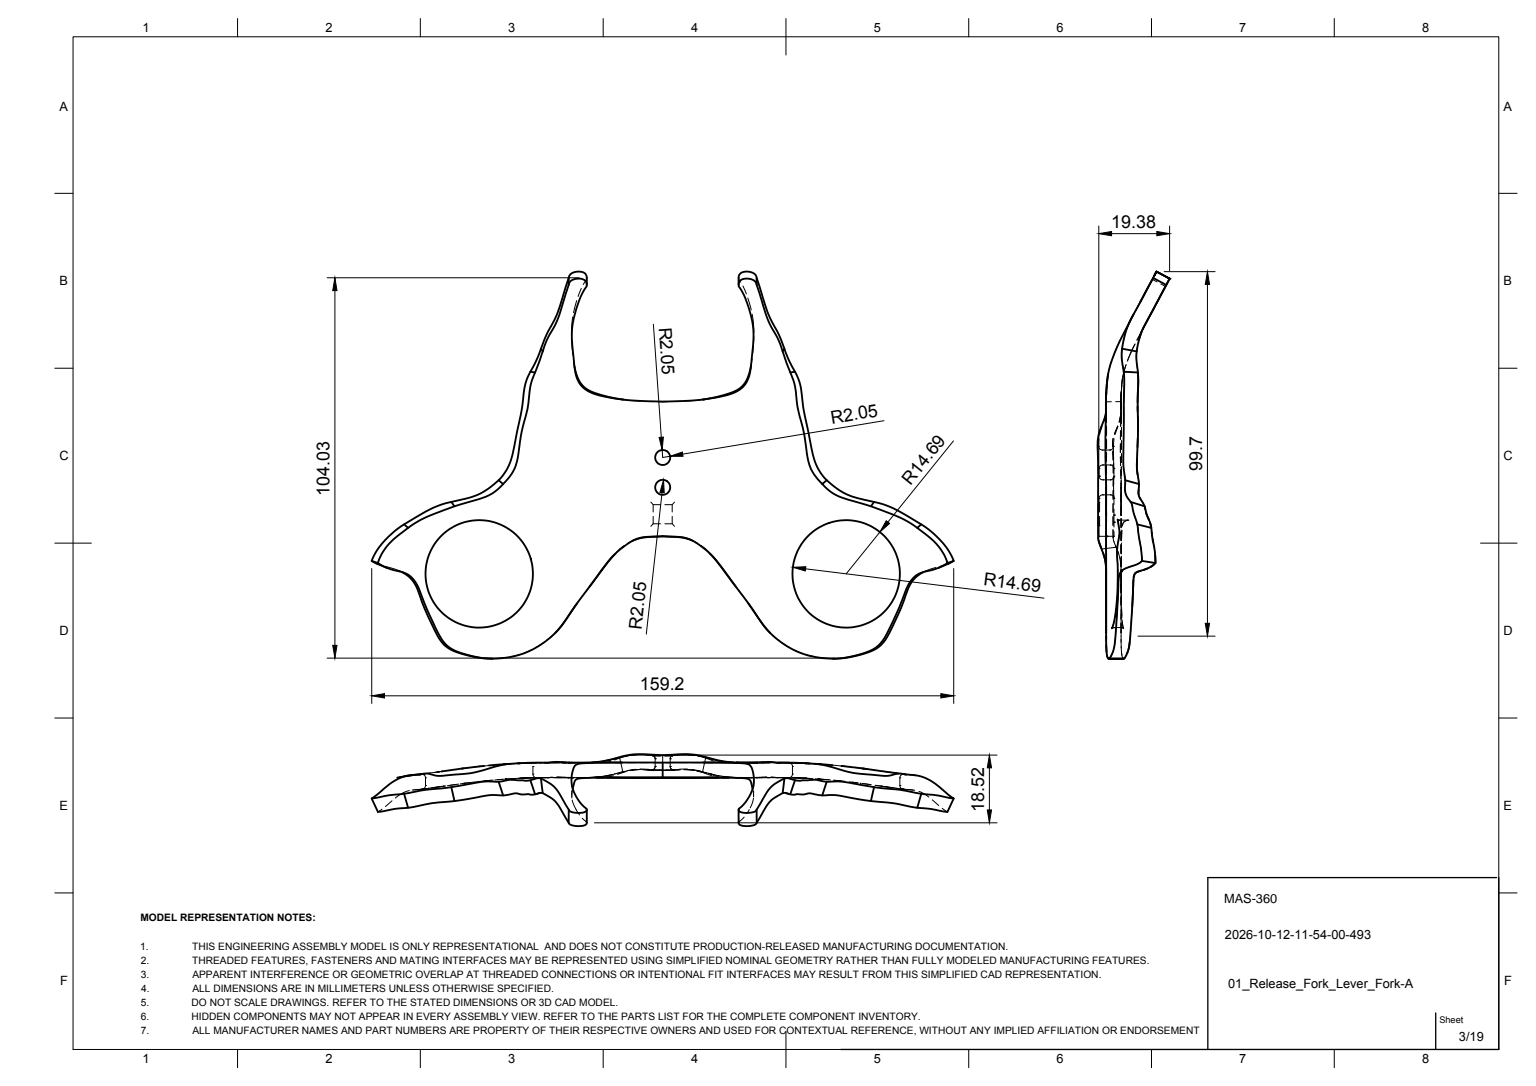
ISO-10303-21;
HEADER;
/* Generated by software containing ST-Developer
 * from STEP Tools, Inc. (www.steptools.com) 
 */

FILE_DESCRIPTION(
/* description */ (''),
/* implementation_level */ '2;1');

FILE_NAME(
/* name */ '01_Release_Fork_Lever_Fork-A.step',
/* time_stamp */ '2026-11-04T18:53:29-08:00',
/* author */ (''),
/* organization */ (''),
/* preprocessor_version */ 'ST-DEVELOPER v20.2',
/* originating_system */ 'Autodesk Translation Framework v15.17.0.0',
/* authorisation */ '');

FILE_SCHEMA (('AUTOMOTIVE_DESIGN { 1 0 10303 214 3 1 1 }'));
ENDSEC;

DATA;
#10=MECHANICAL_DESIGN_GEOMETRIC_PRESENTATION_REPRESENTATION('',(#1327),#100031);
#1291=SHAPE_REPRESENTATION_RELATIONSHIP('SRR','None',#100101,#1309);
#1309=ADVANCED_BREP_SHAPE_REPRESENTATION('',(#1345),#100013);
#1327=STYLED_ITEM('',(#100200),#1345);
#1345=MANIFOLD_SOLID_BREP('Body1',#20117);
#1363=PLANE('',#20342);
#1694=FACE_BOUND('',#6186,.T.);
#1695=FACE_BOUND('',#6187,.T.);
#1696=FACE_BOUND('',#6188,.T.);
#1697=FACE_BOUND('',#6189,.T.);
#1698=FACE_BOUND('',#6190,.T.);
#1699=FACE_BOUND('',#6193,.T.);
#1700=FACE_BOUND('',#6194,.T.);
#1701=FACE_BOUND('',#6195,.T.);
#1702=FACE_BOUND('',#6196,.T.);
#1811=ELLIPSE('',#20337,11.3271425811526,8.17324773003453);
#1812=ELLIPSE('',#20338,11.1453149409752,7.84400958474998);
#1980=LINE('',#28809,#3267);
#1981=LINE('',#55728,#3268);
#1982=LINE('',#56082,#3269);
#1983=LINE('',#56334,#3270);
#1984=LINE('',#56576,#3271);
#1985=LINE('',#56606,#3272);
#1986=LINE('',#56688,#3273);
#1987=LINE('',#56725,#3274);
#1988=LINE('',#56751,#3275);
#1989=LINE('',#56752,#3276);
#1990=LINE('',#56777,#3277);
#1991=LINE('',#56803,#3278);
#1992=LINE('',#56804,#3279);
#1993=LINE('',#56830,#3280);
#1994=LINE('',#56831,#3281);
#1995=LINE('',#56856,#3282);
#1996=LINE('',#56885,#3283);
#1997=LINE('',#56926,#3284);
#1998=LINE('',#56963,#3285);
#1999=LINE('',#56997,#3286);
#2000=LINE('',#56998,#3287);
#2001=LINE('',#57040,#3288);
#2002=LINE('',#57041,#3289);
#2003=LINE('',#57079,#3290);
#2004=LINE('',#57080,#3291);
#2005=LINE('',#57109,#3292);
#2006=LINE('',#57130,#3293);
#2007=LINE('',#57168,#3294);
#2008=LINE('',#57169,#3295);
#2009=LINE('',#57170,#3296);
#2010=LINE('',#57199,#3297);
#2011=LINE('',#57240,#3298);
#2012=LINE('',#57269,#3299);
#2013=LINE('',#57294,#3300);
#2014=LINE('',#57311,#3301);
#2015=LINE('',#57336,#3302);
#2016=LINE('',#57337,#3303);
#2017=LINE('',#57358,#3304);
#2018=LINE('',#57379,#3305);
#2019=LINE('',#57408,#3306);
#2020=LINE('',#57450,#3307);
#2021=LINE('',#57451,#3308);
#2022=LINE('',#57496,#3309);
#2023=LINE('',#57533,#3310);
#2024=LINE('',#57535,#3311);
#2025=LINE('',#57536,#3312);
#2026=LINE('',#57578,#3313);
#2027=LINE('',#57579,#3314);
#2028=LINE('',#57625,#3315);
#2029=LINE('',#57626,#3316);
#2030=LINE('',#57671,#3317);
#2031=LINE('',#57704,#3318);
#2032=LINE('',#57737,#3319);
#2033=LINE('',#57770,#3320);
#2034=LINE('',#57800,#3321);
#2035=LINE('',#57801,#3322);
#2036=LINE('',#57839,#3323);
#2037=LINE('',#57840,#3324);
#2038=LINE('',#57873,#3325);
#2039=LINE('',#57894,#3326);
#2040=LINE('',#57911,#3327);
#2041=LINE('',#57928,#3328);
#2042=LINE('',#57962,#3329);
#2043=LINE('',#57963,#3330);
#2044=LINE('',#57964,#3331);
#2045=LINE('',#58001,#3332);
#2046=LINE('',#58034,#3333);
#2047=LINE('',#58051,#3334);
#2048=LINE('',#58088,#3335);
#2049=LINE('',#58113,#3336);
#2050=LINE('',#58162,#3337);
#2051=LINE('',#58191,#3338);
#2052=LINE('',#58224,#3339);
#2053=LINE('',#58289,#3340);
#2054=LINE('',#58330,#3341);
#2055=LINE('',#58367,#3342);
#2056=LINE('',#58368,#3343);
#2057=LINE('',#58393,#3344);
#2058=LINE('',#58430,#3345);
#2059=LINE('',#58467,#3346);
#2060=LINE('',#58484,#3347);
#2061=LINE('',#58533,#3348);
#2062=LINE('',#58550,#3349);
#2063=LINE('',#58575,#3350);
#2064=LINE('',#58608,#3351);
#2065=LINE('',#58646,#3352);
#2066=LINE('',#58647,#3353);
#2067=LINE('',#58684,#3354);
#2068=LINE('',#58849,#3355);
#2069=LINE('',#59048,#3356);
#3267=VECTOR('',#22531,14.688);
#3268=VECTOR('',#22538,14.688);
#3269=VECTOR('',#22541,2.05);
#3270=VECTOR('',#22544,2.05);
#3271=VECTOR('',#22545,10.);
#3272=VECTOR('',#22546,10.);
#3273=VECTOR('',#22547,10.);
#3274=VECTOR('',#22548,10.);
#3275=VECTOR('',#22551,10.);
#3276=VECTOR('',#22552,10.);
#3277=VECTOR('',#22553,10.);
#3278=VECTOR('',#22554,10.);
#3279=VECTOR('',#22555,10.);
#3280=VECTOR('',#22556,10.);
#3281=VECTOR('',#22557,10.);
#3282=VECTOR('',#22558,10.);
#3283=VECTOR('',#22559,10.);
#3284=VECTOR('',#22560,10.);
#3285=VECTOR('',#22561,10.);
#3286=VECTOR('',#22562,10.);
#3287=VECTOR('',#22563,10.);
#3288=VECTOR('',#22564,10.);
#3289=VECTOR('',#22565,10.);
#3290=VECTOR('',#22566,10.);
#3291=VECTOR('',#22567,10.);
#3292=VECTOR('',#22568,10.);
#3293=VECTOR('',#22569,9.99999999999999);
#3294=VECTOR('',#22570,10.);
#3295=VECTOR('',#22571,10.);
#3296=VECTOR('',#22572,10.);
#3297=VECTOR('',#22573,10.);
#3298=VECTOR('',#22574,9.99999999999999);
#3299=VECTOR('',#22575,10.);
#3300=VECTOR('',#22576,10.);
#3301=VECTOR('',#22577,10.);
#3302=VECTOR('',#22578,9.99999999999999);
#3303=VECTOR('',#22579,10.);
#3304=VECTOR('',#22580,10.);
#3305=VECTOR('',#22581,10.);
#3306=VECTOR('',#22582,10.);
#3307=VECTOR('',#22583,10.);
#3308=VECTOR('',#22584,10.);
#3309=VECTOR('',#22585,10.);
#3310=VECTOR('',#22586,10.);
#3311=VECTOR('',#22587,10.);
#3312=VECTOR('',#22588,10.);
#3313=VECTOR('',#22589,10.);
#3314=VECTOR('',#22590,10.);
#3315=VECTOR('',#22591,10.);
#3316=VECTOR('',#22592,10.);
#3317=VECTOR('',#22593,10.);
#3318=VECTOR('',#22594,10.);
#3319=VECTOR('',#22595,10.);
#3320=VECTOR('',#22596,10.);
#3321=VECTOR('',#22597,10.);
#3322=VECTOR('',#22598,10.);
#3323=VECTOR('',#22599,10.);
#3324=VECTOR('',#22600,10.);
#3325=VECTOR('',#22601,10.);
#3326=VECTOR('',#22602,10.);
#3327=VECTOR('',#22603,10.);
#3328=VECTOR('',#22604,10.);
#3329=VECTOR('',#22605,10.);
#3330=VECTOR('',#22606,10.);
#3331=VECTOR('',#22607,10.);
#3332=VECTOR('',#22608,10.);
#3333=VECTOR('',#22609,10.);
#3334=VECTOR('',#22610,10.);
#3335=VECTOR('',#22611,10.);
#3336=VECTOR('',#22612,10.);
#3337=VECTOR('',#22613,10.);
#3338=VECTOR('',#22614,10.);
#3339=VECTOR('',#22615,10.);
#3340=VECTOR('',#22616,10.);
#3341=VECTOR('',#22617,10.);
#3342=VECTOR('',#22618,10.);
#3343=VECTOR('',#22619,10.);
#3344=VECTOR('',#22620,10.);
#3345=VECTOR('',#22621,10.);
#3346=VECTOR('',#22622,10.);
#3347=VECTOR('',#22623,10.);
#3348=VECTOR('',#22624,10.);
#3349=VECTOR('',#22625,10.);
#3350=VECTOR('',#22626,10.);
#3351=VECTOR('',#22627,10.);
#3352=VECTOR('',#22628,10.);
#3353=VECTOR('',#22629,10.);
#3354=VECTOR('',#22630,10.);
#3355=VECTOR('',#22631,10.);
#3356=VECTOR('',#22632,9.99999999999999);
#4554=CYLINDRICAL_SURFACE('',#20336,14.688);
#4555=CYLINDRICAL_SURFACE('',#20339,14.688);
#4556=CYLINDRICAL_SURFACE('',#20340,2.05);
#4557=CYLINDRICAL_SURFACE('',#20341,2.05);
#5026=FACE_OUTER_BOUND('',#6183,.T.);
#5027=FACE_OUTER_BOUND('',#6184,.T.);
#5028=FACE_OUTER_BOUND('',#6185,.T.);
#5029=FACE_OUTER_BOUND('',#6191,.T.);
#5030=FACE_OUTER_BOUND('',#6192,.T.);
#5031=FACE_OUTER_BOUND('',#6197,.T.);
#5032=FACE_OUTER_BOUND('',#6198,.T.);
#5033=FACE_OUTER_BOUND('',#6199,.T.);
#5034=FACE_OUTER_BOUND('',#6200,.T.);
#5035=FACE_OUTER_BOUND('',#6201,.T.);
#5036=FACE_OUTER_BOUND('',#6202,.T.);
#5037=FACE_OUTER_BOUND('',#6203,.T.);
#5038=FACE_OUTER_BOUND('',#6204,.T.);
#5039=FACE_OUTER_BOUND('',#6205,.T.);
#5040=FACE_OUTER_BOUND('',#6206,.T.);
#5041=FACE_OUTER_BOUND('',#6207,.T.);
#5042=FACE_OUTER_BOUND('',#6208,.T.);
#5043=FACE_OUTER_BOUND('',#6209,.T.);
#5044=FACE_OUTER_BOUND('',#6210,.T.);
#5045=FACE_OUTER_BOUND('',#6211,.T.);
#5046=FACE_OUTER_BOUND('',#6212,.T.);
#5047=FACE_OUTER_BOUND('',#6213,.T.);
#5048=FACE_OUTER_BOUND('',#6214,.T.);
#5049=FACE_OUTER_BOUND('',#6215,.T.);
#5050=FACE_OUTER_BOUND('',#6216,.T.);
#5051=FACE_OUTER_BOUND('',#6217,.T.);
#5052=FACE_OUTER_BOUND('',#6218,.T.);
#5053=FACE_OUTER_BOUND('',#6219,.T.);
#5054=FACE_OUTER_BOUND('',#6220,.T.);
#5055=FACE_OUTER_BOUND('',#6221,.T.);
#5056=FACE_OUTER_BOUND('',#6222,.T.);
#5057=FACE_OUTER_BOUND('',#6223,.T.);
#5058=FACE_OUTER_BOUND('',#6224,.T.);
#5059=FACE_OUTER_BOUND('',#6225,.T.);
#5060=FACE_OUTER_BOUND('',#6226,.T.);
#5061=FACE_OUTER_BOUND('',#6227,.T.);
#5062=FACE_OUTER_BOUND('',#6228,.T.);
#5063=FACE_OUTER_BOUND('',#6229,.T.);
#5064=FACE_OUTER_BOUND('',#6230,.T.);
#5065=FACE_OUTER_BOUND('',#6231,.T.);
#5066=FACE_OUTER_BOUND('',#6232,.T.);
#5067=FACE_OUTER_BOUND('',#6233,.T.);
#5068=FACE_OUTER_BOUND('',#6234,.T.);
#5069=FACE_OUTER_BOUND('',#6235,.T.);
#5070=FACE_OUTER_BOUND('',#6236,.T.);
#5071=FACE_OUTER_BOUND('',#6237,.T.);
#5072=FACE_OUTER_BOUND('',#6238,.T.);
#5073=FACE_OUTER_BOUND('',#6239,.T.);
#5074=FACE_OUTER_BOUND('',#6240,.T.);
#5075=FACE_OUTER_BOUND('',#6241,.T.);
#5076=FACE_OUTER_BOUND('',#6242,.T.);
#5077=FACE_OUTER_BOUND('',#6243,.T.);
#5078=FACE_OUTER_BOUND('',#6244,.T.);
#5079=FACE_OUTER_BOUND('',#6245,.T.);
#5080=FACE_OUTER_BOUND('',#6246,.T.);
#5081=FACE_OUTER_BOUND('',#6247,.T.);
#5082=FACE_OUTER_BOUND('',#6248,.T.);
#5083=FACE_OUTER_BOUND('',#6249,.T.);
#5084=FACE_OUTER_BOUND('',#6250,.T.);
#5085=FACE_OUTER_BOUND('',#6251,.T.);
#5086=FACE_OUTER_BOUND('',#6252,.T.);
#5087=FACE_OUTER_BOUND('',#6253,.T.);
#5088=FACE_OUTER_BOUND('',#6254,.T.);
#5089=FACE_OUTER_BOUND('',#6255,.T.);
#5090=FACE_OUTER_BOUND('',#6256,.T.);
#5091=FACE_OUTER_BOUND('',#6257,.T.);
#5092=FACE_OUTER_BOUND('',#6258,.T.);
#5093=FACE_OUTER_BOUND('',#6259,.T.);
#5094=FACE_OUTER_BOUND('',#6260,.T.);
#5095=FACE_OUTER_BOUND('',#6261,.T.);
#5096=FACE_OUTER_BOUND('',#6262,.T.);
#5097=FACE_OUTER_BOUND('',#6263,.T.);
#5098=FACE_OUTER_BOUND('',#6264,.T.);
#5099=FACE_OUTER_BOUND('',#6265,.T.);
#5100=FACE_OUTER_BOUND('',#6266,.T.);
#5101=FACE_OUTER_BOUND('',#6267,.T.);
#5102=FACE_OUTER_BOUND('',#6268,.T.);
#5103=FACE_OUTER_BOUND('',#6269,.T.);
#5104=FACE_OUTER_BOUND('',#6270,.T.);
#5105=FACE_OUTER_BOUND('',#6271,.T.);
#5106=FACE_OUTER_BOUND('',#6272,.T.);
#5107=FACE_OUTER_BOUND('',#6273,.T.);
#5108=FACE_OUTER_BOUND('',#6274,.T.);
#5109=FACE_OUTER_BOUND('',#6275,.T.);
#5110=FACE_OUTER_BOUND('',#6276,.T.);
#5111=FACE_OUTER_BOUND('',#6277,.T.);
#5112=FACE_OUTER_BOUND('',#6278,.T.);
#6183=EDGE_LOOP('',(#12899,#12900,#12901,#12902,#12903,#12904,#12905,#12906,
#12907,#12908,#12909,#12910,#12911,#12912,#12913));
#6184=EDGE_LOOP('',(#12914,#12915,#12916,#12917,#12918,#12919));
#6185=EDGE_LOOP('',(#12920,#12921,#12922,#12923,#12924,#12925,#12926,#12927,
#12928,#12929,#12930,#12931,#12932,#12933,#12934,#12935,#12936,#12937,#12938,
#12939,#12940,#12941,#12942,#12943,#12944,#12945,#12946,#12947,#12948,#12949,
#12950,#12951,#12952,#12953,#12954,#12955,#12956,#12957,#12958,#12959,#12960,
#12961,#12962,#12963,#12964,#12965,#12966,#12967,#12968,#12969,#12970,#12971,
#12972,#12973,#12974,#12975,#12976,#12977,#12978,#12979,#12980,#12981,#12982,
#12983,#12984,#12985,#12986,#12987));
#6186=EDGE_LOOP('',(#12988,#12989,#12990,#12991,#12992,#12993,#12994,#12995,
#12996,#12997,#12998));
#6187=EDGE_LOOP('',(#12999,#13000,#13001));
#6188=EDGE_LOOP('',(#13002,#13003,#13004,#13005,#13006,#13007,#13008,#13009,
#13010,#13011));
#6189=EDGE_LOOP('',(#13012,#13013,#13014));
#6190=EDGE_LOOP('',(#13015,#13016,#13017,#13018,#13019,#13020,#13021,#13022,
#13023,#13024,#13025));
#6191=EDGE_LOOP('',(#13026,#13027,#13028,#13029,#13030,#13031,#13032,#13033,
#13034,#13035,#13036,#13037,#13038,#13039,#13040));
#6192=EDGE_LOOP('',(#13041,#13042,#13043,#13044,#13045,#13046,#13047,#13048,
#13049,#13050,#13051,#13052,#13053,#13054,#13055,#13056,#13057,#13058,#13059,
#13060,#13061,#13062,#13063,#13064,#13065,#13066,#13067,#13068,#13069,#13070,
#13071,#13072,#13073,#13074,#13075,#13076,#13077,#13078,#13079,#13080,#13081,
#13082,#13083,#13084,#13085,#13086,#13087,#13088,#13089,#13090,#13091,#13092,
#13093,#13094,#13095,#13096,#13097,#13098,#13099,#13100,#13101,#13102,#13103,
#13104,#13105,#13106,#13107,#13108));
#6193=EDGE_LOOP('',(#13109,#13110,#13111,#13112,#13113,#13114,#13115,#13116,
#13117,#13118,#13119));
#6194=EDGE_LOOP('',(#13120,#13121,#13122));
#6195=EDGE_LOOP('',(#13123,#13124,#13125));
#6196=EDGE_LOOP('',(#13126,#13127,#13128,#13129,#13130,#13131,#13132,#13133,
#13134,#13135,#13136));
#6197=EDGE_LOOP('',(#13137,#13138,#13139,#13140,#13141,#13142,#13143,#13144,
#13145,#13146,#13147,#13148,#13149,#13150,#13151));
#6198=EDGE_LOOP('',(#13152,#13153,#13154,#13155,#13156,#13157));
#6199=EDGE_LOOP('',(#13158,#13159,#13160,#13161,#13162,#13163,#13164,#13165,
#13166,#13167,#13168,#13169,#13170,#13171,#13172));
#6200=EDGE_LOOP('',(#13173,#13174,#13175,#13176,#13177,#13178,#13179));
#6201=EDGE_LOOP('',(#13180,#13181,#13182,#13183,#13184,#13185));
#6202=EDGE_LOOP('',(#13186,#13187,#13188,#13189,#13190,#13191,#13192));
#6203=EDGE_LOOP('',(#13193,#13194,#13195,#13196,#13197,#13198,#13199));
#6204=EDGE_LOOP('',(#13200,#13201,#13202,#13203,#13204,#13205));
#6205=EDGE_LOOP('',(#13206,#13207,#13208,#13209,#13210,#13211,#13212));
#6206=EDGE_LOOP('',(#13213,#13214,#13215,#13216));
#6207=EDGE_LOOP('',(#13217,#13218,#13219,#13220,#13221));
#6208=EDGE_LOOP('',(#13222,#13223,#13224,#13225,#13226));
#6209=EDGE_LOOP('',(#13227,#13228,#13229,#13230,#13231,#13232,#13233,#13234));
#6210=EDGE_LOOP('',(#13235,#13236,#13237,#13238));
#6211=EDGE_LOOP('',(#13239,#13240,#13241,#13242));
#6212=EDGE_LOOP('',(#13243,#13244,#13245,#13246));
#6213=EDGE_LOOP('',(#13247,#13248,#13249,#13250,#13251));
#6214=EDGE_LOOP('',(#13252,#13253,#13254,#13255,#13256,#13257));
#6215=EDGE_LOOP('',(#13258,#13259,#13260,#13261,#13262));
#6216=EDGE_LOOP('',(#13263,#13264,#13265,#13266));
#6217=EDGE_LOOP('',(#13267,#13268,#13269,#13270));
#6218=EDGE_LOOP('',(#13271,#13272,#13273,#13274));
#6219=EDGE_LOOP('',(#13275,#13276,#13277,#13278,#13279));
#6220=EDGE_LOOP('',(#13280,#13281,#13282,#13283,#13284,#13285));
#6221=EDGE_LOOP('',(#13286,#13287,#13288,#13289,#13290,#13291));
#6222=EDGE_LOOP('',(#13292,#13293,#13294,#13295,#13296));
#6223=EDGE_LOOP('',(#13297,#13298,#13299,#13300));
#6224=EDGE_LOOP('',(#13301,#13302,#13303,#13304,#13305));
#6225=EDGE_LOOP('',(#13306,#13307,#13308,#13309));
#6226=EDGE_LOOP('',(#13310,#13311,#13312,#13313));
#6227=EDGE_LOOP('',(#13314,#13315,#13316,#13317));
#6228=EDGE_LOOP('',(#13318,#13319,#13320,#13321));
#6229=EDGE_LOOP('',(#13322,#13323,#13324,#13325));
#6230=EDGE_LOOP('',(#13326,#13327,#13328,#13329));
#6231=EDGE_LOOP('',(#13330,#13331,#13332,#13333));
#6232=EDGE_LOOP('',(#13334,#13335,#13336,#13337));
#6233=EDGE_LOOP('',(#13338,#13339,#13340,#13341));
#6234=EDGE_LOOP('',(#13342,#13343,#13344,#13345,#13346));
#6235=EDGE_LOOP('',(#13347,#13348,#13349,#13350,#13351));
#6236=EDGE_LOOP('',(#13352,#13353,#13354,#13355,#13356));
#6237=EDGE_LOOP('',(#13357,#13358,#13359,#13360,#13361,#13362));
#6238=EDGE_LOOP('',(#13363,#13364,#13365,#13366,#13367,#13368));
#6239=EDGE_LOOP('',(#13369,#13370,#13371,#13372,#13373));
#6240=EDGE_LOOP('',(#13374,#13375,#13376,#13377));
#6241=EDGE_LOOP('',(#13378,#13379,#13380,#13381));
#6242=EDGE_LOOP('',(#13382,#13383,#13384,#13385));
#6243=EDGE_LOOP('',(#13386,#13387,#13388,#13389,#13390));
#6244=EDGE_LOOP('',(#13391,#13392,#13393,#13394,#13395,#13396));
#6245=EDGE_LOOP('',(#13397,#13398,#13399,#13400,#13401));
#6246=EDGE_LOOP('',(#13402,#13403,#13404,#13405));
#6247=EDGE_LOOP('',(#13406,#13407,#13408,#13409));
#6248=EDGE_LOOP('',(#13410,#13411,#13412,#13413));
#6249=EDGE_LOOP('',(#13414,#13415,#13416,#13417,#13418));
#6250=EDGE_LOOP('',(#13419,#13420,#13421,#13422));
#6251=EDGE_LOOP('',(#13423,#13424,#13425,#13426));
#6252=EDGE_LOOP('',(#13427,#13428,#13429,#13430));
#6253=EDGE_LOOP('',(#13431,#13432,#13433,#13434));
#6254=EDGE_LOOP('',(#13435,#13436,#13437,#13438));
#6255=EDGE_LOOP('',(#13439,#13440,#13441,#13442));
#6256=EDGE_LOOP('',(#13443,#13444,#13445,#13446));
#6257=EDGE_LOOP('',(#13447,#13448,#13449,#13450));
#6258=EDGE_LOOP('',(#13451,#13452,#13453,#13454));
#6259=EDGE_LOOP('',(#13455,#13456,#13457,#13458));
#6260=EDGE_LOOP('',(#13459,#13460,#13461,#13462));
#6261=EDGE_LOOP('',(#13463,#13464,#13465,#13466));
#6262=EDGE_LOOP('',(#13467,#13468,#13469,#13470));
#6263=EDGE_LOOP('',(#13471,#13472,#13473,#13474));
#6264=EDGE_LOOP('',(#13475,#13476,#13477,#13478));
#6265=EDGE_LOOP('',(#13479,#13480,#13481,#13482));
#6266=EDGE_LOOP('',(#13483,#13484,#13485,#13486));
#6267=EDGE_LOOP('',(#13487,#13488,#13489,#13490));
#6268=EDGE_LOOP('',(#13491,#13492,#13493,#13494));
#6269=EDGE_LOOP('',(#13495,#13496,#13497,#13498,#13499));
#6270=EDGE_LOOP('',(#13500,#13501,#13502,#13503,#13504));
#6271=EDGE_LOOP('',(#13505,#13506,#13507,#13508));
#6272=EDGE_LOOP('',(#13509,#13510,#13511,#13512,#13513));
#6273=EDGE_LOOP('',(#13514,#13515,#13516,#13517));
#6274=EDGE_LOOP('',(#13518,#13519,#13520,#13521));
#6275=EDGE_LOOP('',(#13522,#13523,#13524,#13525));
#6276=EDGE_LOOP('',(#13526,#13527,#13528,#13529,#13530));
#6277=EDGE_LOOP('',(#13531,#13532,#13533,#13534));
#6278=EDGE_LOOP('',(#13535,#13536,#13537,#13538));
#7457=B_SPLINE_CURVE_WITH_KNOTS('',3,(#28468,#28469,#28470,#28471,#28472,
#28473),.UNSPECIFIED.,.F.,.F.,(4,1,1,4),(-0.999999999999995,-0.571428571428571,
-0.285714285714286,0.),.UNSPECIFIED.);
#7458=B_SPLINE_CURVE_WITH_KNOTS('',3,(#28475,#28476,#28477,#28478,#28479,
#28480,#28481,#28482),.UNSPECIFIED.,.F.,.F.,(4,2,2,4),(-13.0076216717983,
-12.6762562420903,-11.8531689108674,-11.7197155434785),.UNSPECIFIED.);
#7459=B_SPLINE_CURVE_WITH_KNOTS('',3,(#28483,#28484,#28485,#28486,#28487,
#28488,#28489,#28490,#28491,#28492,#28493,#28494,#28495,#28496,#28497,#28498,
#28499,#28500,#28501,#28502,#28503,#28504,#28505,#28506,#28507,#28508,#28509,
#28510,#28511,#28512,#28513,#28514,#28515,#28516,#28517,#28518,#28519,#28520,
#28521,#28522,#28523),.UNSPECIFIED.,.F.,.F.,(4,2,2,1,1,2,2,1,2,1,1,1,2,
1,1,1,2,1,1,1,1,1,1,1,1,1,1,2,1,1,4),(-11.7197155434785,-11.05258106389,
-10.1188927640438,-8.47830334468407,-7.04278760274435,-6.83771392532439,
-5.90055842268743,-5.54885349043522,-5.09666143468238,-4.98988621289018,
-4.88311099109797,-4.50939771482526,-4.24245966034475,-3.88978669781647,
-3.67818292029951,-3.43131184652972,-3.11390618025428,-3.0769781504351,
-2.96619406097756,-2.81848194170084,-2.7076978522433,-2.5230577031474,-1.93220922604053,
-1.78449710676381,-1.74756907694463,-1.34136074893366,-1.04593651038022,
-0.750512271826782,-0.60979122085926,-0.469070169891739,0.),
 .UNSPECIFIED.);
#7460=B_SPLINE_CURVE_WITH_KNOTS('',3,(#28525,#28526,#28527,#28528,#28529,
#28530),.UNSPECIFIED.,.F.,.F.,(4,1,1,4),(0.,0.469070169891739,0.60979122085926,
0.750512271826782),.UNSPECIFIED.);
#7461=B_SPLINE_CURVE_WITH_KNOTS('',3,(#28532,#28533,#28534,#28535,#28536,
#28537,#28538,#28539,#28540,#28541,#28542,#28543,#28544,#28545,#28546,#28547,
#28548,#28549,#28550,#28551,#28552,#28553,#28554,#28555,#28556,#28557,#28558,
#28559,#28560,#28561,#28562,#28563,#28564,#28565,#28566,#28567,#28568,#28569,
#28570,#28571,#28572,#28573,#28574,#28575,#28576,#28577,#28578,#28579,#28580,
#28581,#28582,#28583,#28584,#28585,#28586,#28587,#28588,#28589,#28590,#28591,
#28592,#28593,#28594,#28595,#28596,#28597,#28598,#28599,#28600,#28601,#28602,
#28603,#28604,#28605,#28606,#28607,#28608,#28609,#28610,#28611,#28612,#28613,
#28614,#28615,#28616,#28617,#28618,#28619,#28620,#28621,#28622,#28623,#28624,
#28625,#28626,#28627,#28628,#28629,#28630,#28631,#28632,#28633,#28634,#28635,
#28636,#28637,#28638,#28639,#28640,#28641,#28642,#28643,#28644,#28645,#28646,
#28647,#28648,#28649,#28650,#28651,#28652,#28653,#28654,#28655,#28656,#28657,
#28658,#28659,#28660,#28661,#28662,#28663,#28664,#28665,#28666,#28667,#28668,
#28669,#28670,#28671,#28672,#28673,#28674,#28675,#28676,#28677,#28678,#28679,
#28680,#28681,#28682,#28683,#28684,#28685,#28686,#28687,#28688,#28689,#28690,
#28691,#28692,#28693,#28694,#28695,#28696,#28697,#28698,#28699,#28700,#28701,
#28702,#28703,#28704,#28705,#28706),.UNSPECIFIED.,.F.,.F.,(4,3,3,3,3,3,
3,3,3,3,3,3,3,3,3,3,3,3,3,3,3,3,3,3,3,3,3,3,3,3,3,3,3,3,3,3,3,3,3,3,3,3,
3,3,3,3,3,3,3,3,3,3,3,3,3,3,3,3,4),(0.750707263401336,0.751073491522809,
0.770788600839354,0.797141727621928,0.801285493755856,0.847209334720936,
0.851576628686437,0.892702424300306,0.909155014790277,0.945842604423156,
0.959283328964777,0.973653029900114,1.02857295555953,1.04593651038022,1.10213659378528,
1.15946870078418,1.21910603297729,1.25714745759372,1.32249197142089,1.33169604227939,
1.34136074893366,1.40008364166717,1.46200856506941,1.53008670118818,1.60161378753395,
1.67565478609667,1.72643723062008,1.74756907694463,1.78449710676381,1.85969939535229,
1.93220922604053,2.0009848480779,2.06808195029472,2.1044635537539,2.17677612815408,
2.25426089464543,2.33537778995665,2.42383992559276,2.48665348358685,2.5230577031474,
2.55048767867042,2.63206152994388,2.7076978522433,2.81035120800203,2.81848194170084,
2.86928839618313,2.89438186295904,2.94470693815227,2.96619406097756,2.99737852476675,
3.02773642991363,3.05710875945002,3.07552489670663,3.0769781504351,3.08925644295071,
3.10116317170119,3.11177854192958,3.11306990045168,3.11390618025428),
 .UNSPECIFIED.);
#7462=B_SPLINE_CURVE_WITH_KNOTS('',3,(#28708,#28709,#28710,#28711,#28712,
#28713,#28714),.UNSPECIFIED.,.F.,.F.,(4,1,1,1,4),(3.1140516289664,3.43131184652972,
3.67818292029951,3.88978669781647,4.24245966034475),.UNSPECIFIED.);
#7463=B_SPLINE_CURVE_WITH_KNOTS('',3,(#28716,#28717,#28718,#28719,#28720,
#28721,#28722),.UNSPECIFIED.,.F.,.F.,(4,1,1,1,4),(4.24281193045545,4.50939771482526,
4.88311099109797,4.98988621289018,5.09562751764158),.UNSPECIFIED.);
#7464=B_SPLINE_CURVE_WITH_KNOTS('',3,(#28724,#28725,#28726,#28727,#28728,
#28729,#28730,#28731,#28732,#28733,#28734,#28735,#28736,#28737,#28738,#28739,
#28740,#28741,#28742,#28743,#28744,#28745,#28746,#28747,#28748,#28749,#28750,
#28751,#28752,#28753,#28754,#28755,#28756,#28757,#28758,#28759,#28760,#28761,
#28762,#28763,#28764,#28765,#28766,#28767,#28768,#28769,#28770,#28771,#28772,
#28773,#28774,#28775),.UNSPECIFIED.,.F.,.F.,(4,3,3,3,3,3,3,3,3,3,3,3,3,
3,3,3,3,4),(5.09666143468238,5.15433284711348,5.21357578985293,5.27511503720701,
5.34195092279717,5.41296344455248,5.48882370921057,5.4948675217662,5.54885349043522,
5.62257616633349,5.69588741785513,5.71679169498887,5.78286561201951,5.79781169784479,
5.83813276584378,5.84909385748713,5.87479360889014,5.90049336029315),
 .UNSPECIFIED.);
#7465=B_SPLINE_CURVE_WITH_KNOTS('',3,(#28777,#28778,#28779,#28780),
 .UNSPECIFIED.,.F.,.F.,(4,4),(5.90055842268743,6.83750114647945),
 .UNSPECIFIED.);
#7466=B_SPLINE_CURVE_WITH_KNOTS('',3,(#28782,#28783,#28784,#28785,#28786,
#28787),.UNSPECIFIED.,.F.,.F.,(4,1,1,4),(6.83771392532439,7.04278760274435,
8.47830334468407,10.1186669136909),.UNSPECIFIED.);
#7467=B_SPLINE_CURVE_WITH_KNOTS('',3,(#28789,#28790,#28791,#28792),
 .UNSPECIFIED.,.F.,.F.,(4,4),(10.1188927640438,11.05258106389),
 .UNSPECIFIED.);
#7468=B_SPLINE_CURVE_WITH_KNOTS('',3,(#28794,#28795,#28796,#28797),
 .UNSPECIFIED.,.F.,.F.,(4,4),(11.0525853415176,11.8531689108674),
 .UNSPECIFIED.);
#7469=B_SPLINE_CURVE_WITH_KNOTS('',3,(#28799,#28800,#28801,#28802),
 .UNSPECIFIED.,.F.,.F.,(4,4),(11.8532319611187,12.6762562420903),
 .UNSPECIFIED.);
#7470=B_SPLINE_CURVE_WITH_KNOTS('',3,(#28803,#28804,#28805,#28806),
 .UNSPECIFIED.,.F.,.F.,(4,4),(12.6763300349415,13.0076216717983),
 .UNSPECIFIED.);
#7471=B_SPLINE_CURVE_WITH_KNOTS('',3,(#28811,#28812,#28813,#28814,#28815,
#28816,#28817,#28818,#28819,#28820,#28821,#28822,#28823,#28824,#28825,#28826,
#28827,#28828,#28829,#28830,#28831,#28832,#28833,#28834,#28835,#28836,#28837,
#28838,#28839,#28840,#28841,#28842),.UNSPECIFIED.,.F.,.F.,(4,1,1,1,2,1,
1,1,1,2,1,1,1,2,1,1,1,2,2,1,2,2,4),(-9.55960092302324,-9.1896794456085,
-8.81975796819377,-8.44983649077903,-8.0799150133643,-8.03266253512535,
-7.98541005688641,-7.89090510040853,-7.70189518745276,-7.32387536154123,
-7.17881214312514,-7.03374892470906,-6.88868570629297,-6.74362248787689,
-6.67050437063,-6.59738625338311,-6.45115001888933,-6.15867754990177,-5.47160541199434,
-4.26766323501505,-3.06372105803577,-2.37819810334092,-1.88848372186453),
 .UNSPECIFIED.);
#7472=B_SPLINE_CURVE_WITH_KNOTS('',3,(#28843,#28844,#28845,#28846,#28847,
#28848,#28849,#28850,#28851,#28852,#28853,#28854,#28855),.UNSPECIFIED.,
 .F.,.F.,(4,2,2,1,2,1,1,4),(-1.88848372186453,-1.79056374069951,-1.18667868852568,
-0.800342864550781,-0.414007040575882,-0.310505280431912,-0.207003520287941,
0.),.UNSPECIFIED.);
#7473=B_SPLINE_CURVE_WITH_KNOTS('',3,(#38650,#38651,#38652,#38653,#38654,
#38655,#38656,#38657,#38658),.UNSPECIFIED.,.F.,.F.,(4,1,1,1,1,1,4),(0.,
0.208981284264062,0.626943852792187,0.835925137056249,1.04490642132031,
1.25388770558437,1.46286898984844),.UNSPECIFIED.);
#7474=B_SPLINE_CURVE_WITH_KNOTS('',3,(#38660,#38661,#38662,#38663,#38664,
#38665,#38666,#38667,#38668),.UNSPECIFIED.,.F.,.F.,(4,1,1,1,1,1,4),(1.46286898984844,
1.57811142102339,1.80859628337331,1.92383871454827,2.03908114572322,2.15432357689818,
2.26956600807314),.UNSPECIFIED.);
#7475=B_SPLINE_CURVE_WITH_KNOTS('',3,(#38670,#38671,#38672,#38673,#38674,
#38675,#38676,#38677,#38678,#38679,#38680,#38681,#38682,#38683,#38684,#38685,
#38686,#38687,#38688,#38689,#38690,#38691,#38692,#38693,#38694,#38695,#38696,
#38697,#38698,#38699,#38700,#38701,#38702,#38703,#38704,#38705,#38706,#38707,
#38708,#38709,#38710,#38711,#38712,#38713,#38714,#38715,#38716,#38717,#38718,
#38719,#38720,#38721,#38722,#38723,#38724,#38725,#38726,#38727,#38728,#38729,
#38730,#38731,#38732,#38733,#38734,#38735,#38736,#38737,#38738,#38739,#38740,
#38741,#38742,#38743,#38744,#38745,#38746,#38747,#38748,#38749,#38750,#38751,
#38752,#38753,#38754,#38755,#38756,#38757,#38758,#38759,#38760,#38761,#38762,
#38763),.UNSPECIFIED.,.F.,.F.,(4,3,3,3,3,3,3,3,3,3,3,3,3,3,3,3,3,3,3,3,
3,3,3,3,3,3,3,3,3,3,3,4),(2.26956600807314,2.31868576460897,2.36442460789209,
2.40351503906262,2.42718620051329,2.44122087175842,2.44260547023316,2.45341326627912,
2.46020489685124,2.46598765674336,2.4975277476721,2.51361070216978,2.52906783860085,
2.54765629078654,2.56502674195218,2.57656452038008,2.61240308621125,2.61582222590599,
2.62445098833827,2.62880283765034,2.63139315501457,2.63314063742138,2.65910316373393,
2.6848523253642,2.7024591242981,2.70904066964155,2.74512184182599,2.77027473318896,
2.78990851485099,2.83207741398362,2.86861528379491,2.87518401914012),
 .UNSPECIFIED.);
#7476=B_SPLINE_CURVE_WITH_KNOTS('',3,(#38765,#38766,#38767,#38768,#38769,
#38770,#38771,#38772,#38773,#38774),.UNSPECIFIED.,.F.,.F.,(4,2,2,2,4),(7.35574899264912E-13,
0.182950620511092,0.366672640482893,0.532787709398147,0.700945883028127),
 .UNSPECIFIED.);
#7477=B_SPLINE_CURVE_WITH_KNOTS('',3,(#38776,#38777,#38778,#38779,#38780,
#38781),.UNSPECIFIED.,.F.,.F.,(4,2,4),(0.,0.425557203103372,0.889753425869099),
 .UNSPECIFIED.);
#7478=B_SPLINE_CURVE_WITH_KNOTS('',3,(#38783,#38784,#38785,#38786,#38787,
#38788,#38789,#38790,#38791,#38792,#38793,#38794),.UNSPECIFIED.,.F.,.F.,
(4,1,1,1,1,1,1,1,1,4),(4.48918216137468,4.66429138725693,4.75184600019805,
4.83940061313917,5.53983751666817,5.89005596843266,6.06516519431491,6.24027442019716,
6.59049287196166,6.94071132372615),.UNSPECIFIED.);
#7479=B_SPLINE_CURVE_WITH_KNOTS('',3,(#38796,#38797,#38798,#38799),
 .UNSPECIFIED.,.F.,.F.,(4,4),(6.94071132372615,7.92790045161141),
 .UNSPECIFIED.);
#7480=B_SPLINE_CURVE_WITH_KNOTS('',3,(#38801,#38802,#38803,#38804,#38805,
#38806,#38807,#38808,#38809),.UNSPECIFIED.,.F.,.F.,(4,1,1,1,1,1,4),(7.92790045161141,
8.77117777664964,9.19281643916875,9.61445510168786,10.036093764207,10.4577324267261,
10.8793710892452),.UNSPECIFIED.);
#7481=B_SPLINE_CURVE_WITH_KNOTS('',3,(#38811,#38812,#38813,#38814,#38815,
#38816,#38817,#38818),.UNSPECIFIED.,.F.,.F.,(4,2,2,4),(3.5904242252203E-11,
0.260393756917535,0.343613662591379,0.431907573073398),.UNSPECIFIED.);
#7482=B_SPLINE_CURVE_WITH_KNOTS('',3,(#38820,#38821,#38822,#38823,#38824,
#38825),.UNSPECIFIED.,.F.,.F.,(4,1,1,4),(12.3501209228208,13.0134488895805,
13.455667534087,13.897886155505),.UNSPECIFIED.);
#7483=B_SPLINE_CURVE_WITH_KNOTS('',3,(#38827,#38828,#38829,#38830,#38831,
#38832,#38833,#38834,#38835,#38836,#38837,#38838,#38839,#38840,#38841,#38842,
#38843,#38844,#38845,#38846,#38847,#38848,#38849,#38850,#38851,#38852,#38853,
#38854,#38855,#38856,#38857,#38858,#38859,#38860,#38861,#38862,#38863,#38864,
#38865,#38866,#38867,#38868,#38869,#38870,#38871,#38872,#38873,#38874,#38875,
#38876,#38877,#38878,#38879,#38880,#38881,#38882,#38883,#38884,#38885,#38886,
#38887,#38888,#38889,#38890,#38891,#38892,#38893,#38894,#38895,#38896,#38897,
#38898,#38899,#38900,#38901,#38902,#38903,#38904,#38905,#38906,#38907,#38908,
#38909,#38910,#38911,#38912,#38913,#38914,#38915,#38916,#38917,#38918,#38919,
#38920,#38921,#38922,#38923,#38924,#38925,#38926,#38927,#38928,#38929,#38930,
#38931,#38932,#38933,#38934,#38935),.UNSPECIFIED.,.F.,.F.,(4,3,3,3,3,3,
3,3,3,3,3,3,3,3,3,3,3,3,3,3,3,3,3,3,3,3,3,3,3,3,3,3,3,3,3,3,4),(13.8978861785935,
13.9380361760921,13.9783662868224,14.0186963975526,14.0811238320635,14.1320902001938,
14.2193450517567,14.309644201861,14.3469219867698,14.4395096610908,14.5292417963811,
14.6174410389455,14.7034058274742,14.7629556872226,14.8165856516271,14.862262798083,
14.9374055100664,15.0109004941316,15.0838111850265,15.1563912070055,15.1837216712462,
15.255912890478,15.3277216735112,15.398965330592,15.4693404586375,15.5051805444094,
15.5645429684139,15.6227879721599,15.6376791692706,15.6977923210042,15.7622158692884,
15.8266394175726,15.8921244883675,15.960846906809,16.0317141617619,16.1063877532203,
16.1480982806684),.UNSPECIFIED.);
#7484=B_SPLINE_CURVE_WITH_KNOTS('',3,(#38937,#38938,#38939,#38940,#38941,
#38942,#38943,#38944),.UNSPECIFIED.,.F.,.F.,(4,1,1,1,1,4),(16.1480989104869,
17.1122318399124,17.4336096896379,17.7549875393634,17.9156764642262,18.3977432388145),
 .UNSPECIFIED.);
#7485=B_SPLINE_CURVE_WITH_KNOTS('',3,(#38946,#38947,#38948,#38949,#38950),
 .UNSPECIFIED.,.F.,.F.,(4,1,4),(-27.614177239717,-26.6900911654903,-25.4579763998548),
 .UNSPECIFIED.);
#7486=B_SPLINE_CURVE_WITH_KNOTS('',3,(#38952,#38953,#38954,#38955,#38956,
#38957,#38958,#38959,#38960,#38961,#38962,#38963,#38964,#38965,#38966,#38967,
#38968,#38969,#38970,#38971,#38972,#38973,#38974,#38975,#38976,#38977,#38978,
#38979,#38980,#38981,#38982,#38983,#38984,#38985,#38986,#38987,#38988,#38989,
#38990,#38991,#38992,#38993,#38994,#38995,#38996,#38997,#38998,#38999,#39000,
#39001,#39002,#39003,#39004,#39005,#39006,#39007,#39008,#39009,#39010,#39011,
#39012,#39013,#39014,#39015,#39016,#39017,#39018,#39019,#39020,#39021,#39022,
#39023,#39024,#39025,#39026,#39027,#39028,#39029,#39030,#39031,#39032,#39033,
#39034,#39035,#39036,#39037,#39038,#39039,#39040,#39041,#39042,#39043,#39044,
#39045,#39046,#39047,#39048,#39049,#39050,#39051),.UNSPECIFIED.,.F.,.F.,
(4,3,3,3,3,3,3,3,3,3,3,3,3,3,3,3,3,3,3,3,3,3,3,3,3,3,3,3,3,3,3,3,3,4),(-25.4579763998548,
-25.3889893896019,-25.3213768105525,-25.2555098807919,-25.2220083007855,
-25.1146742426374,-25.010880056723,-24.9872519938033,-24.8083237297656,
-24.6450684781262,-24.5215312467475,-24.3975168143727,-24.1846371236323,
-23.9923963326571,-23.8672870216316,-23.7144002286166,-23.6130418747886,
-23.4679899517189,-23.3238431903892,-23.1802452769976,-23.1590824865092,
-23.0157070639962,-22.8650467350538,-22.8068274361495,-22.7212423399242,
-22.5325850737667,-22.3597054148946,-22.2394602855688,-22.0850152108554,
-21.9930212690266,-21.8160728505053,-21.7959801689209,-21.7477190509971,
-21.7463678515301),.UNSPECIFIED.);
#7487=B_SPLINE_CURVE_WITH_KNOTS('',3,(#39053,#39054,#39055,#39056,#39057,
#39058,#39059,#39060,#39061),.UNSPECIFIED.,.F.,.F.,(4,1,1,1,1,1,4),(-21.7463678506673,
-21.0251854504292,-19.5828206499531,-18.861638249715,-18.140455849477,-17.4192734492389,
-16.6980910490008),.UNSPECIFIED.);
#7488=B_SPLINE_CURVE_WITH_KNOTS('',3,(#39063,#39064,#39065,#39066,#39067,
#39068,#39069,#39070,#39071,#39072),.UNSPECIFIED.,.F.,.F.,(4,1,1,1,1,1,
1,4),(-16.6980910490008,-16.0242682824596,-14.6766227493771,-14.0027999828359,
-13.3289772162947,-12.6551544497534,-12.3182430664828,-11.9813316832122),
 .UNSPECIFIED.);
#7489=B_SPLINE_CURVE_WITH_KNOTS('',3,(#39074,#39075,#39076,#39077,#39078,
#39079,#39080,#39081),.UNSPECIFIED.,.F.,.F.,(4,1,1,1,1,4),(-11.9813316832122,
-11.8608434310554,-11.7403551788986,-11.2584021702716,-10.7764491616445,
-10.2944961530174),.UNSPECIFIED.);
#7490=B_SPLINE_CURVE_WITH_KNOTS('',3,(#39083,#39084,#39085,#39086,#39087,
#39088,#39089,#39090,#39091),.UNSPECIFIED.,.F.,.F.,(4,1,1,1,1,1,4),(-10.2944961530174,
-9.9233650238383,-9.5522338946592,-9.18110276548009,-8.43884050712189,-8.06770937794279,
-7.69657824876369),.UNSPECIFIED.);
#7491=B_SPLINE_CURVE_WITH_KNOTS('',3,(#39093,#39094,#39095,#39096,#39097,
#39098,#39099,#39100,#39101,#39102),.UNSPECIFIED.,.F.,.F.,(4,1,1,1,1,1,
1,4),(-7.69657824876369,-7.30181972429585,-7.10444046206193,-6.90706119982801,
-6.80837156871105,-6.70968193759409,-6.51230267536017,-6.31492341312625),
 .UNSPECIFIED.);
#7492=B_SPLINE_CURVE_WITH_KNOTS('',3,(#39104,#39105,#39106,#39107,#39108,
#39109,#39110,#39111,#39112,#39113),.UNSPECIFIED.,.F.,.F.,(4,2,2,2,4),(6.84506442931943E-11,
0.102096969345333,0.201193147379825,0.268916988037693,0.641886390881406),
 .UNSPECIFIED.);
#7493=B_SPLINE_CURVE_WITH_KNOTS('',3,(#39115,#39116,#39117,#39118,#39119,
#39120),.UNSPECIFIED.,.F.,.F.,(4,1,1,4),(-5.24963521037055,-5.08288401419063,
-4.74938156648641,-4.08237667107798),.UNSPECIFIED.);
#7494=B_SPLINE_CURVE_WITH_KNOTS('',3,(#39122,#39123,#39124,#39125,#39126,
#39127),.UNSPECIFIED.,.F.,.F.,(4,1,1,4),(-4.08237667107798,-3.69276867472374,
-3.43303001048758,-3.17329134625142),.UNSPECIFIED.);
#7495=B_SPLINE_CURVE_WITH_KNOTS('',3,(#39129,#39130,#39131,#39132,#39133,
#39134),.UNSPECIFIED.,.F.,.F.,(4,1,1,4),(-3.17329134625142,-3.0004111005852,
-2.65465060925274,-1.96312962658784),.UNSPECIFIED.);
#7496=B_SPLINE_CURVE_WITH_KNOTS('',3,(#39136,#39137,#39138,#39139,#39140,
#39141),.UNSPECIFIED.,.F.,.F.,(4,1,1,4),(-1.96312962658784,-1.63061718285122,
-1.46436096098291,-0.799336073509661),.UNSPECIFIED.);
#7497=B_SPLINE_CURVE_WITH_KNOTS('',3,(#39143,#39144,#39145,#39146,#39147,
#39148,#39149,#39150,#39151,#39152,#39153,#39154,#39155,#39156,#39157,#39158),
 .UNSPECIFIED.,.F.,.F.,(4,2,2,2,2,2,2,4),(0.,0.0152664079390442,0.027653014192354,
0.0523618805947198,0.101540119432788,0.198808909364561,0.307282372348676,
0.415444261708341),.UNSPECIFIED.);
#7498=B_SPLINE_CURVE_WITH_KNOTS('',3,(#39160,#39161,#39162,#39163),
 .UNSPECIFIED.,.F.,.F.,(4,4),(-0.083360384276397,0.),.UNSPECIFIED.);
#7499=B_SPLINE_CURVE_WITH_KNOTS('',3,(#39165,#39166,#39167,#39168,#39169,
#39170,#39171,#39172,#39173,#39174,#39175,#39176,#39177,#39178,#39179,#39180,
#39181,#39182,#39183,#39184),.UNSPECIFIED.,.F.,.F.,(4,2,2,2,2,2,2,2,2,4),
(-0.858618632215441,-0.796721982029608,-0.711742820019591,-0.588477642133705,
-0.447897244908574,-0.350522204727673,-0.263299666311678,-0.166095103471627,
-0.0806423683440006,0.),.UNSPECIFIED.);
#7500=B_SPLINE_CURVE_WITH_KNOTS('',3,(#39186,#39187,#39188,#39189),
 .UNSPECIFIED.,.F.,.F.,(4,4),(0.,0.0412699530886637),.UNSPECIFIED.);
#7501=B_SPLINE_CURVE_WITH_KNOTS('',3,(#39191,#39192,#39193,#39194,#39195,
#39196,#39197,#39198,#39199,#39200,#39201,#39202,#39203,#39204,#39205,#39206,
#39207,#39208,#39209,#39210,#39211,#39212,#39213,#39214,#39215,#39216,#39217,
#39218,#39219,#39220,#39221,#39222,#39223,#39224,#39225,#39226,#39227,#39228,
#39229,#39230,#39231,#39232,#39233,#39234,#39235,#39236,#39237,#39238,#39239,
#39240,#39241,#39242,#39243,#39244,#39245,#39246,#39247,#39248,#39249,#39250,
#39251,#39252,#39253,#39254,#39255,#39256,#39257,#39258,#39259,#39260,#39261,
#39262,#39263),.UNSPECIFIED.,.F.,.F.,(4,3,3,3,3,3,3,3,3,3,3,3,3,3,3,3,3,
3,3,3,3,3,3,3,4),(0.0412699530886637,0.0818316212945925,0.127280583877176,
0.167222965675975,0.208677982151513,0.222888544302312,0.27017141431169,
0.306401513271525,0.345336818831997,0.360014116656582,0.363335263361059,
0.366168598848722,0.380743899105821,0.389827752889108,0.404046010130338,
0.437987441830756,0.459544829305343,0.475688276182035,0.525660573069947,
0.570392796077007,0.596688962991176,0.616464757561649,0.631242934104657,
0.642319205961073,0.675577463733683),.UNSPECIFIED.);
#7502=B_SPLINE_CURVE_WITH_KNOTS('',3,(#39265,#39266,#39267,#39268,#39269,
#39270,#39271),.UNSPECIFIED.,.F.,.F.,(4,1,1,1,4),(0.675577463735769,0.762573445120124,
0.936565407888833,1.11055737065754,1.28454933342625),.UNSPECIFIED.);
#7503=B_SPLINE_CURVE_WITH_KNOTS('',3,(#39273,#39274,#39275,#39276,#39277,
#39278,#39279,#39280,#39281,#39282),.UNSPECIFIED.,.F.,.F.,(4,1,1,1,1,1,
1,4),(1.28454933342625,1.68637707337851,1.88729094335464,1.93751941084867,
1.9877478783427,2.08820481333076,2.28911868330689,2.69094642325915),
 .UNSPECIFIED.);
#7504=B_SPLINE_CURVE_WITH_KNOTS('',3,(#39284,#39285,#39286,#39287,#39288,
#39289,#39290),.UNSPECIFIED.,.F.,.F.,(4,1,1,1,4),(2.69094642325915,3.62889794602885,
4.25419896120866,4.56684946879856,4.87949997638846),.UNSPECIFIED.);
#7505=B_SPLINE_CURVE_WITH_KNOTS('',3,(#39292,#39293,#39294,#39295,#39296,
#39297,#39298,#39299,#39300,#39301,#39302,#39303,#39304,#39305,#39306,#39307,
#39308,#39309,#39310,#39311,#39312,#39313,#39314,#39315,#39316,#39317,#39318,
#39319,#39320,#39321,#39322,#39323,#39324,#39325,#39326,#39327,#39328,#39329,
#39330,#39331,#39332,#39333,#39334,#39335,#39336,#39337,#39338,#39339,#39340,
#39341,#39342,#39343,#39344,#39345,#39346,#39347,#39348,#39349,#39350,#39351,
#39352,#39353,#39354,#39355,#39356,#39357,#39358,#39359,#39360,#39361,#39362,
#39363,#39364,#39365,#39366,#39367,#39368,#39369,#39370),.UNSPECIFIED.,
 .F.,.F.,(4,3,3,3,3,3,3,3,3,3,3,3,3,3,3,3,3,3,3,3,3,3,3,3,3,3,4),(4.87949998907266,
4.95846601833617,5.03754218990488,5.11201692992118,5.20633440915355,5.23893182822998,
5.33304562294149,5.42574668845617,5.51308570121414,5.56887242574961,5.57705083698662,
5.58713238475521,5.66474271049979,5.74432138797377,5.80956779051934,5.8835277857574,
5.96178045115228,5.96678376268769,6.04208474405206,6.13407813110945,6.21754073459664,
6.27460169758478,6.34310415203667,6.36106023233793,6.39702927495987,6.45672816597949,
6.5071186511175),.UNSPECIFIED.);
#7506=B_SPLINE_CURVE_WITH_KNOTS('',3,(#39372,#39373,#39374,#39375,#39376,
#39377,#39378,#39379,#39380,#39381,#39382,#39383,#39384,#39385,#39386,#39387,
#39388,#39389,#39390,#39391,#39392,#39393,#39394,#39395,#39396,#39397,#39398,
#39399,#39400,#39401,#39402,#39403,#39404,#39405,#39406,#39407,#39408,#39409,
#39410,#39411,#39412,#39413,#39414,#39415,#39416,#39417,#39418,#39419,#39420,
#39421,#39422,#39423,#39424,#39425,#39426,#39427,#39428,#39429,#39430,#39431,
#39432,#39433,#39434,#39435,#39436,#39437,#39438,#39439,#39440,#39441,#39442,
#39443,#39444,#39445,#39446,#39447,#39448,#39449,#39450,#39451,#39452,#39453,
#39454,#39455,#39456,#39457,#39458,#39459,#39460,#39461,#39462,#39463,#39464,
#39465,#39466,#39467,#39468,#39469,#39470,#39471,#39472,#39473,#39474),
 .UNSPECIFIED.,.F.,.F.,(4,3,3,3,3,3,3,3,3,3,3,3,3,3,3,3,3,3,3,3,3,3,3,3,
3,3,3,3,3,3,3,3,3,3,4),(6.50711865139611,6.50759747783067,6.55849518506602,
6.6055514827624,6.62030760880029,6.68061776690407,6.712779658626,6.76357285335593,
6.7827251429892,6.78667493342774,6.84072368001367,6.89838802619721,6.91844066613449,
6.9313826792552,6.93513738770287,6.96985591801162,7.02127116988874,7.08319431987471,
7.12333562472304,7.21448912595546,7.22693217739724,7.31027538715254,7.32976268115149,
7.39278093652575,7.48282966703091,7.48400843678286,7.53542368865998,7.54291222503036,
7.6182601558594,7.67703169440616,7.74108469616848,7.80585932729412,7.89114585771929,
7.94672668976107,7.94674570367697),.UNSPECIFIED.);
#7507=B_SPLINE_CURVE_WITH_KNOTS('',3,(#39476,#39477,#39478,#39479,#39480,
#39481,#39482,#39483,#39484,#39485,#39486),.UNSPECIFIED.,.F.,.F.,(4,1,1,
1,1,1,1,1,4),(0.,0.561198674779733,0.701498343474666,0.841798012169599,
0.982097680864532,1.12239734955947,1.40299668694933,1.6835960243392,1.96419536172906),
 .UNSPECIFIED.);
#7508=B_SPLINE_CURVE_WITH_KNOTS('',3,(#39488,#39489,#39490,#39491,#39492,
#39493,#39494,#39495,#39496,#39497,#39498,#39499,#39500,#39501,#39502,#39503,
#39504,#39505,#39506,#39507,#39508,#39509,#39510,#39511,#39512,#39513,#39514,
#39515,#39516,#39517,#39518,#39519,#39520,#39521,#39522,#39523,#39524,#39525,
#39526,#39527,#39528,#39529,#39530,#39531,#39532,#39533,#39534,#39535,#39536,
#39537,#39538,#39539,#39540,#39541,#39542,#39543,#39544,#39545,#39546,#39547,
#39548,#39549,#39550,#39551,#39552,#39553,#39554,#39555,#39556,#39557,#39558,
#39559,#39560,#39561,#39562,#39563,#39564,#39565,#39566,#39567,#39568,#39569,
#39570,#39571,#39572,#39573,#39574,#39575,#39576,#39577,#39578,#39579,#39580,
#39581),.UNSPECIFIED.,.F.,.F.,(4,3,3,3,3,3,3,3,3,3,3,3,3,3,3,3,3,3,3,3,
3,3,3,3,3,3,3,3,3,3,3,4),(1.96419536172906,2.02278079718735,2.08132684226757,
2.14059323164455,2.1643872272574,2.1995405412518,2.29893902795959,2.31381748093507,
2.34843033506652,2.43488572077454,2.55267608477937,2.66314540186569,2.67023090029728,
2.67711184811797,2.7608378847451,2.83320698228256,2.89993723462245,2.90557607982002,
2.97452259973018,3.04107121308078,3.10415755340534,3.12000863076421,3.14092125934276,
3.20590661407528,3.26963227096302,3.33186628772024,3.3762664388655,3.37817772008658,
3.45298028284022,3.52444999935711,3.59189483482569,3.61161161838824),
 .UNSPECIFIED.);
#7509=B_SPLINE_CURVE_WITH_KNOTS('',3,(#39583,#39584,#39585,#39586,#39587,
#39588,#39589),.UNSPECIFIED.,.F.,.F.,(4,1,1,1,4),(3.61161161838824,4.07783568596737,
4.23324370849375,4.54405975354651,4.69946777607289),.UNSPECIFIED.);
#7510=B_SPLINE_CURVE_WITH_KNOTS('',3,(#39591,#39592,#39593,#39594,#39595,
#39596,#39597,#39598,#39599,#39600,#39601,#39602,#39603,#39604,#39605,#39606,
#39607,#39608,#39609,#39610,#39611,#39612,#39613,#39614,#39615,#39616,#39617,
#39618,#39619,#39620,#39621,#39622,#39623,#39624,#39625,#39626,#39627,#39628,
#39629,#39630,#39631,#39632,#39633,#39634,#39635,#39636,#39637,#39638,#39639,
#39640,#39641,#39642,#39643,#39644,#39645,#39646,#39647,#39648,#39649,#39650,
#39651,#39652,#39653,#39654,#39655,#39656,#39657,#39658,#39659,#39660,#39661,
#39662,#39663,#39664,#39665,#39666,#39667,#39668,#39669),.UNSPECIFIED.,
 .F.,.F.,(4,3,3,3,3,3,3,3,3,3,3,3,3,3,3,3,3,3,3,3,3,3,3,3,3,3,4),(4.69946777607289,
4.70008212677047,4.72337034362506,4.74665856047964,4.78464222436074,4.79437105296614,
4.86335173767338,4.89331619143087,4.99100694367976,5.09449896259877,5.10579756798661,
5.21863815454279,5.34210882161955,5.47819569571612,5.58490842306537,5.73454801258545,
5.80455488046634,5.84054271537192,6.04704511696064,6.10124092996291,6.16726926099793,
6.23355124993576,6.36668501266555,6.43343772256572,6.46683837248413,6.50024667222643,
6.63337020876143),.UNSPECIFIED.);
#7511=B_SPLINE_CURVE_WITH_KNOTS('',3,(#39671,#39672,#39673,#39674,#39675,
#39676,#39677,#39678,#39679,#39680,#39681,#39682,#39683,#39684,#39685,#39686,
#39687,#39688,#39689,#39690,#39691,#39692,#39693,#39694,#39695,#39696,#39697,
#39698,#39699,#39700,#39701,#39702,#39703,#39704,#39705,#39706,#39707,#39708,
#39709,#39710,#39711,#39712,#39713,#39714,#39715,#39716,#39717,#39718,#39719,
#39720,#39721,#39722),.UNSPECIFIED.,.F.,.F.,(4,3,3,3,3,3,3,3,3,3,3,3,3,
3,3,3,3,4),(6.63337020876143,6.71835164595222,6.76468949711311,6.7848176488122,
6.86918510077649,6.91824398486027,7.12465942928312,7.21977330459364,7.45975726452654,
7.55231050612421,7.69215232698206,7.72134807390837,7.73908189390303,7.95493068281924,
8.18846010117661,8.41215537152321,8.61841637768341,8.77692550510397),
 .UNSPECIFIED.);
#7512=B_SPLINE_CURVE_WITH_KNOTS('',3,(#39724,#39725,#39726,#39727,#39728,
#39729),.UNSPECIFIED.,.F.,.F.,(4,1,1,4),(8.77692550510397,9.17723620667681,
9.97785760982251,11.5791004161139),.UNSPECIFIED.);
#7513=B_SPLINE_CURVE_WITH_KNOTS('',3,(#39731,#39732,#39733,#39734),
 .UNSPECIFIED.,.F.,.F.,(4,4),(11.5791004161139,11.7855397152994),
 .UNSPECIFIED.);
#7514=B_SPLINE_CURVE_WITH_KNOTS('',3,(#39736,#39737,#39738,#39739,#39740,
#39741,#39742,#39743,#39744,#39745,#39746,#39747,#39748,#39749,#39750,#39751,
#39752,#39753,#39754,#39755,#39756,#39757,#39758,#39759,#39760,#39761,#39762,
#39763,#39764,#39765,#39766,#39767,#39768,#39769,#39770,#39771,#39772,#39773,
#39774,#39775,#39776,#39777,#39778,#39779,#39780,#39781,#39782,#39783,#39784,
#39785,#39786,#39787),.UNSPECIFIED.,.F.,.F.,(4,3,3,3,3,3,3,3,3,3,3,3,3,
3,3,3,3,4),(0.,0.0536833715747986,0.107366743149597,0.161050114724396,0.214733486299194,
0.228154329192894,0.241575172086594,0.268416857873993,0.322100229448792,
0.34058124806175,0.37578360102359,0.429466972598389,0.509992029960587,0.590517087322785,
0.644200458897583,0.648567865518541,0.697883830472382,0.75156720204718),
 .UNSPECIFIED.);
#7515=B_SPLINE_CURVE_WITH_KNOTS('',3,(#39789,#39790,#39791,#39792),
 .UNSPECIFIED.,.F.,.F.,(4,4),(-76.3862538744791,-75.2949305236969),
 .UNSPECIFIED.);
#7516=B_SPLINE_CURVE_WITH_KNOTS('',3,(#39794,#39795,#39796,#39797,#39798,
#39799,#39800,#39801,#39802,#39803,#39804,#39805,#39806,#39807,#39808,#39809),
 .UNSPECIFIED.,.F.,.F.,(4,2,2,2,2,2,2,4),(0.,0.183117048783268,0.366537301552345,
0.538130301316899,0.626221380614023,0.670497094381026,0.692705457368327,
0.719797781043186),.UNSPECIFIED.);
#7517=B_SPLINE_CURVE_WITH_KNOTS('',3,(#39811,#39812,#39813,#39814,#39815),
 .UNSPECIFIED.,.F.,.F.,(4,1,4),(-66.1031756239825,-60.0916422517874,-52.076264422194),
 .UNSPECIFIED.);
#7518=B_SPLINE_CURVE_WITH_KNOTS('',3,(#39817,#39818,#39819,#39820,#39821,
#39822,#39823,#39824),.UNSPECIFIED.,.F.,.F.,(4,1,1,1,1,4),(-52.076264422194,
-47.0953817384218,-43.7747932825737,-42.1144990546496,-41.2843519406876,
-40.4542048267256),.UNSPECIFIED.);
#7519=B_SPLINE_CURVE_WITH_KNOTS('',3,(#39826,#39827,#39828,#39829,#39830,
#39831,#39832,#39833,#39834,#39835,#39836,#39837,#39838,#39839,#39840,#39841,
#39842,#39843,#39844,#39845,#39846,#39847,#39848,#39849,#39850,#39851,#39852,
#39853,#39854,#39855,#39856,#39857,#39858,#39859,#39860,#39861,#39862,#39863,
#39864,#39865,#39866,#39867,#39868,#39869,#39870,#39871,#39872,#39873,#39874,
#39875,#39876,#39877,#39878,#39879,#39880,#39881,#39882,#39883,#39884,#39885,
#39886,#39887,#39888,#39889,#39890,#39891,#39892,#39893,#39894,#39895,#39896,
#39897,#39898,#39899,#39900,#39901,#39902,#39903,#39904,#39905,#39906,#39907,
#39908,#39909,#39910,#39911,#39912,#39913,#39914,#39915,#39916,#39917,#39918,
#39919,#39920,#39921,#39922,#39923,#39924,#39925,#39926,#39927,#39928,#39929,
#39930,#39931,#39932,#39933,#39934,#39935,#39936,#39937,#39938,#39939,#39940,
#39941,#39942,#39943,#39944,#39945,#39946,#39947,#39948,#39949,#39950,#39951,
#39952,#39953,#39954,#39955,#39956,#39957,#39958,#39959,#39960,#39961),
 .UNSPECIFIED.,.F.,.F.,(4,3,3,3,3,3,3,3,3,3,3,3,3,3,3,3,3,3,3,3,3,3,3,3,
3,3,3,3,3,3,3,3,3,3,3,3,3,3,3,3,3,3,3,3,3,4),(-40.4542048267256,-40.1022888941731,
-39.7562065398827,-39.4194632193958,-39.1058191008429,-38.933143939164,
-38.6244983462993,-38.3981006364017,-38.3280947633795,-38.2582169507945,
-38.1717029265041,-38.1044071679005,-38.0424313761866,-37.8847341943161,
-37.8522360082441,-37.8370823843021,-37.6848449686041,-37.5482438086545,
-37.5103390037277,-37.4116426487049,-37.3168209132788,-37.26909277659,-37.2226826845227,
-37.0094865067236,-36.83127763601,-36.7421017606314,-36.702172602122,-36.6530687652964,
-36.5482684339635,-36.4793361229095,-36.3083732393702,-36.2040398925353,
-36.1567733945135,-36.1373900755466,-36.119432910608,-35.9439828384436,
-35.8910398520304,-35.7861271288821,-35.6763044151121,-35.5398153198633,
-35.475355900409,-35.431857525938,-35.3193842642253,-35.2761527725057,-35.1765274058965,
-35.1303480341168),.UNSPECIFIED.);
#7520=B_SPLINE_CURVE_WITH_KNOTS('',3,(#39963,#39964,#39965,#39966,#39967,
#39968,#39969,#39970,#39971,#39972,#39973,#39974,#39975,#39976,#39977,#39978,
#39979,#39980,#39981,#39982,#39983,#39984,#39985,#39986,#39987,#39988,#39989,
#39990,#39991,#39992,#39993,#39994,#39995,#39996,#39997,#39998,#39999,#40000,
#40001,#40002,#40003,#40004,#40005,#40006,#40007,#40008,#40009,#40010,#40011,
#40012,#40013,#40014,#40015,#40016,#40017,#40018,#40019,#40020,#40021,#40022,
#40023,#40024,#40025,#40026,#40027,#40028,#40029,#40030,#40031,#40032,#40033,
#40034,#40035),.UNSPECIFIED.,.F.,.F.,(4,3,3,3,3,3,3,3,3,3,3,3,3,3,3,3,3,
3,3,3,3,3,3,3,4),(-35.1303480022468,-35.1258447959463,-34.8587472887927,
-34.5695675087557,-34.2705671521664,-33.9510365315198,-33.7020281686448,
-33.4584584867811,-33.1570167675092,-32.7424918126182,-32.3093224434396,
-32.2207562081337,-31.7865689394453,-31.4628125680942,-31.1408963345733,
-30.9506241657775,-30.8303818716246,-30.4481649386763,-30.0912580436924,
-29.8395659206186,-29.6953645849095,-29.5361530629831,-29.3729500851293,
-29.2794465468541,-29.2787346184417),.UNSPECIFIED.);
#7521=B_SPLINE_CURVE_WITH_KNOTS('',3,(#40037,#40038,#40039,#40040,#40041,
#40042,#40043,#40044,#40045,#40046),.UNSPECIFIED.,.F.,.F.,(4,2,2,2,4),(0.,
0.081213735526853,0.152682973202012,0.298883812384628,0.584812965668925),
 .UNSPECIFIED.);
#7522=B_SPLINE_CURVE_WITH_KNOTS('',3,(#40048,#40049,#40050,#40051,#40052,
#40053,#40054,#40055),.UNSPECIFIED.,.F.,.F.,(4,1,1,1,1,4),(-20.9230961620266,
-17.7936201740765,-15.7073028487765,-14.6641441861265,-14.1425648548015,
-13.6209855234765),.UNSPECIFIED.);
#7523=B_SPLINE_CURVE_WITH_KNOTS('',3,(#40057,#40058,#40059,#40060,#40061,
#40062,#40063,#40064),.UNSPECIFIED.,.F.,.F.,(4,1,1,1,1,4),(-13.6209855234765,
-10.9458199140635,-10.0540980442592,-9.16237617445491,-8.2706543046506,
-7.37893243484629),.UNSPECIFIED.);
#7524=B_SPLINE_CURVE_WITH_KNOTS('',3,(#40066,#40067,#40068,#40069,#40070,
#40071,#40072,#40073,#40074,#40075,#40076),.UNSPECIFIED.,.F.,.F.,(4,1,1,
1,1,1,1,1,4),(-7.37893243484629,-6.86694230253758,-5.84296203792017,-4.81898177330275,
-4.56298670714839,-4.46698855734051,-4.30699164099404,-4.05099657483969,
-3.79500150868533),.UNSPECIFIED.);
#7525=B_SPLINE_CURVE_WITH_KNOTS('',3,(#40078,#40079,#40080,#40081,#40082,
#40083,#40084,#40085,#40086,#40087,#40088),.UNSPECIFIED.,.F.,.F.,(4,1,1,
1,1,1,1,1,4),(-3.79500150868533,-3.54558322444133,-3.04674665595333,-2.92203751383133,
-2.79732837170933,-2.67261922958733,-2.54791008746534,-2.29849180322134,
-2.04907351897734),.UNSPECIFIED.);
#7526=B_SPLINE_CURVE_WITH_KNOTS('',3,(#40090,#40091,#40092,#40093,#40094,
#40095,#40096,#40097,#40098,#40099),.UNSPECIFIED.,.F.,.F.,(4,1,1,1,1,1,
1,4),(-2.04907351897734,-1.91473526774895,-1.64605876529219,-1.5117205140638,
-1.37738226283542,-1.24304401160704,-1.17587488599285,-1.10870576037865),
 .UNSPECIFIED.);
#7527=B_SPLINE_CURVE_WITH_KNOTS('',3,(#40101,#40102,#40103,#40104,#40105,
#40106,#40107,#40108,#40109),.UNSPECIFIED.,.F.,.F.,(4,1,1,1,1,1,4),(-1.10870576037865,
-1.01091721837057,-0.913128676362484,-0.815340134354398,-0.766445863350356,
-0.619763050338228,-0.424185966322057),.UNSPECIFIED.);
#7528=B_SPLINE_CURVE_WITH_KNOTS('',3,(#40111,#40112,#40113,#40114),
 .UNSPECIFIED.,.F.,.F.,(4,4),(-0.424185966322057,0.),.UNSPECIFIED.);
#7529=B_SPLINE_CURVE_WITH_KNOTS('',3,(#40116,#40117,#40118,#40119,#40120,
#40121,#40122,#40123,#40124,#40125),.UNSPECIFIED.,.F.,.F.,(4,1,1,1,1,1,
1,4),(0.,0.21623669638068,0.324355044571019,0.432473392761359,0.540591740951699,
0.648710089142039,0.702769263237209,0.756828282974645),.UNSPECIFIED.);
#7530=B_SPLINE_CURVE_WITH_KNOTS('',3,(#40127,#40128,#40129,#40130,#40131,
#40132,#40133,#40134,#40135,#40136,#40137,#40138,#40139,#40140,#40141,#40142,
#40143,#40144,#40145,#40146,#40147,#40148,#40149,#40150,#40151,#40152,#40153,
#40154,#40155,#40156,#40157,#40158,#40159,#40160,#40161,#40162,#40163,#40164,
#40165,#40166,#40167,#40168,#40169,#40170,#40171,#40172,#40173,#40174,#40175,
#40176,#40177,#40178,#40179,#40180,#40181,#40182,#40183,#40184,#40185,#40186,
#40187,#40188,#40189,#40190,#40191,#40192,#40193,#40194,#40195,#40196,#40197,
#40198,#40199,#40200,#40201,#40202,#40203,#40204,#40205,#40206,#40207,#40208,
#40209,#40210,#40211,#40212,#40213,#40214,#40215,#40216,#40217,#40218,#40219,
#40220,#40221,#40222,#40223,#40224,#40225,#40226,#40227,#40228,#40229,#40230,
#40231,#40232,#40233,#40234,#40235,#40236,#40237,#40238,#40239,#40240,#40241,
#40242,#40243,#40244,#40245,#40246,#40247,#40248,#40249,#40250),
 .UNSPECIFIED.,.F.,.F.,(4,3,3,3,3,3,3,3,3,3,3,3,3,3,3,3,3,3,3,3,3,3,3,3,
3,3,3,3,3,3,3,3,3,3,3,3,3,3,3,3,3,4),(0.75682843983895,0.777855768006281,
0.798415570084359,0.818399869123068,0.828970599685942,0.84657569246793,
0.863552669234487,0.879734247088197,0.887389032088879,0.901112762039505,
0.912418616344217,0.919148302627896,0.933698235587157,0.937183843216286,
0.958433684197906,0.973254924393068,0.994408075484192,1.00932600556985,
1.02736154615824,1.03637931645244,1.04539708674663,1.06102318516838,1.07723388409314,
1.09375127908744,1.11068703369019,1.11753924910019,1.12521404406605,1.13678529162007,
1.15070887827124,1.16479420266661,1.17931025663697,1.18968141145376,1.20343576632493,
1.20608689093743,1.22052173269292,1.22575249263054,1.23445659171005,1.24399746592949,
1.2482472022461,1.254096563094,1.25979095927171,1.26182357380732),
 .UNSPECIFIED.);
#7531=B_SPLINE_CURVE_WITH_KNOTS('',3,(#40252,#40253,#40254,#40255,#40256,
#40257,#40258,#40259,#40260,#40261,#40262,#40263,#40264,#40265,#40266,#40267,
#40268,#40269,#40270,#40271,#40272,#40273,#40274,#40275,#40276,#40277,#40278,
#40279,#40280,#40281,#40282,#40283,#40284,#40285,#40286,#40287,#40288,#40289,
#40290,#40291,#40292,#40293,#40294,#40295,#40296,#40297,#40298,#40299,#40300,
#40301,#40302,#40303,#40304,#40305,#40306,#40307,#40308,#40309,#40310,#40311,
#40312,#40313,#40314,#40315,#40316,#40317,#40318),.UNSPECIFIED.,.F.,.F.,
(4,3,3,3,3,3,3,3,3,3,3,3,3,3,3,3,3,3,3,3,3,3,4),(1.26182357380732,1.26310836126709,
1.26448943174598,1.28057362669222,1.28823756969933,1.30269384661357,1.30996639391098,
1.32430281701794,1.32960413527727,1.33493261849779,1.34310096601661,1.3469432325596,
1.34924187664357,1.35187874054377,1.3592939367365,1.36865825613663,1.38371245588514,
1.38814353058811,1.39144562654905,1.39590278038911,1.4118599289142,1.42978166972109,
1.43249195629979),.UNSPECIFIED.);
#7532=B_SPLINE_CURVE_WITH_KNOTS('',3,(#40320,#40321,#40322,#40323,#40324,
#40325,#40326,#40327,#40328,#40329,#40330,#40331,#40332,#40333),
 .UNSPECIFIED.,.F.,.F.,(4,2,2,2,2,2,4),(0.,0.0578367417336795,0.106933208379369,
0.202213644056447,0.263225317305196,0.417445308347203,0.566894598811129),
 .UNSPECIFIED.);
#7533=B_SPLINE_CURVE_WITH_KNOTS('',3,(#40335,#40336,#40337,#40338,#40339,
#40340,#40341,#40342,#40343,#40344,#40345,#40346,#40347,#40348,#40349,#40350,
#40351,#40352,#40353,#40354,#40355,#40356,#40357,#40358,#40359,#40360,#40361,
#40362,#40363,#40364,#40365,#40366,#40367,#40368,#40369,#40370,#40371,#40372,
#40373,#40374,#40375,#40376,#40377,#40378,#40379,#40380,#40381,#40382,#40383,
#40384,#40385,#40386,#40387,#40388,#40389,#40390,#40391,#40392,#40393,#40394,
#40395,#40396,#40397,#40398,#40399,#40400,#40401,#40402,#40403,#40404,#40405,
#40406,#40407,#40408,#40409,#40410,#40411,#40412,#40413,#40414,#40415,#40416,
#40417,#40418,#40419,#40420,#40421,#40422,#40423,#40424,#40425),
 .UNSPECIFIED.,.F.,.F.,(4,3,3,3,3,3,3,3,3,3,3,3,3,3,3,3,3,3,3,3,3,3,3,3,
3,3,3,3,3,3,4),(1.56845677767309,1.56846172637483,1.57845303864828,1.58918112661639,
1.60105011224252,1.60181606521468,1.62530741495631,1.65075769300814,1.65649085724454,
1.66853464029784,1.67051106563605,1.69204727198684,1.70189392783942,1.71900500530774,
1.735253215381,1.73723529695383,1.7435930372664,1.74892582684199,1.75193285915179,
1.75254514822567,1.75874043000982,1.76460430548112,1.76861250292259,1.77474630213318,
1.78135331945415,1.78529214669338,1.79226862981698,1.79301029063736,1.79918428811343,
1.80197176948314,1.80197179046417),.UNSPECIFIED.);
#7534=B_SPLINE_CURVE_WITH_KNOTS('',3,(#40427,#40428,#40429,#40430,#40431,
#40432),.UNSPECIFIED.,.F.,.F.,(4,1,1,4),(1.80197179046417,1.80928949299685,
1.8129483442632,1.82758374932857),.UNSPECIFIED.);
#7535=B_SPLINE_CURVE_WITH_KNOTS('',3,(#40434,#40435,#40436,#40437,#40438,
#40439,#40440,#40441,#40442),.UNSPECIFIED.,.F.,.F.,(4,1,1,1,1,1,4),(1.82758374932857,
1.83805116497033,1.84328487279121,1.85898599625385,1.87992082753738,1.89038824317914,
1.9008556588209),.UNSPECIFIED.);
#7536=B_SPLINE_CURVE_WITH_KNOTS('',3,(#40444,#40445,#40446,#40447,#40448,
#40449,#40450,#40451,#40452,#40453,#40454,#40455),.UNSPECIFIED.,.F.,.F.,
(4,2,2,2,2,4),(0.,0.399925490199206,0.590873146475409,0.6853407600757,0.732736191576422,
0.780059088229237),.UNSPECIFIED.);
#7537=B_SPLINE_CURVE_WITH_KNOTS('',3,(#40457,#40458,#40459,#40460,#40461,
#40462,#40463,#40464),.UNSPECIFIED.,.F.,.F.,(4,1,1,1,1,4),(1.96650114296421,
1.97401285460172,1.97651675848088,1.98653237399755,2.00656360503089,2.03661045158091),
 .UNSPECIFIED.);
#7538=B_SPLINE_CURVE_WITH_KNOTS('',3,(#40466,#40467,#40468,#40469,#40470,
#40471,#40472,#40473,#40474,#40475,#40476,#40477,#40478,#40479,#40480,#40481,
#40482,#40483,#40484,#40485,#40486,#40487,#40488,#40489,#40490,#40491,#40492,
#40493,#40494,#40495,#40496,#40497,#40498,#40499,#40500,#40501,#40502,#40503,
#40504,#40505,#40506,#40507,#40508,#40509,#40510,#40511,#40512,#40513,#40514,
#40515,#40516,#40517,#40518,#40519,#40520,#40521,#40522,#40523,#40524,#40525,
#40526,#40527,#40528,#40529,#40530,#40531,#40532,#40533,#40534,#40535,#40536,
#40537,#40538,#40539,#40540,#40541),.UNSPECIFIED.,.F.,.F.,(4,3,3,3,3,3,
3,3,3,3,3,3,3,3,3,3,3,3,3,3,3,3,3,3,3,4),(2.03661045158091,2.04094396755524,
2.04146916453237,2.04613737339918,2.05247626445997,2.05498033734634,2.05614902505797,
2.05989481366869,2.06138177904424,2.06402869927639,2.06416861681123,2.06575962872735,
2.06835564146826,2.06972997740258,2.07334626528165,2.07526740689269,2.07848486059925,
2.08105152526794,2.08251647649159,2.0869107221265,2.09126152036397,2.09170330290054,
2.09261961436811,2.09495872614039,2.09994461036642,2.10087562037983),
 .UNSPECIFIED.);
#7539=B_SPLINE_CURVE_WITH_KNOTS('',3,(#40543,#40544,#40545,#40546,#40547,
#40548,#40549,#40550),.UNSPECIFIED.,.F.,.F.,(4,1,1,1,1,4),(2.10087562037983,
2.11383027239681,2.12678492441379,2.13973957643076,2.15269422844774,2.19155818449868),
 .UNSPECIFIED.);
#7540=B_SPLINE_CURVE_WITH_KNOTS('',3,(#40551,#40552,#40553,#40554,#40555,
#40556,#40557,#40558,#40559,#40560,#40561),.UNSPECIFIED.,.F.,.F.,(4,1,1,
1,1,1,1,1,4),(2.19155818449868,2.25090656855756,2.280580760587,2.31025495261644,
2.32509204863116,2.33992914464588,2.36960333667532,2.48830010479308,2.60699687291084),
 .UNSPECIFIED.);
#7541=B_SPLINE_CURVE_WITH_KNOTS('',3,(#40564,#40565,#40566,#40567),
 .UNSPECIFIED.,.F.,.F.,(4,4),(8.92039936009897,9.19419977830157),
 .UNSPECIFIED.);
#7542=B_SPLINE_CURVE_WITH_KNOTS('',3,(#40569,#40570,#40571,#40572,#40573),
 .UNSPECIFIED.,.F.,.F.,(4,1,4),(8.15775006426363,8.53897544224619,8.92020082022876),
 .UNSPECIFIED.);
#7543=B_SPLINE_CURVE_WITH_KNOTS('',3,(#40575,#40576,#40577,#40578,#40579,
#40580,#40581,#40582,#40583,#40584),.UNSPECIFIED.,.F.,.F.,(4,1,1,1,1,1,
1,4),(6.48647098475663,6.695380869695,6.79983581216419,7.11320063957175,
7.32211052451013,7.73993029438688,7.94884017932526,8.15741223597716),
 .UNSPECIFIED.);
#7544=B_SPLINE_CURVE_WITH_KNOTS('',3,(#40586,#40587,#40588,#40589,#40590,
#40591,#40592,#40593),.UNSPECIFIED.,.F.,.F.,(4,1,1,1,1,4),(5.69008244730366,
5.73985673089448,6.08827671603015,6.28737385039339,6.38692241757501,6.48619760405534),
 .UNSPECIFIED.);
#7545=B_SPLINE_CURVE_WITH_KNOTS('',3,(#40595,#40596,#40597,#40598,#40599,
#40600),.UNSPECIFIED.,.F.,.F.,(4,1,1,4),(5.0872072523488,5.23775148821748,
5.46391696776057,5.68999089118309),.UNSPECIFIED.);
#7546=B_SPLINE_CURVE_WITH_KNOTS('',3,(#40602,#40603,#40604,#40605,#40606,
#40607,#40608,#40609,#40610,#40611,#40612,#40613,#40614,#40615,#40616,#40617,
#40618,#40619,#40620,#40621,#40622,#40623,#40624,#40625,#40626,#40627,#40628,
#40629,#40630,#40631,#40632,#40633,#40634,#40635,#40636,#40637,#40638,#40639,
#40640,#40641,#40642,#40643,#40644,#40645,#40646,#40647,#40648,#40649,#40650,
#40651,#40652,#40653,#40654,#40655,#40656,#40657,#40658,#40659,#40660,#40661,
#40662,#40663,#40664,#40665,#40666,#40667,#40668,#40669,#40670,#40671,#40672,
#40673,#40674,#40675,#40676,#40677,#40678,#40679,#40680,#40681,#40682,#40683,
#40684,#40685,#40686,#40687,#40688,#40689),.UNSPECIFIED.,.F.,.F.,(4,3,3,
3,3,3,3,3,3,3,3,3,3,3,3,3,3,3,3,3,3,3,3,3,3,3,3,3,3,4),(4.51907254078117,
4.53712760209195,4.55524502799627,4.58345241158194,4.59126693036747,4.63722241805352,
4.67952721516863,4.7331373450095,4.76807910083128,4.77947322679447,4.78810538931333,
4.79482326640033,4.80302085665306,4.85270069873456,4.89887935926951,4.92360162081649,
4.94505801980446,4.95913352209898,4.9876580014522,4.99800173990669,5.00635849847016,
5.01618248080543,5.0429821330202,5.04445279252107,5.04585552133343,5.06059676426369,
5.06978178523498,5.07641636177966,5.08212660863856,5.08697450185542),
 .UNSPECIFIED.);
#7547=B_SPLINE_CURVE_WITH_KNOTS('',3,(#40691,#40692,#40693,#40694,#40695,
#40696,#40697,#40698,#40699,#40700,#40701,#40702,#40703,#40704,#40705,#40706,
#40707,#40708,#40709,#40710,#40711,#40712,#40713,#40714,#40715,#40716,#40717,
#40718,#40719,#40720,#40721,#40722,#40723,#40724,#40725,#40726,#40727),
 .UNSPECIFIED.,.F.,.F.,(4,3,3,3,3,3,3,3,3,3,3,3,4),(3.85684119100481,3.91047824257307,
3.95181977233274,4.01079062239622,4.04211759527654,4.1085062410119,4.17423090387904,
4.21136616955803,4.27069680674408,4.33497634591462,4.3997079256963,4.46637693241926,
4.51901017618764),.UNSPECIFIED.);
#7548=B_SPLINE_CURVE_WITH_KNOTS('',3,(#40729,#40730,#40731,#40732,#40733,
#40734,#40735,#40736,#40737,#40738,#40739,#40740,#40741,#40742,#40743,#40744,
#40745,#40746,#40747,#40748,#40749,#40750,#40751,#40752,#40753,#40754,#40755,
#40756,#40757,#40758,#40759,#40760,#40761,#40762,#40763,#40764,#40765,#40766,
#40767,#40768,#40769,#40770,#40771,#40772,#40773,#40774,#40775,#40776,#40777,
#40778,#40779,#40780,#40781,#40782,#40783,#40784,#40785,#40786,#40787,#40788,
#40789,#40790,#40791,#40792,#40793,#40794,#40795,#40796,#40797,#40798,#40799,
#40800,#40801,#40802,#40803,#40804,#40805,#40806,#40807,#40808,#40809,#40810,
#40811,#40812,#40813,#40814,#40815,#40816,#40817,#40818,#40819,#40820,#40821,
#40822,#40823,#40824,#40825,#40826,#40827,#40828),.UNSPECIFIED.,.F.,.F.,
(4,3,3,3,3,3,3,3,3,3,3,3,3,3,3,3,3,3,3,3,3,3,3,3,3,3,3,3,3,3,3,3,3,4),(1.53737298748225,
1.537475501564,1.62471277683277,1.68224296751281,1.77970297709453,1.78982695102308,
1.89509654051106,1.94309417534619,2.01390543033174,2.13717094946317,2.22810612528141,
2.34701828393927,2.47132786358456,2.4844090542388,2.49779593851528,2.611265334802,
2.69705547180907,2.7627193750795,2.88707829944944,2.90505995762026,3.03180902855002,
3.05948850905774,3.17551646821549,3.28049105931471,3.31567602520587,3.3763625860723,
3.46415464024906,3.54686387816802,3.61857318381905,3.62957311608698,3.69899296203923,
3.76450131194205,3.82520333218962,3.8565699837029),.UNSPECIFIED.);
#7549=B_SPLINE_CURVE_WITH_KNOTS('',3,(#40830,#40831,#40832,#40833,#40834),
 .UNSPECIFIED.,.F.,.F.,(4,1,4),(0.876829184656479,1.28960453962952,1.53726975261334),
 .UNSPECIFIED.);
#7550=B_SPLINE_CURVE_WITH_KNOTS('',3,(#40836,#40837,#40838,#40839),
 .UNSPECIFIED.,.F.,.F.,(4,4),(0.308773622131097,0.87661110736348),
 .UNSPECIFIED.);
#7551=B_SPLINE_CURVE_WITH_KNOTS('',3,(#40843,#40844,#40845,#40846,#40847,
#40848,#40849,#40850),.UNSPECIFIED.,.F.,.F.,(4,1,1,1,1,4),(0.775828301632668,
0.878761919402114,0.982054302260506,1.0853466851189,1.18863906797729,1.29193144447076),
 .UNSPECIFIED.);
#7552=B_SPLINE_CURVE_WITH_KNOTS('',3,(#40852,#40853,#40854,#40855,#40856,
#40857,#40858,#40859,#40860,#40861,#40862,#40863,#40864,#40865,#40866,#40867,
#40868,#40869,#40870,#40871,#40872,#40873,#40874,#40875,#40876,#40877,#40878,
#40879,#40880,#40881,#40882,#40883,#40884,#40885,#40886,#40887,#40888,#40889,
#40890,#40891,#40892,#40893,#40894,#40895,#40896,#40897,#40898,#40899,#40900,
#40901,#40902,#40903,#40904,#40905,#40906,#40907,#40908,#40909,#40910,#40911,
#40912,#40913,#40914,#40915,#40916,#40917,#40918,#40919,#40920,#40921),
 .UNSPECIFIED.,.F.,.F.,(4,3,3,3,3,3,3,3,3,3,3,3,3,3,3,3,3,3,3,3,3,3,3,4),
(0.226711159264386,0.240430118696369,0.254149078128352,0.281586996992319,
0.309024915856286,0.336462834720253,0.345475183164287,0.367386959070664,
0.395956346646867,0.424538765869713,0.44621451017612,0.473767544818013,
0.501191131249028,0.528641986740118,0.555966185631988,0.582919689839201,
0.609300375584998,0.634902866651908,0.6564639477599,0.665717861087855,0.694693069811103,
0.720593698815789,0.751264274684911,0.775469536543723),.UNSPECIFIED.);
#7553=B_SPLINE_CURVE_WITH_KNOTS('',3,(#40922,#40923,#40924,#40925,#40926,
#40927,#40928,#40929,#40930,#40931,#40932,#40933,#40934,#40935,#40936,#40937,
#40938,#40939,#40940,#40941,#40942,#40943,#40944,#40945,#40946,#40947,#40948,
#40949,#40950,#40951,#40952,#40953,#40954,#40955,#40956,#40957,#40958,#40959,
#40960,#40961,#40962,#40963,#40964,#40965,#40966,#40967,#40968,#40969,#40970,
#40971,#40972,#40973,#40974,#40975,#40976),.UNSPECIFIED.,.F.,.F.,(4,3,3,
3,3,3,3,3,3,3,3,3,3,3,3,3,3,3,4),(0.,0.00642281904770877,0.0274552042125774,
0.0483280032850625,0.0693493298709818,0.0906129623706381,0.112532404043595,
0.127771446025698,0.136026695558631,0.157567456770955,0.177849900137661,
0.181368927411508,0.193072040312714,0.201907114453229,0.209483636975919,
0.213952085004803,0.218360348732736,0.222453779943677,0.226477259692083),
 .UNSPECIFIED.);
#7554=B_SPLINE_CURVE_WITH_KNOTS('',3,(#40979,#40980,#40981,#40982),
 .UNSPECIFIED.,.F.,.F.,(4,4),(-0.314285883924713,-0.267175740076542),
 .UNSPECIFIED.);
#7555=B_SPLINE_CURVE_WITH_KNOTS('',3,(#40984,#40985,#40986,#40987,#40988,
#40989,#40990,#40991,#40992,#40993,#40994,#40995,#40996,#40997,#40998,#40999,
#41000,#41001,#41002,#41003,#41004,#41005,#41006,#41007,#41008,#41009,#41010,
#41011,#41012,#41013,#41014),.UNSPECIFIED.,.F.,.F.,(4,3,3,3,3,3,3,3,3,3,
4),(-0.267175770913084,-0.202641536318522,-0.184830688168289,-0.122723770586227,
-0.0570251245949306,7.73147172802893E-5,0.0628601143819659,0.123897646499237,
0.184935178616508,0.242766080933253,0.26717572254583),.UNSPECIFIED.);
#7556=B_SPLINE_CURVE_WITH_KNOTS('',3,(#41016,#41017,#41018,#41019),
 .UNSPECIFIED.,.F.,.F.,(4,4),(0.267175770913084,0.314279348079497),
 .UNSPECIFIED.);
#7557=B_SPLINE_CURVE_WITH_KNOTS('',3,(#41021,#41022,#41023,#41024),
 .UNSPECIFIED.,.F.,.F.,(4,4),(0.314279364233837,0.330164730316111),
 .UNSPECIFIED.);
#7558=B_SPLINE_CURVE_WITH_KNOTS('',3,(#41026,#41027,#41028,#41029,#41030,
#41031,#41032,#41033,#41034,#41035,#41036,#41037,#41038,#41039,#41040),
 .UNSPECIFIED.,.F.,.F.,(4,1,1,1,1,1,1,1,1,1,2,4),(-0.292787369885449,-0.24676514268468,
-0.186369611422536,-0.125974080160392,-0.0655785488982472,-0.00518301763610282,
0.0552125136260416,0.115608044888186,0.17600357615033,0.236399107412475,
0.296794638674619,0.297794018458462),.UNSPECIFIED.);
#7559=B_SPLINE_CURVE_WITH_KNOTS('',3,(#41042,#41043,#41044,#41045,#41046,
#41047),.UNSPECIFIED.,.F.,.F.,(4,2,4),(0.292787369885449,0.307160673946825,
0.361386326815235),.UNSPECIFIED.);
#7560=B_SPLINE_CURVE_WITH_KNOTS('',3,(#41049,#41050,#41051,#41052,#41053),
 .UNSPECIFIED.,.F.,.F.,(4,1,4),(-0.297985235446007,0.0164065923085981,0.299498223131783),
 .UNSPECIFIED.);
#7561=B_SPLINE_CURVE_WITH_KNOTS('',3,(#41055,#41056,#41057,#41058),
 .UNSPECIFIED.,.F.,.F.,(4,4),(0.297985235446007,0.361048915455649),
 .UNSPECIFIED.);
#7562=B_SPLINE_CURVE_WITH_KNOTS('',3,(#41060,#41061,#41062,#41063,#41064,
#41065,#41066,#41067),.UNSPECIFIED.,.F.,.F.,(4,2,2,4),(-0.329193263838381,
-0.328202711224253,0.275040863381023,0.32931292451793),.UNSPECIFIED.);
#7563=B_SPLINE_CURVE_WITH_KNOTS('',3,(#41068,#41069,#41070,#41071),
 .UNSPECIFIED.,.F.,.F.,(4,4),(-0.330172300337303,-0.314285888542252),
 .UNSPECIFIED.);
#7564=B_SPLINE_CURVE_WITH_KNOTS('',3,(#41074,#41075,#41076,#41077,#41078,
#41079,#41080,#41081,#41082,#41083,#41084,#41085,#41086,#41087,#41088,#41089,
#41090,#41091,#41092,#41093,#41094,#41095,#41096,#41097,#41098,#41099,#41100,
#41101,#41102,#41103,#41104,#41105,#41106,#41107,#41108,#41109,#41110,#41111,
#41112,#41113,#41114,#41115,#41116,#41117,#41118,#41119,#41120,#41121,#41122,
#41123,#41124,#41125,#41126,#41127,#41128,#41129,#41130,#41131),
 .UNSPECIFIED.,.F.,.F.,(4,3,3,3,3,3,3,3,3,3,3,3,3,3,3,3,3,3,3,4),(0.922264651271228,
0.95196229570932,0.980227193678782,0.985427844641358,1.01109405489662,1.03772298675017,
1.06426603988274,1.07002883462318,1.08636335889452,1.11299901067983,1.14013007212248,
1.14501308601341,1.17206434693218,1.19916477205921,1.2038740932211,1.21783674573549,
1.2452436598711,1.27296352011674,1.27880009503193,1.29174070129165),
 .UNSPECIFIED.);
#7565=B_SPLINE_CURVE_WITH_KNOTS('',3,(#41133,#41134,#41135,#41136,#41137,
#41138,#41139,#41140,#41141,#41142,#41143),.UNSPECIFIED.,.F.,.F.,(4,1,1,
1,1,1,1,1,4),(0.076362086282034,0.245533853727799,0.330119737450682,0.414705621173564,
0.583877388619329,0.668463272342212,0.753049156065094,0.795342097926536,
0.922220923510859),.UNSPECIFIED.);
#7566=B_SPLINE_CURVE_WITH_KNOTS('',3,(#41144,#41145,#41146,#41147,#41148,
#41149,#41150,#41151,#41152,#41153,#41154,#41155,#41156),.UNSPECIFIED.,
 .F.,.F.,(4,3,3,3,4),(0.,0.0131413461079839,0.0403155240278326,0.046632901256244,
0.076362086282034),.UNSPECIFIED.);
#7567=B_SPLINE_CURVE_WITH_KNOTS('',3,(#41363,#41364,#41365,#41366,#41367),
 .UNSPECIFIED.,.F.,.F.,(4,1,4),(-1.,-0.571428571428571,0.),
 .UNSPECIFIED.);
#7568=B_SPLINE_CURVE_WITH_KNOTS('',3,(#41369,#41370,#41371,#41372,#41373,
#41374),.UNSPECIFIED.,.F.,.F.,(4,1,1,4),(0.,0.207003520287941,0.310505280431912,
0.414007040575882),.UNSPECIFIED.);
#7569=B_SPLINE_CURVE_WITH_KNOTS('',3,(#41376,#41377,#41378,#41379,#41380),
 .UNSPECIFIED.,.F.,.F.,(4,1,4),(0.41430190159583,0.800342864550781,1.18640341854514),
 .UNSPECIFIED.);
#7570=B_SPLINE_CURVE_WITH_KNOTS('',3,(#41382,#41383,#41384,#41385),
 .UNSPECIFIED.,.F.,.F.,(4,4),(1.18667868852568,1.79026296795331),
 .UNSPECIFIED.);
#7571=B_SPLINE_CURVE_WITH_KNOTS('',3,(#41387,#41388,#41389,#41390),
 .UNSPECIFIED.,.F.,.F.,(4,4),(1.79056374069951,2.37790470859936),
 .UNSPECIFIED.);
#7572=B_SPLINE_CURVE_WITH_KNOTS('',3,(#41392,#41393,#41394,#41395),
 .UNSPECIFIED.,.F.,.F.,(4,4),(2.37819810334092,3.06372105803577),
 .UNSPECIFIED.);
#7573=B_SPLINE_CURVE_WITH_KNOTS('',3,(#41397,#41398,#41399,#41400,#41401),
 .UNSPECIFIED.,.F.,.F.,(4,1,4),(3.06374723112025,4.26766323501505,5.47160541199434),
 .UNSPECIFIED.);
#7574=B_SPLINE_CURVE_WITH_KNOTS('',3,(#41403,#41404,#41405,#41406,#41407,
#41408,#41409,#41410,#41411,#41412,#41413,#41414,#41415,#41416,#41417,#41418,
#41419,#41420,#41421,#41422,#41423,#41424,#41425,#41426,#41427,#41428,#41429,
#41430,#41431,#41432,#41433,#41434,#41435,#41436,#41437,#41438,#41439,#41440,
#41441,#41442,#41443,#41444,#41445,#41446,#41447,#41448,#41449,#41450,#41451,
#41452,#41453,#41454),.UNSPECIFIED.,.F.,.F.,(4,3,3,3,3,3,3,3,3,3,3,3,3,
3,3,3,3,4),(5.47162410746305,5.47176153560927,5.52922135523733,5.57009016359045,
5.58683833384667,5.64822065753784,5.66347324806546,5.72523068157049,5.78644857689101,
5.83662615005217,5.83886338715682,5.90578533070501,5.97118984657676,5.99390868625701,
6.00292892981675,6.0644494923277,6.1289173026227,6.15867754990177),
 .UNSPECIFIED.);
#7575=B_SPLINE_CURVE_WITH_KNOTS('',3,(#41456,#41457,#41458,#41459,#41460,
#41461,#41462,#41463,#41464,#41465,#41466,#41467,#41468,#41469,#41470,#41471,
#41472,#41473,#41474,#41475,#41476,#41477,#41478,#41479,#41480,#41481,#41482,
#41483,#41484,#41485,#41486,#41487,#41488,#41489,#41490,#41491,#41492,#41493,
#41494,#41495,#41496,#41497,#41498,#41499,#41500,#41501,#41502,#41503,#41504,
#41505,#41506,#41507,#41508,#41509,#41510,#41511,#41512,#41513,#41514,#41515,
#41516),.UNSPECIFIED.,.F.,.F.,(4,3,3,3,3,3,3,3,3,3,3,3,3,3,3,3,3,3,3,3,
4),(6.15871642666174,6.15875530745073,6.17769523512538,6.19663516280003,
6.19981654499319,6.22890881990579,6.23445739445574,6.28406964878603,6.30977254860284,
6.36393898412319,6.4210906697559,6.45115001888933,6.4580679089126,6.52098880059716,
6.5825270089927,6.59738625338311,6.63690964823477,6.67050437063,6.70043365602453,
6.7287738754379,6.74301820316605),.UNSPECIFIED.);
#7576=B_SPLINE_CURVE_WITH_KNOTS('',3,(#41518,#41519,#41520,#41521,#41522,
#41523,#41524),.UNSPECIFIED.,.F.,.F.,(4,1,1,1,4),(6.74362248787689,6.88868570629297,
7.03374892470906,7.17881214312514,7.32387536154123),.UNSPECIFIED.);
#7577=B_SPLINE_CURVE_WITH_KNOTS('',3,(#41526,#41527,#41528,#41529,#41530,
#41531,#41532,#41533),.UNSPECIFIED.,.F.,.F.,(4,1,1,1,1,4),(7.32434227776303,
7.70189518745276,7.89090510040853,7.98541005688641,8.03266253512535,8.0799150133643),
 .UNSPECIFIED.);
#7578=B_SPLINE_CURVE_WITH_KNOTS('',3,(#41534,#41535,#41536,#41537,#41538,
#41539,#41540),.UNSPECIFIED.,.F.,.F.,(4,1,1,1,4),(8.08029222326494,8.44983649077903,
8.81975796819377,9.1896794456085,9.55960092302324),.UNSPECIFIED.);
#7579=B_SPLINE_CURVE_WITH_KNOTS('',3,(#52343,#52344,#52345,#52346,#52347,
#52348,#52349,#52350,#52351),.UNSPECIFIED.,.F.,.F.,(4,1,1,1,1,1,4),(0.,
0.208981284264062,0.626943852792187,0.835925137056249,1.04490642132031,
1.25388770558437,1.46286897295086),.UNSPECIFIED.);
#7580=B_SPLINE_CURVE_WITH_KNOTS('',3,(#52353,#52354,#52355,#52356,#52357,
#52358,#52359,#52360,#52361,#52362,#52363),.UNSPECIFIED.,.F.,.F.,(4,1,1,
1,1,1,1,1,4),(2.19155818661609,2.25090656855756,2.280580760587,2.31025495261644,
2.32509204863116,2.33992914464588,2.36960333667532,2.48830010479308,2.60699687291084),
 .UNSPECIFIED.);
#7581=B_SPLINE_CURVE_WITH_KNOTS('',3,(#52365,#52366,#52367,#52368,#52369,
#52370,#52371,#52372,#52373,#52374,#52375,#52376,#52377,#52378,#52379,#52380,
#52381,#52382,#52383,#52384,#52385,#52386,#52387,#52388,#52389,#52390,#52391,
#52392,#52393,#52394,#52395,#52396,#52397,#52398,#52399,#52400,#52401,#52402,
#52403,#52404,#52405,#52406,#52407,#52408,#52409,#52410,#52411,#52412,#52413,
#52414,#52415,#52416,#52417,#52418,#52419,#52420,#52421,#52422,#52423,#52424,
#52425,#52426,#52427,#52428,#52429,#52430,#52431,#52432,#52433,#52434,#52435,
#52436,#52437,#52438,#52439,#52440,#52441,#52442,#52443,#52444,#52445,#52446,
#52447,#52448,#52449),.UNSPECIFIED.,.F.,.F.,(4,3,3,3,3,3,3,3,3,3,3,3,3,
3,3,3,3,3,3,3,3,3,3,3,3,3,3,3,4),(2.10087562040851,2.10088372270372,2.10247346027013,
2.10307601393069,2.10530413110765,2.10956542752656,2.1098519820788,2.11383027239681,
2.1191966968775,2.12453719979532,2.12678492441379,2.12874159509156,2.13208059695754,
2.13544318756292,2.13854861386098,2.13973957643076,2.14058122681814,2.14566146932938,
2.1509697282011,2.15269422844774,2.15809938906919,2.16160847183393,2.16688124293776,
2.17213694886275,2.17745117941117,2.18283434334936,2.18837389162331,2.19070800154593,
2.1915581843749),.UNSPECIFIED.);
#7582=B_SPLINE_CURVE_WITH_KNOTS('',3,(#52451,#52452,#52453,#52454,#52455,
#52456,#52457,#52458,#52459,#52460,#52461,#52462,#52463,#52464,#52465,#52466,
#52467,#52468,#52469,#52470,#52471,#52472,#52473,#52474,#52475,#52476,#52477,
#52478,#52479,#52480,#52481,#52482,#52483,#52484,#52485,#52486,#52487,#52488,
#52489,#52490,#52491,#52492,#52493,#52494,#52495,#52496,#52497,#52498,#52499,
#52500,#52501,#52502,#52503,#52504,#52505,#52506,#52507,#52508,#52509,#52510,
#52511,#52512,#52513,#52514,#52515,#52516,#52517,#52518,#52519,#52520,#52521,
#52522,#52523,#52524,#52525,#52526,#52527,#52528,#52529),.UNSPECIFIED.,
 .F.,.F.,(4,3,3,3,3,3,3,3,3,3,3,3,3,3,3,3,3,3,3,3,3,3,3,3,3,3,4),(2.03661045158091,
2.04096442896004,2.04146916453237,2.04613737339918,2.05268993684172,2.05312613965519,
2.05483225415638,2.05497936272896,2.05614902505797,2.05989669434489,2.06181300865997,
2.06416787026005,2.06638674823242,2.06835564146826,2.06972997740258,2.07334448964751,
2.07503624001787,2.07828886994786,2.08055225390468,2.08251295441833,2.08611159999046,
2.09083174338144,2.09155081643771,2.09169749444627,2.09495872614039,2.10019830691549,
2.10087562037779),.UNSPECIFIED.);
#7583=B_SPLINE_CURVE_WITH_KNOTS('',3,(#52531,#52532,#52533,#52534,#52535,
#52536,#52537,#52538),.UNSPECIFIED.,.F.,.F.,(4,1,1,1,1,4),(1.96650114296421,
1.97401285460172,1.97651675848088,1.98653237399755,2.00656360503089,2.03661045158091),
 .UNSPECIFIED.);
#7584=B_SPLINE_CURVE_WITH_KNOTS('',3,(#52540,#52541,#52542,#52543),
 .UNSPECIFIED.,.F.,.F.,(4,4),(1.9008556588209,1.96650114296421),
 .UNSPECIFIED.);
#7585=B_SPLINE_CURVE_WITH_KNOTS('',3,(#52545,#52546,#52547,#52548,#52549,
#52550,#52551,#52552,#52553,#52554,#52555,#52556,#52557,#52558,#52559,#52560,
#52561,#52562,#52563,#52564,#52565,#52566,#52567,#52568,#52569,#52570,#52571,
#52572,#52573,#52574,#52575,#52576,#52577,#52578,#52579,#52580,#52581,#52582,
#52583,#52584,#52585,#52586,#52587,#52588,#52589,#52590,#52591,#52592,#52593,
#52594,#52595,#52596,#52597,#52598,#52599,#52600,#52601,#52602,#52603,#52604,
#52605,#52606,#52607,#52608),.UNSPECIFIED.,.F.,.F.,(4,3,3,3,3,3,3,3,3,3,
3,3,3,3,3,3,3,3,3,3,3,4),(1.82758374932864,1.83223656565234,1.83571939203226,
1.83805116497033,1.84328487279121,1.84723441497955,1.84752017146434,1.85145117989987,
1.85343502410761,1.85550702434553,1.85898599625385,1.85962279895688,1.86512727908069,
1.8703298765575,1.87389394219687,1.878955199903,1.87992082753738,1.8853048835742,
1.89038824317914,1.89383938180255,1.89888316294158,1.90085565882082),
 .UNSPECIFIED.);
#7586=B_SPLINE_CURVE_WITH_KNOTS('',3,(#52610,#52611,#52612,#52613,#52614,
#52615,#52616,#52617),.UNSPECIFIED.,.F.,.F.,(4,2,2,4),(0.,0.115811547018689,
0.233145512161403,0.495737219621106),.UNSPECIFIED.);
#7587=B_SPLINE_CURVE_WITH_KNOTS('',3,(#52619,#52620,#52621,#52622,#52623,
#52624,#52625,#52626,#52627,#52628,#52629,#52630,#52631,#52632,#52633,#52634,
#52635,#52636,#52637,#52638,#52639,#52640,#52641,#52642,#52643,#52644,#52645,
#52646,#52647,#52648,#52649,#52650,#52651,#52652,#52653,#52654,#52655,#52656,
#52657,#52658,#52659,#52660,#52661,#52662,#52663,#52664,#52665,#52666,#52667,
#52668,#52669,#52670,#52671,#52672,#52673,#52674,#52675,#52676,#52677,#52678,
#52679,#52680,#52681,#52682,#52683,#52684,#52685,#52686,#52687,#52688,#52689,
#52690,#52691,#52692,#52693,#52694,#52695,#52696,#52697,#52698,#52699,#52700,
#52701,#52702,#52703),.UNSPECIFIED.,.F.,.F.,(4,3,3,3,3,3,3,3,3,3,3,3,3,
3,3,3,3,3,3,3,3,3,3,3,3,3,3,3,4),(1.56845677768168,1.57875898200853,1.5902875236116,
1.60181606521468,1.6232153440662,1.64400711162625,1.65649115942018,1.66853464029784,
1.67051171542687,1.69446829604668,1.70189392783942,1.71857357161021,1.73390383611253,
1.735253215381,1.7372376198041,1.7435930372664,1.74883573095845,1.75193285915179,
1.7525462632204,1.75878493231427,1.76473025775148,1.76861250292259,1.774746297528,
1.78151033410548,1.78529214669338,1.79301009099815,1.79922230536369,1.8019717371715,
1.80197179046417),.UNSPECIFIED.);
#7588=B_SPLINE_CURVE_WITH_KNOTS('',3,(#52705,#52706,#52707,#52708,#52709,
#52710,#52711),.UNSPECIFIED.,.F.,.F.,(4,1,1,1,4),(1.43249195629979,1.45191550221026,
1.4616272751655,1.4907625940312,1.56845677767309),.UNSPECIFIED.);
#7589=B_SPLINE_CURVE_WITH_KNOTS('',3,(#52713,#52714,#52715,#52716,#52717,
#52718,#52719,#52720,#52721,#52722,#52723,#52724,#52725,#52726,#52727,#52728,
#52729,#52730,#52731,#52732,#52733,#52734,#52735,#52736,#52737,#52738,#52739,
#52740,#52741,#52742,#52743,#52744,#52745,#52746,#52747,#52748,#52749,#52750,
#52751,#52752,#52753,#52754,#52755,#52756,#52757,#52758,#52759,#52760,#52761,
#52762,#52763,#52764,#52765,#52766,#52767,#52768,#52769,#52770,#52771,#52772,
#52773,#52774,#52775,#52776,#52777,#52778,#52779,#52780,#52781,#52782),
 .UNSPECIFIED.,.F.,.F.,(4,3,3,3,3,3,3,3,3,3,3,3,3,3,3,3,3,3,3,3,3,3,3,4),
(1.26182357380732,1.26321146371325,1.27965145505579,1.28695964770261,1.30171395524456,
1.30640755132645,1.31070783169197,1.32482659735197,1.32772758608418,1.33496166264828,
1.34362369478369,1.34924187664357,1.35187874054377,1.35931072547827,1.36767009102177,
1.36865825613663,1.38372247757944,1.38551167246194,1.39144562654905,1.39591154434102,
1.40850579340837,1.41185992891419,1.41833945977598,1.43249195629979),
 .UNSPECIFIED.);
#7590=B_SPLINE_CURVE_WITH_KNOTS('',3,(#52784,#52785,#52786,#52787,#52788,
#52789,#52790,#52791,#52792,#52793,#52794,#52795,#52796,#52797,#52798,#52799,
#52800,#52801,#52802,#52803,#52804,#52805,#52806,#52807,#52808,#52809,#52810,
#52811,#52812,#52813,#52814,#52815,#52816,#52817,#52818,#52819,#52820,#52821,
#52822,#52823,#52824,#52825,#52826,#52827,#52828,#52829,#52830,#52831,#52832,
#52833,#52834,#52835,#52836,#52837,#52838,#52839,#52840,#52841,#52842,#52843,
#52844,#52845,#52846,#52847,#52848,#52849,#52850,#52851,#52852,#52853,#52854,
#52855,#52856,#52857,#52858,#52859,#52860,#52861,#52862,#52863,#52864,#52865,
#52866,#52867,#52868,#52869,#52870,#52871,#52872,#52873,#52874,#52875,#52876,
#52877,#52878,#52879,#52880,#52881,#52882,#52883,#52884,#52885,#52886,#52887,
#52888,#52889,#52890,#52891,#52892,#52893,#52894,#52895,#52896,#52897,#52898,
#52899,#52900,#52901,#52902,#52903,#52904,#52905,#52906,#52907),
 .UNSPECIFIED.,.F.,.F.,(4,3,3,3,3,3,3,3,3,3,3,3,3,3,3,3,3,3,3,3,3,3,3,3,
3,3,3,3,3,3,3,3,3,3,3,3,3,3,3,3,3,4),(0.756828437332379,0.758034303676285,
0.783022641448518,0.80599662056723,0.828970599685942,0.847245434940196,
0.865650791288596,0.884491811769908,0.887471652364765,0.901112762039505,
0.914245954975312,0.919148302627896,0.935599586414352,0.937183843216286,
0.958717360320901,0.973254924393068,0.995700399707761,1.00932600556985,
1.02736154615824,1.03637931645244,1.04539708674663,1.06072425960333,1.07628417862955,
1.09205523917646,1.10854629296799,1.11753924910019,1.12498697740592,1.13697906116791,
1.15138005679454,1.16628135084883,1.18230149406609,1.18968141145376,1.20308754755323,
1.20616298993056,1.2203814875239,1.22575249263054,1.23458163997862,1.24312622221273,
1.24848732199679,1.25626046603962,1.26177001350472,1.26182357380732),
 .UNSPECIFIED.);
#7591=B_SPLINE_CURVE_WITH_KNOTS('',3,(#52909,#52910,#52911,#52912,#52913,
#52914,#52915,#52916,#52917,#52918,#52919,#52920,#52921,#52922,#52923,#52924,
#52925,#52926,#52927,#52928,#52929,#52930,#52931,#52932,#52933,#52934,#52935,
#52936,#52937,#52938,#52939,#52940,#52941,#52942,#52943,#52944,#52945,#52946,
#52947,#52948,#52949,#52950,#52951,#52952,#52953,#52954,#52955,#52956,#52957,
#52958,#52959,#52960,#52961,#52962,#52963,#52964,#52965,#52966,#52967,#52968,
#52969,#52970,#52971,#52972,#52973,#52974,#52975,#52976,#52977,#52978,#52979,
#52980,#52981,#52982,#52983,#52984,#52985,#52986,#52987,#52988,#52989,#52990),
 .UNSPECIFIED.,.F.,.F.,(4,3,3,3,3,3,3,3,3,3,3,3,3,3,3,3,3,3,3,3,3,3,3,3,
3,3,3,4),(0.,0.039559842189632,0.0812965112238326,0.126691965812033,0.168113098584215,
0.21623669638068,0.255008832123529,0.297122618085817,0.324355044571019,
0.340152984197433,0.385149402756223,0.417620481855091,0.432473392761359,
0.483357467834262,0.537497172053552,0.540591740951699,0.571362633267615,
0.597869133211754,0.626131984061165,0.648710089142039,0.661547104722673,
0.678554902855057,0.689471163857318,0.702769263237209,0.720830101771721,
0.738829266170943,0.75573965977665,0.756828430570164),.UNSPECIFIED.);
#7592=B_SPLINE_CURVE_WITH_KNOTS('',3,(#52992,#52993,#52994,#52995,#52996,
#52997),.UNSPECIFIED.,.F.,.F.,(4,2,4),(1.03501879872334E-10,0.211555879027688,
0.425996794857508),.UNSPECIFIED.);
#7593=B_SPLINE_CURVE_WITH_KNOTS('',3,(#52999,#53000,#53001,#53002,#53003,
#53004,#53005,#53006,#53007),.UNSPECIFIED.,.F.,.F.,(4,1,1,1,1,1,4),(-1.10870576037865,
-1.01091721837057,-0.913128676362484,-0.815340134354398,-0.766445863350356,
-0.619763050338228,-0.424185972875504),.UNSPECIFIED.);
#7594=B_SPLINE_CURVE_WITH_KNOTS('',3,(#53009,#53010,#53011,#53012,#53013,
#53014,#53015,#53016,#53017,#53018),.UNSPECIFIED.,.F.,.F.,(4,1,1,1,1,1,
1,4),(-2.04907351897734,-1.91473526774895,-1.64605876529219,-1.5117205140638,
-1.37738226283542,-1.24304401160704,-1.17587488599285,-1.10870576037865),
 .UNSPECIFIED.);
#7595=B_SPLINE_CURVE_WITH_KNOTS('',3,(#53020,#53021,#53022,#53023,#53024,
#53025,#53026,#53027,#53028,#53029,#53030),.UNSPECIFIED.,.F.,.F.,(4,1,1,
1,1,1,1,1,4),(-3.79500099688023,-3.54558322444133,-3.04674665595333,-2.92203751383133,
-2.79732837170933,-2.67261922958733,-2.54791008746534,-2.29849180322134,
-2.04907351897734),.UNSPECIFIED.);
#7596=B_SPLINE_CURVE_WITH_KNOTS('',3,(#53032,#53033,#53034,#53035,#53036,
#53037,#53038,#53039,#53040,#53041,#53042,#53043,#53044,#53045,#53046,#53047,
#53048,#53049,#53050,#53051,#53052,#53053,#53054,#53055,#53056,#53057,#53058,
#53059,#53060,#53061,#53062,#53063,#53064,#53065,#53066,#53067,#53068,#53069,
#53070,#53071,#53072,#53073,#53074,#53075,#53076,#53077,#53078,#53079,#53080,
#53081,#53082,#53083,#53084,#53085,#53086,#53087,#53088,#53089,#53090,#53091,
#53092,#53093,#53094,#53095,#53096,#53097,#53098,#53099,#53100,#53101,#53102,
#53103,#53104,#53105,#53106,#53107,#53108,#53109,#53110,#53111,#53112,#53113,
#53114,#53115,#53116,#53117,#53118,#53119,#53120,#53121,#53122,#53123,#53124,
#53125),.UNSPECIFIED.,.F.,.F.,(4,3,3,3,3,3,3,3,3,3,3,3,3,3,3,3,3,3,3,3,
3,3,3,3,3,3,3,3,3,3,3,4),(-7.37893243484629,-7.09721253804601,-6.86694230253758,
-6.54165526017816,-6.25323500527255,-6.10927151562258,-5.88100661174727,
-5.84296203792017,-5.64313657722973,-5.45391307940915,-5.27371499028469,
-5.10400017747741,-5.04555890996164,-4.89298656830114,-4.81898177330275,
-4.64872543377383,-4.56298670714839,-4.50669086603314,-4.46698855734051,
-4.38699009916728,-4.30699164099404,-4.2439746894317,-4.17377747724209,
-4.1052835011459,-4.05099657483969,-4.00647424691738,-3.94815423137164,
-3.9004735048502,-3.87188483858507,-3.84491918341313,-3.81938938067703,
-3.79500153778596),.UNSPECIFIED.);
#7597=B_SPLINE_CURVE_WITH_KNOTS('',3,(#53127,#53128,#53129,#53130,#53131,
#53132,#53133,#53134,#53135,#53136,#53137,#53138,#53139,#53140,#53141,#53142,
#53143,#53144,#53145,#53146,#53147,#53148,#53149,#53150,#53151,#53152,#53153,
#53154,#53155,#53156,#53157,#53158,#53159,#53160,#53161,#53162,#53163,#53164,
#53165,#53166,#53167,#53168,#53169,#53170,#53171,#53172,#53173,#53174,#53175,
#53176,#53177,#53178,#53179,#53180,#53181,#53182,#53183,#53184,#53185,#53186,
#53187,#53188,#53189,#53190),.UNSPECIFIED.,.F.,.F.,(4,3,3,3,3,3,3,3,3,3,
3,3,3,3,3,3,3,3,3,3,3,4),(-13.6209854494249,-12.8511378970195,-12.0643898935444,
-11.3085768590722,-10.9458199140635,-10.4479935674583,-10.0540980442592,
-9.67335324653639,-9.31475312865825,-9.16237617445491,-8.77668431314733,
-8.42708589080824,-8.2706543046506,-8.04416328397843,-7.81656010161982,
-7.70334373657069,-7.58867356571361,-7.5400351581434,-7.47104988566852,
-7.40480342889605,-7.38202025346192,-7.37893251061186),.UNSPECIFIED.);
#7598=B_SPLINE_CURVE_WITH_KNOTS('',3,(#53192,#53193,#53194,#53195,#53196,
#53197,#53198,#53199),.UNSPECIFIED.,.F.,.F.,(4,1,1,1,1,4),(-20.9230961620266,
-17.7936201740765,-15.7073028487765,-14.6641441861265,-14.1425648548015,
-13.6209855234765),.UNSPECIFIED.);
#7599=B_SPLINE_CURVE_WITH_KNOTS('',3,(#53201,#53202,#53203,#53204,#53205,
#53206,#53207,#53208,#53209,#53210,#53211,#53212,#53213,#53214,#53215,#53216,
#53217,#53218,#53219,#53220,#53221,#53222,#53223,#53224,#53225,#53226,#53227,
#53228,#53229,#53230,#53231,#53232,#53233,#53234,#53235,#53236,#53237,#53238,
#53239,#53240,#53241,#53242,#53243,#53244,#53245,#53246,#53247,#53248,#53249,
#53250,#53251,#53252,#53253,#53254,#53255,#53256,#53257,#53258,#53259,#53260,
#53261,#53262,#53263,#53264,#53265,#53266,#53267,#53268,#53269,#53270,#53271,
#53272,#53273,#53274,#53275,#53276,#53277,#53278,#53279,#53280,#53281,#53282,
#53283,#53284,#53285,#53286,#53287,#53288,#53289,#53290,#53291,#53292,#53293,
#53294,#53295,#53296,#53297),.UNSPECIFIED.,.F.,.F.,(4,3,3,3,3,3,3,3,3,3,
3,3,3,3,3,3,3,3,3,3,3,3,3,3,3,3,3,3,3,3,3,3,4),(-29.2787346184417,-29.1096960603127,
-28.9240346326721,-28.7261490220601,-28.6427305271377,-28.6263089729943,
-28.4309678069006,-28.3150441010112,-28.2510346319925,-28.0852673066811,
-27.7865835801735,-27.7048845006206,-27.1030463193419,-26.3994219069812,
-26.2152821750297,-26.0888102114573,-25.6957974946206,-25.5456719507069,
-25.467698483279,-25.227004099114,-25.196215795191,-25.1722521850178,-24.8236888062035,
-24.5049209466192,-23.9082511095742,-23.4566708142076,-23.3115812725292,
-22.884956861632,-22.600429531231,-22.1810961889299,-22.0014436072201,-21.4779708271961,
-20.9230961620266),.UNSPECIFIED.);
#7600=B_SPLINE_CURVE_WITH_KNOTS('',3,(#53299,#53300,#53301,#53302,#53303,
#53304,#53305),.UNSPECIFIED.,.F.,.F.,(4,1,1,1,4),(-35.1303480341168,-33.4584584867811,
-31.7865689394453,-30.9506241657775,-29.2787346184417),.UNSPECIFIED.);
#7601=B_SPLINE_CURVE_WITH_KNOTS('',3,(#53307,#53308,#53309,#53310,#53311,
#53312,#53313,#53314,#53315,#53316,#53317,#53318,#53319,#53320,#53321,#53322,
#53323,#53324,#53325,#53326,#53327,#53328,#53329,#53330,#53331,#53332,#53333,
#53334,#53335,#53336,#53337,#53338,#53339,#53340,#53341,#53342,#53343,#53344,
#53345,#53346,#53347,#53348,#53349,#53350,#53351,#53352,#53353,#53354,#53355,
#53356,#53357,#53358,#53359,#53360,#53361,#53362,#53363,#53364,#53365,#53366,
#53367,#53368,#53369,#53370,#53371,#53372,#53373,#53374,#53375,#53376,#53377,
#53378,#53379,#53380,#53381,#53382,#53383,#53384,#53385,#53386,#53387,#53388,
#53389,#53390,#53391,#53392,#53393,#53394,#53395,#53396,#53397,#53398,#53399,
#53400,#53401,#53402,#53403,#53404,#53405,#53406,#53407,#53408,#53409,#53410,
#53411,#53412,#53413,#53414,#53415,#53416,#53417,#53418,#53419,#53420,#53421,
#53422,#53423,#53424,#53425,#53426,#53427,#53428,#53429,#53430,#53431,#53432,
#53433,#53434,#53435,#53436,#53437,#53438,#53439),.UNSPECIFIED.,.F.,.F.,
(4,3,3,3,3,3,3,3,3,3,3,3,3,3,3,3,3,3,3,3,3,3,3,3,3,3,3,3,3,3,3,3,3,3,3,
3,3,3,3,3,3,3,3,3,4),(-40.4542025593683,-40.2883379357545,-40.1291560510175,
-40.0863253858464,-39.7317546341407,-39.3799231675408,-39.1055719541562,
-38.9809430220555,-38.932487814856,-38.7733967870736,-38.6017505770459,
-38.38709626168,-38.3278541581916,-38.2684208184249,-38.172441946314,-38.0773070542021,
-38.015978412303,-37.8649593582531,-37.8489781650965,-37.8363222855412,
-37.6893279450614,-37.5506150705823,-37.5098081397409,-37.4119021961033,
-37.308503196221,-37.2599229565623,-37.0129942138183,-36.9983061965739,
-36.8094454257336,-36.7412333947959,-36.6544112504103,-36.5012970422284,
-36.3546539033726,-36.1589984452356,-36.1281858125416,-35.929935933668,
-35.8935455269148,-35.8445105517863,-35.7695403285612,-35.5371810458801,
-35.4574426980158,-35.314925666407,-35.27725046187,-35.1434968058668,-35.1303480341168),
 .UNSPECIFIED.);
#7602=B_SPLINE_CURVE_WITH_KNOTS('',3,(#53441,#53442,#53443,#53444,#53445,
#53446,#53447,#53448,#53449,#53450,#53451,#53452,#53453,#53454,#53455,#53456,
#53457,#53458,#53459,#53460,#53461,#53462,#53463,#53464,#53465,#53466,#53467,
#53468,#53469,#53470,#53471,#53472,#53473,#53474,#53475,#53476,#53477,#53478,
#53479,#53480,#53481,#53482,#53483,#53484,#53485,#53486,#53487,#53488,#53489,
#53490,#53491,#53492,#53493,#53494,#53495,#53496,#53497,#53498,#53499,#53500,
#53501,#53502,#53503,#53504,#53505,#53506,#53507,#53508,#53509,#53510,#53511,
#53512,#53513,#53514,#53515,#53516,#53517,#53518,#53519,#53520,#53521,#53522,
#53523,#53524,#53525,#53526,#53527,#53528,#53529,#53530,#53531,#53532,#53533,
#53534,#53535,#53536,#53537),.UNSPECIFIED.,.F.,.F.,(4,3,3,3,3,3,3,3,3,3,
3,3,3,3,3,3,3,3,3,3,3,3,3,3,3,3,3,3,3,3,3,3,4),(-52.076264422194,-52.0737402609872,
-51.1412180731238,-50.9105567633614,-50.6813407101697,-50.2280521562142,
-49.3467857029178,-49.298229902108,-48.9208946312172,-48.5057751083927,
-47.6156904523358,-47.0953817384218,-46.9581990673406,-46.257134327466,
-45.5668109774429,-44.8893364381591,-44.1815864308004,-43.7747932825737,
-42.9979057491396,-42.1621977116501,-42.1144990546496,-41.7255776485795,
-41.2843519406876,-41.0649893227899,-40.9009393220907,-40.7763014969501,
-40.7368893213915,-40.6649750650259,-40.5977989171732,-40.5344428881694,
-40.4755069476578,-40.4591070372058,-40.4542057498323),.UNSPECIFIED.);
#7603=B_SPLINE_CURVE_WITH_KNOTS('',3,(#53539,#53540,#53541,#53542,#53543),
 .UNSPECIFIED.,.F.,.F.,(4,1,4),(-66.1031756239825,-60.0916422517874,-52.076264422194),
 .UNSPECIFIED.);
#7604=B_SPLINE_CURVE_WITH_KNOTS('',3,(#53545,#53546,#53547,#53548),
 .UNSPECIFIED.,.F.,.F.,(4,4),(-75.2949305236969,-66.1031756239825),
 .UNSPECIFIED.);
#7605=B_SPLINE_CURVE_WITH_KNOTS('',3,(#53550,#53551,#53552,#53553,#53554,
#53555),.UNSPECIFIED.,.F.,.F.,(4,2,4),(0.,0.0420132838931537,0.0846653479954924),
 .UNSPECIFIED.);
#7606=B_SPLINE_CURVE_WITH_KNOTS('',3,(#53557,#53558,#53559,#53560,#53561,
#53562,#53563,#53564,#53565,#53566,#53567,#53568,#53569,#53570,#53571,#53572,
#53573,#53574),.UNSPECIFIED.,.F.,.F.,(4,1,1,1,1,1,1,1,1,1,1,1,1,1,1,4),
(0.,0.0536833715747986,0.107366743149597,0.161050114724396,0.214733486299194,
0.228154329192894,0.241575172086594,0.268416857873993,0.322100229448792,
0.37578360102359,0.429466972598389,0.509992029960587,0.590517087322785,
0.644200458897583,0.697883830472382,0.75156720204718),.UNSPECIFIED.);
#7607=B_SPLINE_CURVE_WITH_KNOTS('',3,(#53576,#53577,#53578,#53579,#53580,
#53581),.UNSPECIFIED.,.F.,.F.,(4,2,4),(0.,0.021085550105349,0.0417920803786918),
 .UNSPECIFIED.);
#7608=B_SPLINE_CURVE_WITH_KNOTS('',3,(#53583,#53584,#53585,#53586,#53587,
#53588,#53589,#53590,#53591,#53592,#53593,#53594),.UNSPECIFIED.,.F.,.F.,
(4,2,2,2,2,4),(0.,0.050505315546523,0.100790126577494,0.199632092084437,
0.400786097856356,0.745503643800359),.UNSPECIFIED.);
#7609=B_SPLINE_CURVE_WITH_KNOTS('',3,(#53596,#53597,#53598,#53599,#53600,
#53601,#53602,#53603,#53604,#53605,#53606,#53607,#53608,#53609,#53610,#53611,
#53612,#53613,#53614,#53615,#53616,#53617,#53618,#53619,#53620,#53621,#53622,
#53623,#53624,#53625,#53626,#53627,#53628,#53629,#53630,#53631,#53632,#53633,
#53634,#53635,#53636,#53637,#53638,#53639,#53640,#53641,#53642,#53643,#53644),
 .UNSPECIFIED.,.F.,.F.,(4,3,3,3,3,3,3,3,3,3,3,3,3,3,3,3,4),(6.63337020876143,
6.7190850448111,6.73676856887547,6.77580516745678,6.89645053985051,6.91763430915923,
7.16564608140866,7.19816645514471,7.4501548123097,7.55120883330657,7.59415354968106,
7.72134807390837,7.95982866477617,8.31850358376712,8.58822017944783,8.63541402258988,
8.77692550510397),.UNSPECIFIED.);
#7610=B_SPLINE_CURVE_WITH_KNOTS('',3,(#53646,#53647,#53648,#53649,#53650),
 .UNSPECIFIED.,.F.,.F.,(4,1,4),(4.69946777607289,5.80455488046634,6.63337020876143),
 .UNSPECIFIED.);
#7611=B_SPLINE_CURVE_WITH_KNOTS('',3,(#53652,#53653,#53654,#53655,#53656,
#53657,#53658,#53659,#53660,#53661,#53662,#53663,#53664,#53665,#53666,#53667,
#53668,#53669),.UNSPECIFIED.,.F.,.F.,(4,2,2,2,2,2,2,2,4),(5.5366310029957E-11,
0.170051968698641,0.346390851185846,0.408566423903585,0.45559735651897,
0.526633190057164,0.562379031383655,0.580309052858196,0.602548551079055),
 .UNSPECIFIED.);
#7612=B_SPLINE_CURVE_WITH_KNOTS('',3,(#53671,#53672,#53673,#53674,#53675,
#53676,#53677,#53678,#53679,#53680,#53681,#53682,#53683,#53684,#53685,#53686,
#53687,#53688,#53689,#53690,#53691,#53692,#53693,#53694,#53695,#53696,#53697,
#53698,#53699,#53700,#53701,#53702,#53703,#53704,#53705,#53706,#53707,#53708,
#53709,#53710,#53711,#53712,#53713,#53714,#53715,#53716,#53717,#53718,#53719,
#53720,#53721,#53722,#53723,#53724,#53725,#53726,#53727,#53728,#53729,#53730,
#53731,#53732,#53733,#53734,#53735,#53736,#53737,#53738,#53739,#53740,#53741,
#53742,#53743,#53744,#53745,#53746,#53747,#53748,#53749,#53750,#53751,#53752,
#53753,#53754,#53755,#53756,#53757,#53758,#53759,#53760,#53761,#53762,#53763,
#53764,#53765,#53766,#53767),.UNSPECIFIED.,.F.,.F.,(4,3,3,3,3,3,3,3,3,3,
3,3,3,3,3,3,3,3,3,3,3,3,3,3,3,3,3,3,3,3,3,3,4),(1.96419536172906,1.96505190012007,
2.00759893446084,2.05907348647213,2.14856512578498,2.16116833461418,2.1995405412518,
2.29009841588943,2.31368035746746,2.34538948007777,2.43488572077454,2.56742771999767,
2.67023090029728,2.67502081956359,2.75992963007049,2.83275285494525,2.90048454253916,
2.90557607982002,2.9770366712957,3.04749917809138,3.10307095323777,3.12007497461443,
3.14092125934276,3.20896093626124,3.27403989704861,3.33678902877863,3.3762664388655,
3.37737317695638,3.45628612936796,3.53381374195537,3.60353111799624,3.61134135454277,
3.61161161790059),.UNSPECIFIED.);
#7613=B_SPLINE_CURVE_WITH_KNOTS('',3,(#53769,#53770,#53771,#53772,#53773,
#53774,#53775,#53776,#53777,#53778,#53779,#53780,#53781,#53782,#53783,#53784,
#53785,#53786,#53787,#53788,#53789,#53790,#53791,#53792,#53793,#53794,#53795,
#53796,#53797,#53798,#53799,#53800,#53801,#53802,#53803,#53804,#53805,#53806,
#53807,#53808,#53809,#53810,#53811,#53812,#53813,#53814,#53815,#53816,#53817,
#53818,#53819,#53820,#53821,#53822,#53823,#53824,#53825,#53826,#53827,#53828,
#53829,#53830,#53831,#53832,#53833,#53834,#53835,#53836,#53837,#53838,#53839,
#53840,#53841,#53842,#53843,#53844,#53845,#53846,#53847,#53848,#53849,#53850,
#53851,#53852,#53853,#53854,#53855,#53856,#53857,#53858,#53859,#53860,#53861,
#53862,#53863,#53864,#53865),.UNSPECIFIED.,.F.,.F.,(4,3,3,3,3,3,3,3,3,3,
3,3,3,3,3,3,3,3,3,3,3,3,3,3,3,3,3,3,3,3,3,3,4),(0.,1.8138297394372E-5,0.121063268185862,
0.17473067075732,0.307769204317186,0.337354379440942,0.449276527110338,
0.552000632372627,0.561198674779733,0.602830722877044,0.699305190558911,
0.701498343474666,0.823662523240613,0.841798012169599,0.955815263928068,
0.982097680864532,1.06417937027259,1.11100143720994,1.12239734955947,1.22569592643638,
1.32149205669811,1.32899450331328,1.40299668694933,1.42878061011154,1.50546259251116,
1.55154822774982,1.62807430325076,1.6835960243392,1.77144305862835,1.79740964584924,
1.87394598522444,1.9554396253416,1.96419535735387),.UNSPECIFIED.);
#7614=B_SPLINE_CURVE_WITH_KNOTS('',3,(#53867,#53868,#53869,#53870,#53871,
#53872,#53873,#53874,#53875,#53876,#53877,#53878,#53879),.UNSPECIFIED.,
 .F.,.F.,(4,1,1,1,1,1,1,1,1,1,4),(6.5071186511175,6.712779658626,6.91844066613449,
6.96985591801162,7.02127116988874,7.22693217739724,7.32976268115149,7.48400843678286,
7.53542368865998,7.74108469616848,7.94674570367697),.UNSPECIFIED.);
#7615=B_SPLINE_CURVE_WITH_KNOTS('',3,(#53881,#53882,#53883,#53884,#53885,
#53886,#53887,#53888,#53889),.UNSPECIFIED.,.F.,.F.,(4,1,1,1,1,1,4),(4.87949997638846,
5.11201692992118,5.57705083698662,5.80956779051934,6.04208474405206,6.27460169758478,
6.5071186511175),.UNSPECIFIED.);
#7616=B_SPLINE_CURVE_WITH_KNOTS('',3,(#53891,#53892,#53893,#53894,#53895,
#53896,#53897),.UNSPECIFIED.,.F.,.F.,(4,1,1,1,4),(2.69094642325915,3.62889794602885,
4.25419896120866,4.56684946879856,4.87949997638846),.UNSPECIFIED.);
#7617=B_SPLINE_CURVE_WITH_KNOTS('',3,(#53899,#53900,#53901,#53902,#53903,
#53904,#53905,#53906,#53907,#53908,#53909,#53910,#53911,#53912,#53913,#53914,
#53915,#53916,#53917,#53918,#53919,#53920,#53921,#53922,#53923,#53924,#53925,
#53926,#53927,#53928,#53929,#53930,#53931,#53932,#53933,#53934,#53935,#53936,
#53937,#53938,#53939,#53940,#53941,#53942,#53943,#53944,#53945,#53946,#53947,
#53948,#53949,#53950,#53951,#53952,#53953,#53954,#53955,#53956,#53957,#53958,
#53959,#53960,#53961,#53962,#53963,#53964,#53965,#53966,#53967,#53968,#53969,
#53970,#53971,#53972,#53973,#53974,#53975,#53976,#53977,#53978,#53979,#53980,
#53981,#53982,#53983,#53984,#53985,#53986,#53987,#53988,#53989,#53990,#53991,
#53992,#53993,#53994,#53995,#53996,#53997,#53998),.UNSPECIFIED.,.F.,.F.,
(4,3,3,3,3,3,3,3,3,3,3,3,3,3,3,3,3,3,3,3,3,3,3,3,3,3,3,3,3,3,3,3,3,4),(1.28454933342625,
1.284663099846,1.32335780443299,1.33323468515429,1.34320009665895,1.36341289207583,
1.40509748435979,1.42665711008932,1.44876554198746,1.4998586819635,1.54419214844141,
1.59590059132183,1.64959023195339,1.65716554088604,1.68637707337851,1.75981977009417,
1.84800901712936,1.88729094335464,1.92692609574672,1.93751941084867,1.9877478783427,
2.07341022478126,2.08212877066919,2.08820481333076,2.24310543462275,2.28911868330689,
2.38245055444688,2.50274947638037,2.53443926298747,2.59672405888692,2.61222200346954,
2.65158421336434,2.68765429596537,2.69094642325915),.UNSPECIFIED.);
#7618=B_SPLINE_CURVE_WITH_KNOTS('',3,(#54000,#54001,#54002,#54003,#54004,
#54005,#54006),.UNSPECIFIED.,.F.,.F.,(4,1,1,1,4),(0.675577463735769,0.762573445120124,
0.936565407888833,1.11055737065754,1.28454933342625),.UNSPECIFIED.);
#7619=B_SPLINE_CURVE_WITH_KNOTS('',3,(#54008,#54009,#54010,#54011,#54012,
#54013,#54014,#54015,#54016,#54017,#54018,#54019,#54020,#54021,#54022,#54023,
#54024,#54025,#54026,#54027,#54028,#54029,#54030,#54031,#54032,#54033,#54034,
#54035,#54036,#54037,#54038,#54039,#54040,#54041,#54042,#54043,#54044,#54045,
#54046,#54047,#54048,#54049,#54050,#54051,#54052,#54053,#54054,#54055,#54056,
#54057,#54058,#54059,#54060,#54061,#54062),.UNSPECIFIED.,.F.,.F.,(4,3,3,
3,3,3,3,3,3,3,3,3,3,3,3,3,3,3,4),(0.0412699530928034,0.0821005929720136,
0.127945523936301,0.168857136488049,0.20941548589726,0.22294409466857,0.269878070913077,
0.316812047157585,0.355434901557536,0.364399147418465,0.383769517079644,
0.404141522876379,0.451848303292714,0.459901618097689,0.522642871293701,
0.532913366941116,0.604380509650793,0.639978986693281,0.675577463735768),
 .UNSPECIFIED.);
#7620=B_SPLINE_CURVE_WITH_KNOTS('',3,(#54064,#54065,#54066,#54067),
 .UNSPECIFIED.,.F.,.F.,(4,4),(0.,0.0412699530886637),.UNSPECIFIED.);
#7621=B_SPLINE_CURVE_WITH_KNOTS('',3,(#54069,#54070,#54071,#54072,#54073,
#54074,#54075,#54076,#54077,#54078,#54079,#54080,#54081,#54082,#54083,#54084,
#54085,#54086,#54087,#54088,#54089,#54090,#54091,#54092,#54093,#54094),
 .UNSPECIFIED.,.F.,.F.,(4,1,1,1,1,1,1,1,1,1,1,1,1,1,1,1,1,1,1,1,1,1,1,4),
(0.,0.0539979975781232,0.107995995156246,0.215991990312493,0.269989987890616,
0.323987985468739,0.377985983046862,0.431983980624985,0.458982979414047,
0.472482478808578,0.485981978203109,0.49948147759764,0.51298097699217,0.519730726689436,
0.521418164113752,0.526480476386701,0.529855351235334,0.533230226083967,
0.536605100932599,0.538292538356915,0.539979975781232,0.593977973359355,
0.647975970937478,0.755971966093725),.UNSPECIFIED.);
#7622=B_SPLINE_CURVE_WITH_KNOTS('',3,(#54096,#54097,#54098,#54099),
 .UNSPECIFIED.,.F.,.F.,(4,4),(-0.0833603842763953,0.),.UNSPECIFIED.);
#7623=B_SPLINE_CURVE_WITH_KNOTS('',3,(#54101,#54102,#54103,#54104,#54105,
#54106),.UNSPECIFIED.,.F.,.F.,(4,1,1,4),(-0.799336073509661,-0.594771590871585,
-0.39020710823351,-0.0833603842763964),.UNSPECIFIED.);
#7624=B_SPLINE_CURVE_WITH_KNOTS('',3,(#54108,#54109,#54110,#54111,#54112,
#54113,#54114,#54115,#54116,#54117,#54118,#54119,#54120,#54121,#54122,#54123),
 .UNSPECIFIED.,.F.,.F.,(4,2,2,2,2,2,2,4),(0.0118379321062938,0.107024163210369,
0.335817375141192,0.559775143232002,0.672782851896336,0.729545183131027,
0.757993915544536,0.787301420911162),.UNSPECIFIED.);
#7625=B_SPLINE_CURVE_WITH_KNOTS('',3,(#54125,#54126,#54127,#54128,#54129,
#54130),.UNSPECIFIED.,.F.,.F.,(4,1,1,4),(-3.17329134625142,-3.0004111005852,
-2.65465060925274,-1.96312962658784),.UNSPECIFIED.);
#7626=B_SPLINE_CURVE_WITH_KNOTS('',3,(#54132,#54133,#54134,#54135,#54136,
#54137),.UNSPECIFIED.,.F.,.F.,(4,1,1,4),(-4.08237667107798,-3.69276867472374,
-3.43303001048758,-3.17329134625142),.UNSPECIFIED.);
#7627=B_SPLINE_CURVE_WITH_KNOTS('',3,(#54139,#54140,#54141,#54142,#54143,
#54144,#54145,#54146,#54147,#54148,#54149,#54150,#54151,#54152,#54153,#54154,
#54155,#54156,#54157,#54158,#54159,#54160,#54161,#54162,#54163,#54164,#54165,
#54166,#54167,#54168,#54169,#54170,#54171,#54172,#54173,#54174,#54175,#54176,
#54177,#54178,#54179,#54180,#54181,#54182,#54183,#54184,#54185,#54186,#54187,
#54188,#54189,#54190,#54191,#54192,#54193,#54194,#54195,#54196,#54197,#54198,
#54199,#54200,#54201,#54202,#54203,#54204,#54205,#54206,#54207,#54208,#54209,
#54210,#54211),.UNSPECIFIED.,.F.,.F.,(4,3,3,3,3,3,3,3,3,3,3,3,3,3,3,3,3,
3,3,3,3,3,3,3,4),(-5.24963523804274,-5.22555794291826,-5.19586107911791,
-5.18687812799744,-5.14098553954611,-5.12430645426268,-5.08288401419063,
-5.01504766740605,-4.99102394383036,-4.91855573999006,-4.84257002484868,
-4.76122999602307,-4.74938156648641,-4.68977118521554,-4.60201605684906,
-4.51864743190061,-4.48764588312174,-4.41261409008418,-4.37103514543172,
-4.30477017347109,-4.24196226368263,-4.18335539931493,-4.16463763971098,
-4.11019379776344,-4.08237667199167),.UNSPECIFIED.);
#7628=B_SPLINE_CURVE_WITH_KNOTS('',3,(#54213,#54214,#54215,#54216,#54217,
#54218,#54219),.UNSPECIFIED.,.F.,.F.,(4,1,1,1,4),(-6.31492339087005,-6.01055536310239,
-5.85837133809046,-5.5540032880666,-5.24963523804274),.UNSPECIFIED.);
#7629=B_SPLINE_CURVE_WITH_KNOTS('',3,(#54221,#54222,#54223,#54224,#54225,
#54226,#54227,#54228,#54229,#54230,#54231,#54232,#54233,#54234,#54235,#54236,
#54237,#54238,#54239,#54240,#54241,#54242,#54243,#54244,#54245,#54246,#54247,
#54248,#54249,#54250,#54251,#54252,#54253,#54254,#54255,#54256,#54257,#54258,
#54259,#54260,#54261,#54262,#54263,#54264,#54265,#54266,#54267,#54268,#54269,
#54270,#54271,#54272,#54273,#54274,#54275,#54276,#54277,#54278,#54279,#54280,
#54281,#54282,#54283,#54284),.UNSPECIFIED.,.F.,.F.,(4,3,3,3,3,3,3,3,3,3,
3,3,3,3,3,3,3,3,3,3,3,4),(-7.69657824876369,-7.69585220010023,-7.63949305537026,
-7.5897176515031,-7.56210720609799,-7.48884902843925,-7.43938651036202,
-7.32366994771237,-7.30181972429585,-7.22643881215268,-7.10444046206193,
-7.091900638509,-6.97438837483062,-6.90706119982801,-6.89058485139341,-6.80837156871105,
-6.74329402873901,-6.70968193759409,-6.54917179381872,-6.51230267536017,
-6.37970879985935,-6.31492341362349),.UNSPECIFIED.);
#7630=B_SPLINE_CURVE_WITH_KNOTS('',3,(#54286,#54287,#54288,#54289,#54290,
#54291,#54292,#54293,#54294),.UNSPECIFIED.,.F.,.F.,(4,1,1,1,1,1,4),(-10.2944961530174,
-9.9233650238383,-9.5522338946592,-9.18110276548009,-8.43884050712189,-8.06770937794279,
-7.69657825451453),.UNSPECIFIED.);
#7631=B_SPLINE_CURVE_WITH_KNOTS('',3,(#54296,#54297,#54298,#54299,#54300,
#54301,#54302,#54303),.UNSPECIFIED.,.F.,.F.,(4,1,1,1,1,4),(-11.9813316832122,
-11.8608434310554,-11.7403551788986,-11.2584021702716,-10.7764491616445,
-10.2944961530174),.UNSPECIFIED.);
#7632=B_SPLINE_CURVE_WITH_KNOTS('',3,(#54305,#54306,#54307,#54308,#54309,
#54310,#54311,#54312,#54313,#54314),.UNSPECIFIED.,.F.,.F.,(4,1,1,1,1,1,
1,4),(-16.6980910490008,-16.0242682824596,-14.6766227493771,-14.0027999828359,
-13.3289772162947,-12.6551544497534,-12.3182430664828,-11.9813316832122),
 .UNSPECIFIED.);
#7633=B_SPLINE_CURVE_WITH_KNOTS('',3,(#54316,#54317,#54318,#54319,#54320,
#54321,#54322,#54323,#54324),.UNSPECIFIED.,.F.,.F.,(4,1,1,1,1,1,4),(-21.7463678506673,
-21.0251854504292,-19.5828206499531,-18.861638249715,-18.140455849477,-17.4192734492389,
-16.6980910490008),.UNSPECIFIED.);
#7634=B_SPLINE_CURVE_WITH_KNOTS('',3,(#54326,#54327,#54328,#54329,#54330,
#54331,#54332),.UNSPECIFIED.,.F.,.F.,(4,1,1,1,4),(-25.457976371469,-24.3975168143727,
-23.8672870216316,-22.8068274361495,-21.7463678506673),.UNSPECIFIED.);
#7635=B_SPLINE_CURVE_WITH_KNOTS('',3,(#54334,#54335,#54336,#54337,#54338,
#54339,#54340,#54341),.UNSPECIFIED.,.F.,.F.,(4,2,2,4),(0.,0.213844974168118,
0.318336498142317,0.426627456126852),.UNSPECIFIED.);
#7636=B_SPLINE_CURVE_WITH_KNOTS('',3,(#54343,#54344,#54345,#54346,#54347,
#54348,#54349,#54350,#54351,#54352,#54353,#54354,#54355,#54356,#54357,#54358,
#54359,#54360,#54361,#54362,#54363,#54364,#54365,#54366,#54367,#54368,#54369,
#54370,#54371,#54372,#54373,#54374,#54375,#54376,#54377,#54378,#54379,#54380,
#54381,#54382,#54383,#54384,#54385,#54386,#54387,#54388,#54389,#54390,#54391,
#54392,#54393,#54394,#54395,#54396,#54397,#54398,#54399,#54400,#54401,#54402,
#54403,#54404,#54405,#54406,#54407,#54408,#54409,#54410,#54411,#54412,#54413,
#54414,#54415,#54416,#54417,#54418,#54419,#54420,#54421,#54422,#54423,#54424,
#54425,#54426,#54427),.UNSPECIFIED.,.F.,.F.,(4,3,3,3,3,3,3,3,3,3,3,3,3,
3,3,3,3,3,3,3,3,3,3,3,3,3,3,3,4),(16.1480982907358,16.2248435932826,16.3131664751049,
16.4010510064408,16.4871457020177,16.6179036047363,16.6781446318289,16.8189376696365,
16.955144254623,17.0336892409042,17.0716499935151,17.0956876497882,17.1122342271853,
17.1875859385791,17.2753698848045,17.3642719148437,17.402362983002,17.4328164230854,
17.5413519673841,17.6932989709641,17.7543954310227,17.8465699788546,17.9023081464328,
17.9153013030841,18.0357572506602,18.1619936402749,18.2808910196376,18.3561955540817,
18.3977432388145),.UNSPECIFIED.);
#7637=B_SPLINE_CURVE_WITH_KNOTS('',3,(#54429,#54430,#54431,#54432,#54433,
#54434,#54435,#54436,#54437,#54438,#54439,#54440,#54441,#54442,#54443,#54444,
#54445,#54446,#54447,#54448,#54449,#54450,#54451,#54452,#54453,#54454,#54455,
#54456,#54457,#54458,#54459,#54460,#54461,#54462,#54463,#54464,#54465,#54466,
#54467,#54468,#54469,#54470,#54471,#54472,#54473,#54474,#54475,#54476,#54477,
#54478,#54479,#54480,#54481,#54482,#54483,#54484,#54485,#54486,#54487,#54488,
#54489,#54490,#54491,#54492,#54493,#54494,#54495,#54496,#54497,#54498,#54499,
#54500,#54501,#54502,#54503,#54504,#54505,#54506,#54507,#54508,#54509,#54510,
#54511,#54512,#54513,#54514,#54515,#54516,#54517,#54518,#54519,#54520,#54521,
#54522,#54523,#54524,#54525,#54526,#54527,#54528,#54529,#54530,#54531,#54532,
#54533,#54534),.UNSPECIFIED.,.F.,.F.,(4,3,3,3,3,3,3,3,3,3,3,3,3,3,3,3,3,
3,3,3,3,3,3,3,3,3,3,3,3,3,3,3,3,3,3,4),(13.8978862047801,13.8984130587941,
13.9451297113282,13.9886893494331,14.0168480477334,14.0848270634095,14.131175493238,
14.2193450517567,14.3102533857122,14.3465462347775,14.4385871510249,14.5269329935135,
14.6138701631047,14.6996609714898,14.7622448570774,14.8183725724115,14.862262798083,
14.9426275163738,15.0148788949253,15.0849903110361,15.1538012013756,15.1837216712462,
15.2582774812726,15.3362859342931,15.420896880999,15.5051805444094,15.5789709859087,
15.6375672112739,15.7048255919162,15.7713399419104,15.8266394175726,15.9080154600573,
15.9937473972911,16.0847574555634,16.1427982324843,16.1480982907358),
 .UNSPECIFIED.);
#7638=B_SPLINE_CURVE_WITH_KNOTS('',3,(#54536,#54537,#54538,#54539,#54540,
#54541,#54542,#54543,#54544,#54545,#54546,#54547,#54548,#54549,#54550,#54551,
#54552,#54553,#54554,#54555,#54556,#54557,#54558,#54559,#54560,#54561,#54562,
#54563,#54564,#54565,#54566,#54567,#54568,#54569,#54570,#54571,#54572,#54573,
#54574,#54575,#54576,#54577,#54578,#54579,#54580,#54581,#54582,#54583,#54584),
 .UNSPECIFIED.,.F.,.F.,(4,3,3,3,3,3,3,3,3,3,3,3,3,3,3,3,4),(12.3501209228208,
12.3501377830757,12.4774048190594,12.5359956487871,12.6983861874045,12.7208084228289,
12.8726544490315,12.9290663407961,13.0134488895805,13.0860855995525,13.231115647179,
13.3679133715857,13.455667534087,13.4592103546039,13.6071368603549,13.7603835918095,
13.8978861785935),.UNSPECIFIED.);
#7639=B_SPLINE_CURVE_WITH_KNOTS('',3,(#54586,#54587,#54588,#54589,#54590,
#54591,#54592,#54593,#54594),.UNSPECIFIED.,.F.,.F.,(4,1,1,1,1,1,4),(10.8793710892452,
11.0894782083274,11.2995853274097,11.5096924464919,11.7197995655741,11.9299066846563,
12.3501209228208),.UNSPECIFIED.);
#7640=B_SPLINE_CURVE_WITH_KNOTS('',3,(#54596,#54597,#54598,#54599,#54600,
#54601,#54602,#54603,#54604,#54605,#54606,#54607,#54608,#54609,#54610,#54611,
#54612,#54613,#54614,#54615,#54616,#54617,#54618,#54619,#54620,#54621,#54622,
#54623,#54624,#54625,#54626,#54627,#54628,#54629,#54630,#54631,#54632,#54633,
#54634,#54635,#54636,#54637,#54638,#54639,#54640,#54641,#54642,#54643,#54644,
#54645,#54646,#54647,#54648,#54649,#54650,#54651,#54652,#54653,#54654,#54655,
#54656,#54657,#54658,#54659,#54660,#54661,#54662,#54663,#54664,#54665,#54666,
#54667,#54668),.UNSPECIFIED.,.F.,.F.,(4,3,3,3,3,3,3,3,3,3,3,3,3,3,3,3,3,
3,3,3,3,3,3,3,4),(7.92790045161141,7.92790443383917,8.08238192001809,8.21014604617211,
8.3584935347356,8.50965281881294,8.66649295639789,8.68369720698906,8.77117777664964,
8.93535063493343,9.07053253199945,9.19281643916875,9.2095400889765,9.34694768700197,
9.5026441951939,9.61445510168786,9.81054146163073,9.89179677630612,10.0351653028737,
10.036093764207,10.2469130954665,10.4577324267261,10.6253794515734,10.7842352433031,
10.8793710891041),.UNSPECIFIED.);
#7641=B_SPLINE_CURVE_WITH_KNOTS('',3,(#54670,#54671,#54672,#54673,#54674,
#54675),.UNSPECIFIED.,.F.,.F.,(4,2,4),(0.,0.241870352729709,0.496358334674456),
 .UNSPECIFIED.);
#7642=B_SPLINE_CURVE_WITH_KNOTS('',3,(#54677,#54678,#54679,#54680,#54681,
#54682,#54683,#54684,#54685,#54686,#54687,#54688,#54689,#54690,#54691,#54692,
#54693,#54694,#54695,#54696,#54697,#54698,#54699,#54700,#54701,#54702,#54703,
#54704,#54705,#54706,#54707,#54708,#54709,#54710,#54711,#54712,#54713,#54714,
#54715,#54716,#54717,#54718,#54719,#54720,#54721,#54722,#54723,#54724,#54725,
#54726,#54727,#54728,#54729,#54730,#54731,#54732,#54733,#54734,#54735,#54736,
#54737,#54738,#54739,#54740,#54741,#54742,#54743,#54744,#54745,#54746,#54747,
#54748,#54749,#54750,#54751,#54752,#54753,#54754,#54755),.UNSPECIFIED.,
 .F.,.F.,(4,3,3,3,3,3,3,3,3,3,3,3,3,3,3,3,3,3,3,3,3,3,3,3,3,3,4),(4.48918216137468,
4.57836268956684,4.66429138725693,4.70204447593824,4.75184600019805,4.83940061313917,
4.92497557084337,5.00655520602809,5.10614528180705,5.20279005119437,5.30456419127571,
5.44718714106359,5.5287983194506,5.53983751666817,5.74220502779296,5.79984794218939,
5.89005596843266,5.98727783913441,6.06516519431491,6.21635416528659,6.24027442019716,
6.44087192221132,6.52618822266893,6.59049287196166,6.84221467108407,6.94070913857473,
6.94071132372615),.UNSPECIFIED.);
#7643=B_SPLINE_CURVE_WITH_KNOTS('',3,(#54757,#54758,#54759,#54760),
 .UNSPECIFIED.,.F.,.F.,(4,4),(3.57654770812807,4.48918216137468),
 .UNSPECIFIED.);
#7644=B_SPLINE_CURVE_WITH_KNOTS('',3,(#54762,#54763,#54764,#54765,#54766,
#54767,#54768,#54769,#54770,#54771,#54772,#54773,#54774,#54775,#54776,#54777,
#54778,#54779,#54780,#54781,#54782,#54783,#54784,#54785,#54786,#54787,#54788,
#54789,#54790,#54791,#54792,#54793,#54794,#54795,#54796,#54797,#54798,#54799,
#54800,#54801),.UNSPECIFIED.,.F.,.F.,(4,3,3,3,3,3,3,3,3,3,3,3,3,4),(2.87518401914012,
3.02563515937007,3.11017562117646,3.17608629960003,3.18735576179043,3.2379900880792,
3.30733349478453,3.35480663273688,3.37667690148986,3.39282841371691,3.43385902271625,
3.47939932986374,3.53071044652234,3.57654770812807),.UNSPECIFIED.);
#7645=B_SPLINE_CURVE_WITH_KNOTS('',3,(#54803,#54804,#54805,#54806,#54807,
#54808,#54809,#54810,#54811,#54812,#54813,#54814,#54815,#54816,#54817,#54818,
#54819,#54820,#54821,#54822,#54823,#54824,#54825,#54826,#54827,#54828,#54829,
#54830,#54831,#54832,#54833,#54834,#54835,#54836,#54837,#54838,#54839,#54840,
#54841,#54842,#54843,#54844,#54845,#54846,#54847,#54848,#54849,#54850,#54851,
#54852,#54853,#54854,#54855,#54856,#54857,#54858,#54859,#54860,#54861,#54862,
#54863,#54864,#54865,#54866,#54867,#54868,#54869,#54870,#54871,#54872,#54873,
#54874,#54875,#54876,#54877,#54878,#54879,#54880,#54881),.UNSPECIFIED.,
 .F.,.F.,(4,3,3,3,3,3,3,3,3,3,3,3,3,3,3,3,3,3,3,3,3,3,3,3,3,3,4),(2.26956600808026,
2.30568082207415,2.31814480426122,2.35518314641223,2.39329029907104,2.43342479089149,
2.44265392439187,2.46304008322477,2.5008316930767,2.50395325324957,2.52910268948728,
2.55062012891362,2.55910730470815,2.57081062046563,2.60742859742941,2.61583165898047,
2.62631661195726,2.63142841550033,2.65685256816584,2.68832611522751,2.70246454006634,
2.70904066964155,2.74494826348243,2.77791213560758,2.82654807737385,2.85614989666385,
2.87518401914012),.UNSPECIFIED.);
#7646=B_SPLINE_CURVE_WITH_KNOTS('',3,(#54882,#54883,#54884,#54885,#54886,
#54887,#54888,#54889,#54890,#54891,#54892,#54893,#54894,#54895,#54896,#54897,
#54898,#54899,#54900,#54901,#54902,#54903,#54904,#54905,#54906,#54907,#54908,
#54909,#54910,#54911,#54912,#54913,#54914,#54915,#54916,#54917,#54918,#54919,
#54920,#54921,#54922,#54923,#54924,#54925,#54926,#54927,#54928,#54929,#54930,
#54931,#54932,#54933,#54934,#54935,#54936,#54937,#54938,#54939,#54940,#54941,
#54942,#54943,#54944,#54945,#54946,#54947,#54948,#54949,#54950,#54951,#54952,
#54953,#54954,#54955,#54956,#54957,#54958,#54959,#54960,#54961,#54962,#54963,
#54964,#54965,#54966,#54967,#54968,#54969,#54970,#54971,#54972,#54973,#54974,
#54975,#54976,#54977,#54978),.UNSPECIFIED.,.F.,.F.,(4,3,3,3,3,3,3,3,3,3,
3,3,3,3,3,3,3,3,3,3,3,3,3,3,3,3,3,3,3,3,3,3,4),(1.46286899092626,1.46985285769437,
1.5137075307432,1.55730858759994,1.57811142102339,1.61237368561188,1.64995874630276,
1.68914538920166,1.72860789735176,1.74425867666418,1.78111773623103,1.79707974781328,
1.80859628337331,1.84907728093944,1.889870666217,1.92383871454827,1.96141591955071,
1.96555135546924,2.00234636696739,2.03908114572322,2.05196363571095,2.07839684177744,
2.10581001941975,2.12770951388927,2.15432357689818,2.18891560494525,2.1991989789344,
2.22850627287637,2.23444430767235,2.25199383424393,2.26342001656095,2.26950924404891,
2.26956600807314),.UNSPECIFIED.);
#7647=B_SPLINE_CURVE_WITH_KNOTS('',3,(#54983,#54984,#54985,#54986),
 .UNSPECIFIED.,.F.,.F.,(4,4),(8.29205753853133,8.85500373849296),
 .UNSPECIFIED.);
#7648=B_SPLINE_CURVE_WITH_KNOTS('',3,(#54988,#54989,#54990,#54991),
 .UNSPECIFIED.,.F.,.F.,(4,4),(7.63533633256183,8.29189845043642),
 .UNSPECIFIED.);
#7649=B_SPLINE_CURVE_WITH_KNOTS('',3,(#54993,#54994,#54995,#54996,#54997),
 .UNSPECIFIED.,.F.,.F.,(4,1,4),(5.32811515172559,6.48172574214371,7.63514290575142),
 .UNSPECIFIED.);
#7650=B_SPLINE_CURVE_WITH_KNOTS('',3,(#54999,#55000,#55001,#55002,#55003,
#55004,#55005,#55006,#55007,#55008,#55009,#55010,#55011,#55012,#55013,#55014,
#55015,#55016,#55017,#55018,#55019,#55020,#55021,#55022,#55023,#55024,#55025,
#55026,#55027,#55028,#55029,#55030,#55031,#55032,#55033,#55034,#55035,#55036,
#55037,#55038,#55039,#55040,#55041,#55042,#55043,#55044,#55045,#55046,#55047,
#55048,#55049,#55050),.UNSPECIFIED.,.F.,.F.,(4,3,3,3,3,3,3,3,3,3,3,3,3,
3,3,3,3,4),(4.66932841177279,4.73492083097529,4.79747132048363,4.8190732798771,
4.8275011041002,4.8860357191341,4.94431270889177,4.97628795542774,4.97834918285331,
5.03679836578301,5.09530709015466,5.14398063744379,5.2028087815468,5.21750136742543,
5.23326287582971,5.28067425968518,5.32743480017277,5.32765283089508),
 .UNSPECIFIED.);
#7651=B_SPLINE_CURVE_WITH_KNOTS('',3,(#55052,#55053,#55054,#55055),
 .UNSPECIFIED.,.F.,.F.,(4,4),(4.10897615004708,4.66916207727921),
 .UNSPECIFIED.);
#7652=B_SPLINE_CURVE_WITH_KNOTS('',3,(#55057,#55058,#55059,#55060,#55061,
#55062,#55063,#55064,#55065,#55066,#55067,#55068,#55069,#55070,#55071,#55072,
#55073,#55074,#55075,#55076,#55077,#55078,#55079,#55080,#55081,#55082,#55083,
#55084,#55085,#55086,#55087,#55088,#55089,#55090,#55091,#55092,#55093,#55094,
#55095,#55096,#55097,#55098,#55099,#55100,#55101,#55102,#55103,#55104,#55105,
#55106,#55107,#55108,#55109,#55110,#55111,#55112,#55113,#55114,#55115,#55116,
#55117,#55118,#55119,#55120,#55121,#55122,#55123,#55124,#55125,#55126,#55127,
#55128,#55129,#55130,#55131,#55132,#55133,#55134,#55135,#55136,#55137,#55138),
 .UNSPECIFIED.,.F.,.F.,(4,3,3,3,3,3,3,3,3,3,3,3,3,3,3,3,3,3,3,3,3,3,3,3,
3,3,3,4),(3.55050287755944,3.58233413005538,3.61346023613394,3.64477916715078,
3.67699342493071,3.685706834098,3.71988312339799,3.7380145269766,3.77519268224312,
3.81488249921756,3.82215303959738,3.8294256312647,3.86853740020997,3.89174467951658,
3.93186243524685,3.96260357314154,3.96888700811733,4.00385538849654,4.03492331319416,
4.03861769654365,4.05423052961338,4.07222654910159,4.08279331553507,4.09092247278122,
4.09689520868099,4.10262179682547,4.10783906800098,4.10834838496996),
 .UNSPECIFIED.);
#7653=B_SPLINE_CURVE_WITH_KNOTS('',3,(#55140,#55141,#55142,#55143,#55144),
 .UNSPECIFIED.,.F.,.F.,(4,1,4),(2.82488904953941,3.18769596354942,3.5497180136926),
 .UNSPECIFIED.);
#7654=B_SPLINE_CURVE_WITH_KNOTS('',3,(#55146,#55147,#55148,#55149,#55150,
#55151,#55152,#55153,#55154,#55155,#55156),.UNSPECIFIED.,.F.,.F.,(4,1,1,
1,1,1,1,1,4),(1.00983872354131,1.23672001429108,1.46360130504084,1.91736388654036,
2.37112646803988,2.59800775878964,2.71144840416452,2.76816872685197,2.82467737519672),
 .UNSPECIFIED.);
#7655=B_SPLINE_CURVE_WITH_KNOTS('',3,(#55158,#55159,#55160,#55161,#55162,
#55163),.UNSPECIFIED.,.F.,.F.,(4,1,1,4),(0.268956516008204,0.639397619774759,
0.824618171658037,1.00958216337679),.UNSPECIFIED.);
#7656=B_SPLINE_CURVE_WITH_KNOTS('',3,(#55164,#55165,#55166,#55167),
 .UNSPECIFIED.,.F.,.F.,(4,4),(0.,0.268918781548623),.UNSPECIFIED.);
#7657=B_SPLINE_CURVE_WITH_KNOTS('',3,(#55170,#55171,#55172,#55173,#55174),
 .UNSPECIFIED.,.F.,.F.,(4,1,4),(1.03844659662145,1.19032888736264,1.29158374785677),
 .UNSPECIFIED.);
#7658=B_SPLINE_CURVE_WITH_KNOTS('',3,(#55176,#55177,#55178,#55179,#55180,
#55181,#55182,#55183,#55184),.UNSPECIFIED.,.F.,.F.,(4,1,1,1,1,1,4),(0.489962919054084,
0.599485472462595,0.709225753502309,0.818966034542023,0.928706315581737,
0.983576456101594,1.03817397537901),.UNSPECIFIED.);
#7659=B_SPLINE_CURVE_WITH_KNOTS('',3,(#55185,#55186,#55187,#55188,#55189,
#55190,#55191,#55192,#55193),.UNSPECIFIED.,.F.,.F.,(4,1,1,1,1,1,4),(0.,
0.0979490382845762,0.195898076569152,0.293847114853729,0.391796153138305,
0.440770672280593,0.489745191422881),.UNSPECIFIED.);
#7660=B_SPLINE_CURVE_WITH_KNOTS('',3,(#55196,#55197,#55198,#55199),
 .UNSPECIFIED.,.F.,.F.,(4,4),(1.18065640410841,1.2915881661436),
 .UNSPECIFIED.);
#7661=B_SPLINE_CURVE_WITH_KNOTS('',3,(#55201,#55202,#55203,#55204,#55205,
#55206,#55207,#55208,#55209),.UNSPECIFIED.,.F.,.F.,(4,1,1,1,1,1,4),(0.334860544053774,
0.50397957342097,0.673148781092829,0.757733384928759,0.842317988764689,
1.01148719643655,1.18065599249865),.UNSPECIFIED.);
#7662=B_SPLINE_CURVE_WITH_KNOTS('',3,(#55210,#55211,#55212,#55213,#55214,
#55215),.UNSPECIFIED.,.F.,.F.,(4,1,1,4),(0.,0.133924146299644,0.234367256024377,
0.334810365749111),.UNSPECIFIED.);
#7663=B_SPLINE_CURVE_WITH_KNOTS('',3,(#55493,#55494,#55495,#55496,#55497,
#55498),.UNSPECIFIED.,.F.,.F.,(4,1,1,4),(-1.,-0.571428571428571,-0.285714285714286,
0.),.UNSPECIFIED.);
#7664=B_SPLINE_CURVE_WITH_KNOTS('',3,(#55500,#55501,#55502,#55503,#55504,
#55505,#55506,#55507,#55508,#55509,#55510,#55511,#55512,#55513,#55514,#55515,
#55516,#55517,#55518,#55519,#55520,#55521,#55522,#55523,#55524,#55525,#55526,
#55527,#55528,#55529,#55530,#55531,#55532,#55533,#55534,#55535,#55536,#55537,
#55538,#55539,#55540,#55541,#55542,#55543,#55544,#55545,#55546,#55547,#55548,
#55549,#55550,#55551,#55552,#55553,#55554,#55555,#55556,#55557,#55558,#55559,
#55560,#55561,#55562,#55563,#55564,#55565,#55566,#55567,#55568,#55569,#55570,
#55571,#55572,#55573,#55574,#55575,#55576,#55577,#55578,#55579,#55580,#55581,
#55582,#55583,#55584,#55585,#55586,#55587,#55588,#55589,#55590,#55591,#55592,
#55593,#55594,#55595,#55596,#55597,#55598,#55599,#55600,#55601,#55602,#55603,
#55604,#55605,#55606,#55607,#55608,#55609,#55610,#55611,#55612,#55613,#55614,
#55615,#55616,#55617,#55618,#55619,#55620,#55621,#55622,#55623,#55624,#55625,
#55626,#55627,#55628,#55629,#55630,#55631,#55632,#55633,#55634,#55635,#55636,
#55637,#55638,#55639,#55640,#55641,#55642,#55643,#55644,#55645,#55646,#55647,
#55648,#55649,#55650,#55651,#55652,#55653,#55654,#55655,#55656,#55657,#55658,
#55659,#55660,#55661,#55662,#55663,#55664,#55665,#55666,#55667,#55668,#55669,
#55670,#55671,#55672,#55673,#55674,#55675,#55676,#55677,#55678,#55679,#55680,
#55681,#55682,#55683,#55684,#55685,#55686,#55687,#55688,#55689,#55690,#55691,
#55692,#55693,#55694,#55695,#55696,#55697,#55698,#55699,#55700,#55701,#55702,
#55703,#55704),.UNSPECIFIED.,.F.,.F.,(4,3,3,3,3,3,3,3,3,3,3,3,3,3,3,3,3,
3,3,3,3,3,3,3,3,3,3,3,3,3,3,3,3,3,3,3,3,3,3,3,3,3,3,3,3,3,3,3,3,3,3,3,3,
3,3,3,3,3,3,3,3,3,3,3,3,3,3,3,4),(-9.19419977830157,-9.10967608036533,-9.02523282363516,
-8.94087429868734,-8.92020082022876,-8.83188380164302,-8.74236525285732,
-8.65258172389636,-8.56298604858251,-8.53897544224619,-8.46560848396481,
-8.38864387903952,-8.31528837316212,-8.2419149911821,-8.16847927352024,
-8.15775006426363,-8.07380735585024,-7.98974952828677,-7.94884017932526,
-7.87139630781852,-7.79379299394296,-7.73993029438688,-7.66519283888366,
-7.59001323218429,-7.5145357766191,-7.43911146275571,-7.36405403236351,
-7.32211052451013,-7.21765558204094,-7.12139380485458,-7.11320063957175,
-7.04908916983143,-6.9851270843274,-6.92121820544923,-6.85730830828777,
-6.79983581216419,-6.73688596392217,-6.695380869695,-6.62424896314964,-6.55311746674484,
-6.48647098475663,-6.43485622044857,-6.38692241757501,-6.33535788303195,
-6.28737385039339,-6.22503102968951,-6.16273885291714,-6.1004508403693,
-6.08827671603015,-5.99093468403265,-5.89334485331293,-5.79536092392622,
-5.73985673089448,-5.70857737642468,-5.69008244730366,-5.63354107741789,
-5.5779611592562,-5.52093906350838,-5.46391696776057,-5.39948019473393,
-5.33491566029492,-5.27038189381646,-5.23775148821748,-5.16837194734185,
-5.09905627112296,-5.08697450185542,-5.0692256166783,-5.01597896114694,
-4.99026184062722),.UNSPECIFIED.);
#7665=B_SPLINE_CURVE_WITH_KNOTS('',3,(#55705,#55706,#55707,#55708,#55709,
#55710,#55711,#55712,#55713,#55714,#55715,#55716,#55717,#55718,#55719,#55720,
#55721,#55722,#55723,#55724,#55725),.UNSPECIFIED.,.F.,.F.,(4,1,1,2,1,2,
1,1,1,2,1,2,2,4),(-4.99026184062445,-4.94498342043847,-4.80299233902153,
-4.51901017618764,-4.27069680674408,-3.85684119100481,-3.05948850905774,
-2.69705547180907,-1.68224296751281,-1.53726975261334,-1.28960453962952,
-0.876829184656479,-0.308773384377632,0.),.UNSPECIFIED.);
#7666=B_SPLINE_CURVE_WITH_KNOTS('',3,(#55730,#55731,#55732,#55733,#55734,
#55735,#55736,#55737,#55738,#55739,#55740,#55741,#55742,#55743,#55744),
 .UNSPECIFIED.,.F.,.F.,(4,2,2,2,1,2,2,4),(-9.1649736818217,-8.85500373849296,
-8.29205753853133,-7.63533633256183,-6.48172574214371,-5.32811515172559,
-4.66932841177279,-4.19968198790815),.UNSPECIFIED.);
#7667=B_SPLINE_CURVE_WITH_KNOTS('',3,(#55745,#55746,#55747,#55748,#55749,
#55750,#55751,#55752,#55753,#55754,#55755,#55756,#55757,#55758,#55759,#55760,
#55761,#55762,#55763,#55764,#55765,#55766,#55767,#55768,#55769,#55770,#55771),
 .UNSPECIFIED.,.F.,.F.,(4,2,1,1,1,2,1,2,1,1,1,1,1,1,1,2,1,1,2,4),(-4.19968198790815,
-4.10834838496996,-4.03861769654365,-3.96888700811733,-3.8294256312647,
-3.55050287755944,-3.18769596354942,-2.82488904953941,-2.76816872685197,
-2.71144840416452,-2.59800775878964,-2.37112646803988,-1.91736388654036,
-1.46360130504084,-1.23672001429108,-1.00983872354131,-0.824618171658037,
-0.639397619774759,-0.268956516008204,0.),.UNSPECIFIED.);
#7668=B_SPLINE_CURVE_WITH_KNOTS('',3,(#55962,#55963,#55964,#55965,#55966),
 .UNSPECIFIED.,.F.,.F.,(4,1,4),(-1.,-0.571428571428571,0.),
 .UNSPECIFIED.);
#7669=B_SPLINE_CURVE_WITH_KNOTS('',3,(#56053,#56054,#56055,#56056,#56057),
 .UNSPECIFIED.,.F.,.F.,(4,1,4),(-0.999999907726918,-0.571428571428571,0.),
 .UNSPECIFIED.);
#7670=B_SPLINE_CURVE_WITH_KNOTS('',3,(#56059,#56060,#56061,#56062,#56063,
#56064,#56065,#56066),.UNSPECIFIED.,.F.,.F.,(4,1,1,2,4),(-1.29174070129165,
-1.21783674573549,-1.07002883462318,-0.922220923510859,-0.822192426456486),
 .UNSPECIFIED.);
#7671=B_SPLINE_CURVE_WITH_KNOTS('',3,(#56067,#56068,#56069,#56070,#56071,
#56072,#56073,#56074,#56075,#56076,#56077,#56078,#56079),.UNSPECIFIED.,
 .F.,.F.,(4,1,1,1,1,1,1,1,2,4),(-0.822192426456486,-0.795342097926536,-0.753049156065094,
-0.668463272342212,-0.583877388619329,-0.414705621173564,-0.330119737450682,
-0.245533853727799,-0.076362086282034,0.),.UNSPECIFIED.);
#7672=B_SPLINE_CURVE_WITH_KNOTS('',3,(#56084,#56085,#56086,#56087,#56088,
#56089,#56090,#56091,#56092,#56093,#56094),.UNSPECIFIED.,.F.,.F.,(4,2,1,
1,1,1,1,4),(-1.2915881661436,-1.18065640410841,-1.01148719643655,-0.842317988764689,
-0.757733384928759,-0.673148781092829,-0.50397957342097,-0.434852353670097),
 .UNSPECIFIED.);
#7673=B_SPLINE_CURVE_WITH_KNOTS('',3,(#56095,#56096,#56097,#56098,#56099,
#56100,#56101,#56102),.UNSPECIFIED.,.F.,.F.,(4,2,1,1,4),(-0.434852353670097,
-0.334810365749111,-0.234367256024377,-0.133924146299644,0.),
 .UNSPECIFIED.);
#7674=B_SPLINE_CURVE_WITH_KNOTS('',3,(#56178,#56179,#56180,#56181,#56182),
 .UNSPECIFIED.,.F.,.F.,(4,1,4),(-1.,-0.571428571428571,0.),
 .UNSPECIFIED.);
#7675=B_SPLINE_CURVE_WITH_KNOTS('',3,(#56299,#56300,#56301,#56302,#56303),
 .UNSPECIFIED.,.F.,.F.,(4,1,4),(-0.999999920592112,-0.571428571428571,0.),
 .UNSPECIFIED.);
#7676=B_SPLINE_CURVE_WITH_KNOTS('',3,(#56305,#56306,#56307,#56308,#56309,
#56310,#56311,#56312),.UNSPECIFIED.,.F.,.F.,(4,1,1,1,1,4),(-1.29193145083568,
-1.18863906797729,-1.0853466851189,-0.982054302260506,-0.878761919402114,
-0.824095347984701),.UNSPECIFIED.);
#7677=B_SPLINE_CURVE_WITH_KNOTS('',3,(#56313,#56314,#56315,#56316,#56317,
#56318,#56319,#56320,#56321,#56322,#56323,#56324,#56325,#56326,#56327,#56328,
#56329,#56330,#56331),.UNSPECIFIED.,.F.,.F.,(4,2,1,1,1,1,1,1,1,1,1,2,1,
1,4),(-0.824095347984701,-0.775469536543723,-0.720593698815789,-0.665717861087855,
-0.555966185631988,-0.44621451017612,-0.336462834720253,-0.309024915856286,
-0.281586996992319,-0.254149078128352,-0.240430118696369,-0.226711159264386,
-0.181368927411508,-0.136026695558631,0.),.UNSPECIFIED.);
#7678=B_SPLINE_CURVE_WITH_KNOTS('',3,(#56336,#56337,#56338,#56339,#56340,
#56341,#56342,#56343,#56344,#56345,#56346,#56347,#56348,#56349),
 .UNSPECIFIED.,.F.,.F.,(4,1,2,1,1,1,1,1,2,4),(-1.29158374785677,-1.19032888736264,
-1.03844659662145,-0.983576456101594,-0.928706315581737,-0.818966034542023,
-0.709225753502309,-0.599485472462595,-0.489745191422881,-0.441202445761129),
 .UNSPECIFIED.);
#7679=B_SPLINE_CURVE_WITH_KNOTS('',3,(#56350,#56351,#56352,#56353,#56354,
#56355,#56356,#56357,#56358,#56359,#56360,#56361,#56362,#56363,#56364,#56365,
#56366,#56367,#56368,#56369,#56370,#56371,#56372,#56373,#56374,#56375,#56376,
#56377,#56378,#56379,#56380,#56381,#56382,#56383,#56384,#56385,#56386,#56387,
#56388,#56389,#56390,#56391,#56392,#56393,#56394,#56395,#56396,#56397,#56398,
#56399,#56400,#56401,#56402,#56403,#56404,#56405,#56406,#56407,#56408,#56409,
#56410,#56411,#56412,#56413,#56414,#56415,#56416,#56417,#56418,#56419),
 .UNSPECIFIED.,.F.,.F.,(4,3,3,3,3,3,3,3,3,3,3,3,3,3,3,3,3,3,3,3,3,3,3,4),
(-0.441202445748346,-0.440770672280593,-0.405187169748375,-0.391796153138305,
-0.370654147970551,-0.34952071493269,-0.328392763829246,-0.307253153744854,
-0.293847114853729,-0.270911242372769,-0.247950260814622,-0.224979378588364,
-0.201991894436606,-0.195898076569152,-0.171410816998008,-0.148142630717063,
-0.124879289690075,-0.101624933779237,-0.0979490382845762,-0.0768368069651967,
-0.055721769904546,-0.0346058366391704,-0.013467980506352,0.),
 .UNSPECIFIED.);
#7680=B_SPLINE_CURVE_WITH_KNOTS('',3,(#56515,#56516,#56517,#56518,#56519),
 .UNSPECIFIED.,.F.,.F.,(4,1,4),(-1.,-0.571428571428571,0.),
 .UNSPECIFIED.);
#7681=B_SPLINE_CURVE_WITH_KNOTS('',3,(#56553,#56554,#56555,#56556,#56557,
#56558,#56559,#56560,#56561,#56562,#56563,#56564,#56565,#56566),
 .UNSPECIFIED.,.F.,.F.,(4,2,2,2,2,2,4),(-0.0984980483372994,-0.0979809036544454,
-0.0915892250220569,-0.0852756446727988,-0.0728984092156269,-0.0491501163779407,
0.),.UNSPECIFIED.);
#7682=B_SPLINE_CURVE_WITH_KNOTS('',3,(#56568,#56569,#56570,#56571,#56572,
#56573,#56574,#56575),.UNSPECIFIED.,.F.,.F.,(4,2,2,4),(-0.0967838852773191,
-0.0481707148393364,0.,0.000510029835108177),.UNSPECIFIED.);
#7683=B_SPLINE_CURVE_WITH_KNOTS('',3,(#56598,#56599,#56600,#56601,#56602,
#56603,#56604,#56605),.UNSPECIFIED.,.F.,.F.,(4,2,2,4),(0.,0.0483258768809437,
0.0962566348254112,0.096764418539181),.UNSPECIFIED.);
#7684=B_SPLINE_CURVE_WITH_KNOTS('',3,(#56676,#56677,#56678,#56679,#56680,
#56681,#56682,#56683,#56684,#56685,#56686,#56687),.UNSPECIFIED.,.F.,.F.,
(4,2,2,2,2,4),(-0.0983831478381398,-0.0490393370760392,-0.0251933545123771,
-0.012733468587,0.,0.000519901458665688),.UNSPECIFIED.);
#8043=VERTEX_POINT('',#28466);
#8044=VERTEX_POINT('',#28467);
#8045=VERTEX_POINT('',#28474);
#8046=VERTEX_POINT('',#28524);
#8047=VERTEX_POINT('',#28531);
#8048=VERTEX_POINT('',#28707);
#8049=VERTEX_POINT('',#28715);
#8050=VERTEX_POINT('',#28723);
#8051=VERTEX_POINT('',#28776);
#8052=VERTEX_POINT('',#28781);
#8053=VERTEX_POINT('',#28788);
#8054=VERTEX_POINT('',#28793);
#8055=VERTEX_POINT('',#28798);
#8056=VERTEX_POINT('',#28808);
#8057=VERTEX_POINT('',#28810);
#8058=VERTEX_POINT('',#38648);
#8059=VERTEX_POINT('',#38649);
#8060=VERTEX_POINT('',#38659);
#8061=VERTEX_POINT('',#38669);
#8062=VERTEX_POINT('',#38764);
#8063=VERTEX_POINT('',#38775);
#8064=VERTEX_POINT('',#38782);
#8065=VERTEX_POINT('',#38795);
#8066=VERTEX_POINT('',#38800);
#8067=VERTEX_POINT('',#38810);
#8068=VERTEX_POINT('',#38819);
#8069=VERTEX_POINT('',#38826);
#8070=VERTEX_POINT('',#38936);
#8071=VERTEX_POINT('',#38945);
#8072=VERTEX_POINT('',#38951);
#8073=VERTEX_POINT('',#39052);
#8074=VERTEX_POINT('',#39062);
#8075=VERTEX_POINT('',#39073);
#8076=VERTEX_POINT('',#39082);
#8077=VERTEX_POINT('',#39092);
#8078=VERTEX_POINT('',#39103);
#8079=VERTEX_POINT('',#39114);
#8080=VERTEX_POINT('',#39121);
#8081=VERTEX_POINT('',#39128);
#8082=VERTEX_POINT('',#39135);
#8083=VERTEX_POINT('',#39142);
#8084=VERTEX_POINT('',#39159);
#8085=VERTEX_POINT('',#39164);
#8086=VERTEX_POINT('',#39185);
#8087=VERTEX_POINT('',#39190);
#8088=VERTEX_POINT('',#39264);
#8089=VERTEX_POINT('',#39272);
#8090=VERTEX_POINT('',#39283);
#8091=VERTEX_POINT('',#39291);
#8092=VERTEX_POINT('',#39371);
#8093=VERTEX_POINT('',#39475);
#8094=VERTEX_POINT('',#39487);
#8095=VERTEX_POINT('',#39582);
#8096=VERTEX_POINT('',#39590);
#8097=VERTEX_POINT('',#39670);
#8098=VERTEX_POINT('',#39723);
#8099=VERTEX_POINT('',#39730);
#8100=VERTEX_POINT('',#39735);
#8101=VERTEX_POINT('',#39788);
#8102=VERTEX_POINT('',#39793);
#8103=VERTEX_POINT('',#39810);
#8104=VERTEX_POINT('',#39816);
#8105=VERTEX_POINT('',#39825);
#8106=VERTEX_POINT('',#39962);
#8107=VERTEX_POINT('',#40036);
#8108=VERTEX_POINT('',#40047);
#8109=VERTEX_POINT('',#40056);
#8110=VERTEX_POINT('',#40065);
#8111=VERTEX_POINT('',#40077);
#8112=VERTEX_POINT('',#40089);
#8113=VERTEX_POINT('',#40100);
#8114=VERTEX_POINT('',#40110);
#8115=VERTEX_POINT('',#40115);
#8116=VERTEX_POINT('',#40126);
#8117=VERTEX_POINT('',#40251);
#8118=VERTEX_POINT('',#40319);
#8119=VERTEX_POINT('',#40334);
#8120=VERTEX_POINT('',#40426);
#8121=VERTEX_POINT('',#40433);
#8122=VERTEX_POINT('',#40443);
#8123=VERTEX_POINT('',#40456);
#8124=VERTEX_POINT('',#40465);
#8125=VERTEX_POINT('',#40542);
#8126=VERTEX_POINT('',#40562);
#8127=VERTEX_POINT('',#40563);
#8128=VERTEX_POINT('',#40568);
#8129=VERTEX_POINT('',#40574);
#8130=VERTEX_POINT('',#40585);
#8131=VERTEX_POINT('',#40594);
#8132=VERTEX_POINT('',#40601);
#8133=VERTEX_POINT('',#40690);
#8134=VERTEX_POINT('',#40728);
#8135=VERTEX_POINT('',#40829);
#8136=VERTEX_POINT('',#40835);
#8137=VERTEX_POINT('',#40841);
#8138=VERTEX_POINT('',#40842);
#8139=VERTEX_POINT('',#40851);
#8140=VERTEX_POINT('',#40977);
#8141=VERTEX_POINT('',#40978);
#8142=VERTEX_POINT('',#40983);
#8143=VERTEX_POINT('',#41015);
#8144=VERTEX_POINT('',#41020);
#8145=VERTEX_POINT('',#41025);
#8146=VERTEX_POINT('',#41041);
#8147=VERTEX_POINT('',#41048);
#8148=VERTEX_POINT('',#41054);
#8149=VERTEX_POINT('',#41059);
#8150=VERTEX_POINT('',#41072);
#8151=VERTEX_POINT('',#41073);
#8152=VERTEX_POINT('',#41132);
#8153=VERTEX_POINT('',#41362);
#8154=VERTEX_POINT('',#41368);
#8155=VERTEX_POINT('',#41375);
#8156=VERTEX_POINT('',#41381);
#8157=VERTEX_POINT('',#41386);
#8158=VERTEX_POINT('',#41391);
#8159=VERTEX_POINT('',#41396);
#8160=VERTEX_POINT('',#41402);
#8161=VERTEX_POINT('',#41455);
#8162=VERTEX_POINT('',#41517);
#8163=VERTEX_POINT('',#41525);
#8164=VERTEX_POINT('',#52341);
#8165=VERTEX_POINT('',#52342);
#8166=VERTEX_POINT('',#52352);
#8167=VERTEX_POINT('',#52364);
#8168=VERTEX_POINT('',#52450);
#8169=VERTEX_POINT('',#52530);
#8170=VERTEX_POINT('',#52539);
#8171=VERTEX_POINT('',#52544);
#8172=VERTEX_POINT('',#52609);
#8173=VERTEX_POINT('',#52618);
#8174=VERTEX_POINT('',#52704);
#8175=VERTEX_POINT('',#52712);
#8176=VERTEX_POINT('',#52783);
#8177=VERTEX_POINT('',#52908);
#8178=VERTEX_POINT('',#52991);
#8179=VERTEX_POINT('',#52998);
#8180=VERTEX_POINT('',#53008);
#8181=VERTEX_POINT('',#53019);
#8182=VERTEX_POINT('',#53031);
#8183=VERTEX_POINT('',#53126);
#8184=VERTEX_POINT('',#53191);
#8185=VERTEX_POINT('',#53200);
#8186=VERTEX_POINT('',#53298);
#8187=VERTEX_POINT('',#53306);
#8188=VERTEX_POINT('',#53440);
#8189=VERTEX_POINT('',#53538);
#8190=VERTEX_POINT('',#53544);
#8191=VERTEX_POINT('',#53549);
#8192=VERTEX_POINT('',#53556);
#8193=VERTEX_POINT('',#53575);
#8194=VERTEX_POINT('',#53582);
#8195=VERTEX_POINT('',#53595);
#8196=VERTEX_POINT('',#53645);
#8197=VERTEX_POINT('',#53651);
#8198=VERTEX_POINT('',#53670);
#8199=VERTEX_POINT('',#53768);
#8200=VERTEX_POINT('',#53866);
#8201=VERTEX_POINT('',#53880);
#8202=VERTEX_POINT('',#53890);
#8203=VERTEX_POINT('',#53898);
#8204=VERTEX_POINT('',#53999);
#8205=VERTEX_POINT('',#54007);
#8206=VERTEX_POINT('',#54063);
#8207=VERTEX_POINT('',#54068);
#8208=VERTEX_POINT('',#54095);
#8209=VERTEX_POINT('',#54100);
#8210=VERTEX_POINT('',#54107);
#8211=VERTEX_POINT('',#54124);
#8212=VERTEX_POINT('',#54131);
#8213=VERTEX_POINT('',#54138);
#8214=VERTEX_POINT('',#54212);
#8215=VERTEX_POINT('',#54220);
#8216=VERTEX_POINT('',#54285);
#8217=VERTEX_POINT('',#54295);
#8218=VERTEX_POINT('',#54304);
#8219=VERTEX_POINT('',#54315);
#8220=VERTEX_POINT('',#54325);
#8221=VERTEX_POINT('',#54333);
#8222=VERTEX_POINT('',#54342);
#8223=VERTEX_POINT('',#54428);
#8224=VERTEX_POINT('',#54535);
#8225=VERTEX_POINT('',#54585);
#8226=VERTEX_POINT('',#54595);
#8227=VERTEX_POINT('',#54669);
#8228=VERTEX_POINT('',#54676);
#8229=VERTEX_POINT('',#54756);
#8230=VERTEX_POINT('',#54761);
#8231=VERTEX_POINT('',#54802);
#8232=VERTEX_POINT('',#54979);
#8233=VERTEX_POINT('',#54980);
#8234=VERTEX_POINT('',#54982);
#8235=VERTEX_POINT('',#54987);
#8236=VERTEX_POINT('',#54992);
#8237=VERTEX_POINT('',#54998);
#8238=VERTEX_POINT('',#55051);
#8239=VERTEX_POINT('',#55056);
#8240=VERTEX_POINT('',#55139);
#8241=VERTEX_POINT('',#55145);
#8242=VERTEX_POINT('',#55157);
#8243=VERTEX_POINT('',#55168);
#8244=VERTEX_POINT('',#55169);
#8245=VERTEX_POINT('',#55175);
#8246=VERTEX_POINT('',#55194);
#8247=VERTEX_POINT('',#55195);
#8248=VERTEX_POINT('',#55200);
#8249=VERTEX_POINT('',#55492);
#8250=VERTEX_POINT('',#55499);
#8251=VERTEX_POINT('',#55727);
#8252=VERTEX_POINT('',#55729);
#8253=VERTEX_POINT('',#56052);
#8254=VERTEX_POINT('',#56058);
#8255=VERTEX_POINT('',#56081);
#8256=VERTEX_POINT('',#56083);
#8257=VERTEX_POINT('',#56298);
#8258=VERTEX_POINT('',#56304);
#8259=VERTEX_POINT('',#56333);
#8260=VERTEX_POINT('',#56335);
#8261=VERTEX_POINT('',#56552);
#8262=VERTEX_POINT('',#56567);
#8263=VERTEX_POINT('',#56597);
#8264=VERTEX_POINT('',#56675);
#8265=VERTEX_POINT('',#56802);
#8266=VERTEX_POINT('',#56829);
#8267=VERTEX_POINT('',#56996);
#8268=VERTEX_POINT('',#57039);
#8269=VERTEX_POINT('',#57078);
#8270=VERTEX_POINT('',#57167);
#8271=VERTEX_POINT('',#57449);
#8272=VERTEX_POINT('',#57534);
#8273=VERTEX_POINT('',#57577);
#8274=VERTEX_POINT('',#57624);
#8275=VERTEX_POINT('',#57799);
#8276=VERTEX_POINT('',#57838);
#8277=VERTEX_POINT('',#57961);
#8278=VERTEX_POINT('',#58645);
#9924=EDGE_CURVE('',#8043,#8044,#7457,.T.);
#9925=EDGE_CURVE('',#8044,#8045,#7458,.T.);
#9926=EDGE_CURVE('',#8045,#8044,#7459,.T.);
#9927=EDGE_CURVE('',#8043,#8046,#7460,.T.);
#9928=EDGE_CURVE('',#8046,#8047,#7461,.T.);
#9929=EDGE_CURVE('',#8047,#8048,#7462,.T.);
#9930=EDGE_CURVE('',#8048,#8049,#7463,.T.);
#9931=EDGE_CURVE('',#8049,#8050,#7464,.T.);
#9932=EDGE_CURVE('',#8050,#8051,#7465,.T.);
#9933=EDGE_CURVE('',#8051,#8052,#7466,.T.);
#9934=EDGE_CURVE('',#8052,#8053,#7467,.T.);
#9935=EDGE_CURVE('',#8053,#8054,#7468,.T.);
#9936=EDGE_CURVE('',#8054,#8055,#7469,.T.);
#9937=EDGE_CURVE('',#8055,#8043,#7470,.T.);
#9938=EDGE_CURVE('',#8045,#8056,#1980,.T.);
#9939=EDGE_CURVE('',#8057,#8056,#7471,.T.);
#9940=EDGE_CURVE('',#8056,#8057,#7472,.T.);
#9941=EDGE_CURVE('',#8058,#8059,#7473,.T.);
#9942=EDGE_CURVE('',#8059,#8060,#7474,.T.);
#9943=EDGE_CURVE('',#8060,#8061,#7475,.T.);
#9944=EDGE_CURVE('',#8061,#8062,#7476,.T.);
#9945=EDGE_CURVE('',#8062,#8063,#7477,.T.);
#9946=EDGE_CURVE('',#8063,#8064,#7478,.T.);
#9947=EDGE_CURVE('',#8064,#8065,#7479,.T.);
#9948=EDGE_CURVE('',#8065,#8066,#7480,.T.);
#9949=EDGE_CURVE('',#8066,#8067,#7481,.T.);
#9950=EDGE_CURVE('',#8067,#8068,#7482,.T.);
#9951=EDGE_CURVE('',#8068,#8069,#7483,.T.);
#9952=EDGE_CURVE('',#8069,#8070,#7484,.T.);
#9953=EDGE_CURVE('',#8070,#8071,#7485,.T.);
#9954=EDGE_CURVE('',#8071,#8072,#7486,.T.);
#9955=EDGE_CURVE('',#8072,#8073,#7487,.T.);
#9956=EDGE_CURVE('',#8073,#8074,#7488,.T.);
#9957=EDGE_CURVE('',#8074,#8075,#7489,.T.);
#9958=EDGE_CURVE('',#8075,#8076,#7490,.T.);
#9959=EDGE_CURVE('',#8076,#8077,#7491,.T.);
#9960=EDGE_CURVE('',#8077,#8078,#7492,.T.);
#9961=EDGE_CURVE('',#8078,#8079,#7493,.T.);
#9962=EDGE_CURVE('',#8079,#8080,#7494,.T.);
#9963=EDGE_CURVE('',#8080,#8081,#7495,.T.);
#9964=EDGE_CURVE('',#8081,#8082,#7496,.T.);
#9965=EDGE_CURVE('',#8082,#8083,#7497,.T.);
#9966=EDGE_CURVE('',#8083,#8084,#7498,.T.);
#9967=EDGE_CURVE('',#8084,#8085,#7499,.T.);
#9968=EDGE_CURVE('',#8085,#8086,#7500,.T.);
#9969=EDGE_CURVE('',#8086,#8087,#7501,.T.);
#9970=EDGE_CURVE('',#8087,#8088,#7502,.T.);
#9971=EDGE_CURVE('',#8088,#8089,#7503,.T.);
#9972=EDGE_CURVE('',#8089,#8090,#7504,.T.);
#9973=EDGE_CURVE('',#8090,#8091,#7505,.T.);
#9974=EDGE_CURVE('',#8091,#8092,#7506,.T.);
#9975=EDGE_CURVE('',#8092,#8093,#7507,.T.);
#9976=EDGE_CURVE('',#8093,#8094,#7508,.T.);
#9977=EDGE_CURVE('',#8094,#8095,#7509,.T.);
#9978=EDGE_CURVE('',#8095,#8096,#7510,.T.);
#9979=EDGE_CURVE('',#8096,#8097,#7511,.T.);
#9980=EDGE_CURVE('',#8097,#8098,#7512,.T.);
#9981=EDGE_CURVE('',#8098,#8099,#7513,.T.);
#9982=EDGE_CURVE('',#8099,#8100,#7514,.T.);
#9983=EDGE_CURVE('',#8100,#8101,#7515,.T.);
#9984=EDGE_CURVE('',#8101,#8102,#7516,.T.);
#9985=EDGE_CURVE('',#8102,#8103,#7517,.T.);
#9986=EDGE_CURVE('',#8103,#8104,#7518,.T.);
#9987=EDGE_CURVE('',#8104,#8105,#7519,.T.);
#9988=EDGE_CURVE('',#8105,#8106,#7520,.T.);
#9989=EDGE_CURVE('',#8106,#8107,#7521,.T.);
#9990=EDGE_CURVE('',#8107,#8108,#7522,.T.);
#9991=EDGE_CURVE('',#8108,#8109,#7523,.T.);
#9992=EDGE_CURVE('',#8109,#8110,#7524,.T.);
#9993=EDGE_CURVE('',#8110,#8111,#7525,.T.);
#9994=EDGE_CURVE('',#8111,#8112,#7526,.T.);
#9995=EDGE_CURVE('',#8112,#8113,#7527,.T.);
#9996=EDGE_CURVE('',#8113,#8114,#7528,.T.);
#9997=EDGE_CURVE('',#8114,#8115,#7529,.T.);
#9998=EDGE_CURVE('',#8115,#8116,#7530,.T.);
#9999=EDGE_CURVE('',#8116,#8117,#7531,.T.);
#10000=EDGE_CURVE('',#8117,#8118,#7532,.T.);
#10001=EDGE_CURVE('',#8118,#8119,#7533,.T.);
#10002=EDGE_CURVE('',#8119,#8120,#7534,.T.);
#10003=EDGE_CURVE('',#8120,#8121,#7535,.T.);
#10004=EDGE_CURVE('',#8121,#8122,#7536,.T.);
#10005=EDGE_CURVE('',#8122,#8123,#7537,.T.);
#10006=EDGE_CURVE('',#8123,#8124,#7538,.T.);
#10007=EDGE_CURVE('',#8124,#8125,#7539,.T.);
#10008=EDGE_CURVE('',#8125,#8058,#7540,.T.);
#10009=EDGE_CURVE('',#8126,#8127,#7541,.T.);
#10010=EDGE_CURVE('',#8128,#8126,#7542,.T.);
#10011=EDGE_CURVE('',#8129,#8128,#7543,.T.);
#10012=EDGE_CURVE('',#8130,#8129,#7544,.T.);
#10013=EDGE_CURVE('',#8131,#8130,#7545,.T.);
#10014=EDGE_CURVE('',#8132,#8131,#7546,.T.);
#10015=EDGE_CURVE('',#8133,#8132,#7547,.T.);
#10016=EDGE_CURVE('',#8134,#8133,#7548,.T.);
#10017=EDGE_CURVE('',#8135,#8134,#7549,.T.);
#10018=EDGE_CURVE('',#8136,#8135,#7550,.T.);
#10019=EDGE_CURVE('',#8127,#8136,#1811,.T.);
#10020=EDGE_CURVE('',#8137,#8138,#7551,.T.);
#10021=EDGE_CURVE('',#8139,#8137,#7552,.T.);
#10022=EDGE_CURVE('',#8138,#8139,#7553,.T.);
#10023=EDGE_CURVE('',#8140,#8141,#7554,.T.);
#10024=EDGE_CURVE('',#8142,#8141,#7555,.T.);
#10025=EDGE_CURVE('',#8142,#8143,#7556,.T.);
#10026=EDGE_CURVE('',#8143,#8144,#7557,.T.);
#10027=EDGE_CURVE('',#8145,#8144,#7558,.T.);
#10028=EDGE_CURVE('',#8145,#8146,#7559,.T.);
#10029=EDGE_CURVE('',#8147,#8146,#7560,.T.);
#10030=EDGE_CURVE('',#8147,#8148,#7561,.T.);
#10031=EDGE_CURVE('',#8149,#8148,#7562,.T.);
#10032=EDGE_CURVE('',#8149,#8140,#7563,.T.);
#10033=EDGE_CURVE('',#8150,#8151,#7564,.T.);
#10034=EDGE_CURVE('',#8152,#8150,#7565,.T.);
#10035=EDGE_CURVE('',#8151,#8152,#7566,.T.);
#10036=EDGE_CURVE('',#8153,#8057,#7567,.T.);
#10037=EDGE_CURVE('',#8153,#8154,#7568,.T.);
#10038=EDGE_CURVE('',#8154,#8155,#7569,.T.);
#10039=EDGE_CURVE('',#8155,#8156,#7570,.T.);
#10040=EDGE_CURVE('',#8156,#8157,#7571,.T.);
#10041=EDGE_CURVE('',#8157,#8158,#7572,.T.);
#10042=EDGE_CURVE('',#8158,#8159,#7573,.T.);
#10043=EDGE_CURVE('',#8159,#8160,#7574,.T.);
#10044=EDGE_CURVE('',#8160,#8161,#7575,.T.);
#10045=EDGE_CURVE('',#8161,#8162,#7576,.T.);
#10046=EDGE_CURVE('',#8162,#8163,#7577,.T.);
#10047=EDGE_CURVE('',#8163,#8153,#7578,.T.);
#10048=EDGE_CURVE('',#8164,#8165,#7579,.T.);
#10049=EDGE_CURVE('',#8166,#8164,#7580,.T.);
#10050=EDGE_CURVE('',#8167,#8166,#7581,.T.);
#10051=EDGE_CURVE('',#8168,#8167,#7582,.T.);
#10052=EDGE_CURVE('',#8169,#8168,#7583,.T.);
#10053=EDGE_CURVE('',#8170,#8169,#7584,.T.);
#10054=EDGE_CURVE('',#8171,#8170,#7585,.T.);
#10055=EDGE_CURVE('',#8172,#8171,#7586,.T.);
#10056=EDGE_CURVE('',#8173,#8172,#7587,.T.);
#10057=EDGE_CURVE('',#8174,#8173,#7588,.T.);
#10058=EDGE_CURVE('',#8175,#8174,#7589,.T.);
#10059=EDGE_CURVE('',#8176,#8175,#7590,.T.);
#10060=EDGE_CURVE('',#8177,#8176,#7591,.T.);
#10061=EDGE_CURVE('',#8178,#8177,#7592,.T.);
#10062=EDGE_CURVE('',#8179,#8178,#7593,.T.);
#10063=EDGE_CURVE('',#8180,#8179,#7594,.T.);
#10064=EDGE_CURVE('',#8181,#8180,#7595,.T.);
#10065=EDGE_CURVE('',#8182,#8181,#7596,.T.);
#10066=EDGE_CURVE('',#8183,#8182,#7597,.T.);
#10067=EDGE_CURVE('',#8184,#8183,#7598,.T.);
#10068=EDGE_CURVE('',#8185,#8184,#7599,.T.);
#10069=EDGE_CURVE('',#8186,#8185,#7600,.T.);
#10070=EDGE_CURVE('',#8187,#8186,#7601,.T.);
#10071=EDGE_CURVE('',#8188,#8187,#7602,.T.);
#10072=EDGE_CURVE('',#8189,#8188,#7603,.T.);
#10073=EDGE_CURVE('',#8190,#8189,#7604,.T.);
#10074=EDGE_CURVE('',#8191,#8190,#7605,.T.);
#10075=EDGE_CURVE('',#8192,#8191,#7606,.T.);
#10076=EDGE_CURVE('',#8193,#8192,#7607,.T.);
#10077=EDGE_CURVE('',#8194,#8193,#7608,.T.);
#10078=EDGE_CURVE('',#8195,#8194,#7609,.T.);
#10079=EDGE_CURVE('',#8196,#8195,#7610,.T.);
#10080=EDGE_CURVE('',#8197,#8196,#7611,.T.);
#10081=EDGE_CURVE('',#8198,#8197,#7612,.T.);
#10082=EDGE_CURVE('',#8199,#8198,#7613,.T.);
#10083=EDGE_CURVE('',#8200,#8199,#7614,.T.);
#10084=EDGE_CURVE('',#8201,#8200,#7615,.T.);
#10085=EDGE_CURVE('',#8202,#8201,#7616,.T.);
#10086=EDGE_CURVE('',#8203,#8202,#7617,.T.);
#10087=EDGE_CURVE('',#8204,#8203,#7618,.T.);
#10088=EDGE_CURVE('',#8205,#8204,#7619,.T.);
#10089=EDGE_CURVE('',#8206,#8205,#7620,.T.);
#10090=EDGE_CURVE('',#8207,#8206,#7621,.T.);
#10091=EDGE_CURVE('',#8208,#8207,#7622,.T.);
#10092=EDGE_CURVE('',#8209,#8208,#7623,.T.);
#10093=EDGE_CURVE('',#8210,#8209,#7624,.T.);
#10094=EDGE_CURVE('',#8211,#8210,#7625,.T.);
#10095=EDGE_CURVE('',#8212,#8211,#7626,.T.);
#10096=EDGE_CURVE('',#8213,#8212,#7627,.T.);
#10097=EDGE_CURVE('',#8214,#8213,#7628,.T.);
#10098=EDGE_CURVE('',#8215,#8214,#7629,.T.);
#10099=EDGE_CURVE('',#8216,#8215,#7630,.T.);
#10100=EDGE_CURVE('',#8217,#8216,#7631,.T.);
#10101=EDGE_CURVE('',#8218,#8217,#7632,.T.);
#10102=EDGE_CURVE('',#8219,#8218,#7633,.T.);
#10103=EDGE_CURVE('',#8220,#8219,#7634,.T.);
#10104=EDGE_CURVE('',#8221,#8220,#7635,.T.);
#10105=EDGE_CURVE('',#8222,#8221,#7636,.T.);
#10106=EDGE_CURVE('',#8223,#8222,#7637,.T.);
#10107=EDGE_CURVE('',#8224,#8223,#7638,.T.);
#10108=EDGE_CURVE('',#8225,#8224,#7639,.T.);
#10109=EDGE_CURVE('',#8226,#8225,#7640,.T.);
#10110=EDGE_CURVE('',#8227,#8226,#7641,.T.);
#10111=EDGE_CURVE('',#8228,#8227,#7642,.T.);
#10112=EDGE_CURVE('',#8229,#8228,#7643,.T.);
#10113=EDGE_CURVE('',#8230,#8229,#7644,.T.);
#10114=EDGE_CURVE('',#8231,#8230,#7645,.T.);
#10115=EDGE_CURVE('',#8165,#8231,#7646,.T.);
#10116=EDGE_CURVE('',#8232,#8233,#1812,.T.);
#10117=EDGE_CURVE('',#8234,#8232,#7647,.T.);
#10118=EDGE_CURVE('',#8235,#8234,#7648,.T.);
#10119=EDGE_CURVE('',#8236,#8235,#7649,.T.);
#10120=EDGE_CURVE('',#8237,#8236,#7650,.T.);
#10121=EDGE_CURVE('',#8238,#8237,#7651,.T.);
#10122=EDGE_CURVE('',#8239,#8238,#7652,.T.);
#10123=EDGE_CURVE('',#8240,#8239,#7653,.T.);
#10124=EDGE_CURVE('',#8241,#8240,#7654,.T.);
#10125=EDGE_CURVE('',#8242,#8241,#7655,.T.);
#10126=EDGE_CURVE('',#8233,#8242,#7656,.T.);
#10127=EDGE_CURVE('',#8243,#8244,#7657,.T.);
#10128=EDGE_CURVE('',#8245,#8243,#7658,.T.);
#10129=EDGE_CURVE('',#8244,#8245,#7659,.T.);
#10130=EDGE_CURVE('',#8246,#8247,#7660,.T.);
#10131=EDGE_CURVE('',#8248,#8246,#7661,.T.);
#10132=EDGE_CURVE('',#8247,#8248,#7662,.T.);
#10133=EDGE_CURVE('',#8127,#8249,#7663,.T.);
#10134=EDGE_CURVE('',#8249,#8250,#7664,.T.);
#10135=EDGE_CURVE('',#8250,#8249,#7665,.T.);
#10136=EDGE_CURVE('',#8250,#8251,#1981,.T.);
#10137=EDGE_CURVE('',#8252,#8251,#7666,.T.);
#10138=EDGE_CURVE('',#8251,#8252,#7667,.T.);
#10139=EDGE_CURVE('',#8233,#8252,#7668,.T.);
#10140=EDGE_CURVE('',#8151,#8253,#7669,.T.);
#10141=EDGE_CURVE('',#8253,#8254,#7670,.T.);
#10142=EDGE_CURVE('',#8254,#8253,#7671,.T.);
#10143=EDGE_CURVE('',#8254,#8255,#1982,.T.);
#10144=EDGE_CURVE('',#8256,#8255,#7672,.T.);
#10145=EDGE_CURVE('',#8255,#8256,#7673,.T.);
#10146=EDGE_CURVE('',#8247,#8256,#7674,.T.);
#10147=EDGE_CURVE('',#8138,#8257,#7675,.T.);
#10148=EDGE_CURVE('',#8257,#8258,#7676,.T.);
#10149=EDGE_CURVE('',#8258,#8257,#7677,.T.);
#10150=EDGE_CURVE('',#8258,#8259,#1983,.T.);
#10151=EDGE_CURVE('',#8260,#8259,#7678,.T.);
#10152=EDGE_CURVE('',#8259,#8260,#7679,.T.);
#10153=EDGE_CURVE('',#8244,#8260,#7680,.T.);
#10154=EDGE_CURVE('',#8149,#8261,#7681,.T.);
#10155=EDGE_CURVE('',#8148,#8262,#7682,.F.);
#10156=EDGE_CURVE('',#8262,#8261,#1984,.T.);
#10157=EDGE_CURVE('',#8146,#8263,#7683,.F.);
#10158=EDGE_CURVE('',#8263,#8262,#1985,.T.);
#10159=EDGE_CURVE('',#8144,#8264,#7684,.F.);
#10160=EDGE_CURVE('',#8264,#8263,#1986,.T.);
#10161=EDGE_CURVE('',#8261,#8264,#1987,.T.);
#10162=EDGE_CURVE('',#8083,#8208,#1988,.T.);
#10163=EDGE_CURVE('',#8082,#8209,#1989,.T.);
#10164=EDGE_CURVE('',#8081,#8210,#1990,.T.);
#10165=EDGE_CURVE('',#8080,#8265,#1991,.T.);
#10166=EDGE_CURVE('',#8265,#8211,#1992,.T.);
#10167=EDGE_CURVE('',#8079,#8266,#1993,.T.);
#10168=EDGE_CURVE('',#8266,#8212,#1994,.T.);
#10169=EDGE_CURVE('',#8078,#8213,#1995,.T.);
#10170=EDGE_CURVE('',#8077,#8214,#1996,.T.);
#10171=EDGE_CURVE('',#8076,#8215,#1997,.T.);
#10172=EDGE_CURVE('',#8075,#8216,#1998,.T.);
#10173=EDGE_CURVE('',#8074,#8267,#1999,.T.);
#10174=EDGE_CURVE('',#8267,#8217,#2000,.T.);
#10175=EDGE_CURVE('',#8073,#8268,#2001,.T.);
#10176=EDGE_CURVE('',#8268,#8218,#2002,.T.);
#10177=EDGE_CURVE('',#8072,#8269,#2003,.T.);
#10178=EDGE_CURVE('',#8269,#8219,#2004,.T.);
#10179=EDGE_CURVE('',#8071,#8220,#2005,.T.);
#10180=EDGE_CURVE('',#8070,#8221,#2006,.T.);
#10181=EDGE_CURVE('',#8091,#8270,#2007,.T.);
#10182=EDGE_CURVE('',#8090,#8201,#2008,.T.);
#10183=EDGE_CURVE('',#8270,#8200,#2009,.T.);
#10184=EDGE_CURVE('',#8089,#8202,#2010,.T.);
#10185=EDGE_CURVE('',#8088,#8203,#2011,.T.);
#10186=EDGE_CURVE('',#8087,#8204,#2012,.T.);
#10187=EDGE_CURVE('',#8086,#8205,#2013,.T.);
#10188=EDGE_CURVE('',#8085,#8206,#2014,.T.);
#10189=EDGE_CURVE('',#8098,#8193,#2015,.T.);
#10190=EDGE_CURVE('',#8097,#8194,#2016,.T.);
#10191=EDGE_CURVE('',#8096,#8195,#2017,.T.);
#10192=EDGE_CURVE('',#8095,#8196,#2018,.T.);
#10193=EDGE_CURVE('',#8094,#8197,#2019,.T.);
#10194=EDGE_CURVE('',#8093,#8271,#2020,.T.);
#10195=EDGE_CURVE('',#8271,#8198,#2021,.T.);
#10196=EDGE_CURVE('',#8092,#8199,#2022,.T.);
#10197=EDGE_CURVE('',#8113,#8178,#2023,.T.);
#10198=EDGE_CURVE('',#8112,#8272,#2024,.T.);
#10199=EDGE_CURVE('',#8272,#8179,#2025,.T.);
#10200=EDGE_CURVE('',#8111,#8273,#2026,.T.);
#10201=EDGE_CURVE('',#8273,#8180,#2027,.T.);
#10202=EDGE_CURVE('',#8110,#8274,#2028,.T.);
#10203=EDGE_CURVE('',#8274,#8181,#2029,.T.);
#10204=EDGE_CURVE('',#8109,#8182,#2030,.T.);
#10205=EDGE_CURVE('',#8108,#8183,#2031,.T.);
#10206=EDGE_CURVE('',#8107,#8184,#2032,.T.);
#10207=EDGE_CURVE('',#8106,#8185,#2033,.T.);
#10208=EDGE_CURVE('',#8105,#8275,#2034,.T.);
#10209=EDGE_CURVE('',#8275,#8186,#2035,.T.);
#10210=EDGE_CURVE('',#8104,#8276,#2036,.T.);
#10211=EDGE_CURVE('',#8276,#8187,#2037,.T.);
#10212=EDGE_CURVE('',#8103,#8188,#2038,.T.);
#10213=EDGE_CURVE('',#8102,#8189,#2039,.T.);
#10214=EDGE_CURVE('',#8101,#8190,#2040,.T.);
#10215=EDGE_CURVE('',#8100,#8191,#2041,.T.);
#10216=EDGE_CURVE('',#8125,#8277,#2042,.T.);
#10217=EDGE_CURVE('',#8124,#8167,#2043,.T.);
#10218=EDGE_CURVE('',#8277,#8166,#2044,.T.);
#10219=EDGE_CURVE('',#8123,#8168,#2045,.T.);
#10220=EDGE_CURVE('',#8122,#8169,#2046,.T.);
#10221=EDGE_CURVE('',#8121,#8170,#2047,.T.);
#10222=EDGE_CURVE('',#8120,#8171,#2048,.T.);
#10223=EDGE_CURVE('',#8119,#8172,#2049,.T.);
#10224=EDGE_CURVE('',#8118,#8173,#2050,.T.);
#10225=EDGE_CURVE('',#8117,#8174,#2051,.T.);
#10226=EDGE_CURVE('',#8116,#8175,#2052,.T.);
#10227=EDGE_CURVE('',#8115,#8176,#2053,.T.);
#10228=EDGE_CURVE('',#8114,#8177,#2054,.T.);
#10229=EDGE_CURVE('',#8069,#8222,#2055,.T.);
#10230=EDGE_CURVE('',#8068,#8223,#2056,.T.);
#10231=EDGE_CURVE('',#8067,#8224,#2057,.T.);
#10232=EDGE_CURVE('',#8066,#8225,#2058,.T.);
#10233=EDGE_CURVE('',#8065,#8226,#2059,.T.);
#10234=EDGE_CURVE('',#8064,#8227,#2060,.T.);
#10235=EDGE_CURVE('',#8063,#8228,#2061,.T.);
#10236=EDGE_CURVE('',#8062,#8229,#2062,.T.);
#10237=EDGE_CURVE('',#8061,#8230,#2063,.T.);
#10238=EDGE_CURVE('',#8060,#8231,#2064,.T.);
#10239=EDGE_CURVE('',#8059,#8278,#2065,.T.);
#10240=EDGE_CURVE('',#8278,#8165,#2066,.T.);
#10241=EDGE_CURVE('',#8058,#8164,#2067,.T.);
#10242=EDGE_CURVE('',#8099,#8192,#2068,.T.);
#10243=EDGE_CURVE('',#8084,#8207,#2069,.T.);
#12899=ORIENTED_EDGE('',*,*,#9924,.T.);
#12900=ORIENTED_EDGE('',*,*,#9925,.T.);
#12901=ORIENTED_EDGE('',*,*,#9926,.T.);
#12902=ORIENTED_EDGE('',*,*,#9924,.F.);
#12903=ORIENTED_EDGE('',*,*,#9927,.T.);
#12904=ORIENTED_EDGE('',*,*,#9928,.T.);
#12905=ORIENTED_EDGE('',*,*,#9929,.T.);
#12906=ORIENTED_EDGE('',*,*,#9930,.T.);
#12907=ORIENTED_EDGE('',*,*,#9931,.T.);
#12908=ORIENTED_EDGE('',*,*,#9932,.T.);
#12909=ORIENTED_EDGE('',*,*,#9933,.T.);
#12910=ORIENTED_EDGE('',*,*,#9934,.T.);
#12911=ORIENTED_EDGE('',*,*,#9935,.T.);
#12912=ORIENTED_EDGE('',*,*,#9936,.T.);
#12913=ORIENTED_EDGE('',*,*,#9937,.T.);
#12914=ORIENTED_EDGE('',*,*,#9925,.F.);
#12915=ORIENTED_EDGE('',*,*,#9926,.F.);
#12916=ORIENTED_EDGE('',*,*,#9938,.T.);
#12917=ORIENTED_EDGE('',*,*,#9939,.F.);
#12918=ORIENTED_EDGE('',*,*,#9940,.F.);
#12919=ORIENTED_EDGE('',*,*,#9938,.F.);
#12920=ORIENTED_EDGE('',*,*,#9941,.T.);
#12921=ORIENTED_EDGE('',*,*,#9942,.T.);
#12922=ORIENTED_EDGE('',*,*,#9943,.T.);
#12923=ORIENTED_EDGE('',*,*,#9944,.T.);
#12924=ORIENTED_EDGE('',*,*,#9945,.T.);
#12925=ORIENTED_EDGE('',*,*,#9946,.T.);
#12926=ORIENTED_EDGE('',*,*,#9947,.T.);
#12927=ORIENTED_EDGE('',*,*,#9948,.T.);
#12928=ORIENTED_EDGE('',*,*,#9949,.T.);
#12929=ORIENTED_EDGE('',*,*,#9950,.T.);
#12930=ORIENTED_EDGE('',*,*,#9951,.T.);
#12931=ORIENTED_EDGE('',*,*,#9952,.T.);
#12932=ORIENTED_EDGE('',*,*,#9953,.T.);
#12933=ORIENTED_EDGE('',*,*,#9954,.T.);
#12934=ORIENTED_EDGE('',*,*,#9955,.T.);
#12935=ORIENTED_EDGE('',*,*,#9956,.T.);
#12936=ORIENTED_EDGE('',*,*,#9957,.T.);
#12937=ORIENTED_EDGE('',*,*,#9958,.T.);
#12938=ORIENTED_EDGE('',*,*,#9959,.T.);
#12939=ORIENTED_EDGE('',*,*,#9960,.T.);
#12940=ORIENTED_EDGE('',*,*,#9961,.T.);
#12941=ORIENTED_EDGE('',*,*,#9962,.T.);
#12942=ORIENTED_EDGE('',*,*,#9963,.T.);
#12943=ORIENTED_EDGE('',*,*,#9964,.T.);
#12944=ORIENTED_EDGE('',*,*,#9965,.T.);
#12945=ORIENTED_EDGE('',*,*,#9966,.T.);
#12946=ORIENTED_EDGE('',*,*,#9967,.T.);
#12947=ORIENTED_EDGE('',*,*,#9968,.T.);
#12948=ORIENTED_EDGE('',*,*,#9969,.T.);
#12949=ORIENTED_EDGE('',*,*,#9970,.T.);
#12950=ORIENTED_EDGE('',*,*,#9971,.T.);
#12951=ORIENTED_EDGE('',*,*,#9972,.T.);
#12952=ORIENTED_EDGE('',*,*,#9973,.T.);
#12953=ORIENTED_EDGE('',*,*,#9974,.T.);
#12954=ORIENTED_EDGE('',*,*,#9975,.T.);
#12955=ORIENTED_EDGE('',*,*,#9976,.T.);
#12956=ORIENTED_EDGE('',*,*,#9977,.T.);
#12957=ORIENTED_EDGE('',*,*,#9978,.T.);
#12958=ORIENTED_EDGE('',*,*,#9979,.T.);
#12959=ORIENTED_EDGE('',*,*,#9980,.T.);
#12960=ORIENTED_EDGE('',*,*,#9981,.T.);
#12961=ORIENTED_EDGE('',*,*,#9982,.T.);
#12962=ORIENTED_EDGE('',*,*,#9983,.T.);
#12963=ORIENTED_EDGE('',*,*,#9984,.T.);
#12964=ORIENTED_EDGE('',*,*,#9985,.T.);
#12965=ORIENTED_EDGE('',*,*,#9986,.T.);
#12966=ORIENTED_EDGE('',*,*,#9987,.T.);
#12967=ORIENTED_EDGE('',*,*,#9988,.T.);
#12968=ORIENTED_EDGE('',*,*,#9989,.T.);
#12969=ORIENTED_EDGE('',*,*,#9990,.T.);
#12970=ORIENTED_EDGE('',*,*,#9991,.T.);
#12971=ORIENTED_EDGE('',*,*,#9992,.T.);
#12972=ORIENTED_EDGE('',*,*,#9993,.T.);
#12973=ORIENTED_EDGE('',*,*,#9994,.T.);
#12974=ORIENTED_EDGE('',*,*,#9995,.T.);
#12975=ORIENTED_EDGE('',*,*,#9996,.T.);
#12976=ORIENTED_EDGE('',*,*,#9997,.T.);
#12977=ORIENTED_EDGE('',*,*,#9998,.T.);
#12978=ORIENTED_EDGE('',*,*,#9999,.T.);
#12979=ORIENTED_EDGE('',*,*,#10000,.T.);
#12980=ORIENTED_EDGE('',*,*,#10001,.T.);
#12981=ORIENTED_EDGE('',*,*,#10002,.T.);
#12982=ORIENTED_EDGE('',*,*,#10003,.T.);
#12983=ORIENTED_EDGE('',*,*,#10004,.T.);
#12984=ORIENTED_EDGE('',*,*,#10005,.T.);
#12985=ORIENTED_EDGE('',*,*,#10006,.T.);
#12986=ORIENTED_EDGE('',*,*,#10007,.T.);
#12987=ORIENTED_EDGE('',*,*,#10008,.T.);
#12988=ORIENTED_EDGE('',*,*,#10009,.F.);
#12989=ORIENTED_EDGE('',*,*,#10010,.F.);
#12990=ORIENTED_EDGE('',*,*,#10011,.F.);
#12991=ORIENTED_EDGE('',*,*,#10012,.F.);
#12992=ORIENTED_EDGE('',*,*,#10013,.F.);
#12993=ORIENTED_EDGE('',*,*,#10014,.F.);
#12994=ORIENTED_EDGE('',*,*,#10015,.F.);
#12995=ORIENTED_EDGE('',*,*,#10016,.F.);
#12996=ORIENTED_EDGE('',*,*,#10017,.F.);
#12997=ORIENTED_EDGE('',*,*,#10018,.F.);
#12998=ORIENTED_EDGE('',*,*,#10019,.F.);
#12999=ORIENTED_EDGE('',*,*,#10020,.F.);
#13000=ORIENTED_EDGE('',*,*,#10021,.F.);
#13001=ORIENTED_EDGE('',*,*,#10022,.F.);
#13002=ORIENTED_EDGE('',*,*,#10023,.T.);
#13003=ORIENTED_EDGE('',*,*,#10024,.F.);
#13004=ORIENTED_EDGE('',*,*,#10025,.T.);
#13005=ORIENTED_EDGE('',*,*,#10026,.T.);
#13006=ORIENTED_EDGE('',*,*,#10027,.F.);
#13007=ORIENTED_EDGE('',*,*,#10028,.T.);
#13008=ORIENTED_EDGE('',*,*,#10029,.F.);
#13009=ORIENTED_EDGE('',*,*,#10030,.T.);
#13010=ORIENTED_EDGE('',*,*,#10031,.F.);
#13011=ORIENTED_EDGE('',*,*,#10032,.T.);
#13012=ORIENTED_EDGE('',*,*,#10033,.F.);
#13013=ORIENTED_EDGE('',*,*,#10034,.F.);
#13014=ORIENTED_EDGE('',*,*,#10035,.F.);
#13015=ORIENTED_EDGE('',*,*,#9937,.F.);
#13016=ORIENTED_EDGE('',*,*,#9936,.F.);
#13017=ORIENTED_EDGE('',*,*,#9935,.F.);
#13018=ORIENTED_EDGE('',*,*,#9934,.F.);
#13019=ORIENTED_EDGE('',*,*,#9933,.F.);
#13020=ORIENTED_EDGE('',*,*,#9932,.F.);
#13021=ORIENTED_EDGE('',*,*,#9931,.F.);
#13022=ORIENTED_EDGE('',*,*,#9930,.F.);
#13023=ORIENTED_EDGE('',*,*,#9929,.F.);
#13024=ORIENTED_EDGE('',*,*,#9928,.F.);
#13025=ORIENTED_EDGE('',*,*,#9927,.F.);
#13026=ORIENTED_EDGE('',*,*,#10036,.T.);
#13027=ORIENTED_EDGE('',*,*,#9939,.T.);
#13028=ORIENTED_EDGE('',*,*,#9940,.T.);
#13029=ORIENTED_EDGE('',*,*,#10036,.F.);
#13030=ORIENTED_EDGE('',*,*,#10037,.T.);
#13031=ORIENTED_EDGE('',*,*,#10038,.T.);
#13032=ORIENTED_EDGE('',*,*,#10039,.T.);
#13033=ORIENTED_EDGE('',*,*,#10040,.T.);
#13034=ORIENTED_EDGE('',*,*,#10041,.T.);
#13035=ORIENTED_EDGE('',*,*,#10042,.T.);
#13036=ORIENTED_EDGE('',*,*,#10043,.T.);
#13037=ORIENTED_EDGE('',*,*,#10044,.T.);
#13038=ORIENTED_EDGE('',*,*,#10045,.T.);
#13039=ORIENTED_EDGE('',*,*,#10046,.T.);
#13040=ORIENTED_EDGE('',*,*,#10047,.T.);
#13041=ORIENTED_EDGE('',*,*,#10048,.F.);
#13042=ORIENTED_EDGE('',*,*,#10049,.F.);
#13043=ORIENTED_EDGE('',*,*,#10050,.F.);
#13044=ORIENTED_EDGE('',*,*,#10051,.F.);
#13045=ORIENTED_EDGE('',*,*,#10052,.F.);
#13046=ORIENTED_EDGE('',*,*,#10053,.F.);
#13047=ORIENTED_EDGE('',*,*,#10054,.F.);
#13048=ORIENTED_EDGE('',*,*,#10055,.F.);
#13049=ORIENTED_EDGE('',*,*,#10056,.F.);
#13050=ORIENTED_EDGE('',*,*,#10057,.F.);
#13051=ORIENTED_EDGE('',*,*,#10058,.F.);
#13052=ORIENTED_EDGE('',*,*,#10059,.F.);
#13053=ORIENTED_EDGE('',*,*,#10060,.F.);
#13054=ORIENTED_EDGE('',*,*,#10061,.F.);
#13055=ORIENTED_EDGE('',*,*,#10062,.F.);
#13056=ORIENTED_EDGE('',*,*,#10063,.F.);
#13057=ORIENTED_EDGE('',*,*,#10064,.F.);
#13058=ORIENTED_EDGE('',*,*,#10065,.F.);
#13059=ORIENTED_EDGE('',*,*,#10066,.F.);
#13060=ORIENTED_EDGE('',*,*,#10067,.F.);
#13061=ORIENTED_EDGE('',*,*,#10068,.F.);
#13062=ORIENTED_EDGE('',*,*,#10069,.F.);
#13063=ORIENTED_EDGE('',*,*,#10070,.F.);
#13064=ORIENTED_EDGE('',*,*,#10071,.F.);
#13065=ORIENTED_EDGE('',*,*,#10072,.F.);
#13066=ORIENTED_EDGE('',*,*,#10073,.F.);
#13067=ORIENTED_EDGE('',*,*,#10074,.F.);
#13068=ORIENTED_EDGE('',*,*,#10075,.F.);
#13069=ORIENTED_EDGE('',*,*,#10076,.F.);
#13070=ORIENTED_EDGE('',*,*,#10077,.F.);
#13071=ORIENTED_EDGE('',*,*,#10078,.F.);
#13072=ORIENTED_EDGE('',*,*,#10079,.F.);
#13073=ORIENTED_EDGE('',*,*,#10080,.F.);
#13074=ORIENTED_EDGE('',*,*,#10081,.F.);
#13075=ORIENTED_EDGE('',*,*,#10082,.F.);
#13076=ORIENTED_EDGE('',*,*,#10083,.F.);
#13077=ORIENTED_EDGE('',*,*,#10084,.F.);
#13078=ORIENTED_EDGE('',*,*,#10085,.F.);
#13079=ORIENTED_EDGE('',*,*,#10086,.F.);
#13080=ORIENTED_EDGE('',*,*,#10087,.F.);
#13081=ORIENTED_EDGE('',*,*,#10088,.F.);
#13082=ORIENTED_EDGE('',*,*,#10089,.F.);
#13083=ORIENTED_EDGE('',*,*,#10090,.F.);
#13084=ORIENTED_EDGE('',*,*,#10091,.F.);
#13085=ORIENTED_EDGE('',*,*,#10092,.F.);
#13086=ORIENTED_EDGE('',*,*,#10093,.F.);
#13087=ORIENTED_EDGE('',*,*,#10094,.F.);
#13088=ORIENTED_EDGE('',*,*,#10095,.F.);
#13089=ORIENTED_EDGE('',*,*,#10096,.F.);
#13090=ORIENTED_EDGE('',*,*,#10097,.F.);
#13091=ORIENTED_EDGE('',*,*,#10098,.F.);
#13092=ORIENTED_EDGE('',*,*,#10099,.F.);
#13093=ORIENTED_EDGE('',*,*,#10100,.F.);
#13094=ORIENTED_EDGE('',*,*,#10101,.F.);
#13095=ORIENTED_EDGE('',*,*,#10102,.F.);
#13096=ORIENTED_EDGE('',*,*,#10103,.F.);
#13097=ORIENTED_EDGE('',*,*,#10104,.F.);
#13098=ORIENTED_EDGE('',*,*,#10105,.F.);
#13099=ORIENTED_EDGE('',*,*,#10106,.F.);
#13100=ORIENTED_EDGE('',*,*,#10107,.F.);
#13101=ORIENTED_EDGE('',*,*,#10108,.F.);
#13102=ORIENTED_EDGE('',*,*,#10109,.F.);
#13103=ORIENTED_EDGE('',*,*,#10110,.F.);
#13104=ORIENTED_EDGE('',*,*,#10111,.F.);
#13105=ORIENTED_EDGE('',*,*,#10112,.F.);
#13106=ORIENTED_EDGE('',*,*,#10113,.F.);
#13107=ORIENTED_EDGE('',*,*,#10114,.F.);
#13108=ORIENTED_EDGE('',*,*,#10115,.F.);
#13109=ORIENTED_EDGE('',*,*,#10116,.F.);
#13110=ORIENTED_EDGE('',*,*,#10117,.F.);
#13111=ORIENTED_EDGE('',*,*,#10118,.F.);
#13112=ORIENTED_EDGE('',*,*,#10119,.F.);
#13113=ORIENTED_EDGE('',*,*,#10120,.F.);
#13114=ORIENTED_EDGE('',*,*,#10121,.F.);
#13115=ORIENTED_EDGE('',*,*,#10122,.F.);
#13116=ORIENTED_EDGE('',*,*,#10123,.F.);
#13117=ORIENTED_EDGE('',*,*,#10124,.F.);
#13118=ORIENTED_EDGE('',*,*,#10125,.F.);
#13119=ORIENTED_EDGE('',*,*,#10126,.F.);
#13120=ORIENTED_EDGE('',*,*,#10127,.F.);
#13121=ORIENTED_EDGE('',*,*,#10128,.F.);
#13122=ORIENTED_EDGE('',*,*,#10129,.F.);
#13123=ORIENTED_EDGE('',*,*,#10130,.F.);
#13124=ORIENTED_EDGE('',*,*,#10131,.F.);
#13125=ORIENTED_EDGE('',*,*,#10132,.F.);
#13126=ORIENTED_EDGE('',*,*,#10047,.F.);
#13127=ORIENTED_EDGE('',*,*,#10046,.F.);
#13128=ORIENTED_EDGE('',*,*,#10045,.F.);
#13129=ORIENTED_EDGE('',*,*,#10044,.F.);
#13130=ORIENTED_EDGE('',*,*,#10043,.F.);
#13131=ORIENTED_EDGE('',*,*,#10042,.F.);
#13132=ORIENTED_EDGE('',*,*,#10041,.F.);
#13133=ORIENTED_EDGE('',*,*,#10040,.F.);
#13134=ORIENTED_EDGE('',*,*,#10039,.F.);
#13135=ORIENTED_EDGE('',*,*,#10038,.F.);
#13136=ORIENTED_EDGE('',*,*,#10037,.F.);
#13137=ORIENTED_EDGE('',*,*,#10133,.T.);
#13138=ORIENTED_EDGE('',*,*,#10134,.T.);
#13139=ORIENTED_EDGE('',*,*,#10135,.T.);
#13140=ORIENTED_EDGE('',*,*,#10133,.F.);
#13141=ORIENTED_EDGE('',*,*,#10019,.T.);
#13142=ORIENTED_EDGE('',*,*,#10018,.T.);
#13143=ORIENTED_EDGE('',*,*,#10017,.T.);
#13144=ORIENTED_EDGE('',*,*,#10016,.T.);
#13145=ORIENTED_EDGE('',*,*,#10015,.T.);
#13146=ORIENTED_EDGE('',*,*,#10014,.T.);
#13147=ORIENTED_EDGE('',*,*,#10013,.T.);
#13148=ORIENTED_EDGE('',*,*,#10012,.T.);
#13149=ORIENTED_EDGE('',*,*,#10011,.T.);
#13150=ORIENTED_EDGE('',*,*,#10010,.T.);
#13151=ORIENTED_EDGE('',*,*,#10009,.T.);
#13152=ORIENTED_EDGE('',*,*,#10134,.F.);
#13153=ORIENTED_EDGE('',*,*,#10135,.F.);
#13154=ORIENTED_EDGE('',*,*,#10136,.T.);
#13155=ORIENTED_EDGE('',*,*,#10137,.F.);
#13156=ORIENTED_EDGE('',*,*,#10138,.F.);
#13157=ORIENTED_EDGE('',*,*,#10136,.F.);
#13158=ORIENTED_EDGE('',*,*,#10139,.T.);
#13159=ORIENTED_EDGE('',*,*,#10137,.T.);
#13160=ORIENTED_EDGE('',*,*,#10138,.T.);
#13161=ORIENTED_EDGE('',*,*,#10139,.F.);
#13162=ORIENTED_EDGE('',*,*,#10126,.T.);
#13163=ORIENTED_EDGE('',*,*,#10125,.T.);
#13164=ORIENTED_EDGE('',*,*,#10124,.T.);
#13165=ORIENTED_EDGE('',*,*,#10123,.T.);
#13166=ORIENTED_EDGE('',*,*,#10122,.T.);
#13167=ORIENTED_EDGE('',*,*,#10121,.T.);
#13168=ORIENTED_EDGE('',*,*,#10120,.T.);
#13169=ORIENTED_EDGE('',*,*,#10119,.T.);
#13170=ORIENTED_EDGE('',*,*,#10118,.T.);
#13171=ORIENTED_EDGE('',*,*,#10117,.T.);
#13172=ORIENTED_EDGE('',*,*,#10116,.T.);
#13173=ORIENTED_EDGE('',*,*,#10140,.T.);
#13174=ORIENTED_EDGE('',*,*,#10141,.T.);
#13175=ORIENTED_EDGE('',*,*,#10142,.T.);
#13176=ORIENTED_EDGE('',*,*,#10140,.F.);
#13177=ORIENTED_EDGE('',*,*,#10035,.T.);
#13178=ORIENTED_EDGE('',*,*,#10034,.T.);
#13179=ORIENTED_EDGE('',*,*,#10033,.T.);
#13180=ORIENTED_EDGE('',*,*,#10141,.F.);
#13181=ORIENTED_EDGE('',*,*,#10142,.F.);
#13182=ORIENTED_EDGE('',*,*,#10143,.T.);
#13183=ORIENTED_EDGE('',*,*,#10144,.F.);
#13184=ORIENTED_EDGE('',*,*,#10145,.F.);
#13185=ORIENTED_EDGE('',*,*,#10143,.F.);
#13186=ORIENTED_EDGE('',*,*,#10146,.T.);
#13187=ORIENTED_EDGE('',*,*,#10144,.T.);
#13188=ORIENTED_EDGE('',*,*,#10145,.T.);
#13189=ORIENTED_EDGE('',*,*,#10146,.F.);
#13190=ORIENTED_EDGE('',*,*,#10132,.T.);
#13191=ORIENTED_EDGE('',*,*,#10131,.T.);
#13192=ORIENTED_EDGE('',*,*,#10130,.T.);
#13193=ORIENTED_EDGE('',*,*,#10147,.T.);
#13194=ORIENTED_EDGE('',*,*,#10148,.T.);
#13195=ORIENTED_EDGE('',*,*,#10149,.T.);
#13196=ORIENTED_EDGE('',*,*,#10147,.F.);
#13197=ORIENTED_EDGE('',*,*,#10022,.T.);
#13198=ORIENTED_EDGE('',*,*,#10021,.T.);
#13199=ORIENTED_EDGE('',*,*,#10020,.T.);
#13200=ORIENTED_EDGE('',*,*,#10148,.F.);
#13201=ORIENTED_EDGE('',*,*,#10149,.F.);
#13202=ORIENTED_EDGE('',*,*,#10150,.T.);
#13203=ORIENTED_EDGE('',*,*,#10151,.F.);
#13204=ORIENTED_EDGE('',*,*,#10152,.F.);
#13205=ORIENTED_EDGE('',*,*,#10150,.F.);
#13206=ORIENTED_EDGE('',*,*,#10153,.T.);
#13207=ORIENTED_EDGE('',*,*,#10151,.T.);
#13208=ORIENTED_EDGE('',*,*,#10152,.T.);
#13209=ORIENTED_EDGE('',*,*,#10153,.F.);
#13210=ORIENTED_EDGE('',*,*,#10129,.T.);
#13211=ORIENTED_EDGE('',*,*,#10128,.T.);
#13212=ORIENTED_EDGE('',*,*,#10127,.T.);
#13213=ORIENTED_EDGE('',*,*,#10154,.F.);
#13214=ORIENTED_EDGE('',*,*,#10031,.T.);
#13215=ORIENTED_EDGE('',*,*,#10155,.T.);
#13216=ORIENTED_EDGE('',*,*,#10156,.T.);
#13217=ORIENTED_EDGE('',*,*,#10029,.T.);
#13218=ORIENTED_EDGE('',*,*,#10157,.T.);
#13219=ORIENTED_EDGE('',*,*,#10158,.T.);
#13220=ORIENTED_EDGE('',*,*,#10155,.F.);
#13221=ORIENTED_EDGE('',*,*,#10030,.F.);
#13222=ORIENTED_EDGE('',*,*,#10027,.T.);
#13223=ORIENTED_EDGE('',*,*,#10159,.T.);
#13224=ORIENTED_EDGE('',*,*,#10160,.T.);
#13225=ORIENTED_EDGE('',*,*,#10157,.F.);
#13226=ORIENTED_EDGE('',*,*,#10028,.F.);
#13227=ORIENTED_EDGE('',*,*,#10024,.T.);
#13228=ORIENTED_EDGE('',*,*,#10023,.F.);
#13229=ORIENTED_EDGE('',*,*,#10032,.F.);
#13230=ORIENTED_EDGE('',*,*,#10154,.T.);
#13231=ORIENTED_EDGE('',*,*,#10161,.T.);
#13232=ORIENTED_EDGE('',*,*,#10159,.F.);
#13233=ORIENTED_EDGE('',*,*,#10026,.F.);
#13234=ORIENTED_EDGE('',*,*,#10025,.F.);
#13235=ORIENTED_EDGE('',*,*,#10156,.F.);
#13236=ORIENTED_EDGE('',*,*,#10158,.F.);
#13237=ORIENTED_EDGE('',*,*,#10160,.F.);
#13238=ORIENTED_EDGE('',*,*,#10161,.F.);
#13239=ORIENTED_EDGE('',*,*,#10162,.F.);
#13240=ORIENTED_EDGE('',*,*,#9965,.F.);
#13241=ORIENTED_EDGE('',*,*,#10163,.T.);
#13242=ORIENTED_EDGE('',*,*,#10092,.T.);
#13243=ORIENTED_EDGE('',*,*,#10163,.F.);
#13244=ORIENTED_EDGE('',*,*,#9964,.F.);
#13245=ORIENTED_EDGE('',*,*,#10164,.T.);
#13246=ORIENTED_EDGE('',*,*,#10093,.T.);
#13247=ORIENTED_EDGE('',*,*,#10164,.F.);
#13248=ORIENTED_EDGE('',*,*,#9963,.F.);
#13249=ORIENTED_EDGE('',*,*,#10165,.T.);
#13250=ORIENTED_EDGE('',*,*,#10166,.T.);
#13251=ORIENTED_EDGE('',*,*,#10094,.T.);
#13252=ORIENTED_EDGE('',*,*,#10165,.F.);
#13253=ORIENTED_EDGE('',*,*,#9962,.F.);
#13254=ORIENTED_EDGE('',*,*,#10167,.T.);
#13255=ORIENTED_EDGE('',*,*,#10168,.T.);
#13256=ORIENTED_EDGE('',*,*,#10095,.T.);
#13257=ORIENTED_EDGE('',*,*,#10166,.F.);
#13258=ORIENTED_EDGE('',*,*,#10167,.F.);
#13259=ORIENTED_EDGE('',*,*,#9961,.F.);
#13260=ORIENTED_EDGE('',*,*,#10169,.T.);
#13261=ORIENTED_EDGE('',*,*,#10096,.T.);
#13262=ORIENTED_EDGE('',*,*,#10168,.F.);
#13263=ORIENTED_EDGE('',*,*,#10169,.F.);
#13264=ORIENTED_EDGE('',*,*,#9960,.F.);
#13265=ORIENTED_EDGE('',*,*,#10170,.T.);
#13266=ORIENTED_EDGE('',*,*,#10097,.T.);
#13267=ORIENTED_EDGE('',*,*,#10170,.F.);
#13268=ORIENTED_EDGE('',*,*,#9959,.F.);
#13269=ORIENTED_EDGE('',*,*,#10171,.T.);
#13270=ORIENTED_EDGE('',*,*,#10098,.T.);
#13271=ORIENTED_EDGE('',*,*,#10171,.F.);
#13272=ORIENTED_EDGE('',*,*,#9958,.F.);
#13273=ORIENTED_EDGE('',*,*,#10172,.T.);
#13274=ORIENTED_EDGE('',*,*,#10099,.T.);
#13275=ORIENTED_EDGE('',*,*,#10172,.F.);
#13276=ORIENTED_EDGE('',*,*,#9957,.F.);
#13277=ORIENTED_EDGE('',*,*,#10173,.T.);
#13278=ORIENTED_EDGE('',*,*,#10174,.T.);
#13279=ORIENTED_EDGE('',*,*,#10100,.T.);
#13280=ORIENTED_EDGE('',*,*,#10173,.F.);
#13281=ORIENTED_EDGE('',*,*,#9956,.F.);
#13282=ORIENTED_EDGE('',*,*,#10175,.T.);
#13283=ORIENTED_EDGE('',*,*,#10176,.T.);
#13284=ORIENTED_EDGE('',*,*,#10101,.T.);
#13285=ORIENTED_EDGE('',*,*,#10174,.F.);
#13286=ORIENTED_EDGE('',*,*,#10175,.F.);
#13287=ORIENTED_EDGE('',*,*,#9955,.F.);
#13288=ORIENTED_EDGE('',*,*,#10177,.T.);
#13289=ORIENTED_EDGE('',*,*,#10178,.T.);
#13290=ORIENTED_EDGE('',*,*,#10102,.T.);
#13291=ORIENTED_EDGE('',*,*,#10176,.F.);
#13292=ORIENTED_EDGE('',*,*,#10177,.F.);
#13293=ORIENTED_EDGE('',*,*,#9954,.F.);
#13294=ORIENTED_EDGE('',*,*,#10179,.T.);
#13295=ORIENTED_EDGE('',*,*,#10103,.T.);
#13296=ORIENTED_EDGE('',*,*,#10178,.F.);
#13297=ORIENTED_EDGE('',*,*,#10179,.F.);
#13298=ORIENTED_EDGE('',*,*,#9953,.F.);
#13299=ORIENTED_EDGE('',*,*,#10180,.T.);
#13300=ORIENTED_EDGE('',*,*,#10104,.T.);
#13301=ORIENTED_EDGE('',*,*,#10181,.F.);
#13302=ORIENTED_EDGE('',*,*,#9973,.F.);
#13303=ORIENTED_EDGE('',*,*,#10182,.T.);
#13304=ORIENTED_EDGE('',*,*,#10084,.T.);
#13305=ORIENTED_EDGE('',*,*,#10183,.F.);
#13306=ORIENTED_EDGE('',*,*,#10182,.F.);
#13307=ORIENTED_EDGE('',*,*,#9972,.F.);
#13308=ORIENTED_EDGE('',*,*,#10184,.T.);
#13309=ORIENTED_EDGE('',*,*,#10085,.T.);
#13310=ORIENTED_EDGE('',*,*,#10184,.F.);
#13311=ORIENTED_EDGE('',*,*,#9971,.F.);
#13312=ORIENTED_EDGE('',*,*,#10185,.T.);
#13313=ORIENTED_EDGE('',*,*,#10086,.T.);
#13314=ORIENTED_EDGE('',*,*,#10185,.F.);
#13315=ORIENTED_EDGE('',*,*,#9970,.F.);
#13316=ORIENTED_EDGE('',*,*,#10186,.T.);
#13317=ORIENTED_EDGE('',*,*,#10087,.T.);
#13318=ORIENTED_EDGE('',*,*,#10186,.F.);
#13319=ORIENTED_EDGE('',*,*,#9969,.F.);
#13320=ORIENTED_EDGE('',*,*,#10187,.T.);
#13321=ORIENTED_EDGE('',*,*,#10088,.T.);
#13322=ORIENTED_EDGE('',*,*,#10187,.F.);
#13323=ORIENTED_EDGE('',*,*,#9968,.F.);
#13324=ORIENTED_EDGE('',*,*,#10188,.T.);
#13325=ORIENTED_EDGE('',*,*,#10089,.T.);
#13326=ORIENTED_EDGE('',*,*,#10189,.F.);
#13327=ORIENTED_EDGE('',*,*,#9980,.F.);
#13328=ORIENTED_EDGE('',*,*,#10190,.T.);
#13329=ORIENTED_EDGE('',*,*,#10077,.T.);
#13330=ORIENTED_EDGE('',*,*,#10190,.F.);
#13331=ORIENTED_EDGE('',*,*,#9979,.F.);
#13332=ORIENTED_EDGE('',*,*,#10191,.T.);
#13333=ORIENTED_EDGE('',*,*,#10078,.T.);
#13334=ORIENTED_EDGE('',*,*,#10191,.F.);
#13335=ORIENTED_EDGE('',*,*,#9978,.F.);
#13336=ORIENTED_EDGE('',*,*,#10192,.T.);
#13337=ORIENTED_EDGE('',*,*,#10079,.T.);
#13338=ORIENTED_EDGE('',*,*,#10192,.F.);
#13339=ORIENTED_EDGE('',*,*,#9977,.F.);
#13340=ORIENTED_EDGE('',*,*,#10193,.T.);
#13341=ORIENTED_EDGE('',*,*,#10080,.T.);
#13342=ORIENTED_EDGE('',*,*,#10193,.F.);
#13343=ORIENTED_EDGE('',*,*,#9976,.F.);
#13344=ORIENTED_EDGE('',*,*,#10194,.T.);
#13345=ORIENTED_EDGE('',*,*,#10195,.T.);
#13346=ORIENTED_EDGE('',*,*,#10081,.T.);
#13347=ORIENTED_EDGE('',*,*,#10194,.F.);
#13348=ORIENTED_EDGE('',*,*,#9975,.F.);
#13349=ORIENTED_EDGE('',*,*,#10196,.T.);
#13350=ORIENTED_EDGE('',*,*,#10082,.T.);
#13351=ORIENTED_EDGE('',*,*,#10195,.F.);
#13352=ORIENTED_EDGE('',*,*,#10197,.F.);
#13353=ORIENTED_EDGE('',*,*,#9995,.F.);
#13354=ORIENTED_EDGE('',*,*,#10198,.T.);
#13355=ORIENTED_EDGE('',*,*,#10199,.T.);
#13356=ORIENTED_EDGE('',*,*,#10062,.T.);
#13357=ORIENTED_EDGE('',*,*,#10198,.F.);
#13358=ORIENTED_EDGE('',*,*,#9994,.F.);
#13359=ORIENTED_EDGE('',*,*,#10200,.T.);
#13360=ORIENTED_EDGE('',*,*,#10201,.T.);
#13361=ORIENTED_EDGE('',*,*,#10063,.T.);
#13362=ORIENTED_EDGE('',*,*,#10199,.F.);
#13363=ORIENTED_EDGE('',*,*,#10200,.F.);
#13364=ORIENTED_EDGE('',*,*,#9993,.F.);
#13365=ORIENTED_EDGE('',*,*,#10202,.T.);
#13366=ORIENTED_EDGE('',*,*,#10203,.T.);
#13367=ORIENTED_EDGE('',*,*,#10064,.T.);
#13368=ORIENTED_EDGE('',*,*,#10201,.F.);
#13369=ORIENTED_EDGE('',*,*,#10202,.F.);
#13370=ORIENTED_EDGE('',*,*,#9992,.F.);
#13371=ORIENTED_EDGE('',*,*,#10204,.T.);
#13372=ORIENTED_EDGE('',*,*,#10065,.T.);
#13373=ORIENTED_EDGE('',*,*,#10203,.F.);
#13374=ORIENTED_EDGE('',*,*,#10204,.F.);
#13375=ORIENTED_EDGE('',*,*,#9991,.F.);
#13376=ORIENTED_EDGE('',*,*,#10205,.T.);
#13377=ORIENTED_EDGE('',*,*,#10066,.T.);
#13378=ORIENTED_EDGE('',*,*,#10205,.F.);
#13379=ORIENTED_EDGE('',*,*,#9990,.F.);
#13380=ORIENTED_EDGE('',*,*,#10206,.T.);
#13381=ORIENTED_EDGE('',*,*,#10067,.T.);
#13382=ORIENTED_EDGE('',*,*,#10206,.F.);
#13383=ORIENTED_EDGE('',*,*,#9989,.F.);
#13384=ORIENTED_EDGE('',*,*,#10207,.T.);
#13385=ORIENTED_EDGE('',*,*,#10068,.T.);
#13386=ORIENTED_EDGE('',*,*,#10207,.F.);
#13387=ORIENTED_EDGE('',*,*,#9988,.F.);
#13388=ORIENTED_EDGE('',*,*,#10208,.T.);
#13389=ORIENTED_EDGE('',*,*,#10209,.T.);
#13390=ORIENTED_EDGE('',*,*,#10069,.T.);
#13391=ORIENTED_EDGE('',*,*,#10208,.F.);
#13392=ORIENTED_EDGE('',*,*,#9987,.F.);
#13393=ORIENTED_EDGE('',*,*,#10210,.T.);
#13394=ORIENTED_EDGE('',*,*,#10211,.T.);
#13395=ORIENTED_EDGE('',*,*,#10070,.T.);
#13396=ORIENTED_EDGE('',*,*,#10209,.F.);
#13397=ORIENTED_EDGE('',*,*,#10210,.F.);
#13398=ORIENTED_EDGE('',*,*,#9986,.F.);
#13399=ORIENTED_EDGE('',*,*,#10212,.T.);
#13400=ORIENTED_EDGE('',*,*,#10071,.T.);
#13401=ORIENTED_EDGE('',*,*,#10211,.F.);
#13402=ORIENTED_EDGE('',*,*,#10212,.F.);
#13403=ORIENTED_EDGE('',*,*,#9985,.F.);
#13404=ORIENTED_EDGE('',*,*,#10213,.T.);
#13405=ORIENTED_EDGE('',*,*,#10072,.T.);
#13406=ORIENTED_EDGE('',*,*,#10213,.F.);
#13407=ORIENTED_EDGE('',*,*,#9984,.F.);
#13408=ORIENTED_EDGE('',*,*,#10214,.T.);
#13409=ORIENTED_EDGE('',*,*,#10073,.T.);
#13410=ORIENTED_EDGE('',*,*,#10214,.F.);
#13411=ORIENTED_EDGE('',*,*,#9983,.F.);
#13412=ORIENTED_EDGE('',*,*,#10215,.T.);
#13413=ORIENTED_EDGE('',*,*,#10074,.T.);
#13414=ORIENTED_EDGE('',*,*,#10216,.F.);
#13415=ORIENTED_EDGE('',*,*,#10007,.F.);
#13416=ORIENTED_EDGE('',*,*,#10217,.T.);
#13417=ORIENTED_EDGE('',*,*,#10050,.T.);
#13418=ORIENTED_EDGE('',*,*,#10218,.F.);
#13419=ORIENTED_EDGE('',*,*,#10217,.F.);
#13420=ORIENTED_EDGE('',*,*,#10006,.F.);
#13421=ORIENTED_EDGE('',*,*,#10219,.T.);
#13422=ORIENTED_EDGE('',*,*,#10051,.T.);
#13423=ORIENTED_EDGE('',*,*,#10219,.F.);
#13424=ORIENTED_EDGE('',*,*,#10005,.F.);
#13425=ORIENTED_EDGE('',*,*,#10220,.T.);
#13426=ORIENTED_EDGE('',*,*,#10052,.T.);
#13427=ORIENTED_EDGE('',*,*,#10220,.F.);
#13428=ORIENTED_EDGE('',*,*,#10004,.F.);
#13429=ORIENTED_EDGE('',*,*,#10221,.T.);
#13430=ORIENTED_EDGE('',*,*,#10053,.T.);
#13431=ORIENTED_EDGE('',*,*,#10221,.F.);
#13432=ORIENTED_EDGE('',*,*,#10003,.F.);
#13433=ORIENTED_EDGE('',*,*,#10222,.T.);
#13434=ORIENTED_EDGE('',*,*,#10054,.T.);
#13435=ORIENTED_EDGE('',*,*,#10222,.F.);
#13436=ORIENTED_EDGE('',*,*,#10002,.F.);
#13437=ORIENTED_EDGE('',*,*,#10223,.T.);
#13438=ORIENTED_EDGE('',*,*,#10055,.T.);
#13439=ORIENTED_EDGE('',*,*,#10223,.F.);
#13440=ORIENTED_EDGE('',*,*,#10001,.F.);
#13441=ORIENTED_EDGE('',*,*,#10224,.T.);
#13442=ORIENTED_EDGE('',*,*,#10056,.T.);
#13443=ORIENTED_EDGE('',*,*,#10224,.F.);
#13444=ORIENTED_EDGE('',*,*,#10000,.F.);
#13445=ORIENTED_EDGE('',*,*,#10225,.T.);
#13446=ORIENTED_EDGE('',*,*,#10057,.T.);
#13447=ORIENTED_EDGE('',*,*,#10225,.F.);
#13448=ORIENTED_EDGE('',*,*,#9999,.F.);
#13449=ORIENTED_EDGE('',*,*,#10226,.T.);
#13450=ORIENTED_EDGE('',*,*,#10058,.T.);
#13451=ORIENTED_EDGE('',*,*,#10226,.F.);
#13452=ORIENTED_EDGE('',*,*,#9998,.F.);
#13453=ORIENTED_EDGE('',*,*,#10227,.T.);
#13454=ORIENTED_EDGE('',*,*,#10059,.T.);
#13455=ORIENTED_EDGE('',*,*,#10227,.F.);
#13456=ORIENTED_EDGE('',*,*,#9997,.F.);
#13457=ORIENTED_EDGE('',*,*,#10228,.T.);
#13458=ORIENTED_EDGE('',*,*,#10060,.T.);
#13459=ORIENTED_EDGE('',*,*,#10229,.F.);
#13460=ORIENTED_EDGE('',*,*,#9951,.F.);
#13461=ORIENTED_EDGE('',*,*,#10230,.T.);
#13462=ORIENTED_EDGE('',*,*,#10106,.T.);
#13463=ORIENTED_EDGE('',*,*,#10230,.F.);
#13464=ORIENTED_EDGE('',*,*,#9950,.F.);
#13465=ORIENTED_EDGE('',*,*,#10231,.T.);
#13466=ORIENTED_EDGE('',*,*,#10107,.T.);
#13467=ORIENTED_EDGE('',*,*,#10231,.F.);
#13468=ORIENTED_EDGE('',*,*,#9949,.F.);
#13469=ORIENTED_EDGE('',*,*,#10232,.T.);
#13470=ORIENTED_EDGE('',*,*,#10108,.T.);
#13471=ORIENTED_EDGE('',*,*,#10232,.F.);
#13472=ORIENTED_EDGE('',*,*,#9948,.F.);
#13473=ORIENTED_EDGE('',*,*,#10233,.T.);
#13474=ORIENTED_EDGE('',*,*,#10109,.T.);
#13475=ORIENTED_EDGE('',*,*,#10233,.F.);
#13476=ORIENTED_EDGE('',*,*,#9947,.F.);
#13477=ORIENTED_EDGE('',*,*,#10234,.T.);
#13478=ORIENTED_EDGE('',*,*,#10110,.T.);
#13479=ORIENTED_EDGE('',*,*,#10234,.F.);
#13480=ORIENTED_EDGE('',*,*,#9946,.F.);
#13481=ORIENTED_EDGE('',*,*,#10235,.T.);
#13482=ORIENTED_EDGE('',*,*,#10111,.T.);
#13483=ORIENTED_EDGE('',*,*,#10235,.F.);
#13484=ORIENTED_EDGE('',*,*,#9945,.F.);
#13485=ORIENTED_EDGE('',*,*,#10236,.T.);
#13486=ORIENTED_EDGE('',*,*,#10112,.T.);
#13487=ORIENTED_EDGE('',*,*,#10236,.F.);
#13488=ORIENTED_EDGE('',*,*,#9944,.F.);
#13489=ORIENTED_EDGE('',*,*,#10237,.T.);
#13490=ORIENTED_EDGE('',*,*,#10113,.T.);
#13491=ORIENTED_EDGE('',*,*,#10237,.F.);
#13492=ORIENTED_EDGE('',*,*,#9943,.F.);
#13493=ORIENTED_EDGE('',*,*,#10238,.T.);
#13494=ORIENTED_EDGE('',*,*,#10114,.T.);
#13495=ORIENTED_EDGE('',*,*,#10238,.F.);
#13496=ORIENTED_EDGE('',*,*,#9942,.F.);
#13497=ORIENTED_EDGE('',*,*,#10239,.T.);
#13498=ORIENTED_EDGE('',*,*,#10240,.T.);
#13499=ORIENTED_EDGE('',*,*,#10115,.T.);
#13500=ORIENTED_EDGE('',*,*,#10239,.F.);
#13501=ORIENTED_EDGE('',*,*,#9941,.F.);
#13502=ORIENTED_EDGE('',*,*,#10241,.T.);
#13503=ORIENTED_EDGE('',*,*,#10048,.T.);
#13504=ORIENTED_EDGE('',*,*,#10240,.F.);
#13505=ORIENTED_EDGE('',*,*,#10229,.T.);
#13506=ORIENTED_EDGE('',*,*,#10105,.T.);
#13507=ORIENTED_EDGE('',*,*,#10180,.F.);
#13508=ORIENTED_EDGE('',*,*,#9952,.F.);
#13509=ORIENTED_EDGE('',*,*,#10216,.T.);
#13510=ORIENTED_EDGE('',*,*,#10218,.T.);
#13511=ORIENTED_EDGE('',*,*,#10049,.T.);
#13512=ORIENTED_EDGE('',*,*,#10241,.F.);
#13513=ORIENTED_EDGE('',*,*,#10008,.F.);
#13514=ORIENTED_EDGE('',*,*,#10197,.T.);
#13515=ORIENTED_EDGE('',*,*,#10061,.T.);
#13516=ORIENTED_EDGE('',*,*,#10228,.F.);
#13517=ORIENTED_EDGE('',*,*,#9996,.F.);
#13518=ORIENTED_EDGE('',*,*,#9982,.F.);
#13519=ORIENTED_EDGE('',*,*,#10242,.T.);
#13520=ORIENTED_EDGE('',*,*,#10075,.T.);
#13521=ORIENTED_EDGE('',*,*,#10215,.F.);
#13522=ORIENTED_EDGE('',*,*,#10189,.T.);
#13523=ORIENTED_EDGE('',*,*,#10076,.T.);
#13524=ORIENTED_EDGE('',*,*,#10242,.F.);
#13525=ORIENTED_EDGE('',*,*,#9981,.F.);
#13526=ORIENTED_EDGE('',*,*,#10181,.T.);
#13527=ORIENTED_EDGE('',*,*,#10183,.T.);
#13528=ORIENTED_EDGE('',*,*,#10083,.T.);
#13529=ORIENTED_EDGE('',*,*,#10196,.F.);
#13530=ORIENTED_EDGE('',*,*,#9974,.F.);
#13531=ORIENTED_EDGE('',*,*,#9967,.F.);
#13532=ORIENTED_EDGE('',*,*,#10243,.T.);
#13533=ORIENTED_EDGE('',*,*,#10090,.T.);
#13534=ORIENTED_EDGE('',*,*,#10188,.F.);
#13535=ORIENTED_EDGE('',*,*,#10162,.T.);
#13536=ORIENTED_EDGE('',*,*,#10091,.T.);
#13537=ORIENTED_EDGE('',*,*,#10243,.F.);
#13538=ORIENTED_EDGE('',*,*,#9966,.F.);
#18849=B_SPLINE_SURFACE_WITH_KNOTS('',3,3,((#28196,#28197,#28198,#28199,
#28200,#28201,#28202,#28203,#28204,#28205,#28206,#28207,#28208,#28209,#28210,
#28211,#28212,#28213,#28214,#28215,#28216,#28217,#28218,#28219,#28220,#28221,
#28222,#28223,#28224,#28225,#28226,#28227,#28228,#28229,#28230,#28231,#28232,
#28233,#28234,#28235,#28236,#28237,#28238,#28239,#28240),(#28241,#28242,
#28243,#28244,#28245,#28246,#28247,#28248,#28249,#28250,#28251,#28252,#28253,
#28254,#28255,#28256,#28257,#28258,#28259,#28260,#28261,#28262,#28263,#28264,
#28265,#28266,#28267,#28268,#28269,#28270,#28271,#28272,#28273,#28274,#28275,
#28276,#28277,#28278,#28279,#28280,#28281,#28282,#28283,#28284,#28285),
(#28286,#28287,#28288,#28289,#28290,#28291,#28292,#28293,#28294,#28295,
#28296,#28297,#28298,#28299,#28300,#28301,#28302,#28303,#28304,#28305,#28306,
#28307,#28308,#28309,#28310,#28311,#28312,#28313,#28314,#28315,#28316,#28317,
#28318,#28319,#28320,#28321,#28322,#28323,#28324,#28325,#28326,#28327,#28328,
#28329,#28330),(#28331,#28332,#28333,#28334,#28335,#28336,#28337,#28338,
#28339,#28340,#28341,#28342,#28343,#28344,#28345,#28346,#28347,#28348,#28349,
#28350,#28351,#28352,#28353,#28354,#28355,#28356,#28357,#28358,#28359,#28360,
#28361,#28362,#28363,#28364,#28365,#28366,#28367,#28368,#28369,#28370,#28371,
#28372,#28373,#28374,#28375),(#28376,#28377,#28378,#28379,#28380,#28381,
#28382,#28383,#28384,#28385,#28386,#28387,#28388,#28389,#28390,#28391,#28392,
#28393,#28394,#28395,#28396,#28397,#28398,#28399,#28400,#28401,#28402,#28403,
#28404,#28405,#28406,#28407,#28408,#28409,#28410,#28411,#28412,#28413,#28414,
#28415,#28416,#28417,#28418,#28419,#28420),(#28421,#28422,#28423,#28424,
#28425,#28426,#28427,#28428,#28429,#28430,#28431,#28432,#28433,#28434,#28435,
#28436,#28437,#28438,#28439,#28440,#28441,#28442,#28443,#28444,#28445,#28446,
#28447,#28448,#28449,#28450,#28451,#28452,#28453,#28454,#28455,#28456,#28457,
#28458,#28459,#28460,#28461,#28462,#28463,#28464,#28465)),.UNSPECIFIED.,
 .F.,.T.,.F.,(4,1,1,4),(4,2,2,2,2,1,1,2,2,1,2,1,1,1,2,1,1,1,2,1,1,1,1,1,
1,1,1,1,1,2,1,1,4),(0.,0.285714285714286,0.571428571428571,1.00025096923236),
(-13.0076216717983,-12.6762562420903,-11.8531689108674,-11.05258106389,
-10.1188927640438,-8.47830334468407,-7.04278760274435,-6.83771392532439,
-5.90055842268743,-5.54885349043522,-5.09666143468238,-4.98988621289018,
-4.88311099109797,-4.50939771482526,-4.24245966034475,-3.88978669781647,
-3.67818292029951,-3.43131184652972,-3.11390618025428,-3.0769781504351,
-2.96619406097756,-2.81848194170084,-2.7076978522433,-2.5230577031474,-1.93220922604053,
-1.78449710676381,-1.74756907694463,-1.34136074893366,-1.04593651038022,
-0.750512271826782,-0.60979122085926,-0.469070169891739,0.),
 .UNSPECIFIED.);
#18850=B_SPLINE_SURFACE_WITH_KNOTS('',3,3,((#28856,#28857,#28858,#28859,
#28860,#28861,#28862,#28863,#28864,#28865,#28866,#28867,#28868,#28869,#28870,
#28871,#28872,#28873,#28874,#28875,#28876,#28877,#28878,#28879,#28880,#28881,
#28882,#28883,#28884,#28885,#28886,#28887,#28888,#28889,#28890,#28891,#28892,
#28893,#28894,#28895,#28896,#28897,#28898,#28899,#28900,#28901,#28902,#28903,
#28904,#28905,#28906,#28907,#28908,#28909,#28910,#28911,#28912,#28913,#28914,
#28915,#28916,#28917,#28918,#28919,#28920,#28921,#28922,#28923,#28924,#28925,
#28926,#28927,#28928,#28929,#28930,#28931,#28932,#28933,#28934,#28935,#28936,
#28937,#28938,#28939,#28940,#28941,#28942,#28943,#28944,#28945,#28946,#28947,
#28948,#28949,#28950,#28951,#28952,#28953,#28954,#28955,#28956,#28957,#28958,
#28959,#28960,#28961,#28962,#28963,#28964,#28965,#28966,#28967,#28968,#28969,
#28970,#28971,#28972,#28973,#28974,#28975,#28976,#28977,#28978,#28979,#28980,
#28981,#28982,#28983,#28984,#28985,#28986,#28987,#28988,#28989,#28990,#28991,
#28992,#28993,#28994,#28995,#28996,#28997,#28998,#28999),(#29000,#29001,
#29002,#29003,#29004,#29005,#29006,#29007,#29008,#29009,#29010,#29011,#29012,
#29013,#29014,#29015,#29016,#29017,#29018,#29019,#29020,#29021,#29022,#29023,
#29024,#29025,#29026,#29027,#29028,#29029,#29030,#29031,#29032,#29033,#29034,
#29035,#29036,#29037,#29038,#29039,#29040,#29041,#29042,#29043,#29044,#29045,
#29046,#29047,#29048,#29049,#29050,#29051,#29052,#29053,#29054,#29055,#29056,
#29057,#29058,#29059,#29060,#29061,#29062,#29063,#29064,#29065,#29066,#29067,
#29068,#29069,#29070,#29071,#29072,#29073,#29074,#29075,#29076,#29077,#29078,
#29079,#29080,#29081,#29082,#29083,#29084,#29085,#29086,#29087,#29088,#29089,
#29090,#29091,#29092,#29093,#29094,#29095,#29096,#29097,#29098,#29099,#29100,
#29101,#29102,#29103,#29104,#29105,#29106,#29107,#29108,#29109,#29110,#29111,
#29112,#29113,#29114,#29115,#29116,#29117,#29118,#29119,#29120,#29121,#29122,
#29123,#29124,#29125,#29126,#29127,#29128,#29129,#29130,#29131,#29132,#29133,
#29134,#29135,#29136,#29137,#29138,#29139,#29140,#29141,#29142,#29143),
(#29144,#29145,#29146,#29147,#29148,#29149,#29150,#29151,#29152,#29153,
#29154,#29155,#29156,#29157,#29158,#29159,#29160,#29161,#29162,#29163,#29164,
#29165,#29166,#29167,#29168,#29169,#29170,#29171,#29172,#29173,#29174,#29175,
#29176,#29177,#29178,#29179,#29180,#29181,#29182,#29183,#29184,#29185,#29186,
#29187,#29188,#29189,#29190,#29191,#29192,#29193,#29194,#29195,#29196,#29197,
#29198,#29199,#29200,#29201,#29202,#29203,#29204,#29205,#29206,#29207,#29208,
#29209,#29210,#29211,#29212,#29213,#29214,#29215,#29216,#29217,#29218,#29219,
#29220,#29221,#29222,#29223,#29224,#29225,#29226,#29227,#29228,#29229,#29230,
#29231,#29232,#29233,#29234,#29235,#29236,#29237,#29238,#29239,#29240,#29241,
#29242,#29243,#29244,#29245,#29246,#29247,#29248,#29249,#29250,#29251,#29252,
#29253,#29254,#29255,#29256,#29257,#29258,#29259,#29260,#29261,#29262,#29263,
#29264,#29265,#29266,#29267,#29268,#29269,#29270,#29271,#29272,#29273,#29274,
#29275,#29276,#29277,#29278,#29279,#29280,#29281,#29282,#29283,#29284,#29285,
#29286,#29287),(#29288,#29289,#29290,#29291,#29292,#29293,#29294,#29295,
#29296,#29297,#29298,#29299,#29300,#29301,#29302,#29303,#29304,#29305,#29306,
#29307,#29308,#29309,#29310,#29311,#29312,#29313,#29314,#29315,#29316,#29317,
#29318,#29319,#29320,#29321,#29322,#29323,#29324,#29325,#29326,#29327,#29328,
#29329,#29330,#29331,#29332,#29333,#29334,#29335,#29336,#29337,#29338,#29339,
#29340,#29341,#29342,#29343,#29344,#29345,#29346,#29347,#29348,#29349,#29350,
#29351,#29352,#29353,#29354,#29355,#29356,#29357,#29358,#29359,#29360,#29361,
#29362,#29363,#29364,#29365,#29366,#29367,#29368,#29369,#29370,#29371,#29372,
#29373,#29374,#29375,#29376,#29377,#29378,#29379,#29380,#29381,#29382,#29383,
#29384,#29385,#29386,#29387,#29388,#29389,#29390,#29391,#29392,#29393,#29394,
#29395,#29396,#29397,#29398,#29399,#29400,#29401,#29402,#29403,#29404,#29405,
#29406,#29407,#29408,#29409,#29410,#29411,#29412,#29413,#29414,#29415,#29416,
#29417,#29418,#29419,#29420,#29421,#29422,#29423,#29424,#29425,#29426,#29427,
#29428,#29429,#29430,#29431),(#29432,#29433,#29434,#29435,#29436,#29437,
#29438,#29439,#29440,#29441,#29442,#29443,#29444,#29445,#29446,#29447,#29448,
#29449,#29450,#29451,#29452,#29453,#29454,#29455,#29456,#29457,#29458,#29459,
#29460,#29461,#29462,#29463,#29464,#29465,#29466,#29467,#29468,#29469,#29470,
#29471,#29472,#29473,#29474,#29475,#29476,#29477,#29478,#29479,#29480,#29481,
#29482,#29483,#29484,#29485,#29486,#29487,#29488,#29489,#29490,#29491,#29492,
#29493,#29494,#29495,#29496,#29497,#29498,#29499,#29500,#29501,#29502,#29503,
#29504,#29505,#29506,#29507,#29508,#29509,#29510,#29511,#29512,#29513,#29514,
#29515,#29516,#29517,#29518,#29519,#29520,#29521,#29522,#29523,#29524,#29525,
#29526,#29527,#29528,#29529,#29530,#29531,#29532,#29533,#29534,#29535,#29536,
#29537,#29538,#29539,#29540,#29541,#29542,#29543,#29544,#29545,#29546,#29547,
#29548,#29549,#29550,#29551,#29552,#29553,#29554,#29555,#29556,#29557,#29558,
#29559,#29560,#29561,#29562,#29563,#29564,#29565,#29566,#29567,#29568,#29569,
#29570,#29571,#29572,#29573,#29574,#29575),(#29576,#29577,#29578,#29579,
#29580,#29581,#29582,#29583,#29584,#29585,#29586,#29587,#29588,#29589,#29590,
#29591,#29592,#29593,#29594,#29595,#29596,#29597,#29598,#29599,#29600,#29601,
#29602,#29603,#29604,#29605,#29606,#29607,#29608,#29609,#29610,#29611,#29612,
#29613,#29614,#29615,#29616,#29617,#29618,#29619,#29620,#29621,#29622,#29623,
#29624,#29625,#29626,#29627,#29628,#29629,#29630,#29631,#29632,#29633,#29634,
#29635,#29636,#29637,#29638,#29639,#29640,#29641,#29642,#29643,#29644,#29645,
#29646,#29647,#29648,#29649,#29650,#29651,#29652,#29653,#29654,#29655,#29656,
#29657,#29658,#29659,#29660,#29661,#29662,#29663,#29664,#29665,#29666,#29667,
#29668,#29669,#29670,#29671,#29672,#29673,#29674,#29675,#29676,#29677,#29678,
#29679,#29680,#29681,#29682,#29683,#29684,#29685,#29686,#29687,#29688,#29689,
#29690,#29691,#29692,#29693,#29694,#29695,#29696,#29697,#29698,#29699,#29700,
#29701,#29702,#29703,#29704,#29705,#29706,#29707,#29708,#29709,#29710,#29711,
#29712,#29713,#29714,#29715,#29716,#29717,#29718,#29719),(#29720,#29721,
#29722,#29723,#29724,#29725,#29726,#29727,#29728,#29729,#29730,#29731,#29732,
#29733,#29734,#29735,#29736,#29737,#29738,#29739,#29740,#29741,#29742,#29743,
#29744,#29745,#29746,#29747,#29748,#29749,#29750,#29751,#29752,#29753,#29754,
#29755,#29756,#29757,#29758,#29759,#29760,#29761,#29762,#29763,#29764,#29765,
#29766,#29767,#29768,#29769,#29770,#29771,#29772,#29773,#29774,#29775,#29776,
#29777,#29778,#29779,#29780,#29781,#29782,#29783,#29784,#29785,#29786,#29787,
#29788,#29789,#29790,#29791,#29792,#29793,#29794,#29795,#29796,#29797,#29798,
#29799,#29800,#29801,#29802,#29803,#29804,#29805,#29806,#29807,#29808,#29809,
#29810,#29811,#29812,#29813,#29814,#29815,#29816,#29817,#29818,#29819,#29820,
#29821,#29822,#29823,#29824,#29825,#29826,#29827,#29828,#29829,#29830,#29831,
#29832,#29833,#29834,#29835,#29836,#29837,#29838,#29839,#29840,#29841,#29842,
#29843,#29844,#29845,#29846,#29847,#29848,#29849,#29850,#29851,#29852,#29853,
#29854,#29855,#29856,#29857,#29858,#29859,#29860,#29861,#29862,#29863),
(#29864,#29865,#29866,#29867,#29868,#29869,#29870,#29871,#29872,#29873,
#29874,#29875,#29876,#29877,#29878,#29879,#29880,#29881,#29882,#29883,#29884,
#29885,#29886,#29887,#29888,#29889,#29890,#29891,#29892,#29893,#29894,#29895,
#29896,#29897,#29898,#29899,#29900,#29901,#29902,#29903,#29904,#29905,#29906,
#29907,#29908,#29909,#29910,#29911,#29912,#29913,#29914,#29915,#29916,#29917,
#29918,#29919,#29920,#29921,#29922,#29923,#29924,#29925,#29926,#29927,#29928,
#29929,#29930,#29931,#29932,#29933,#29934,#29935,#29936,#29937,#29938,#29939,
#29940,#29941,#29942,#29943,#29944,#29945,#29946,#29947,#29948,#29949,#29950,
#29951,#29952,#29953,#29954,#29955,#29956,#29957,#29958,#29959,#29960,#29961,
#29962,#29963,#29964,#29965,#29966,#29967,#29968,#29969,#29970,#29971,#29972,
#29973,#29974,#29975,#29976,#29977,#29978,#29979,#29980,#29981,#29982,#29983,
#29984,#29985,#29986,#29987,#29988,#29989,#29990,#29991,#29992,#29993,#29994,
#29995,#29996,#29997,#29998,#29999,#30000,#30001,#30002,#30003,#30004,#30005,
#30006,#30007),(#30008,#30009,#30010,#30011,#30012,#30013,#30014,#30015,
#30016,#30017,#30018,#30019,#30020,#30021,#30022,#30023,#30024,#30025,#30026,
#30027,#30028,#30029,#30030,#30031,#30032,#30033,#30034,#30035,#30036,#30037,
#30038,#30039,#30040,#30041,#30042,#30043,#30044,#30045,#30046,#30047,#30048,
#30049,#30050,#30051,#30052,#30053,#30054,#30055,#30056,#30057,#30058,#30059,
#30060,#30061,#30062,#30063,#30064,#30065,#30066,#30067,#30068,#30069,#30070,
#30071,#30072,#30073,#30074,#30075,#30076,#30077,#30078,#30079,#30080,#30081,
#30082,#30083,#30084,#30085,#30086,#30087,#30088,#30089,#30090,#30091,#30092,
#30093,#30094,#30095,#30096,#30097,#30098,#30099,#30100,#30101,#30102,#30103,
#30104,#30105,#30106,#30107,#30108,#30109,#30110,#30111,#30112,#30113,#30114,
#30115,#30116,#30117,#30118,#30119,#30120,#30121,#30122,#30123,#30124,#30125,
#30126,#30127,#30128,#30129,#30130,#30131,#30132,#30133,#30134,#30135,#30136,
#30137,#30138,#30139,#30140,#30141,#30142,#30143,#30144,#30145,#30146,#30147,
#30148,#30149,#30150,#30151),(#30152,#30153,#30154,#30155,#30156,#30157,
#30158,#30159,#30160,#30161,#30162,#30163,#30164,#30165,#30166,#30167,#30168,
#30169,#30170,#30171,#30172,#30173,#30174,#30175,#30176,#30177,#30178,#30179,
#30180,#30181,#30182,#30183,#30184,#30185,#30186,#30187,#30188,#30189,#30190,
#30191,#30192,#30193,#30194,#30195,#30196,#30197,#30198,#30199,#30200,#30201,
#30202,#30203,#30204,#30205,#30206,#30207,#30208,#30209,#30210,#30211,#30212,
#30213,#30214,#30215,#30216,#30217,#30218,#30219,#30220,#30221,#30222,#30223,
#30224,#30225,#30226,#30227,#30228,#30229,#30230,#30231,#30232,#30233,#30234,
#30235,#30236,#30237,#30238,#30239,#30240,#30241,#30242,#30243,#30244,#30245,
#30246,#30247,#30248,#30249,#30250,#30251,#30252,#30253,#30254,#30255,#30256,
#30257,#30258,#30259,#30260,#30261,#30262,#30263,#30264,#30265,#30266,#30267,
#30268,#30269,#30270,#30271,#30272,#30273,#30274,#30275,#30276,#30277,#30278,
#30279,#30280,#30281,#30282,#30283,#30284,#30285,#30286,#30287,#30288,#30289,
#30290,#30291,#30292,#30293,#30294,#30295),(#30296,#30297,#30298,#30299,
#30300,#30301,#30302,#30303,#30304,#30305,#30306,#30307,#30308,#30309,#30310,
#30311,#30312,#30313,#30314,#30315,#30316,#30317,#30318,#30319,#30320,#30321,
#30322,#30323,#30324,#30325,#30326,#30327,#30328,#30329,#30330,#30331,#30332,
#30333,#30334,#30335,#30336,#30337,#30338,#30339,#30340,#30341,#30342,#30343,
#30344,#30345,#30346,#30347,#30348,#30349,#30350,#30351,#30352,#30353,#30354,
#30355,#30356,#30357,#30358,#30359,#30360,#30361,#30362,#30363,#30364,#30365,
#30366,#30367,#30368,#30369,#30370,#30371,#30372,#30373,#30374,#30375,#30376,
#30377,#30378,#30379,#30380,#30381,#30382,#30383,#30384,#30385,#30386,#30387,
#30388,#30389,#30390,#30391,#30392,#30393,#30394,#30395,#30396,#30397,#30398,
#30399,#30400,#30401,#30402,#30403,#30404,#30405,#30406,#30407,#30408,#30409,
#30410,#30411,#30412,#30413,#30414,#30415,#30416,#30417,#30418,#30419,#30420,
#30421,#30422,#30423,#30424,#30425,#30426,#30427,#30428,#30429,#30430,#30431,
#30432,#30433,#30434,#30435,#30436,#30437,#30438,#30439),(#30440,#30441,
#30442,#30443,#30444,#30445,#30446,#30447,#30448,#30449,#30450,#30451,#30452,
#30453,#30454,#30455,#30456,#30457,#30458,#30459,#30460,#30461,#30462,#30463,
#30464,#30465,#30466,#30467,#30468,#30469,#30470,#30471,#30472,#30473,#30474,
#30475,#30476,#30477,#30478,#30479,#30480,#30481,#30482,#30483,#30484,#30485,
#30486,#30487,#30488,#30489,#30490,#30491,#30492,#30493,#30494,#30495,#30496,
#30497,#30498,#30499,#30500,#30501,#30502,#30503,#30504,#30505,#30506,#30507,
#30508,#30509,#30510,#30511,#30512,#30513,#30514,#30515,#30516,#30517,#30518,
#30519,#30520,#30521,#30522,#30523,#30524,#30525,#30526,#30527,#30528,#30529,
#30530,#30531,#30532,#30533,#30534,#30535,#30536,#30537,#30538,#30539,#30540,
#30541,#30542,#30543,#30544,#30545,#30546,#30547,#30548,#30549,#30550,#30551,
#30552,#30553,#30554,#30555,#30556,#30557,#30558,#30559,#30560,#30561,#30562,
#30563,#30564,#30565,#30566,#30567,#30568,#30569,#30570,#30571,#30572,#30573,
#30574,#30575,#30576,#30577,#30578,#30579,#30580,#30581,#30582,#30583),
(#30584,#30585,#30586,#30587,#30588,#30589,#30590,#30591,#30592,#30593,
#30594,#30595,#30596,#30597,#30598,#30599,#30600,#30601,#30602,#30603,#30604,
#30605,#30606,#30607,#30608,#30609,#30610,#30611,#30612,#30613,#30614,#30615,
#30616,#30617,#30618,#30619,#30620,#30621,#30622,#30623,#30624,#30625,#30626,
#30627,#30628,#30629,#30630,#30631,#30632,#30633,#30634,#30635,#30636,#30637,
#30638,#30639,#30640,#30641,#30642,#30643,#30644,#30645,#30646,#30647,#30648,
#30649,#30650,#30651,#30652,#30653,#30654,#30655,#30656,#30657,#30658,#30659,
#30660,#30661,#30662,#30663,#30664,#30665,#30666,#30667,#30668,#30669,#30670,
#30671,#30672,#30673,#30674,#30675,#30676,#30677,#30678,#30679,#30680,#30681,
#30682,#30683,#30684,#30685,#30686,#30687,#30688,#30689,#30690,#30691,#30692,
#30693,#30694,#30695,#30696,#30697,#30698,#30699,#30700,#30701,#30702,#30703,
#30704,#30705,#30706,#30707,#30708,#30709,#30710,#30711,#30712,#30713,#30714,
#30715,#30716,#30717,#30718,#30719,#30720,#30721,#30722,#30723,#30724,#30725,
#30726,#30727),(#30728,#30729,#30730,#30731,#30732,#30733,#30734,#30735,
#30736,#30737,#30738,#30739,#30740,#30741,#30742,#30743,#30744,#30745,#30746,
#30747,#30748,#30749,#30750,#30751,#30752,#30753,#30754,#30755,#30756,#30757,
#30758,#30759,#30760,#30761,#30762,#30763,#30764,#30765,#30766,#30767,#30768,
#30769,#30770,#30771,#30772,#30773,#30774,#30775,#30776,#30777,#30778,#30779,
#30780,#30781,#30782,#30783,#30784,#30785,#30786,#30787,#30788,#30789,#30790,
#30791,#30792,#30793,#30794,#30795,#30796,#30797,#30798,#30799,#30800,#30801,
#30802,#30803,#30804,#30805,#30806,#30807,#30808,#30809,#30810,#30811,#30812,
#30813,#30814,#30815,#30816,#30817,#30818,#30819,#30820,#30821,#30822,#30823,
#30824,#30825,#30826,#30827,#30828,#30829,#30830,#30831,#30832,#30833,#30834,
#30835,#30836,#30837,#30838,#30839,#30840,#30841,#30842,#30843,#30844,#30845,
#30846,#30847,#30848,#30849,#30850,#30851,#30852,#30853,#30854,#30855,#30856,
#30857,#30858,#30859,#30860,#30861,#30862,#30863,#30864,#30865,#30866,#30867,
#30868,#30869,#30870,#30871),(#30872,#30873,#30874,#30875,#30876,#30877,
#30878,#30879,#30880,#30881,#30882,#30883,#30884,#30885,#30886,#30887,#30888,
#30889,#30890,#30891,#30892,#30893,#30894,#30895,#30896,#30897,#30898,#30899,
#30900,#30901,#30902,#30903,#30904,#30905,#30906,#30907,#30908,#30909,#30910,
#30911,#30912,#30913,#30914,#30915,#30916,#30917,#30918,#30919,#30920,#30921,
#30922,#30923,#30924,#30925,#30926,#30927,#30928,#30929,#30930,#30931,#30932,
#30933,#30934,#30935,#30936,#30937,#30938,#30939,#30940,#30941,#30942,#30943,
#30944,#30945,#30946,#30947,#30948,#30949,#30950,#30951,#30952,#30953,#30954,
#30955,#30956,#30957,#30958,#30959,#30960,#30961,#30962,#30963,#30964,#30965,
#30966,#30967,#30968,#30969,#30970,#30971,#30972,#30973,#30974,#30975,#30976,
#30977,#30978,#30979,#30980,#30981,#30982,#30983,#30984,#30985,#30986,#30987,
#30988,#30989,#30990,#30991,#30992,#30993,#30994,#30995,#30996,#30997,#30998,
#30999,#31000,#31001,#31002,#31003,#31004,#31005,#31006,#31007,#31008,#31009,
#31010,#31011,#31012,#31013,#31014,#31015),(#31016,#31017,#31018,#31019,
#31020,#31021,#31022,#31023,#31024,#31025,#31026,#31027,#31028,#31029,#31030,
#31031,#31032,#31033,#31034,#31035,#31036,#31037,#31038,#31039,#31040,#31041,
#31042,#31043,#31044,#31045,#31046,#31047,#31048,#31049,#31050,#31051,#31052,
#31053,#31054,#31055,#31056,#31057,#31058,#31059,#31060,#31061,#31062,#31063,
#31064,#31065,#31066,#31067,#31068,#31069,#31070,#31071,#31072,#31073,#31074,
#31075,#31076,#31077,#31078,#31079,#31080,#31081,#31082,#31083,#31084,#31085,
#31086,#31087,#31088,#31089,#31090,#31091,#31092,#31093,#31094,#31095,#31096,
#31097,#31098,#31099,#31100,#31101,#31102,#31103,#31104,#31105,#31106,#31107,
#31108,#31109,#31110,#31111,#31112,#31113,#31114,#31115,#31116,#31117,#31118,
#31119,#31120,#31121,#31122,#31123,#31124,#31125,#31126,#31127,#31128,#31129,
#31130,#31131,#31132,#31133,#31134,#31135,#31136,#31137,#31138,#31139,#31140,
#31141,#31142,#31143,#31144,#31145,#31146,#31147,#31148,#31149,#31150,#31151,
#31152,#31153,#31154,#31155,#31156,#31157,#31158,#31159),(#31160,#31161,
#31162,#31163,#31164,#31165,#31166,#31167,#31168,#31169,#31170,#31171,#31172,
#31173,#31174,#31175,#31176,#31177,#31178,#31179,#31180,#31181,#31182,#31183,
#31184,#31185,#31186,#31187,#31188,#31189,#31190,#31191,#31192,#31193,#31194,
#31195,#31196,#31197,#31198,#31199,#31200,#31201,#31202,#31203,#31204,#31205,
#31206,#31207,#31208,#31209,#31210,#31211,#31212,#31213,#31214,#31215,#31216,
#31217,#31218,#31219,#31220,#31221,#31222,#31223,#31224,#31225,#31226,#31227,
#31228,#31229,#31230,#31231,#31232,#31233,#31234,#31235,#31236,#31237,#31238,
#31239,#31240,#31241,#31242,#31243,#31244,#31245,#31246,#31247,#31248,#31249,
#31250,#31251,#31252,#31253,#31254,#31255,#31256,#31257,#31258,#31259,#31260,
#31261,#31262,#31263,#31264,#31265,#31266,#31267,#31268,#31269,#31270,#31271,
#31272,#31273,#31274,#31275,#31276,#31277,#31278,#31279,#31280,#31281,#31282,
#31283,#31284,#31285,#31286,#31287,#31288,#31289,#31290,#31291,#31292,#31293,
#31294,#31295,#31296,#31297,#31298,#31299,#31300,#31301,#31302,#31303),
(#31304,#31305,#31306,#31307,#31308,#31309,#31310,#31311,#31312,#31313,
#31314,#31315,#31316,#31317,#31318,#31319,#31320,#31321,#31322,#31323,#31324,
#31325,#31326,#31327,#31328,#31329,#31330,#31331,#31332,#31333,#31334,#31335,
#31336,#31337,#31338,#31339,#31340,#31341,#31342,#31343,#31344,#31345,#31346,
#31347,#31348,#31349,#31350,#31351,#31352,#31353,#31354,#31355,#31356,#31357,
#31358,#31359,#31360,#31361,#31362,#31363,#31364,#31365,#31366,#31367,#31368,
#31369,#31370,#31371,#31372,#31373,#31374,#31375,#31376,#31377,#31378,#31379,
#31380,#31381,#31382,#31383,#31384,#31385,#31386,#31387,#31388,#31389,#31390,
#31391,#31392,#31393,#31394,#31395,#31396,#31397,#31398,#31399,#31400,#31401,
#31402,#31403,#31404,#31405,#31406,#31407,#31408,#31409,#31410,#31411,#31412,
#31413,#31414,#31415,#31416,#31417,#31418,#31419,#31420,#31421,#31422,#31423,
#31424,#31425,#31426,#31427,#31428,#31429,#31430,#31431,#31432,#31433,#31434,
#31435,#31436,#31437,#31438,#31439,#31440,#31441,#31442,#31443,#31444,#31445,
#31446,#31447),(#31448,#31449,#31450,#31451,#31452,#31453,#31454,#31455,
#31456,#31457,#31458,#31459,#31460,#31461,#31462,#31463,#31464,#31465,#31466,
#31467,#31468,#31469,#31470,#31471,#31472,#31473,#31474,#31475,#31476,#31477,
#31478,#31479,#31480,#31481,#31482,#31483,#31484,#31485,#31486,#31487,#31488,
#31489,#31490,#31491,#31492,#31493,#31494,#31495,#31496,#31497,#31498,#31499,
#31500,#31501,#31502,#31503,#31504,#31505,#31506,#31507,#31508,#31509,#31510,
#31511,#31512,#31513,#31514,#31515,#31516,#31517,#31518,#31519,#31520,#31521,
#31522,#31523,#31524,#31525,#31526,#31527,#31528,#31529,#31530,#31531,#31532,
#31533,#31534,#31535,#31536,#31537,#31538,#31539,#31540,#31541,#31542,#31543,
#31544,#31545,#31546,#31547,#31548,#31549,#31550,#31551,#31552,#31553,#31554,
#31555,#31556,#31557,#31558,#31559,#31560,#31561,#31562,#31563,#31564,#31565,
#31566,#31567,#31568,#31569,#31570,#31571,#31572,#31573,#31574,#31575,#31576,
#31577,#31578,#31579,#31580,#31581,#31582,#31583,#31584,#31585,#31586,#31587,
#31588,#31589,#31590,#31591),(#31592,#31593,#31594,#31595,#31596,#31597,
#31598,#31599,#31600,#31601,#31602,#31603,#31604,#31605,#31606,#31607,#31608,
#31609,#31610,#31611,#31612,#31613,#31614,#31615,#31616,#31617,#31618,#31619,
#31620,#31621,#31622,#31623,#31624,#31625,#31626,#31627,#31628,#31629,#31630,
#31631,#31632,#31633,#31634,#31635,#31636,#31637,#31638,#31639,#31640,#31641,
#31642,#31643,#31644,#31645,#31646,#31647,#31648,#31649,#31650,#31651,#31652,
#31653,#31654,#31655,#31656,#31657,#31658,#31659,#31660,#31661,#31662,#31663,
#31664,#31665,#31666,#31667,#31668,#31669,#31670,#31671,#31672,#31673,#31674,
#31675,#31676,#31677,#31678,#31679,#31680,#31681,#31682,#31683,#31684,#31685,
#31686,#31687,#31688,#31689,#31690,#31691,#31692,#31693,#31694,#31695,#31696,
#31697,#31698,#31699,#31700,#31701,#31702,#31703,#31704,#31705,#31706,#31707,
#31708,#31709,#31710,#31711,#31712,#31713,#31714,#31715,#31716,#31717,#31718,
#31719,#31720,#31721,#31722,#31723,#31724,#31725,#31726,#31727,#31728,#31729,
#31730,#31731,#31732,#31733,#31734,#31735),(#31736,#31737,#31738,#31739,
#31740,#31741,#31742,#31743,#31744,#31745,#31746,#31747,#31748,#31749,#31750,
#31751,#31752,#31753,#31754,#31755,#31756,#31757,#31758,#31759,#31760,#31761,
#31762,#31763,#31764,#31765,#31766,#31767,#31768,#31769,#31770,#31771,#31772,
#31773,#31774,#31775,#31776,#31777,#31778,#31779,#31780,#31781,#31782,#31783,
#31784,#31785,#31786,#31787,#31788,#31789,#31790,#31791,#31792,#31793,#31794,
#31795,#31796,#31797,#31798,#31799,#31800,#31801,#31802,#31803,#31804,#31805,
#31806,#31807,#31808,#31809,#31810,#31811,#31812,#31813,#31814,#31815,#31816,
#31817,#31818,#31819,#31820,#31821,#31822,#31823,#31824,#31825,#31826,#31827,
#31828,#31829,#31830,#31831,#31832,#31833,#31834,#31835,#31836,#31837,#31838,
#31839,#31840,#31841,#31842,#31843,#31844,#31845,#31846,#31847,#31848,#31849,
#31850,#31851,#31852,#31853,#31854,#31855,#31856,#31857,#31858,#31859,#31860,
#31861,#31862,#31863,#31864,#31865,#31866,#31867,#31868,#31869,#31870,#31871,
#31872,#31873,#31874,#31875,#31876,#31877,#31878,#31879),(#31880,#31881,
#31882,#31883,#31884,#31885,#31886,#31887,#31888,#31889,#31890,#31891,#31892,
#31893,#31894,#31895,#31896,#31897,#31898,#31899,#31900,#31901,#31902,#31903,
#31904,#31905,#31906,#31907,#31908,#31909,#31910,#31911,#31912,#31913,#31914,
#31915,#31916,#31917,#31918,#31919,#31920,#31921,#31922,#31923,#31924,#31925,
#31926,#31927,#31928,#31929,#31930,#31931,#31932,#31933,#31934,#31935,#31936,
#31937,#31938,#31939,#31940,#31941,#31942,#31943,#31944,#31945,#31946,#31947,
#31948,#31949,#31950,#31951,#31952,#31953,#31954,#31955,#31956,#31957,#31958,
#31959,#31960,#31961,#31962,#31963,#31964,#31965,#31966,#31967,#31968,#31969,
#31970,#31971,#31972,#31973,#31974,#31975,#31976,#31977,#31978,#31979,#31980,
#31981,#31982,#31983,#31984,#31985,#31986,#31987,#31988,#31989,#31990,#31991,
#31992,#31993,#31994,#31995,#31996,#31997,#31998,#31999,#32000,#32001,#32002,
#32003,#32004,#32005,#32006,#32007,#32008,#32009,#32010,#32011,#32012,#32013,
#32014,#32015,#32016,#32017,#32018,#32019,#32020,#32021,#32022,#32023),
(#32024,#32025,#32026,#32027,#32028,#32029,#32030,#32031,#32032,#32033,
#32034,#32035,#32036,#32037,#32038,#32039,#32040,#32041,#32042,#32043,#32044,
#32045,#32046,#32047,#32048,#32049,#32050,#32051,#32052,#32053,#32054,#32055,
#32056,#32057,#32058,#32059,#32060,#32061,#32062,#32063,#32064,#32065,#32066,
#32067,#32068,#32069,#32070,#32071,#32072,#32073,#32074,#32075,#32076,#32077,
#32078,#32079,#32080,#32081,#32082,#32083,#32084,#32085,#32086,#32087,#32088,
#32089,#32090,#32091,#32092,#32093,#32094,#32095,#32096,#32097,#32098,#32099,
#32100,#32101,#32102,#32103,#32104,#32105,#32106,#32107,#32108,#32109,#32110,
#32111,#32112,#32113,#32114,#32115,#32116,#32117,#32118,#32119,#32120,#32121,
#32122,#32123,#32124,#32125,#32126,#32127,#32128,#32129,#32130,#32131,#32132,
#32133,#32134,#32135,#32136,#32137,#32138,#32139,#32140,#32141,#32142,#32143,
#32144,#32145,#32146,#32147,#32148,#32149,#32150,#32151,#32152,#32153,#32154,
#32155,#32156,#32157,#32158,#32159,#32160,#32161,#32162,#32163,#32164,#32165,
#32166,#32167),(#32168,#32169,#32170,#32171,#32172,#32173,#32174,#32175,
#32176,#32177,#32178,#32179,#32180,#32181,#32182,#32183,#32184,#32185,#32186,
#32187,#32188,#32189,#32190,#32191,#32192,#32193,#32194,#32195,#32196,#32197,
#32198,#32199,#32200,#32201,#32202,#32203,#32204,#32205,#32206,#32207,#32208,
#32209,#32210,#32211,#32212,#32213,#32214,#32215,#32216,#32217,#32218,#32219,
#32220,#32221,#32222,#32223,#32224,#32225,#32226,#32227,#32228,#32229,#32230,
#32231,#32232,#32233,#32234,#32235,#32236,#32237,#32238,#32239,#32240,#32241,
#32242,#32243,#32244,#32245,#32246,#32247,#32248,#32249,#32250,#32251,#32252,
#32253,#32254,#32255,#32256,#32257,#32258,#32259,#32260,#32261,#32262,#32263,
#32264,#32265,#32266,#32267,#32268,#32269,#32270,#32271,#32272,#32273,#32274,
#32275,#32276,#32277,#32278,#32279,#32280,#32281,#32282,#32283,#32284,#32285,
#32286,#32287,#32288,#32289,#32290,#32291,#32292,#32293,#32294,#32295,#32296,
#32297,#32298,#32299,#32300,#32301,#32302,#32303,#32304,#32305,#32306,#32307,
#32308,#32309,#32310,#32311),(#32312,#32313,#32314,#32315,#32316,#32317,
#32318,#32319,#32320,#32321,#32322,#32323,#32324,#32325,#32326,#32327,#32328,
#32329,#32330,#32331,#32332,#32333,#32334,#32335,#32336,#32337,#32338,#32339,
#32340,#32341,#32342,#32343,#32344,#32345,#32346,#32347,#32348,#32349,#32350,
#32351,#32352,#32353,#32354,#32355,#32356,#32357,#32358,#32359,#32360,#32361,
#32362,#32363,#32364,#32365,#32366,#32367,#32368,#32369,#32370,#32371,#32372,
#32373,#32374,#32375,#32376,#32377,#32378,#32379,#32380,#32381,#32382,#32383,
#32384,#32385,#32386,#32387,#32388,#32389,#32390,#32391,#32392,#32393,#32394,
#32395,#32396,#32397,#32398,#32399,#32400,#32401,#32402,#32403,#32404,#32405,
#32406,#32407,#32408,#32409,#32410,#32411,#32412,#32413,#32414,#32415,#32416,
#32417,#32418,#32419,#32420,#32421,#32422,#32423,#32424,#32425,#32426,#32427,
#32428,#32429,#32430,#32431,#32432,#32433,#32434,#32435,#32436,#32437,#32438,
#32439,#32440,#32441,#32442,#32443,#32444,#32445,#32446,#32447,#32448,#32449,
#32450,#32451,#32452,#32453,#32454,#32455),(#32456,#32457,#32458,#32459,
#32460,#32461,#32462,#32463,#32464,#32465,#32466,#32467,#32468,#32469,#32470,
#32471,#32472,#32473,#32474,#32475,#32476,#32477,#32478,#32479,#32480,#32481,
#32482,#32483,#32484,#32485,#32486,#32487,#32488,#32489,#32490,#32491,#32492,
#32493,#32494,#32495,#32496,#32497,#32498,#32499,#32500,#32501,#32502,#32503,
#32504,#32505,#32506,#32507,#32508,#32509,#32510,#32511,#32512,#32513,#32514,
#32515,#32516,#32517,#32518,#32519,#32520,#32521,#32522,#32523,#32524,#32525,
#32526,#32527,#32528,#32529,#32530,#32531,#32532,#32533,#32534,#32535,#32536,
#32537,#32538,#32539,#32540,#32541,#32542,#32543,#32544,#32545,#32546,#32547,
#32548,#32549,#32550,#32551,#32552,#32553,#32554,#32555,#32556,#32557,#32558,
#32559,#32560,#32561,#32562,#32563,#32564,#32565,#32566,#32567,#32568,#32569,
#32570,#32571,#32572,#32573,#32574,#32575,#32576,#32577,#32578,#32579,#32580,
#32581,#32582,#32583,#32584,#32585,#32586,#32587,#32588,#32589,#32590,#32591,
#32592,#32593,#32594,#32595,#32596,#32597,#32598,#32599),(#32600,#32601,
#32602,#32603,#32604,#32605,#32606,#32607,#32608,#32609,#32610,#32611,#32612,
#32613,#32614,#32615,#32616,#32617,#32618,#32619,#32620,#32621,#32622,#32623,
#32624,#32625,#32626,#32627,#32628,#32629,#32630,#32631,#32632,#32633,#32634,
#32635,#32636,#32637,#32638,#32639,#32640,#32641,#32642,#32643,#32644,#32645,
#32646,#32647,#32648,#32649,#32650,#32651,#32652,#32653,#32654,#32655,#32656,
#32657,#32658,#32659,#32660,#32661,#32662,#32663,#32664,#32665,#32666,#32667,
#32668,#32669,#32670,#32671,#32672,#32673,#32674,#32675,#32676,#32677,#32678,
#32679,#32680,#32681,#32682,#32683,#32684,#32685,#32686,#32687,#32688,#32689,
#32690,#32691,#32692,#32693,#32694,#32695,#32696,#32697,#32698,#32699,#32700,
#32701,#32702,#32703,#32704,#32705,#32706,#32707,#32708,#32709,#32710,#32711,
#32712,#32713,#32714,#32715,#32716,#32717,#32718,#32719,#32720,#32721,#32722,
#32723,#32724,#32725,#32726,#32727,#32728,#32729,#32730,#32731,#32732,#32733,
#32734,#32735,#32736,#32737,#32738,#32739,#32740,#32741,#32742,#32743),
(#32744,#32745,#32746,#32747,#32748,#32749,#32750,#32751,#32752,#32753,
#32754,#32755,#32756,#32757,#32758,#32759,#32760,#32761,#32762,#32763,#32764,
#32765,#32766,#32767,#32768,#32769,#32770,#32771,#32772,#32773,#32774,#32775,
#32776,#32777,#32778,#32779,#32780,#32781,#32782,#32783,#32784,#32785,#32786,
#32787,#32788,#32789,#32790,#32791,#32792,#32793,#32794,#32795,#32796,#32797,
#32798,#32799,#32800,#32801,#32802,#32803,#32804,#32805,#32806,#32807,#32808,
#32809,#32810,#32811,#32812,#32813,#32814,#32815,#32816,#32817,#32818,#32819,
#32820,#32821,#32822,#32823,#32824,#32825,#32826,#32827,#32828,#32829,#32830,
#32831,#32832,#32833,#32834,#32835,#32836,#32837,#32838,#32839,#32840,#32841,
#32842,#32843,#32844,#32845,#32846,#32847,#32848,#32849,#32850,#32851,#32852,
#32853,#32854,#32855,#32856,#32857,#32858,#32859,#32860,#32861,#32862,#32863,
#32864,#32865,#32866,#32867,#32868,#32869,#32870,#32871,#32872,#32873,#32874,
#32875,#32876,#32877,#32878,#32879,#32880,#32881,#32882,#32883,#32884,#32885,
#32886,#32887),(#32888,#32889,#32890,#32891,#32892,#32893,#32894,#32895,
#32896,#32897,#32898,#32899,#32900,#32901,#32902,#32903,#32904,#32905,#32906,
#32907,#32908,#32909,#32910,#32911,#32912,#32913,#32914,#32915,#32916,#32917,
#32918,#32919,#32920,#32921,#32922,#32923,#32924,#32925,#32926,#32927,#32928,
#32929,#32930,#32931,#32932,#32933,#32934,#32935,#32936,#32937,#32938,#32939,
#32940,#32941,#32942,#32943,#32944,#32945,#32946,#32947,#32948,#32949,#32950,
#32951,#32952,#32953,#32954,#32955,#32956,#32957,#32958,#32959,#32960,#32961,
#32962,#32963,#32964,#32965,#32966,#32967,#32968,#32969,#32970,#32971,#32972,
#32973,#32974,#32975,#32976,#32977,#32978,#32979,#32980,#32981,#32982,#32983,
#32984,#32985,#32986,#32987,#32988,#32989,#32990,#32991,#32992,#32993,#32994,
#32995,#32996,#32997,#32998,#32999,#33000,#33001,#33002,#33003,#33004,#33005,
#33006,#33007,#33008,#33009,#33010,#33011,#33012,#33013,#33014,#33015,#33016,
#33017,#33018,#33019,#33020,#33021,#33022,#33023,#33024,#33025,#33026,#33027,
#33028,#33029,#33030,#33031),(#33032,#33033,#33034,#33035,#33036,#33037,
#33038,#33039,#33040,#33041,#33042,#33043,#33044,#33045,#33046,#33047,#33048,
#33049,#33050,#33051,#33052,#33053,#33054,#33055,#33056,#33057,#33058,#33059,
#33060,#33061,#33062,#33063,#33064,#33065,#33066,#33067,#33068,#33069,#33070,
#33071,#33072,#33073,#33074,#33075,#33076,#33077,#33078,#33079,#33080,#33081,
#33082,#33083,#33084,#33085,#33086,#33087,#33088,#33089,#33090,#33091,#33092,
#33093,#33094,#33095,#33096,#33097,#33098,#33099,#33100,#33101,#33102,#33103,
#33104,#33105,#33106,#33107,#33108,#33109,#33110,#33111,#33112,#33113,#33114,
#33115,#33116,#33117,#33118,#33119,#33120,#33121,#33122,#33123,#33124,#33125,
#33126,#33127,#33128,#33129,#33130,#33131,#33132,#33133,#33134,#33135,#33136,
#33137,#33138,#33139,#33140,#33141,#33142,#33143,#33144,#33145,#33146,#33147,
#33148,#33149,#33150,#33151,#33152,#33153,#33154,#33155,#33156,#33157,#33158,
#33159,#33160,#33161,#33162,#33163,#33164,#33165,#33166,#33167,#33168,#33169,
#33170,#33171,#33172,#33173,#33174,#33175),(#33176,#33177,#33178,#33179,
#33180,#33181,#33182,#33183,#33184,#33185,#33186,#33187,#33188,#33189,#33190,
#33191,#33192,#33193,#33194,#33195,#33196,#33197,#33198,#33199,#33200,#33201,
#33202,#33203,#33204,#33205,#33206,#33207,#33208,#33209,#33210,#33211,#33212,
#33213,#33214,#33215,#33216,#33217,#33218,#33219,#33220,#33221,#33222,#33223,
#33224,#33225,#33226,#33227,#33228,#33229,#33230,#33231,#33232,#33233,#33234,
#33235,#33236,#33237,#33238,#33239,#33240,#33241,#33242,#33243,#33244,#33245,
#33246,#33247,#33248,#33249,#33250,#33251,#33252,#33253,#33254,#33255,#33256,
#33257,#33258,#33259,#33260,#33261,#33262,#33263,#33264,#33265,#33266,#33267,
#33268,#33269,#33270,#33271,#33272,#33273,#33274,#33275,#33276,#33277,#33278,
#33279,#33280,#33281,#33282,#33283,#33284,#33285,#33286,#33287,#33288,#33289,
#33290,#33291,#33292,#33293,#33294,#33295,#33296,#33297,#33298,#33299,#33300,
#33301,#33302,#33303,#33304,#33305,#33306,#33307,#33308,#33309,#33310,#33311,
#33312,#33313,#33314,#33315,#33316,#33317,#33318,#33319),(#33320,#33321,
#33322,#33323,#33324,#33325,#33326,#33327,#33328,#33329,#33330,#33331,#33332,
#33333,#33334,#33335,#33336,#33337,#33338,#33339,#33340,#33341,#33342,#33343,
#33344,#33345,#33346,#33347,#33348,#33349,#33350,#33351,#33352,#33353,#33354,
#33355,#33356,#33357,#33358,#33359,#33360,#33361,#33362,#33363,#33364,#33365,
#33366,#33367,#33368,#33369,#33370,#33371,#33372,#33373,#33374,#33375,#33376,
#33377,#33378,#33379,#33380,#33381,#33382,#33383,#33384,#33385,#33386,#33387,
#33388,#33389,#33390,#33391,#33392,#33393,#33394,#33395,#33396,#33397,#33398,
#33399,#33400,#33401,#33402,#33403,#33404,#33405,#33406,#33407,#33408,#33409,
#33410,#33411,#33412,#33413,#33414,#33415,#33416,#33417,#33418,#33419,#33420,
#33421,#33422,#33423,#33424,#33425,#33426,#33427,#33428,#33429,#33430,#33431,
#33432,#33433,#33434,#33435,#33436,#33437,#33438,#33439,#33440,#33441,#33442,
#33443,#33444,#33445,#33446,#33447,#33448,#33449,#33450,#33451,#33452,#33453,
#33454,#33455,#33456,#33457,#33458,#33459,#33460,#33461,#33462,#33463),
(#33464,#33465,#33466,#33467,#33468,#33469,#33470,#33471,#33472,#33473,
#33474,#33475,#33476,#33477,#33478,#33479,#33480,#33481,#33482,#33483,#33484,
#33485,#33486,#33487,#33488,#33489,#33490,#33491,#33492,#33493,#33494,#33495,
#33496,#33497,#33498,#33499,#33500,#33501,#33502,#33503,#33504,#33505,#33506,
#33507,#33508,#33509,#33510,#33511,#33512,#33513,#33514,#33515,#33516,#33517,
#33518,#33519,#33520,#33521,#33522,#33523,#33524,#33525,#33526,#33527,#33528,
#33529,#33530,#33531,#33532,#33533,#33534,#33535,#33536,#33537,#33538,#33539,
#33540,#33541,#33542,#33543,#33544,#33545,#33546,#33547,#33548,#33549,#33550,
#33551,#33552,#33553,#33554,#33555,#33556,#33557,#33558,#33559,#33560,#33561,
#33562,#33563,#33564,#33565,#33566,#33567,#33568,#33569,#33570,#33571,#33572,
#33573,#33574,#33575,#33576,#33577,#33578,#33579,#33580,#33581,#33582,#33583,
#33584,#33585,#33586,#33587,#33588,#33589,#33590,#33591,#33592,#33593,#33594,
#33595,#33596,#33597,#33598,#33599,#33600,#33601,#33602,#33603,#33604,#33605,
#33606,#33607),(#33608,#33609,#33610,#33611,#33612,#33613,#33614,#33615,
#33616,#33617,#33618,#33619,#33620,#33621,#33622,#33623,#33624,#33625,#33626,
#33627,#33628,#33629,#33630,#33631,#33632,#33633,#33634,#33635,#33636,#33637,
#33638,#33639,#33640,#33641,#33642,#33643,#33644,#33645,#33646,#33647,#33648,
#33649,#33650,#33651,#33652,#33653,#33654,#33655,#33656,#33657,#33658,#33659,
#33660,#33661,#33662,#33663,#33664,#33665,#33666,#33667,#33668,#33669,#33670,
#33671,#33672,#33673,#33674,#33675,#33676,#33677,#33678,#33679,#33680,#33681,
#33682,#33683,#33684,#33685,#33686,#33687,#33688,#33689,#33690,#33691,#33692,
#33693,#33694,#33695,#33696,#33697,#33698,#33699,#33700,#33701,#33702,#33703,
#33704,#33705,#33706,#33707,#33708,#33709,#33710,#33711,#33712,#33713,#33714,
#33715,#33716,#33717,#33718,#33719,#33720,#33721,#33722,#33723,#33724,#33725,
#33726,#33727,#33728,#33729,#33730,#33731,#33732,#33733,#33734,#33735,#33736,
#33737,#33738,#33739,#33740,#33741,#33742,#33743,#33744,#33745,#33746,#33747,
#33748,#33749,#33750,#33751),(#33752,#33753,#33754,#33755,#33756,#33757,
#33758,#33759,#33760,#33761,#33762,#33763,#33764,#33765,#33766,#33767,#33768,
#33769,#33770,#33771,#33772,#33773,#33774,#33775,#33776,#33777,#33778,#33779,
#33780,#33781,#33782,#33783,#33784,#33785,#33786,#33787,#33788,#33789,#33790,
#33791,#33792,#33793,#33794,#33795,#33796,#33797,#33798,#33799,#33800,#33801,
#33802,#33803,#33804,#33805,#33806,#33807,#33808,#33809,#33810,#33811,#33812,
#33813,#33814,#33815,#33816,#33817,#33818,#33819,#33820,#33821,#33822,#33823,
#33824,#33825,#33826,#33827,#33828,#33829,#33830,#33831,#33832,#33833,#33834,
#33835,#33836,#33837,#33838,#33839,#33840,#33841,#33842,#33843,#33844,#33845,
#33846,#33847,#33848,#33849,#33850,#33851,#33852,#33853,#33854,#33855,#33856,
#33857,#33858,#33859,#33860,#33861,#33862,#33863,#33864,#33865,#33866,#33867,
#33868,#33869,#33870,#33871,#33872,#33873,#33874,#33875,#33876,#33877,#33878,
#33879,#33880,#33881,#33882,#33883,#33884,#33885,#33886,#33887,#33888,#33889,
#33890,#33891,#33892,#33893,#33894,#33895),(#33896,#33897,#33898,#33899,
#33900,#33901,#33902,#33903,#33904,#33905,#33906,#33907,#33908,#33909,#33910,
#33911,#33912,#33913,#33914,#33915,#33916,#33917,#33918,#33919,#33920,#33921,
#33922,#33923,#33924,#33925,#33926,#33927,#33928,#33929,#33930,#33931,#33932,
#33933,#33934,#33935,#33936,#33937,#33938,#33939,#33940,#33941,#33942,#33943,
#33944,#33945,#33946,#33947,#33948,#33949,#33950,#33951,#33952,#33953,#33954,
#33955,#33956,#33957,#33958,#33959,#33960,#33961,#33962,#33963,#33964,#33965,
#33966,#33967,#33968,#33969,#33970,#33971,#33972,#33973,#33974,#33975,#33976,
#33977,#33978,#33979,#33980,#33981,#33982,#33983,#33984,#33985,#33986,#33987,
#33988,#33989,#33990,#33991,#33992,#33993,#33994,#33995,#33996,#33997,#33998,
#33999,#34000,#34001,#34002,#34003,#34004,#34005,#34006,#34007,#34008,#34009,
#34010,#34011,#34012,#34013,#34014,#34015,#34016,#34017,#34018,#34019,#34020,
#34021,#34022,#34023,#34024,#34025,#34026,#34027,#34028,#34029,#34030,#34031,
#34032,#34033,#34034,#34035,#34036,#34037,#34038,#34039),(#34040,#34041,
#34042,#34043,#34044,#34045,#34046,#34047,#34048,#34049,#34050,#34051,#34052,
#34053,#34054,#34055,#34056,#34057,#34058,#34059,#34060,#34061,#34062,#34063,
#34064,#34065,#34066,#34067,#34068,#34069,#34070,#34071,#34072,#34073,#34074,
#34075,#34076,#34077,#34078,#34079,#34080,#34081,#34082,#34083,#34084,#34085,
#34086,#34087,#34088,#34089,#34090,#34091,#34092,#34093,#34094,#34095,#34096,
#34097,#34098,#34099,#34100,#34101,#34102,#34103,#34104,#34105,#34106,#34107,
#34108,#34109,#34110,#34111,#34112,#34113,#34114,#34115,#34116,#34117,#34118,
#34119,#34120,#34121,#34122,#34123,#34124,#34125,#34126,#34127,#34128,#34129,
#34130,#34131,#34132,#34133,#34134,#34135,#34136,#34137,#34138,#34139,#34140,
#34141,#34142,#34143,#34144,#34145,#34146,#34147,#34148,#34149,#34150,#34151,
#34152,#34153,#34154,#34155,#34156,#34157,#34158,#34159,#34160,#34161,#34162,
#34163,#34164,#34165,#34166,#34167,#34168,#34169,#34170,#34171,#34172,#34173,
#34174,#34175,#34176,#34177,#34178,#34179,#34180,#34181,#34182,#34183),
(#34184,#34185,#34186,#34187,#34188,#34189,#34190,#34191,#34192,#34193,
#34194,#34195,#34196,#34197,#34198,#34199,#34200,#34201,#34202,#34203,#34204,
#34205,#34206,#34207,#34208,#34209,#34210,#34211,#34212,#34213,#34214,#34215,
#34216,#34217,#34218,#34219,#34220,#34221,#34222,#34223,#34224,#34225,#34226,
#34227,#34228,#34229,#34230,#34231,#34232,#34233,#34234,#34235,#34236,#34237,
#34238,#34239,#34240,#34241,#34242,#34243,#34244,#34245,#34246,#34247,#34248,
#34249,#34250,#34251,#34252,#34253,#34254,#34255,#34256,#34257,#34258,#34259,
#34260,#34261,#34262,#34263,#34264,#34265,#34266,#34267,#34268,#34269,#34270,
#34271,#34272,#34273,#34274,#34275,#34276,#34277,#34278,#34279,#34280,#34281,
#34282,#34283,#34284,#34285,#34286,#34287,#34288,#34289,#34290,#34291,#34292,
#34293,#34294,#34295,#34296,#34297,#34298,#34299,#34300,#34301,#34302,#34303,
#34304,#34305,#34306,#34307,#34308,#34309,#34310,#34311,#34312,#34313,#34314,
#34315,#34316,#34317,#34318,#34319,#34320,#34321,#34322,#34323,#34324,#34325,
#34326,#34327),(#34328,#34329,#34330,#34331,#34332,#34333,#34334,#34335,
#34336,#34337,#34338,#34339,#34340,#34341,#34342,#34343,#34344,#34345,#34346,
#34347,#34348,#34349,#34350,#34351,#34352,#34353,#34354,#34355,#34356,#34357,
#34358,#34359,#34360,#34361,#34362,#34363,#34364,#34365,#34366,#34367,#34368,
#34369,#34370,#34371,#34372,#34373,#34374,#34375,#34376,#34377,#34378,#34379,
#34380,#34381,#34382,#34383,#34384,#34385,#34386,#34387,#34388,#34389,#34390,
#34391,#34392,#34393,#34394,#34395,#34396,#34397,#34398,#34399,#34400,#34401,
#34402,#34403,#34404,#34405,#34406,#34407,#34408,#34409,#34410,#34411,#34412,
#34413,#34414,#34415,#34416,#34417,#34418,#34419,#34420,#34421,#34422,#34423,
#34424,#34425,#34426,#34427,#34428,#34429,#34430,#34431,#34432,#34433,#34434,
#34435,#34436,#34437,#34438,#34439,#34440,#34441,#34442,#34443,#34444,#34445,
#34446,#34447,#34448,#34449,#34450,#34451,#34452,#34453,#34454,#34455,#34456,
#34457,#34458,#34459,#34460,#34461,#34462,#34463,#34464,#34465,#34466,#34467,
#34468,#34469,#34470,#34471),(#34472,#34473,#34474,#34475,#34476,#34477,
#34478,#34479,#34480,#34481,#34482,#34483,#34484,#34485,#34486,#34487,#34488,
#34489,#34490,#34491,#34492,#34493,#34494,#34495,#34496,#34497,#34498,#34499,
#34500,#34501,#34502,#34503,#34504,#34505,#34506,#34507,#34508,#34509,#34510,
#34511,#34512,#34513,#34514,#34515,#34516,#34517,#34518,#34519,#34520,#34521,
#34522,#34523,#34524,#34525,#34526,#34527,#34528,#34529,#34530,#34531,#34532,
#34533,#34534,#34535,#34536,#34537,#34538,#34539,#34540,#34541,#34542,#34543,
#34544,#34545,#34546,#34547,#34548,#34549,#34550,#34551,#34552,#34553,#34554,
#34555,#34556,#34557,#34558,#34559,#34560,#34561,#34562,#34563,#34564,#34565,
#34566,#34567,#34568,#34569,#34570,#34571,#34572,#34573,#34574,#34575,#34576,
#34577,#34578,#34579,#34580,#34581,#34582,#34583,#34584,#34585,#34586,#34587,
#34588,#34589,#34590,#34591,#34592,#34593,#34594,#34595,#34596,#34597,#34598,
#34599,#34600,#34601,#34602,#34603,#34604,#34605,#34606,#34607,#34608,#34609,
#34610,#34611,#34612,#34613,#34614,#34615),(#34616,#34617,#34618,#34619,
#34620,#34621,#34622,#34623,#34624,#34625,#34626,#34627,#34628,#34629,#34630,
#34631,#34632,#34633,#34634,#34635,#34636,#34637,#34638,#34639,#34640,#34641,
#34642,#34643,#34644,#34645,#34646,#34647,#34648,#34649,#34650,#34651,#34652,
#34653,#34654,#34655,#34656,#34657,#34658,#34659,#34660,#34661,#34662,#34663,
#34664,#34665,#34666,#34667,#34668,#34669,#34670,#34671,#34672,#34673,#34674,
#34675,#34676,#34677,#34678,#34679,#34680,#34681,#34682,#34683,#34684,#34685,
#34686,#34687,#34688,#34689,#34690,#34691,#34692,#34693,#34694,#34695,#34696,
#34697,#34698,#34699,#34700,#34701,#34702,#34703,#34704,#34705,#34706,#34707,
#34708,#34709,#34710,#34711,#34712,#34713,#34714,#34715,#34716,#34717,#34718,
#34719,#34720,#34721,#34722,#34723,#34724,#34725,#34726,#34727,#34728,#34729,
#34730,#34731,#34732,#34733,#34734,#34735,#34736,#34737,#34738,#34739,#34740,
#34741,#34742,#34743,#34744,#34745,#34746,#34747,#34748,#34749,#34750,#34751,
#34752,#34753,#34754,#34755,#34756,#34757,#34758,#34759),(#34760,#34761,
#34762,#34763,#34764,#34765,#34766,#34767,#34768,#34769,#34770,#34771,#34772,
#34773,#34774,#34775,#34776,#34777,#34778,#34779,#34780,#34781,#34782,#34783,
#34784,#34785,#34786,#34787,#34788,#34789,#34790,#34791,#34792,#34793,#34794,
#34795,#34796,#34797,#34798,#34799,#34800,#34801,#34802,#34803,#34804,#34805,
#34806,#34807,#34808,#34809,#34810,#34811,#34812,#34813,#34814,#34815,#34816,
#34817,#34818,#34819,#34820,#34821,#34822,#34823,#34824,#34825,#34826,#34827,
#34828,#34829,#34830,#34831,#34832,#34833,#34834,#34835,#34836,#34837,#34838,
#34839,#34840,#34841,#34842,#34843,#34844,#34845,#34846,#34847,#34848,#34849,
#34850,#34851,#34852,#34853,#34854,#34855,#34856,#34857,#34858,#34859,#34860,
#34861,#34862,#34863,#34864,#34865,#34866,#34867,#34868,#34869,#34870,#34871,
#34872,#34873,#34874,#34875,#34876,#34877,#34878,#34879,#34880,#34881,#34882,
#34883,#34884,#34885,#34886,#34887,#34888,#34889,#34890,#34891,#34892,#34893,
#34894,#34895,#34896,#34897,#34898,#34899,#34900,#34901,#34902,#34903),
(#34904,#34905,#34906,#34907,#34908,#34909,#34910,#34911,#34912,#34913,
#34914,#34915,#34916,#34917,#34918,#34919,#34920,#34921,#34922,#34923,#34924,
#34925,#34926,#34927,#34928,#34929,#34930,#34931,#34932,#34933,#34934,#34935,
#34936,#34937,#34938,#34939,#34940,#34941,#34942,#34943,#34944,#34945,#34946,
#34947,#34948,#34949,#34950,#34951,#34952,#34953,#34954,#34955,#34956,#34957,
#34958,#34959,#34960,#34961,#34962,#34963,#34964,#34965,#34966,#34967,#34968,
#34969,#34970,#34971,#34972,#34973,#34974,#34975,#34976,#34977,#34978,#34979,
#34980,#34981,#34982,#34983,#34984,#34985,#34986,#34987,#34988,#34989,#34990,
#34991,#34992,#34993,#34994,#34995,#34996,#34997,#34998,#34999,#35000,#35001,
#35002,#35003,#35004,#35005,#35006,#35007,#35008,#35009,#35010,#35011,#35012,
#35013,#35014,#35015,#35016,#35017,#35018,#35019,#35020,#35021,#35022,#35023,
#35024,#35025,#35026,#35027,#35028,#35029,#35030,#35031,#35032,#35033,#35034,
#35035,#35036,#35037,#35038,#35039,#35040,#35041,#35042,#35043,#35044,#35045,
#35046,#35047),(#35048,#35049,#35050,#35051,#35052,#35053,#35054,#35055,
#35056,#35057,#35058,#35059,#35060,#35061,#35062,#35063,#35064,#35065,#35066,
#35067,#35068,#35069,#35070,#35071,#35072,#35073,#35074,#35075,#35076,#35077,
#35078,#35079,#35080,#35081,#35082,#35083,#35084,#35085,#35086,#35087,#35088,
#35089,#35090,#35091,#35092,#35093,#35094,#35095,#35096,#35097,#35098,#35099,
#35100,#35101,#35102,#35103,#35104,#35105,#35106,#35107,#35108,#35109,#35110,
#35111,#35112,#35113,#35114,#35115,#35116,#35117,#35118,#35119,#35120,#35121,
#35122,#35123,#35124,#35125,#35126,#35127,#35128,#35129,#35130,#35131,#35132,
#35133,#35134,#35135,#35136,#35137,#35138,#35139,#35140,#35141,#35142,#35143,
#35144,#35145,#35146,#35147,#35148,#35149,#35150,#35151,#35152,#35153,#35154,
#35155,#35156,#35157,#35158,#35159,#35160,#35161,#35162,#35163,#35164,#35165,
#35166,#35167,#35168,#35169,#35170,#35171,#35172,#35173,#35174,#35175,#35176,
#35177,#35178,#35179,#35180,#35181,#35182,#35183,#35184,#35185,#35186,#35187,
#35188,#35189,#35190,#35191),(#35192,#35193,#35194,#35195,#35196,#35197,
#35198,#35199,#35200,#35201,#35202,#35203,#35204,#35205,#35206,#35207,#35208,
#35209,#35210,#35211,#35212,#35213,#35214,#35215,#35216,#35217,#35218,#35219,
#35220,#35221,#35222,#35223,#35224,#35225,#35226,#35227,#35228,#35229,#35230,
#35231,#35232,#35233,#35234,#35235,#35236,#35237,#35238,#35239,#35240,#35241,
#35242,#35243,#35244,#35245,#35246,#35247,#35248,#35249,#35250,#35251,#35252,
#35253,#35254,#35255,#35256,#35257,#35258,#35259,#35260,#35261,#35262,#35263,
#35264,#35265,#35266,#35267,#35268,#35269,#35270,#35271,#35272,#35273,#35274,
#35275,#35276,#35277,#35278,#35279,#35280,#35281,#35282,#35283,#35284,#35285,
#35286,#35287,#35288,#35289,#35290,#35291,#35292,#35293,#35294,#35295,#35296,
#35297,#35298,#35299,#35300,#35301,#35302,#35303,#35304,#35305,#35306,#35307,
#35308,#35309,#35310,#35311,#35312,#35313,#35314,#35315,#35316,#35317,#35318,
#35319,#35320,#35321,#35322,#35323,#35324,#35325,#35326,#35327,#35328,#35329,
#35330,#35331,#35332,#35333,#35334,#35335),(#35336,#35337,#35338,#35339,
#35340,#35341,#35342,#35343,#35344,#35345,#35346,#35347,#35348,#35349,#35350,
#35351,#35352,#35353,#35354,#35355,#35356,#35357,#35358,#35359,#35360,#35361,
#35362,#35363,#35364,#35365,#35366,#35367,#35368,#35369,#35370,#35371,#35372,
#35373,#35374,#35375,#35376,#35377,#35378,#35379,#35380,#35381,#35382,#35383,
#35384,#35385,#35386,#35387,#35388,#35389,#35390,#35391,#35392,#35393,#35394,
#35395,#35396,#35397,#35398,#35399,#35400,#35401,#35402,#35403,#35404,#35405,
#35406,#35407,#35408,#35409,#35410,#35411,#35412,#35413,#35414,#35415,#35416,
#35417,#35418,#35419,#35420,#35421,#35422,#35423,#35424,#35425,#35426,#35427,
#35428,#35429,#35430,#35431,#35432,#35433,#35434,#35435,#35436,#35437,#35438,
#35439,#35440,#35441,#35442,#35443,#35444,#35445,#35446,#35447,#35448,#35449,
#35450,#35451,#35452,#35453,#35454,#35455,#35456,#35457,#35458,#35459,#35460,
#35461,#35462,#35463,#35464,#35465,#35466,#35467,#35468,#35469,#35470,#35471,
#35472,#35473,#35474,#35475,#35476,#35477,#35478,#35479),(#35480,#35481,
#35482,#35483,#35484,#35485,#35486,#35487,#35488,#35489,#35490,#35491,#35492,
#35493,#35494,#35495,#35496,#35497,#35498,#35499,#35500,#35501,#35502,#35503,
#35504,#35505,#35506,#35507,#35508,#35509,#35510,#35511,#35512,#35513,#35514,
#35515,#35516,#35517,#35518,#35519,#35520,#35521,#35522,#35523,#35524,#35525,
#35526,#35527,#35528,#35529,#35530,#35531,#35532,#35533,#35534,#35535,#35536,
#35537,#35538,#35539,#35540,#35541,#35542,#35543,#35544,#35545,#35546,#35547,
#35548,#35549,#35550,#35551,#35552,#35553,#35554,#35555,#35556,#35557,#35558,
#35559,#35560,#35561,#35562,#35563,#35564,#35565,#35566,#35567,#35568,#35569,
#35570,#35571,#35572,#35573,#35574,#35575,#35576,#35577,#35578,#35579,#35580,
#35581,#35582,#35583,#35584,#35585,#35586,#35587,#35588,#35589,#35590,#35591,
#35592,#35593,#35594,#35595,#35596,#35597,#35598,#35599,#35600,#35601,#35602,
#35603,#35604,#35605,#35606,#35607,#35608,#35609,#35610,#35611,#35612,#35613,
#35614,#35615,#35616,#35617,#35618,#35619,#35620,#35621,#35622,#35623),
(#35624,#35625,#35626,#35627,#35628,#35629,#35630,#35631,#35632,#35633,
#35634,#35635,#35636,#35637,#35638,#35639,#35640,#35641,#35642,#35643,#35644,
#35645,#35646,#35647,#35648,#35649,#35650,#35651,#35652,#35653,#35654,#35655,
#35656,#35657,#35658,#35659,#35660,#35661,#35662,#35663,#35664,#35665,#35666,
#35667,#35668,#35669,#35670,#35671,#35672,#35673,#35674,#35675,#35676,#35677,
#35678,#35679,#35680,#35681,#35682,#35683,#35684,#35685,#35686,#35687,#35688,
#35689,#35690,#35691,#35692,#35693,#35694,#35695,#35696,#35697,#35698,#35699,
#35700,#35701,#35702,#35703,#35704,#35705,#35706,#35707,#35708,#35709,#35710,
#35711,#35712,#35713,#35714,#35715,#35716,#35717,#35718,#35719,#35720,#35721,
#35722,#35723,#35724,#35725,#35726,#35727,#35728,#35729,#35730,#35731,#35732,
#35733,#35734,#35735,#35736,#35737,#35738,#35739,#35740,#35741,#35742,#35743,
#35744,#35745,#35746,#35747,#35748,#35749,#35750,#35751,#35752,#35753,#35754,
#35755,#35756,#35757,#35758,#35759,#35760,#35761,#35762,#35763,#35764,#35765,
#35766,#35767),(#35768,#35769,#35770,#35771,#35772,#35773,#35774,#35775,
#35776,#35777,#35778,#35779,#35780,#35781,#35782,#35783,#35784,#35785,#35786,
#35787,#35788,#35789,#35790,#35791,#35792,#35793,#35794,#35795,#35796,#35797,
#35798,#35799,#35800,#35801,#35802,#35803,#35804,#35805,#35806,#35807,#35808,
#35809,#35810,#35811,#35812,#35813,#35814,#35815,#35816,#35817,#35818,#35819,
#35820,#35821,#35822,#35823,#35824,#35825,#35826,#35827,#35828,#35829,#35830,
#35831,#35832,#35833,#35834,#35835,#35836,#35837,#35838,#35839,#35840,#35841,
#35842,#35843,#35844,#35845,#35846,#35847,#35848,#35849,#35850,#35851,#35852,
#35853,#35854,#35855,#35856,#35857,#35858,#35859,#35860,#35861,#35862,#35863,
#35864,#35865,#35866,#35867,#35868,#35869,#35870,#35871,#35872,#35873,#35874,
#35875,#35876,#35877,#35878,#35879,#35880,#35881,#35882,#35883,#35884,#35885,
#35886,#35887,#35888,#35889,#35890,#35891,#35892,#35893,#35894,#35895,#35896,
#35897,#35898,#35899,#35900,#35901,#35902,#35903,#35904,#35905,#35906,#35907,
#35908,#35909,#35910,#35911),(#35912,#35913,#35914,#35915,#35916,#35917,
#35918,#35919,#35920,#35921,#35922,#35923,#35924,#35925,#35926,#35927,#35928,
#35929,#35930,#35931,#35932,#35933,#35934,#35935,#35936,#35937,#35938,#35939,
#35940,#35941,#35942,#35943,#35944,#35945,#35946,#35947,#35948,#35949,#35950,
#35951,#35952,#35953,#35954,#35955,#35956,#35957,#35958,#35959,#35960,#35961,
#35962,#35963,#35964,#35965,#35966,#35967,#35968,#35969,#35970,#35971,#35972,
#35973,#35974,#35975,#35976,#35977,#35978,#35979,#35980,#35981,#35982,#35983,
#35984,#35985,#35986,#35987,#35988,#35989,#35990,#35991,#35992,#35993,#35994,
#35995,#35996,#35997,#35998,#35999,#36000,#36001,#36002,#36003,#36004,#36005,
#36006,#36007,#36008,#36009,#36010,#36011,#36012,#36013,#36014,#36015,#36016,
#36017,#36018,#36019,#36020,#36021,#36022,#36023,#36024,#36025,#36026,#36027,
#36028,#36029,#36030,#36031,#36032,#36033,#36034,#36035,#36036,#36037,#36038,
#36039,#36040,#36041,#36042,#36043,#36044,#36045,#36046,#36047,#36048,#36049,
#36050,#36051,#36052,#36053,#36054,#36055),(#36056,#36057,#36058,#36059,
#36060,#36061,#36062,#36063,#36064,#36065,#36066,#36067,#36068,#36069,#36070,
#36071,#36072,#36073,#36074,#36075,#36076,#36077,#36078,#36079,#36080,#36081,
#36082,#36083,#36084,#36085,#36086,#36087,#36088,#36089,#36090,#36091,#36092,
#36093,#36094,#36095,#36096,#36097,#36098,#36099,#36100,#36101,#36102,#36103,
#36104,#36105,#36106,#36107,#36108,#36109,#36110,#36111,#36112,#36113,#36114,
#36115,#36116,#36117,#36118,#36119,#36120,#36121,#36122,#36123,#36124,#36125,
#36126,#36127,#36128,#36129,#36130,#36131,#36132,#36133,#36134,#36135,#36136,
#36137,#36138,#36139,#36140,#36141,#36142,#36143,#36144,#36145,#36146,#36147,
#36148,#36149,#36150,#36151,#36152,#36153,#36154,#36155,#36156,#36157,#36158,
#36159,#36160,#36161,#36162,#36163,#36164,#36165,#36166,#36167,#36168,#36169,
#36170,#36171,#36172,#36173,#36174,#36175,#36176,#36177,#36178,#36179,#36180,
#36181,#36182,#36183,#36184,#36185,#36186,#36187,#36188,#36189,#36190,#36191,
#36192,#36193,#36194,#36195,#36196,#36197,#36198,#36199),(#36200,#36201,
#36202,#36203,#36204,#36205,#36206,#36207,#36208,#36209,#36210,#36211,#36212,
#36213,#36214,#36215,#36216,#36217,#36218,#36219,#36220,#36221,#36222,#36223,
#36224,#36225,#36226,#36227,#36228,#36229,#36230,#36231,#36232,#36233,#36234,
#36235,#36236,#36237,#36238,#36239,#36240,#36241,#36242,#36243,#36244,#36245,
#36246,#36247,#36248,#36249,#36250,#36251,#36252,#36253,#36254,#36255,#36256,
#36257,#36258,#36259,#36260,#36261,#36262,#36263,#36264,#36265,#36266,#36267,
#36268,#36269,#36270,#36271,#36272,#36273,#36274,#36275,#36276,#36277,#36278,
#36279,#36280,#36281,#36282,#36283,#36284,#36285,#36286,#36287,#36288,#36289,
#36290,#36291,#36292,#36293,#36294,#36295,#36296,#36297,#36298,#36299,#36300,
#36301,#36302,#36303,#36304,#36305,#36306,#36307,#36308,#36309,#36310,#36311,
#36312,#36313,#36314,#36315,#36316,#36317,#36318,#36319,#36320,#36321,#36322,
#36323,#36324,#36325,#36326,#36327,#36328,#36329,#36330,#36331,#36332,#36333,
#36334,#36335,#36336,#36337,#36338,#36339,#36340,#36341,#36342,#36343),
(#36344,#36345,#36346,#36347,#36348,#36349,#36350,#36351,#36352,#36353,
#36354,#36355,#36356,#36357,#36358,#36359,#36360,#36361,#36362,#36363,#36364,
#36365,#36366,#36367,#36368,#36369,#36370,#36371,#36372,#36373,#36374,#36375,
#36376,#36377,#36378,#36379,#36380,#36381,#36382,#36383,#36384,#36385,#36386,
#36387,#36388,#36389,#36390,#36391,#36392,#36393,#36394,#36395,#36396,#36397,
#36398,#36399,#36400,#36401,#36402,#36403,#36404,#36405,#36406,#36407,#36408,
#36409,#36410,#36411,#36412,#36413,#36414,#36415,#36416,#36417,#36418,#36419,
#36420,#36421,#36422,#36423,#36424,#36425,#36426,#36427,#36428,#36429,#36430,
#36431,#36432,#36433,#36434,#36435,#36436,#36437,#36438,#36439,#36440,#36441,
#36442,#36443,#36444,#36445,#36446,#36447,#36448,#36449,#36450,#36451,#36452,
#36453,#36454,#36455,#36456,#36457,#36458,#36459,#36460,#36461,#36462,#36463,
#36464,#36465,#36466,#36467,#36468,#36469,#36470,#36471,#36472,#36473,#36474,
#36475,#36476,#36477,#36478,#36479,#36480,#36481,#36482,#36483,#36484,#36485,
#36486,#36487),(#36488,#36489,#36490,#36491,#36492,#36493,#36494,#36495,
#36496,#36497,#36498,#36499,#36500,#36501,#36502,#36503,#36504,#36505,#36506,
#36507,#36508,#36509,#36510,#36511,#36512,#36513,#36514,#36515,#36516,#36517,
#36518,#36519,#36520,#36521,#36522,#36523,#36524,#36525,#36526,#36527,#36528,
#36529,#36530,#36531,#36532,#36533,#36534,#36535,#36536,#36537,#36538,#36539,
#36540,#36541,#36542,#36543,#36544,#36545,#36546,#36547,#36548,#36549,#36550,
#36551,#36552,#36553,#36554,#36555,#36556,#36557,#36558,#36559,#36560,#36561,
#36562,#36563,#36564,#36565,#36566,#36567,#36568,#36569,#36570,#36571,#36572,
#36573,#36574,#36575,#36576,#36577,#36578,#36579,#36580,#36581,#36582,#36583,
#36584,#36585,#36586,#36587,#36588,#36589,#36590,#36591,#36592,#36593,#36594,
#36595,#36596,#36597,#36598,#36599,#36600,#36601,#36602,#36603,#36604,#36605,
#36606,#36607,#36608,#36609,#36610,#36611,#36612,#36613,#36614,#36615,#36616,
#36617,#36618,#36619,#36620,#36621,#36622,#36623,#36624,#36625,#36626,#36627,
#36628,#36629,#36630,#36631),(#36632,#36633,#36634,#36635,#36636,#36637,
#36638,#36639,#36640,#36641,#36642,#36643,#36644,#36645,#36646,#36647,#36648,
#36649,#36650,#36651,#36652,#36653,#36654,#36655,#36656,#36657,#36658,#36659,
#36660,#36661,#36662,#36663,#36664,#36665,#36666,#36667,#36668,#36669,#36670,
#36671,#36672,#36673,#36674,#36675,#36676,#36677,#36678,#36679,#36680,#36681,
#36682,#36683,#36684,#36685,#36686,#36687,#36688,#36689,#36690,#36691,#36692,
#36693,#36694,#36695,#36696,#36697,#36698,#36699,#36700,#36701,#36702,#36703,
#36704,#36705,#36706,#36707,#36708,#36709,#36710,#36711,#36712,#36713,#36714,
#36715,#36716,#36717,#36718,#36719,#36720,#36721,#36722,#36723,#36724,#36725,
#36726,#36727,#36728,#36729,#36730,#36731,#36732,#36733,#36734,#36735,#36736,
#36737,#36738,#36739,#36740,#36741,#36742,#36743,#36744,#36745,#36746,#36747,
#36748,#36749,#36750,#36751,#36752,#36753,#36754,#36755,#36756,#36757,#36758,
#36759,#36760,#36761,#36762,#36763,#36764,#36765,#36766,#36767,#36768,#36769,
#36770,#36771,#36772,#36773,#36774,#36775),(#36776,#36777,#36778,#36779,
#36780,#36781,#36782,#36783,#36784,#36785,#36786,#36787,#36788,#36789,#36790,
#36791,#36792,#36793,#36794,#36795,#36796,#36797,#36798,#36799,#36800,#36801,
#36802,#36803,#36804,#36805,#36806,#36807,#36808,#36809,#36810,#36811,#36812,
#36813,#36814,#36815,#36816,#36817,#36818,#36819,#36820,#36821,#36822,#36823,
#36824,#36825,#36826,#36827,#36828,#36829,#36830,#36831,#36832,#36833,#36834,
#36835,#36836,#36837,#36838,#36839,#36840,#36841,#36842,#36843,#36844,#36845,
#36846,#36847,#36848,#36849,#36850,#36851,#36852,#36853,#36854,#36855,#36856,
#36857,#36858,#36859,#36860,#36861,#36862,#36863,#36864,#36865,#36866,#36867,
#36868,#36869,#36870,#36871,#36872,#36873,#36874,#36875,#36876,#36877,#36878,
#36879,#36880,#36881,#36882,#36883,#36884,#36885,#36886,#36887,#36888,#36889,
#36890,#36891,#36892,#36893,#36894,#36895,#36896,#36897,#36898,#36899,#36900,
#36901,#36902,#36903,#36904,#36905,#36906,#36907,#36908,#36909,#36910,#36911,
#36912,#36913,#36914,#36915,#36916,#36917,#36918,#36919),(#36920,#36921,
#36922,#36923,#36924,#36925,#36926,#36927,#36928,#36929,#36930,#36931,#36932,
#36933,#36934,#36935,#36936,#36937,#36938,#36939,#36940,#36941,#36942,#36943,
#36944,#36945,#36946,#36947,#36948,#36949,#36950,#36951,#36952,#36953,#36954,
#36955,#36956,#36957,#36958,#36959,#36960,#36961,#36962,#36963,#36964,#36965,
#36966,#36967,#36968,#36969,#36970,#36971,#36972,#36973,#36974,#36975,#36976,
#36977,#36978,#36979,#36980,#36981,#36982,#36983,#36984,#36985,#36986,#36987,
#36988,#36989,#36990,#36991,#36992,#36993,#36994,#36995,#36996,#36997,#36998,
#36999,#37000,#37001,#37002,#37003,#37004,#37005,#37006,#37007,#37008,#37009,
#37010,#37011,#37012,#37013,#37014,#37015,#37016,#37017,#37018,#37019,#37020,
#37021,#37022,#37023,#37024,#37025,#37026,#37027,#37028,#37029,#37030,#37031,
#37032,#37033,#37034,#37035,#37036,#37037,#37038,#37039,#37040,#37041,#37042,
#37043,#37044,#37045,#37046,#37047,#37048,#37049,#37050,#37051,#37052,#37053,
#37054,#37055,#37056,#37057,#37058,#37059,#37060,#37061,#37062,#37063),
(#37064,#37065,#37066,#37067,#37068,#37069,#37070,#37071,#37072,#37073,
#37074,#37075,#37076,#37077,#37078,#37079,#37080,#37081,#37082,#37083,#37084,
#37085,#37086,#37087,#37088,#37089,#37090,#37091,#37092,#37093,#37094,#37095,
#37096,#37097,#37098,#37099,#37100,#37101,#37102,#37103,#37104,#37105,#37106,
#37107,#37108,#37109,#37110,#37111,#37112,#37113,#37114,#37115,#37116,#37117,
#37118,#37119,#37120,#37121,#37122,#37123,#37124,#37125,#37126,#37127,#37128,
#37129,#37130,#37131,#37132,#37133,#37134,#37135,#37136,#37137,#37138,#37139,
#37140,#37141,#37142,#37143,#37144,#37145,#37146,#37147,#37148,#37149,#37150,
#37151,#37152,#37153,#37154,#37155,#37156,#37157,#37158,#37159,#37160,#37161,
#37162,#37163,#37164,#37165,#37166,#37167,#37168,#37169,#37170,#37171,#37172,
#37173,#37174,#37175,#37176,#37177,#37178,#37179,#37180,#37181,#37182,#37183,
#37184,#37185,#37186,#37187,#37188,#37189,#37190,#37191,#37192,#37193,#37194,
#37195,#37196,#37197,#37198,#37199,#37200,#37201,#37202,#37203,#37204,#37205,
#37206,#37207),(#37208,#37209,#37210,#37211,#37212,#37213,#37214,#37215,
#37216,#37217,#37218,#37219,#37220,#37221,#37222,#37223,#37224,#37225,#37226,
#37227,#37228,#37229,#37230,#37231,#37232,#37233,#37234,#37235,#37236,#37237,
#37238,#37239,#37240,#37241,#37242,#37243,#37244,#37245,#37246,#37247,#37248,
#37249,#37250,#37251,#37252,#37253,#37254,#37255,#37256,#37257,#37258,#37259,
#37260,#37261,#37262,#37263,#37264,#37265,#37266,#37267,#37268,#37269,#37270,
#37271,#37272,#37273,#37274,#37275,#37276,#37277,#37278,#37279,#37280,#37281,
#37282,#37283,#37284,#37285,#37286,#37287,#37288,#37289,#37290,#37291,#37292,
#37293,#37294,#37295,#37296,#37297,#37298,#37299,#37300,#37301,#37302,#37303,
#37304,#37305,#37306,#37307,#37308,#37309,#37310,#37311,#37312,#37313,#37314,
#37315,#37316,#37317,#37318,#37319,#37320,#37321,#37322,#37323,#37324,#37325,
#37326,#37327,#37328,#37329,#37330,#37331,#37332,#37333,#37334,#37335,#37336,
#37337,#37338,#37339,#37340,#37341,#37342,#37343,#37344,#37345,#37346,#37347,
#37348,#37349,#37350,#37351),(#37352,#37353,#37354,#37355,#37356,#37357,
#37358,#37359,#37360,#37361,#37362,#37363,#37364,#37365,#37366,#37367,#37368,
#37369,#37370,#37371,#37372,#37373,#37374,#37375,#37376,#37377,#37378,#37379,
#37380,#37381,#37382,#37383,#37384,#37385,#37386,#37387,#37388,#37389,#37390,
#37391,#37392,#37393,#37394,#37395,#37396,#37397,#37398,#37399,#37400,#37401,
#37402,#37403,#37404,#37405,#37406,#37407,#37408,#37409,#37410,#37411,#37412,
#37413,#37414,#37415,#37416,#37417,#37418,#37419,#37420,#37421,#37422,#37423,
#37424,#37425,#37426,#37427,#37428,#37429,#37430,#37431,#37432,#37433,#37434,
#37435,#37436,#37437,#37438,#37439,#37440,#37441,#37442,#37443,#37444,#37445,
#37446,#37447,#37448,#37449,#37450,#37451,#37452,#37453,#37454,#37455,#37456,
#37457,#37458,#37459,#37460,#37461,#37462,#37463,#37464,#37465,#37466,#37467,
#37468,#37469,#37470,#37471,#37472,#37473,#37474,#37475,#37476,#37477,#37478,
#37479,#37480,#37481,#37482,#37483,#37484,#37485,#37486,#37487,#37488,#37489,
#37490,#37491,#37492,#37493,#37494,#37495),(#37496,#37497,#37498,#37499,
#37500,#37501,#37502,#37503,#37504,#37505,#37506,#37507,#37508,#37509,#37510,
#37511,#37512,#37513,#37514,#37515,#37516,#37517,#37518,#37519,#37520,#37521,
#37522,#37523,#37524,#37525,#37526,#37527,#37528,#37529,#37530,#37531,#37532,
#37533,#37534,#37535,#37536,#37537,#37538,#37539,#37540,#37541,#37542,#37543,
#37544,#37545,#37546,#37547,#37548,#37549,#37550,#37551,#37552,#37553,#37554,
#37555,#37556,#37557,#37558,#37559,#37560,#37561,#37562,#37563,#37564,#37565,
#37566,#37567,#37568,#37569,#37570,#37571,#37572,#37573,#37574,#37575,#37576,
#37577,#37578,#37579,#37580,#37581,#37582,#37583,#37584,#37585,#37586,#37587,
#37588,#37589,#37590,#37591,#37592,#37593,#37594,#37595,#37596,#37597,#37598,
#37599,#37600,#37601,#37602,#37603,#37604,#37605,#37606,#37607,#37608,#37609,
#37610,#37611,#37612,#37613,#37614,#37615,#37616,#37617,#37618,#37619,#37620,
#37621,#37622,#37623,#37624,#37625,#37626,#37627,#37628,#37629,#37630,#37631,
#37632,#37633,#37634,#37635,#37636,#37637,#37638,#37639),(#37640,#37641,
#37642,#37643,#37644,#37645,#37646,#37647,#37648,#37649,#37650,#37651,#37652,
#37653,#37654,#37655,#37656,#37657,#37658,#37659,#37660,#37661,#37662,#37663,
#37664,#37665,#37666,#37667,#37668,#37669,#37670,#37671,#37672,#37673,#37674,
#37675,#37676,#37677,#37678,#37679,#37680,#37681,#37682,#37683,#37684,#37685,
#37686,#37687,#37688,#37689,#37690,#37691,#37692,#37693,#37694,#37695,#37696,
#37697,#37698,#37699,#37700,#37701,#37702,#37703,#37704,#37705,#37706,#37707,
#37708,#37709,#37710,#37711,#37712,#37713,#37714,#37715,#37716,#37717,#37718,
#37719,#37720,#37721,#37722,#37723,#37724,#37725,#37726,#37727,#37728,#37729,
#37730,#37731,#37732,#37733,#37734,#37735,#37736,#37737,#37738,#37739,#37740,
#37741,#37742,#37743,#37744,#37745,#37746,#37747,#37748,#37749,#37750,#37751,
#37752,#37753,#37754,#37755,#37756,#37757,#37758,#37759,#37760,#37761,#37762,
#37763,#37764,#37765,#37766,#37767,#37768,#37769,#37770,#37771,#37772,#37773,
#37774,#37775,#37776,#37777,#37778,#37779,#37780,#37781,#37782,#37783),
(#37784,#37785,#37786,#37787,#37788,#37789,#37790,#37791,#37792,#37793,
#37794,#37795,#37796,#37797,#37798,#37799,#37800,#37801,#37802,#37803,#37804,
#37805,#37806,#37807,#37808,#37809,#37810,#37811,#37812,#37813,#37814,#37815,
#37816,#37817,#37818,#37819,#37820,#37821,#37822,#37823,#37824,#37825,#37826,
#37827,#37828,#37829,#37830,#37831,#37832,#37833,#37834,#37835,#37836,#37837,
#37838,#37839,#37840,#37841,#37842,#37843,#37844,#37845,#37846,#37847,#37848,
#37849,#37850,#37851,#37852,#37853,#37854,#37855,#37856,#37857,#37858,#37859,
#37860,#37861,#37862,#37863,#37864,#37865,#37866,#37867,#37868,#37869,#37870,
#37871,#37872,#37873,#37874,#37875,#37876,#37877,#37878,#37879,#37880,#37881,
#37882,#37883,#37884,#37885,#37886,#37887,#37888,#37889,#37890,#37891,#37892,
#37893,#37894,#37895,#37896,#37897,#37898,#37899,#37900,#37901,#37902,#37903,
#37904,#37905,#37906,#37907,#37908,#37909,#37910,#37911,#37912,#37913,#37914,
#37915,#37916,#37917,#37918,#37919,#37920,#37921,#37922,#37923,#37924,#37925,
#37926,#37927),(#37928,#37929,#37930,#37931,#37932,#37933,#37934,#37935,
#37936,#37937,#37938,#37939,#37940,#37941,#37942,#37943,#37944,#37945,#37946,
#37947,#37948,#37949,#37950,#37951,#37952,#37953,#37954,#37955,#37956,#37957,
#37958,#37959,#37960,#37961,#37962,#37963,#37964,#37965,#37966,#37967,#37968,
#37969,#37970,#37971,#37972,#37973,#37974,#37975,#37976,#37977,#37978,#37979,
#37980,#37981,#37982,#37983,#37984,#37985,#37986,#37987,#37988,#37989,#37990,
#37991,#37992,#37993,#37994,#37995,#37996,#37997,#37998,#37999,#38000,#38001,
#38002,#38003,#38004,#38005,#38006,#38007,#38008,#38009,#38010,#38011,#38012,
#38013,#38014,#38015,#38016,#38017,#38018,#38019,#38020,#38021,#38022,#38023,
#38024,#38025,#38026,#38027,#38028,#38029,#38030,#38031,#38032,#38033,#38034,
#38035,#38036,#38037,#38038,#38039,#38040,#38041,#38042,#38043,#38044,#38045,
#38046,#38047,#38048,#38049,#38050,#38051,#38052,#38053,#38054,#38055,#38056,
#38057,#38058,#38059,#38060,#38061,#38062,#38063,#38064,#38065,#38066,#38067,
#38068,#38069,#38070,#38071),(#38072,#38073,#38074,#38075,#38076,#38077,
#38078,#38079,#38080,#38081,#38082,#38083,#38084,#38085,#38086,#38087,#38088,
#38089,#38090,#38091,#38092,#38093,#38094,#38095,#38096,#38097,#38098,#38099,
#38100,#38101,#38102,#38103,#38104,#38105,#38106,#38107,#38108,#38109,#38110,
#38111,#38112,#38113,#38114,#38115,#38116,#38117,#38118,#38119,#38120,#38121,
#38122,#38123,#38124,#38125,#38126,#38127,#38128,#38129,#38130,#38131,#38132,
#38133,#38134,#38135,#38136,#38137,#38138,#38139,#38140,#38141,#38142,#38143,
#38144,#38145,#38146,#38147,#38148,#38149,#38150,#38151,#38152,#38153,#38154,
#38155,#38156,#38157,#38158,#38159,#38160,#38161,#38162,#38163,#38164,#38165,
#38166,#38167,#38168,#38169,#38170,#38171,#38172,#38173,#38174,#38175,#38176,
#38177,#38178,#38179,#38180,#38181,#38182,#38183,#38184,#38185,#38186,#38187,
#38188,#38189,#38190,#38191,#38192,#38193,#38194,#38195,#38196,#38197,#38198,
#38199,#38200,#38201,#38202,#38203,#38204,#38205,#38206,#38207,#38208,#38209,
#38210,#38211,#38212,#38213,#38214,#38215),(#38216,#38217,#38218,#38219,
#38220,#38221,#38222,#38223,#38224,#38225,#38226,#38227,#38228,#38229,#38230,
#38231,#38232,#38233,#38234,#38235,#38236,#38237,#38238,#38239,#38240,#38241,
#38242,#38243,#38244,#38245,#38246,#38247,#38248,#38249,#38250,#38251,#38252,
#38253,#38254,#38255,#38256,#38257,#38258,#38259,#38260,#38261,#38262,#38263,
#38264,#38265,#38266,#38267,#38268,#38269,#38270,#38271,#38272,#38273,#38274,
#38275,#38276,#38277,#38278,#38279,#38280,#38281,#38282,#38283,#38284,#38285,
#38286,#38287,#38288,#38289,#38290,#38291,#38292,#38293,#38294,#38295,#38296,
#38297,#38298,#38299,#38300,#38301,#38302,#38303,#38304,#38305,#38306,#38307,
#38308,#38309,#38310,#38311,#38312,#38313,#38314,#38315,#38316,#38317,#38318,
#38319,#38320,#38321,#38322,#38323,#38324,#38325,#38326,#38327,#38328,#38329,
#38330,#38331,#38332,#38333,#38334,#38335,#38336,#38337,#38338,#38339,#38340,
#38341,#38342,#38343,#38344,#38345,#38346,#38347,#38348,#38349,#38350,#38351,
#38352,#38353,#38354,#38355,#38356,#38357,#38358,#38359),(#38360,#38361,
#38362,#38363,#38364,#38365,#38366,#38367,#38368,#38369,#38370,#38371,#38372,
#38373,#38374,#38375,#38376,#38377,#38378,#38379,#38380,#38381,#38382,#38383,
#38384,#38385,#38386,#38387,#38388,#38389,#38390,#38391,#38392,#38393,#38394,
#38395,#38396,#38397,#38398,#38399,#38400,#38401,#38402,#38403,#38404,#38405,
#38406,#38407,#38408,#38409,#38410,#38411,#38412,#38413,#38414,#38415,#38416,
#38417,#38418,#38419,#38420,#38421,#38422,#38423,#38424,#38425,#38426,#38427,
#38428,#38429,#38430,#38431,#38432,#38433,#38434,#38435,#38436,#38437,#38438,
#38439,#38440,#38441,#38442,#38443,#38444,#38445,#38446,#38447,#38448,#38449,
#38450,#38451,#38452,#38453,#38454,#38455,#38456,#38457,#38458,#38459,#38460,
#38461,#38462,#38463,#38464,#38465,#38466,#38467,#38468,#38469,#38470,#38471,
#38472,#38473,#38474,#38475,#38476,#38477,#38478,#38479,#38480,#38481,#38482,
#38483,#38484,#38485,#38486,#38487,#38488,#38489,#38490,#38491,#38492,#38493,
#38494,#38495,#38496,#38497,#38498,#38499,#38500,#38501,#38502,#38503),
(#38504,#38505,#38506,#38507,#38508,#38509,#38510,#38511,#38512,#38513,
#38514,#38515,#38516,#38517,#38518,#38519,#38520,#38521,#38522,#38523,#38524,
#38525,#38526,#38527,#38528,#38529,#38530,#38531,#38532,#38533,#38534,#38535,
#38536,#38537,#38538,#38539,#38540,#38541,#38542,#38543,#38544,#38545,#38546,
#38547,#38548,#38549,#38550,#38551,#38552,#38553,#38554,#38555,#38556,#38557,
#38558,#38559,#38560,#38561,#38562,#38563,#38564,#38565,#38566,#38567,#38568,
#38569,#38570,#38571,#38572,#38573,#38574,#38575,#38576,#38577,#38578,#38579,
#38580,#38581,#38582,#38583,#38584,#38585,#38586,#38587,#38588,#38589,#38590,
#38591,#38592,#38593,#38594,#38595,#38596,#38597,#38598,#38599,#38600,#38601,
#38602,#38603,#38604,#38605,#38606,#38607,#38608,#38609,#38610,#38611,#38612,
#38613,#38614,#38615,#38616,#38617,#38618,#38619,#38620,#38621,#38622,#38623,
#38624,#38625,#38626,#38627,#38628,#38629,#38630,#38631,#38632,#38633,#38634,
#38635,#38636,#38637,#38638,#38639,#38640,#38641,#38642,#38643,#38644,#38645,
#38646,#38647)),.UNSPECIFIED.,.F.,.F.,.F.,(4,1,1,1,1,1,1,1,1,1,1,1,1,1,
1,1,1,1,1,1,1,1,1,1,1,1,1,1,1,1,1,1,1,1,1,1,1,1,1,1,1,1,1,1,1,1,1,1,1,1,
1,1,1,1,1,1,1,1,1,1,1,1,1,1,1,4),(4,2,1,1,2,1,1,1,2,1,1,1,2,1,1,1,1,2,1,
1,1,1,1,1,1,2,1,1,1,1,1,1,1,2,1,1,1,1,1,1,1,1,2,1,1,1,1,1,1,1,1,1,1,1,2,
1,1,1,1,1,2,1,1,1,1,1,1,1,1,2,1,1,1,1,2,1,1,1,1,1,1,1,1,1,1,1,2,1,1,1,1,
1,2,1,1,1,1,2,1,1,1,1,1,1,1,1,1,1,1,1,1,2,1,1,1,1,2,1,1,1,1,1,2,4),(0.0268159196746105,
0.0437158964674566,0.0606153077094141,0.0775147189513715,0.094414130193329,
0.111313541435286,0.128212952677244,0.145112363919201,0.162011775161159,
0.178911186403116,0.195810597645074,0.212710008887031,0.229609420128989,
0.246508831370946,0.254958536991925,0.263408242612904,0.280307653854861,
0.297207065096819,0.308473339258124,0.319739613419429,0.331005887580734,
0.342272161742039,0.353538435903344,0.364804710064649,0.387337258387259,
0.398603532548564,0.409869806709869,0.421136080871174,0.432402355032479,
0.454934903355088,0.466201177516393,0.477467451677698,0.488733725839003,
0.500000000000308,0.511266274161613,0.522532548322918,0.545065096645528,
0.556331370806833,0.567597644968138,0.584497056210096,0.601396467452053,
0.618295878694011,0.635195289935968,0.652094701177926,0.668994112419883,
0.677443818040862,0.685893523661841,0.694343229282819,0.702792934903798,
0.719692346145756,0.736591757387713,0.745041463008692,0.75349116862967,
0.770390579871628,0.787289991113585,0.804189402355543,0.8210888135975,0.837988224839458,
0.854887636081415,0.871787047323373,0.88868645856533,0.905585869807288,
0.922485281049245,0.939384692291203,0.95628410353316,0.973184071869037),
(0.0960305811261702,0.0972154775043869,0.109378606187391,0.121541734870394,
0.145867992236401,0.151993923775347,0.158119855314292,0.170371718392183,
0.194875444547964,0.200989580746302,0.207103716944641,0.219331989341318,
0.243788534134673,0.246827927163601,0.24986732019253,0.255946106250386,
0.2681036783661,0.292418822597527,0.293959106599555,0.295499390601583,0.29857995860564,
0.304741094613752,0.310902230621865,0.317063366629978,0.329385638646203,
0.341707910662428,0.344790082003921,0.347872253345414,0.354036596028399,
0.36636528139437,0.37869396676034,0.384858309443326,0.387940480784818,0.391022652126311,
0.392583125212554,0.394143598298796,0.397264544471281,0.403506436816251,
0.422232113851161,0.428474006196132,0.434715898541102,0.437836844713587,
0.440957790886072,0.442498863959882,0.444039937033693,0.447122083181315,
0.448663156255125,0.450204229328936,0.450974765865841,0.451745302402747,
0.453286375476557,0.4594506677718,0.465614960067043,0.477943544657529,0.490272129248014,
0.493311253959715,0.496350378671415,0.502428628094816,0.514585126941617,
0.526741625788419,0.53889812463522,0.540417366609575,0.541936608583929,
0.544975092532638,0.551052060430056,0.563205996224891,0.569282964122308,
0.575359932019726,0.581436899917144,0.587513867814562,0.590576684581802,
0.593639501349043,0.599765134883524,0.612016401952486,0.636518936090411,
0.639559223907375,0.642599511724338,0.645639799541302,0.648680087358265,
0.654760662992193,0.66084123862612,0.666921814260047,0.669962102077011,
0.673002389893974,0.676042677710938,0.679082965527902,0.685163541161829,
0.688226234079092,0.691288926996354,0.697414312830879,0.70966508449993,
0.72191585616898,0.734166627838031,0.737264704064826,0.740362780291622,
0.746558932745213,0.758951237652395,0.783735847466759,0.785338745832564,
0.78694164419837,0.790147440929981,0.796559034393203,0.809382221319647,
0.815793814782869,0.822205408246091,0.823808306611897,0.825411204977702,
0.828617001709314,0.830219900075119,0.831021349258022,0.831822798440925,
0.835028595172536,0.838457852551916,0.841887109931297,0.848745624690058,
0.86246265420758,0.889896713242625,0.893337440953794,0.896778168664963,
0.9036596240873,0.910541079509638,0.917422534931976,0.944948356621327,0.967478850977141),
 .UNSPECIFIED.);
#18851=B_SPLINE_SURFACE_WITH_KNOTS('',3,3,((#41157,#41158,#41159,#41160,
#41161,#41162,#41163,#41164,#41165,#41166,#41167,#41168,#41169,#41170,#41171,
#41172,#41173,#41174,#41175,#41176,#41177,#41178,#41179,#41180,#41181,#41182,
#41183,#41184,#41185,#41186,#41187,#41188,#41189,#41190,#41191,#41192,#41193,
#41194,#41195,#41196,#41197),(#41198,#41199,#41200,#41201,#41202,#41203,
#41204,#41205,#41206,#41207,#41208,#41209,#41210,#41211,#41212,#41213,#41214,
#41215,#41216,#41217,#41218,#41219,#41220,#41221,#41222,#41223,#41224,#41225,
#41226,#41227,#41228,#41229,#41230,#41231,#41232,#41233,#41234,#41235,#41236,
#41237,#41238),(#41239,#41240,#41241,#41242,#41243,#41244,#41245,#41246,
#41247,#41248,#41249,#41250,#41251,#41252,#41253,#41254,#41255,#41256,#41257,
#41258,#41259,#41260,#41261,#41262,#41263,#41264,#41265,#41266,#41267,#41268,
#41269,#41270,#41271,#41272,#41273,#41274,#41275,#41276,#41277,#41278,#41279),
(#41280,#41281,#41282,#41283,#41284,#41285,#41286,#41287,#41288,#41289,
#41290,#41291,#41292,#41293,#41294,#41295,#41296,#41297,#41298,#41299,#41300,
#41301,#41302,#41303,#41304,#41305,#41306,#41307,#41308,#41309,#41310,#41311,
#41312,#41313,#41314,#41315,#41316,#41317,#41318,#41319,#41320),(#41321,
#41322,#41323,#41324,#41325,#41326,#41327,#41328,#41329,#41330,#41331,#41332,
#41333,#41334,#41335,#41336,#41337,#41338,#41339,#41340,#41341,#41342,#41343,
#41344,#41345,#41346,#41347,#41348,#41349,#41350,#41351,#41352,#41353,#41354,
#41355,#41356,#41357,#41358,#41359,#41360,#41361)),.UNSPECIFIED.,.F.,.T.,
 .F.,(4,1,4),(4,1,1,1,2,1,1,1,1,2,1,1,1,2,1,1,1,2,2,1,2,2,2,2,1,2,1,1,4),
(0.,0.571428571428571,1.),(-9.55960092302324,-9.1896794456085,-8.81975796819377,
-8.44983649077903,-8.0799150133643,-8.03266253512535,-7.98541005688641,
-7.89090510040853,-7.70189518745276,-7.32387536154123,-7.17881214312514,
-7.03374892470906,-6.88868570629297,-6.74362248787689,-6.67050437063,-6.59738625338311,
-6.45115001888933,-6.15867754990177,-5.47160541199434,-4.26766323501505,
-3.06372105803577,-2.37819810334092,-1.79056374069951,-1.18667868852568,
-0.800342864550781,-0.414007040575882,-0.310505280431912,-0.207003520287941,
0.),.UNSPECIFIED.);
#18852=B_SPLINE_SURFACE_WITH_KNOTS('',3,3,((#41541,#41542,#41543,#41544,
#41545,#41546,#41547,#41548,#41549,#41550,#41551,#41552,#41553,#41554,#41555,
#41556,#41557,#41558,#41559,#41560,#41561,#41562,#41563,#41564,#41565,#41566,
#41567,#41568,#41569,#41570,#41571,#41572,#41573,#41574,#41575,#41576,#41577,
#41578,#41579,#41580,#41581,#41582,#41583,#41584,#41585,#41586,#41587,#41588,
#41589,#41590,#41591,#41592,#41593,#41594,#41595,#41596,#41597,#41598,#41599,
#41600,#41601,#41602,#41603,#41604,#41605,#41606,#41607,#41608,#41609,#41610,
#41611,#41612,#41613,#41614,#41615,#41616,#41617,#41618,#41619,#41620,#41621,
#41622,#41623,#41624,#41625,#41626,#41627,#41628,#41629,#41630,#41631,#41632,
#41633,#41634,#41635,#41636,#41637,#41638,#41639,#41640,#41641,#41642,#41643,
#41644,#41645,#41646,#41647,#41648,#41649,#41650,#41651,#41652,#41653,#41654,
#41655,#41656,#41657,#41658,#41659,#41660,#41661,#41662,#41663,#41664,#41665,
#41666,#41667,#41668,#41669,#41670,#41671,#41672,#41673,#41674,#41675,#41676,
#41677,#41678,#41679,#41680,#41681,#41682,#41683,#41684),(#41685,#41686,
#41687,#41688,#41689,#41690,#41691,#41692,#41693,#41694,#41695,#41696,#41697,
#41698,#41699,#41700,#41701,#41702,#41703,#41704,#41705,#41706,#41707,#41708,
#41709,#41710,#41711,#41712,#41713,#41714,#41715,#41716,#41717,#41718,#41719,
#41720,#41721,#41722,#41723,#41724,#41725,#41726,#41727,#41728,#41729,#41730,
#41731,#41732,#41733,#41734,#41735,#41736,#41737,#41738,#41739,#41740,#41741,
#41742,#41743,#41744,#41745,#41746,#41747,#41748,#41749,#41750,#41751,#41752,
#41753,#41754,#41755,#41756,#41757,#41758,#41759,#41760,#41761,#41762,#41763,
#41764,#41765,#41766,#41767,#41768,#41769,#41770,#41771,#41772,#41773,#41774,
#41775,#41776,#41777,#41778,#41779,#41780,#41781,#41782,#41783,#41784,#41785,
#41786,#41787,#41788,#41789,#41790,#41791,#41792,#41793,#41794,#41795,#41796,
#41797,#41798,#41799,#41800,#41801,#41802,#41803,#41804,#41805,#41806,#41807,
#41808,#41809,#41810,#41811,#41812,#41813,#41814,#41815,#41816,#41817,#41818,
#41819,#41820,#41821,#41822,#41823,#41824,#41825,#41826,#41827,#41828),
(#41829,#41830,#41831,#41832,#41833,#41834,#41835,#41836,#41837,#41838,
#41839,#41840,#41841,#41842,#41843,#41844,#41845,#41846,#41847,#41848,#41849,
#41850,#41851,#41852,#41853,#41854,#41855,#41856,#41857,#41858,#41859,#41860,
#41861,#41862,#41863,#41864,#41865,#41866,#41867,#41868,#41869,#41870,#41871,
#41872,#41873,#41874,#41875,#41876,#41877,#41878,#41879,#41880,#41881,#41882,
#41883,#41884,#41885,#41886,#41887,#41888,#41889,#41890,#41891,#41892,#41893,
#41894,#41895,#41896,#41897,#41898,#41899,#41900,#41901,#41902,#41903,#41904,
#41905,#41906,#41907,#41908,#41909,#41910,#41911,#41912,#41913,#41914,#41915,
#41916,#41917,#41918,#41919,#41920,#41921,#41922,#41923,#41924,#41925,#41926,
#41927,#41928,#41929,#41930,#41931,#41932,#41933,#41934,#41935,#41936,#41937,
#41938,#41939,#41940,#41941,#41942,#41943,#41944,#41945,#41946,#41947,#41948,
#41949,#41950,#41951,#41952,#41953,#41954,#41955,#41956,#41957,#41958,#41959,
#41960,#41961,#41962,#41963,#41964,#41965,#41966,#41967,#41968,#41969,#41970,
#41971,#41972),(#41973,#41974,#41975,#41976,#41977,#41978,#41979,#41980,
#41981,#41982,#41983,#41984,#41985,#41986,#41987,#41988,#41989,#41990,#41991,
#41992,#41993,#41994,#41995,#41996,#41997,#41998,#41999,#42000,#42001,#42002,
#42003,#42004,#42005,#42006,#42007,#42008,#42009,#42010,#42011,#42012,#42013,
#42014,#42015,#42016,#42017,#42018,#42019,#42020,#42021,#42022,#42023,#42024,
#42025,#42026,#42027,#42028,#42029,#42030,#42031,#42032,#42033,#42034,#42035,
#42036,#42037,#42038,#42039,#42040,#42041,#42042,#42043,#42044,#42045,#42046,
#42047,#42048,#42049,#42050,#42051,#42052,#42053,#42054,#42055,#42056,#42057,
#42058,#42059,#42060,#42061,#42062,#42063,#42064,#42065,#42066,#42067,#42068,
#42069,#42070,#42071,#42072,#42073,#42074,#42075,#42076,#42077,#42078,#42079,
#42080,#42081,#42082,#42083,#42084,#42085,#42086,#42087,#42088,#42089,#42090,
#42091,#42092,#42093,#42094,#42095,#42096,#42097,#42098,#42099,#42100,#42101,
#42102,#42103,#42104,#42105,#42106,#42107,#42108,#42109,#42110,#42111,#42112,
#42113,#42114,#42115,#42116),(#42117,#42118,#42119,#42120,#42121,#42122,
#42123,#42124,#42125,#42126,#42127,#42128,#42129,#42130,#42131,#42132,#42133,
#42134,#42135,#42136,#42137,#42138,#42139,#42140,#42141,#42142,#42143,#42144,
#42145,#42146,#42147,#42148,#42149,#42150,#42151,#42152,#42153,#42154,#42155,
#42156,#42157,#42158,#42159,#42160,#42161,#42162,#42163,#42164,#42165,#42166,
#42167,#42168,#42169,#42170,#42171,#42172,#42173,#42174,#42175,#42176,#42177,
#42178,#42179,#42180,#42181,#42182,#42183,#42184,#42185,#42186,#42187,#42188,
#42189,#42190,#42191,#42192,#42193,#42194,#42195,#42196,#42197,#42198,#42199,
#42200,#42201,#42202,#42203,#42204,#42205,#42206,#42207,#42208,#42209,#42210,
#42211,#42212,#42213,#42214,#42215,#42216,#42217,#42218,#42219,#42220,#42221,
#42222,#42223,#42224,#42225,#42226,#42227,#42228,#42229,#42230,#42231,#42232,
#42233,#42234,#42235,#42236,#42237,#42238,#42239,#42240,#42241,#42242,#42243,
#42244,#42245,#42246,#42247,#42248,#42249,#42250,#42251,#42252,#42253,#42254,
#42255,#42256,#42257,#42258,#42259,#42260),(#42261,#42262,#42263,#42264,
#42265,#42266,#42267,#42268,#42269,#42270,#42271,#42272,#42273,#42274,#42275,
#42276,#42277,#42278,#42279,#42280,#42281,#42282,#42283,#42284,#42285,#42286,
#42287,#42288,#42289,#42290,#42291,#42292,#42293,#42294,#42295,#42296,#42297,
#42298,#42299,#42300,#42301,#42302,#42303,#42304,#42305,#42306,#42307,#42308,
#42309,#42310,#42311,#42312,#42313,#42314,#42315,#42316,#42317,#42318,#42319,
#42320,#42321,#42322,#42323,#42324,#42325,#42326,#42327,#42328,#42329,#42330,
#42331,#42332,#42333,#42334,#42335,#42336,#42337,#42338,#42339,#42340,#42341,
#42342,#42343,#42344,#42345,#42346,#42347,#42348,#42349,#42350,#42351,#42352,
#42353,#42354,#42355,#42356,#42357,#42358,#42359,#42360,#42361,#42362,#42363,
#42364,#42365,#42366,#42367,#42368,#42369,#42370,#42371,#42372,#42373,#42374,
#42375,#42376,#42377,#42378,#42379,#42380,#42381,#42382,#42383,#42384,#42385,
#42386,#42387,#42388,#42389,#42390,#42391,#42392,#42393,#42394,#42395,#42396,
#42397,#42398,#42399,#42400,#42401,#42402,#42403,#42404),(#42405,#42406,
#42407,#42408,#42409,#42410,#42411,#42412,#42413,#42414,#42415,#42416,#42417,
#42418,#42419,#42420,#42421,#42422,#42423,#42424,#42425,#42426,#42427,#42428,
#42429,#42430,#42431,#42432,#42433,#42434,#42435,#42436,#42437,#42438,#42439,
#42440,#42441,#42442,#42443,#42444,#42445,#42446,#42447,#42448,#42449,#42450,
#42451,#42452,#42453,#42454,#42455,#42456,#42457,#42458,#42459,#42460,#42461,
#42462,#42463,#42464,#42465,#42466,#42467,#42468,#42469,#42470,#42471,#42472,
#42473,#42474,#42475,#42476,#42477,#42478,#42479,#42480,#42481,#42482,#42483,
#42484,#42485,#42486,#42487,#42488,#42489,#42490,#42491,#42492,#42493,#42494,
#42495,#42496,#42497,#42498,#42499,#42500,#42501,#42502,#42503,#42504,#42505,
#42506,#42507,#42508,#42509,#42510,#42511,#42512,#42513,#42514,#42515,#42516,
#42517,#42518,#42519,#42520,#42521,#42522,#42523,#42524,#42525,#42526,#42527,
#42528,#42529,#42530,#42531,#42532,#42533,#42534,#42535,#42536,#42537,#42538,
#42539,#42540,#42541,#42542,#42543,#42544,#42545,#42546,#42547,#42548),
(#42549,#42550,#42551,#42552,#42553,#42554,#42555,#42556,#42557,#42558,
#42559,#42560,#42561,#42562,#42563,#42564,#42565,#42566,#42567,#42568,#42569,
#42570,#42571,#42572,#42573,#42574,#42575,#42576,#42577,#42578,#42579,#42580,
#42581,#42582,#42583,#42584,#42585,#42586,#42587,#42588,#42589,#42590,#42591,
#42592,#42593,#42594,#42595,#42596,#42597,#42598,#42599,#42600,#42601,#42602,
#42603,#42604,#42605,#42606,#42607,#42608,#42609,#42610,#42611,#42612,#42613,
#42614,#42615,#42616,#42617,#42618,#42619,#42620,#42621,#42622,#42623,#42624,
#42625,#42626,#42627,#42628,#42629,#42630,#42631,#42632,#42633,#42634,#42635,
#42636,#42637,#42638,#42639,#42640,#42641,#42642,#42643,#42644,#42645,#42646,
#42647,#42648,#42649,#42650,#42651,#42652,#42653,#42654,#42655,#42656,#42657,
#42658,#42659,#42660,#42661,#42662,#42663,#42664,#42665,#42666,#42667,#42668,
#42669,#42670,#42671,#42672,#42673,#42674,#42675,#42676,#42677,#42678,#42679,
#42680,#42681,#42682,#42683,#42684,#42685,#42686,#42687,#42688,#42689,#42690,
#42691,#42692),(#42693,#42694,#42695,#42696,#42697,#42698,#42699,#42700,
#42701,#42702,#42703,#42704,#42705,#42706,#42707,#42708,#42709,#42710,#42711,
#42712,#42713,#42714,#42715,#42716,#42717,#42718,#42719,#42720,#42721,#42722,
#42723,#42724,#42725,#42726,#42727,#42728,#42729,#42730,#42731,#42732,#42733,
#42734,#42735,#42736,#42737,#42738,#42739,#42740,#42741,#42742,#42743,#42744,
#42745,#42746,#42747,#42748,#42749,#42750,#42751,#42752,#42753,#42754,#42755,
#42756,#42757,#42758,#42759,#42760,#42761,#42762,#42763,#42764,#42765,#42766,
#42767,#42768,#42769,#42770,#42771,#42772,#42773,#42774,#42775,#42776,#42777,
#42778,#42779,#42780,#42781,#42782,#42783,#42784,#42785,#42786,#42787,#42788,
#42789,#42790,#42791,#42792,#42793,#42794,#42795,#42796,#42797,#42798,#42799,
#42800,#42801,#42802,#42803,#42804,#42805,#42806,#42807,#42808,#42809,#42810,
#42811,#42812,#42813,#42814,#42815,#42816,#42817,#42818,#42819,#42820,#42821,
#42822,#42823,#42824,#42825,#42826,#42827,#42828,#42829,#42830,#42831,#42832,
#42833,#42834,#42835,#42836),(#42837,#42838,#42839,#42840,#42841,#42842,
#42843,#42844,#42845,#42846,#42847,#42848,#42849,#42850,#42851,#42852,#42853,
#42854,#42855,#42856,#42857,#42858,#42859,#42860,#42861,#42862,#42863,#42864,
#42865,#42866,#42867,#42868,#42869,#42870,#42871,#42872,#42873,#42874,#42875,
#42876,#42877,#42878,#42879,#42880,#42881,#42882,#42883,#42884,#42885,#42886,
#42887,#42888,#42889,#42890,#42891,#42892,#42893,#42894,#42895,#42896,#42897,
#42898,#42899,#42900,#42901,#42902,#42903,#42904,#42905,#42906,#42907,#42908,
#42909,#42910,#42911,#42912,#42913,#42914,#42915,#42916,#42917,#42918,#42919,
#42920,#42921,#42922,#42923,#42924,#42925,#42926,#42927,#42928,#42929,#42930,
#42931,#42932,#42933,#42934,#42935,#42936,#42937,#42938,#42939,#42940,#42941,
#42942,#42943,#42944,#42945,#42946,#42947,#42948,#42949,#42950,#42951,#42952,
#42953,#42954,#42955,#42956,#42957,#42958,#42959,#42960,#42961,#42962,#42963,
#42964,#42965,#42966,#42967,#42968,#42969,#42970,#42971,#42972,#42973,#42974,
#42975,#42976,#42977,#42978,#42979,#42980),(#42981,#42982,#42983,#42984,
#42985,#42986,#42987,#42988,#42989,#42990,#42991,#42992,#42993,#42994,#42995,
#42996,#42997,#42998,#42999,#43000,#43001,#43002,#43003,#43004,#43005,#43006,
#43007,#43008,#43009,#43010,#43011,#43012,#43013,#43014,#43015,#43016,#43017,
#43018,#43019,#43020,#43021,#43022,#43023,#43024,#43025,#43026,#43027,#43028,
#43029,#43030,#43031,#43032,#43033,#43034,#43035,#43036,#43037,#43038,#43039,
#43040,#43041,#43042,#43043,#43044,#43045,#43046,#43047,#43048,#43049,#43050,
#43051,#43052,#43053,#43054,#43055,#43056,#43057,#43058,#43059,#43060,#43061,
#43062,#43063,#43064,#43065,#43066,#43067,#43068,#43069,#43070,#43071,#43072,
#43073,#43074,#43075,#43076,#43077,#43078,#43079,#43080,#43081,#43082,#43083,
#43084,#43085,#43086,#43087,#43088,#43089,#43090,#43091,#43092,#43093,#43094,
#43095,#43096,#43097,#43098,#43099,#43100,#43101,#43102,#43103,#43104,#43105,
#43106,#43107,#43108,#43109,#43110,#43111,#43112,#43113,#43114,#43115,#43116,
#43117,#43118,#43119,#43120,#43121,#43122,#43123,#43124),(#43125,#43126,
#43127,#43128,#43129,#43130,#43131,#43132,#43133,#43134,#43135,#43136,#43137,
#43138,#43139,#43140,#43141,#43142,#43143,#43144,#43145,#43146,#43147,#43148,
#43149,#43150,#43151,#43152,#43153,#43154,#43155,#43156,#43157,#43158,#43159,
#43160,#43161,#43162,#43163,#43164,#43165,#43166,#43167,#43168,#43169,#43170,
#43171,#43172,#43173,#43174,#43175,#43176,#43177,#43178,#43179,#43180,#43181,
#43182,#43183,#43184,#43185,#43186,#43187,#43188,#43189,#43190,#43191,#43192,
#43193,#43194,#43195,#43196,#43197,#43198,#43199,#43200,#43201,#43202,#43203,
#43204,#43205,#43206,#43207,#43208,#43209,#43210,#43211,#43212,#43213,#43214,
#43215,#43216,#43217,#43218,#43219,#43220,#43221,#43222,#43223,#43224,#43225,
#43226,#43227,#43228,#43229,#43230,#43231,#43232,#43233,#43234,#43235,#43236,
#43237,#43238,#43239,#43240,#43241,#43242,#43243,#43244,#43245,#43246,#43247,
#43248,#43249,#43250,#43251,#43252,#43253,#43254,#43255,#43256,#43257,#43258,
#43259,#43260,#43261,#43262,#43263,#43264,#43265,#43266,#43267,#43268),
(#43269,#43270,#43271,#43272,#43273,#43274,#43275,#43276,#43277,#43278,
#43279,#43280,#43281,#43282,#43283,#43284,#43285,#43286,#43287,#43288,#43289,
#43290,#43291,#43292,#43293,#43294,#43295,#43296,#43297,#43298,#43299,#43300,
#43301,#43302,#43303,#43304,#43305,#43306,#43307,#43308,#43309,#43310,#43311,
#43312,#43313,#43314,#43315,#43316,#43317,#43318,#43319,#43320,#43321,#43322,
#43323,#43324,#43325,#43326,#43327,#43328,#43329,#43330,#43331,#43332,#43333,
#43334,#43335,#43336,#43337,#43338,#43339,#43340,#43341,#43342,#43343,#43344,
#43345,#43346,#43347,#43348,#43349,#43350,#43351,#43352,#43353,#43354,#43355,
#43356,#43357,#43358,#43359,#43360,#43361,#43362,#43363,#43364,#43365,#43366,
#43367,#43368,#43369,#43370,#43371,#43372,#43373,#43374,#43375,#43376,#43377,
#43378,#43379,#43380,#43381,#43382,#43383,#43384,#43385,#43386,#43387,#43388,
#43389,#43390,#43391,#43392,#43393,#43394,#43395,#43396,#43397,#43398,#43399,
#43400,#43401,#43402,#43403,#43404,#43405,#43406,#43407,#43408,#43409,#43410,
#43411,#43412),(#43413,#43414,#43415,#43416,#43417,#43418,#43419,#43420,
#43421,#43422,#43423,#43424,#43425,#43426,#43427,#43428,#43429,#43430,#43431,
#43432,#43433,#43434,#43435,#43436,#43437,#43438,#43439,#43440,#43441,#43442,
#43443,#43444,#43445,#43446,#43447,#43448,#43449,#43450,#43451,#43452,#43453,
#43454,#43455,#43456,#43457,#43458,#43459,#43460,#43461,#43462,#43463,#43464,
#43465,#43466,#43467,#43468,#43469,#43470,#43471,#43472,#43473,#43474,#43475,
#43476,#43477,#43478,#43479,#43480,#43481,#43482,#43483,#43484,#43485,#43486,
#43487,#43488,#43489,#43490,#43491,#43492,#43493,#43494,#43495,#43496,#43497,
#43498,#43499,#43500,#43501,#43502,#43503,#43504,#43505,#43506,#43507,#43508,
#43509,#43510,#43511,#43512,#43513,#43514,#43515,#43516,#43517,#43518,#43519,
#43520,#43521,#43522,#43523,#43524,#43525,#43526,#43527,#43528,#43529,#43530,
#43531,#43532,#43533,#43534,#43535,#43536,#43537,#43538,#43539,#43540,#43541,
#43542,#43543,#43544,#43545,#43546,#43547,#43548,#43549,#43550,#43551,#43552,
#43553,#43554,#43555,#43556),(#43557,#43558,#43559,#43560,#43561,#43562,
#43563,#43564,#43565,#43566,#43567,#43568,#43569,#43570,#43571,#43572,#43573,
#43574,#43575,#43576,#43577,#43578,#43579,#43580,#43581,#43582,#43583,#43584,
#43585,#43586,#43587,#43588,#43589,#43590,#43591,#43592,#43593,#43594,#43595,
#43596,#43597,#43598,#43599,#43600,#43601,#43602,#43603,#43604,#43605,#43606,
#43607,#43608,#43609,#43610,#43611,#43612,#43613,#43614,#43615,#43616,#43617,
#43618,#43619,#43620,#43621,#43622,#43623,#43624,#43625,#43626,#43627,#43628,
#43629,#43630,#43631,#43632,#43633,#43634,#43635,#43636,#43637,#43638,#43639,
#43640,#43641,#43642,#43643,#43644,#43645,#43646,#43647,#43648,#43649,#43650,
#43651,#43652,#43653,#43654,#43655,#43656,#43657,#43658,#43659,#43660,#43661,
#43662,#43663,#43664,#43665,#43666,#43667,#43668,#43669,#43670,#43671,#43672,
#43673,#43674,#43675,#43676,#43677,#43678,#43679,#43680,#43681,#43682,#43683,
#43684,#43685,#43686,#43687,#43688,#43689,#43690,#43691,#43692,#43693,#43694,
#43695,#43696,#43697,#43698,#43699,#43700),(#43701,#43702,#43703,#43704,
#43705,#43706,#43707,#43708,#43709,#43710,#43711,#43712,#43713,#43714,#43715,
#43716,#43717,#43718,#43719,#43720,#43721,#43722,#43723,#43724,#43725,#43726,
#43727,#43728,#43729,#43730,#43731,#43732,#43733,#43734,#43735,#43736,#43737,
#43738,#43739,#43740,#43741,#43742,#43743,#43744,#43745,#43746,#43747,#43748,
#43749,#43750,#43751,#43752,#43753,#43754,#43755,#43756,#43757,#43758,#43759,
#43760,#43761,#43762,#43763,#43764,#43765,#43766,#43767,#43768,#43769,#43770,
#43771,#43772,#43773,#43774,#43775,#43776,#43777,#43778,#43779,#43780,#43781,
#43782,#43783,#43784,#43785,#43786,#43787,#43788,#43789,#43790,#43791,#43792,
#43793,#43794,#43795,#43796,#43797,#43798,#43799,#43800,#43801,#43802,#43803,
#43804,#43805,#43806,#43807,#43808,#43809,#43810,#43811,#43812,#43813,#43814,
#43815,#43816,#43817,#43818,#43819,#43820,#43821,#43822,#43823,#43824,#43825,
#43826,#43827,#43828,#43829,#43830,#43831,#43832,#43833,#43834,#43835,#43836,
#43837,#43838,#43839,#43840,#43841,#43842,#43843,#43844),(#43845,#43846,
#43847,#43848,#43849,#43850,#43851,#43852,#43853,#43854,#43855,#43856,#43857,
#43858,#43859,#43860,#43861,#43862,#43863,#43864,#43865,#43866,#43867,#43868,
#43869,#43870,#43871,#43872,#43873,#43874,#43875,#43876,#43877,#43878,#43879,
#43880,#43881,#43882,#43883,#43884,#43885,#43886,#43887,#43888,#43889,#43890,
#43891,#43892,#43893,#43894,#43895,#43896,#43897,#43898,#43899,#43900,#43901,
#43902,#43903,#43904,#43905,#43906,#43907,#43908,#43909,#43910,#43911,#43912,
#43913,#43914,#43915,#43916,#43917,#43918,#43919,#43920,#43921,#43922,#43923,
#43924,#43925,#43926,#43927,#43928,#43929,#43930,#43931,#43932,#43933,#43934,
#43935,#43936,#43937,#43938,#43939,#43940,#43941,#43942,#43943,#43944,#43945,
#43946,#43947,#43948,#43949,#43950,#43951,#43952,#43953,#43954,#43955,#43956,
#43957,#43958,#43959,#43960,#43961,#43962,#43963,#43964,#43965,#43966,#43967,
#43968,#43969,#43970,#43971,#43972,#43973,#43974,#43975,#43976,#43977,#43978,
#43979,#43980,#43981,#43982,#43983,#43984,#43985,#43986,#43987,#43988),
(#43989,#43990,#43991,#43992,#43993,#43994,#43995,#43996,#43997,#43998,
#43999,#44000,#44001,#44002,#44003,#44004,#44005,#44006,#44007,#44008,#44009,
#44010,#44011,#44012,#44013,#44014,#44015,#44016,#44017,#44018,#44019,#44020,
#44021,#44022,#44023,#44024,#44025,#44026,#44027,#44028,#44029,#44030,#44031,
#44032,#44033,#44034,#44035,#44036,#44037,#44038,#44039,#44040,#44041,#44042,
#44043,#44044,#44045,#44046,#44047,#44048,#44049,#44050,#44051,#44052,#44053,
#44054,#44055,#44056,#44057,#44058,#44059,#44060,#44061,#44062,#44063,#44064,
#44065,#44066,#44067,#44068,#44069,#44070,#44071,#44072,#44073,#44074,#44075,
#44076,#44077,#44078,#44079,#44080,#44081,#44082,#44083,#44084,#44085,#44086,
#44087,#44088,#44089,#44090,#44091,#44092,#44093,#44094,#44095,#44096,#44097,
#44098,#44099,#44100,#44101,#44102,#44103,#44104,#44105,#44106,#44107,#44108,
#44109,#44110,#44111,#44112,#44113,#44114,#44115,#44116,#44117,#44118,#44119,
#44120,#44121,#44122,#44123,#44124,#44125,#44126,#44127,#44128,#44129,#44130,
#44131,#44132),(#44133,#44134,#44135,#44136,#44137,#44138,#44139,#44140,
#44141,#44142,#44143,#44144,#44145,#44146,#44147,#44148,#44149,#44150,#44151,
#44152,#44153,#44154,#44155,#44156,#44157,#44158,#44159,#44160,#44161,#44162,
#44163,#44164,#44165,#44166,#44167,#44168,#44169,#44170,#44171,#44172,#44173,
#44174,#44175,#44176,#44177,#44178,#44179,#44180,#44181,#44182,#44183,#44184,
#44185,#44186,#44187,#44188,#44189,#44190,#44191,#44192,#44193,#44194,#44195,
#44196,#44197,#44198,#44199,#44200,#44201,#44202,#44203,#44204,#44205,#44206,
#44207,#44208,#44209,#44210,#44211,#44212,#44213,#44214,#44215,#44216,#44217,
#44218,#44219,#44220,#44221,#44222,#44223,#44224,#44225,#44226,#44227,#44228,
#44229,#44230,#44231,#44232,#44233,#44234,#44235,#44236,#44237,#44238,#44239,
#44240,#44241,#44242,#44243,#44244,#44245,#44246,#44247,#44248,#44249,#44250,
#44251,#44252,#44253,#44254,#44255,#44256,#44257,#44258,#44259,#44260,#44261,
#44262,#44263,#44264,#44265,#44266,#44267,#44268,#44269,#44270,#44271,#44272,
#44273,#44274,#44275,#44276),(#44277,#44278,#44279,#44280,#44281,#44282,
#44283,#44284,#44285,#44286,#44287,#44288,#44289,#44290,#44291,#44292,#44293,
#44294,#44295,#44296,#44297,#44298,#44299,#44300,#44301,#44302,#44303,#44304,
#44305,#44306,#44307,#44308,#44309,#44310,#44311,#44312,#44313,#44314,#44315,
#44316,#44317,#44318,#44319,#44320,#44321,#44322,#44323,#44324,#44325,#44326,
#44327,#44328,#44329,#44330,#44331,#44332,#44333,#44334,#44335,#44336,#44337,
#44338,#44339,#44340,#44341,#44342,#44343,#44344,#44345,#44346,#44347,#44348,
#44349,#44350,#44351,#44352,#44353,#44354,#44355,#44356,#44357,#44358,#44359,
#44360,#44361,#44362,#44363,#44364,#44365,#44366,#44367,#44368,#44369,#44370,
#44371,#44372,#44373,#44374,#44375,#44376,#44377,#44378,#44379,#44380,#44381,
#44382,#44383,#44384,#44385,#44386,#44387,#44388,#44389,#44390,#44391,#44392,
#44393,#44394,#44395,#44396,#44397,#44398,#44399,#44400,#44401,#44402,#44403,
#44404,#44405,#44406,#44407,#44408,#44409,#44410,#44411,#44412,#44413,#44414,
#44415,#44416,#44417,#44418,#44419,#44420),(#44421,#44422,#44423,#44424,
#44425,#44426,#44427,#44428,#44429,#44430,#44431,#44432,#44433,#44434,#44435,
#44436,#44437,#44438,#44439,#44440,#44441,#44442,#44443,#44444,#44445,#44446,
#44447,#44448,#44449,#44450,#44451,#44452,#44453,#44454,#44455,#44456,#44457,
#44458,#44459,#44460,#44461,#44462,#44463,#44464,#44465,#44466,#44467,#44468,
#44469,#44470,#44471,#44472,#44473,#44474,#44475,#44476,#44477,#44478,#44479,
#44480,#44481,#44482,#44483,#44484,#44485,#44486,#44487,#44488,#44489,#44490,
#44491,#44492,#44493,#44494,#44495,#44496,#44497,#44498,#44499,#44500,#44501,
#44502,#44503,#44504,#44505,#44506,#44507,#44508,#44509,#44510,#44511,#44512,
#44513,#44514,#44515,#44516,#44517,#44518,#44519,#44520,#44521,#44522,#44523,
#44524,#44525,#44526,#44527,#44528,#44529,#44530,#44531,#44532,#44533,#44534,
#44535,#44536,#44537,#44538,#44539,#44540,#44541,#44542,#44543,#44544,#44545,
#44546,#44547,#44548,#44549,#44550,#44551,#44552,#44553,#44554,#44555,#44556,
#44557,#44558,#44559,#44560,#44561,#44562,#44563,#44564),(#44565,#44566,
#44567,#44568,#44569,#44570,#44571,#44572,#44573,#44574,#44575,#44576,#44577,
#44578,#44579,#44580,#44581,#44582,#44583,#44584,#44585,#44586,#44587,#44588,
#44589,#44590,#44591,#44592,#44593,#44594,#44595,#44596,#44597,#44598,#44599,
#44600,#44601,#44602,#44603,#44604,#44605,#44606,#44607,#44608,#44609,#44610,
#44611,#44612,#44613,#44614,#44615,#44616,#44617,#44618,#44619,#44620,#44621,
#44622,#44623,#44624,#44625,#44626,#44627,#44628,#44629,#44630,#44631,#44632,
#44633,#44634,#44635,#44636,#44637,#44638,#44639,#44640,#44641,#44642,#44643,
#44644,#44645,#44646,#44647,#44648,#44649,#44650,#44651,#44652,#44653,#44654,
#44655,#44656,#44657,#44658,#44659,#44660,#44661,#44662,#44663,#44664,#44665,
#44666,#44667,#44668,#44669,#44670,#44671,#44672,#44673,#44674,#44675,#44676,
#44677,#44678,#44679,#44680,#44681,#44682,#44683,#44684,#44685,#44686,#44687,
#44688,#44689,#44690,#44691,#44692,#44693,#44694,#44695,#44696,#44697,#44698,
#44699,#44700,#44701,#44702,#44703,#44704,#44705,#44706,#44707,#44708),
(#44709,#44710,#44711,#44712,#44713,#44714,#44715,#44716,#44717,#44718,
#44719,#44720,#44721,#44722,#44723,#44724,#44725,#44726,#44727,#44728,#44729,
#44730,#44731,#44732,#44733,#44734,#44735,#44736,#44737,#44738,#44739,#44740,
#44741,#44742,#44743,#44744,#44745,#44746,#44747,#44748,#44749,#44750,#44751,
#44752,#44753,#44754,#44755,#44756,#44757,#44758,#44759,#44760,#44761,#44762,
#44763,#44764,#44765,#44766,#44767,#44768,#44769,#44770,#44771,#44772,#44773,
#44774,#44775,#44776,#44777,#44778,#44779,#44780,#44781,#44782,#44783,#44784,
#44785,#44786,#44787,#44788,#44789,#44790,#44791,#44792,#44793,#44794,#44795,
#44796,#44797,#44798,#44799,#44800,#44801,#44802,#44803,#44804,#44805,#44806,
#44807,#44808,#44809,#44810,#44811,#44812,#44813,#44814,#44815,#44816,#44817,
#44818,#44819,#44820,#44821,#44822,#44823,#44824,#44825,#44826,#44827,#44828,
#44829,#44830,#44831,#44832,#44833,#44834,#44835,#44836,#44837,#44838,#44839,
#44840,#44841,#44842,#44843,#44844,#44845,#44846,#44847,#44848,#44849,#44850,
#44851,#44852),(#44853,#44854,#44855,#44856,#44857,#44858,#44859,#44860,
#44861,#44862,#44863,#44864,#44865,#44866,#44867,#44868,#44869,#44870,#44871,
#44872,#44873,#44874,#44875,#44876,#44877,#44878,#44879,#44880,#44881,#44882,
#44883,#44884,#44885,#44886,#44887,#44888,#44889,#44890,#44891,#44892,#44893,
#44894,#44895,#44896,#44897,#44898,#44899,#44900,#44901,#44902,#44903,#44904,
#44905,#44906,#44907,#44908,#44909,#44910,#44911,#44912,#44913,#44914,#44915,
#44916,#44917,#44918,#44919,#44920,#44921,#44922,#44923,#44924,#44925,#44926,
#44927,#44928,#44929,#44930,#44931,#44932,#44933,#44934,#44935,#44936,#44937,
#44938,#44939,#44940,#44941,#44942,#44943,#44944,#44945,#44946,#44947,#44948,
#44949,#44950,#44951,#44952,#44953,#44954,#44955,#44956,#44957,#44958,#44959,
#44960,#44961,#44962,#44963,#44964,#44965,#44966,#44967,#44968,#44969,#44970,
#44971,#44972,#44973,#44974,#44975,#44976,#44977,#44978,#44979,#44980,#44981,
#44982,#44983,#44984,#44985,#44986,#44987,#44988,#44989,#44990,#44991,#44992,
#44993,#44994,#44995,#44996),(#44997,#44998,#44999,#45000,#45001,#45002,
#45003,#45004,#45005,#45006,#45007,#45008,#45009,#45010,#45011,#45012,#45013,
#45014,#45015,#45016,#45017,#45018,#45019,#45020,#45021,#45022,#45023,#45024,
#45025,#45026,#45027,#45028,#45029,#45030,#45031,#45032,#45033,#45034,#45035,
#45036,#45037,#45038,#45039,#45040,#45041,#45042,#45043,#45044,#45045,#45046,
#45047,#45048,#45049,#45050,#45051,#45052,#45053,#45054,#45055,#45056,#45057,
#45058,#45059,#45060,#45061,#45062,#45063,#45064,#45065,#45066,#45067,#45068,
#45069,#45070,#45071,#45072,#45073,#45074,#45075,#45076,#45077,#45078,#45079,
#45080,#45081,#45082,#45083,#45084,#45085,#45086,#45087,#45088,#45089,#45090,
#45091,#45092,#45093,#45094,#45095,#45096,#45097,#45098,#45099,#45100,#45101,
#45102,#45103,#45104,#45105,#45106,#45107,#45108,#45109,#45110,#45111,#45112,
#45113,#45114,#45115,#45116,#45117,#45118,#45119,#45120,#45121,#45122,#45123,
#45124,#45125,#45126,#45127,#45128,#45129,#45130,#45131,#45132,#45133,#45134,
#45135,#45136,#45137,#45138,#45139,#45140),(#45141,#45142,#45143,#45144,
#45145,#45146,#45147,#45148,#45149,#45150,#45151,#45152,#45153,#45154,#45155,
#45156,#45157,#45158,#45159,#45160,#45161,#45162,#45163,#45164,#45165,#45166,
#45167,#45168,#45169,#45170,#45171,#45172,#45173,#45174,#45175,#45176,#45177,
#45178,#45179,#45180,#45181,#45182,#45183,#45184,#45185,#45186,#45187,#45188,
#45189,#45190,#45191,#45192,#45193,#45194,#45195,#45196,#45197,#45198,#45199,
#45200,#45201,#45202,#45203,#45204,#45205,#45206,#45207,#45208,#45209,#45210,
#45211,#45212,#45213,#45214,#45215,#45216,#45217,#45218,#45219,#45220,#45221,
#45222,#45223,#45224,#45225,#45226,#45227,#45228,#45229,#45230,#45231,#45232,
#45233,#45234,#45235,#45236,#45237,#45238,#45239,#45240,#45241,#45242,#45243,
#45244,#45245,#45246,#45247,#45248,#45249,#45250,#45251,#45252,#45253,#45254,
#45255,#45256,#45257,#45258,#45259,#45260,#45261,#45262,#45263,#45264,#45265,
#45266,#45267,#45268,#45269,#45270,#45271,#45272,#45273,#45274,#45275,#45276,
#45277,#45278,#45279,#45280,#45281,#45282,#45283,#45284),(#45285,#45286,
#45287,#45288,#45289,#45290,#45291,#45292,#45293,#45294,#45295,#45296,#45297,
#45298,#45299,#45300,#45301,#45302,#45303,#45304,#45305,#45306,#45307,#45308,
#45309,#45310,#45311,#45312,#45313,#45314,#45315,#45316,#45317,#45318,#45319,
#45320,#45321,#45322,#45323,#45324,#45325,#45326,#45327,#45328,#45329,#45330,
#45331,#45332,#45333,#45334,#45335,#45336,#45337,#45338,#45339,#45340,#45341,
#45342,#45343,#45344,#45345,#45346,#45347,#45348,#45349,#45350,#45351,#45352,
#45353,#45354,#45355,#45356,#45357,#45358,#45359,#45360,#45361,#45362,#45363,
#45364,#45365,#45366,#45367,#45368,#45369,#45370,#45371,#45372,#45373,#45374,
#45375,#45376,#45377,#45378,#45379,#45380,#45381,#45382,#45383,#45384,#45385,
#45386,#45387,#45388,#45389,#45390,#45391,#45392,#45393,#45394,#45395,#45396,
#45397,#45398,#45399,#45400,#45401,#45402,#45403,#45404,#45405,#45406,#45407,
#45408,#45409,#45410,#45411,#45412,#45413,#45414,#45415,#45416,#45417,#45418,
#45419,#45420,#45421,#45422,#45423,#45424,#45425,#45426,#45427,#45428),
(#45429,#45430,#45431,#45432,#45433,#45434,#45435,#45436,#45437,#45438,
#45439,#45440,#45441,#45442,#45443,#45444,#45445,#45446,#45447,#45448,#45449,
#45450,#45451,#45452,#45453,#45454,#45455,#45456,#45457,#45458,#45459,#45460,
#45461,#45462,#45463,#45464,#45465,#45466,#45467,#45468,#45469,#45470,#45471,
#45472,#45473,#45474,#45475,#45476,#45477,#45478,#45479,#45480,#45481,#45482,
#45483,#45484,#45485,#45486,#45487,#45488,#45489,#45490,#45491,#45492,#45493,
#45494,#45495,#45496,#45497,#45498,#45499,#45500,#45501,#45502,#45503,#45504,
#45505,#45506,#45507,#45508,#45509,#45510,#45511,#45512,#45513,#45514,#45515,
#45516,#45517,#45518,#45519,#45520,#45521,#45522,#45523,#45524,#45525,#45526,
#45527,#45528,#45529,#45530,#45531,#45532,#45533,#45534,#45535,#45536,#45537,
#45538,#45539,#45540,#45541,#45542,#45543,#45544,#45545,#45546,#45547,#45548,
#45549,#45550,#45551,#45552,#45553,#45554,#45555,#45556,#45557,#45558,#45559,
#45560,#45561,#45562,#45563,#45564,#45565,#45566,#45567,#45568,#45569,#45570,
#45571,#45572),(#45573,#45574,#45575,#45576,#45577,#45578,#45579,#45580,
#45581,#45582,#45583,#45584,#45585,#45586,#45587,#45588,#45589,#45590,#45591,
#45592,#45593,#45594,#45595,#45596,#45597,#45598,#45599,#45600,#45601,#45602,
#45603,#45604,#45605,#45606,#45607,#45608,#45609,#45610,#45611,#45612,#45613,
#45614,#45615,#45616,#45617,#45618,#45619,#45620,#45621,#45622,#45623,#45624,
#45625,#45626,#45627,#45628,#45629,#45630,#45631,#45632,#45633,#45634,#45635,
#45636,#45637,#45638,#45639,#45640,#45641,#45642,#45643,#45644,#45645,#45646,
#45647,#45648,#45649,#45650,#45651,#45652,#45653,#45654,#45655,#45656,#45657,
#45658,#45659,#45660,#45661,#45662,#45663,#45664,#45665,#45666,#45667,#45668,
#45669,#45670,#45671,#45672,#45673,#45674,#45675,#45676,#45677,#45678,#45679,
#45680,#45681,#45682,#45683,#45684,#45685,#45686,#45687,#45688,#45689,#45690,
#45691,#45692,#45693,#45694,#45695,#45696,#45697,#45698,#45699,#45700,#45701,
#45702,#45703,#45704,#45705,#45706,#45707,#45708,#45709,#45710,#45711,#45712,
#45713,#45714,#45715,#45716),(#45717,#45718,#45719,#45720,#45721,#45722,
#45723,#45724,#45725,#45726,#45727,#45728,#45729,#45730,#45731,#45732,#45733,
#45734,#45735,#45736,#45737,#45738,#45739,#45740,#45741,#45742,#45743,#45744,
#45745,#45746,#45747,#45748,#45749,#45750,#45751,#45752,#45753,#45754,#45755,
#45756,#45757,#45758,#45759,#45760,#45761,#45762,#45763,#45764,#45765,#45766,
#45767,#45768,#45769,#45770,#45771,#45772,#45773,#45774,#45775,#45776,#45777,
#45778,#45779,#45780,#45781,#45782,#45783,#45784,#45785,#45786,#45787,#45788,
#45789,#45790,#45791,#45792,#45793,#45794,#45795,#45796,#45797,#45798,#45799,
#45800,#45801,#45802,#45803,#45804,#45805,#45806,#45807,#45808,#45809,#45810,
#45811,#45812,#45813,#45814,#45815,#45816,#45817,#45818,#45819,#45820,#45821,
#45822,#45823,#45824,#45825,#45826,#45827,#45828,#45829,#45830,#45831,#45832,
#45833,#45834,#45835,#45836,#45837,#45838,#45839,#45840,#45841,#45842,#45843,
#45844,#45845,#45846,#45847,#45848,#45849,#45850,#45851,#45852,#45853,#45854,
#45855,#45856,#45857,#45858,#45859,#45860),(#45861,#45862,#45863,#45864,
#45865,#45866,#45867,#45868,#45869,#45870,#45871,#45872,#45873,#45874,#45875,
#45876,#45877,#45878,#45879,#45880,#45881,#45882,#45883,#45884,#45885,#45886,
#45887,#45888,#45889,#45890,#45891,#45892,#45893,#45894,#45895,#45896,#45897,
#45898,#45899,#45900,#45901,#45902,#45903,#45904,#45905,#45906,#45907,#45908,
#45909,#45910,#45911,#45912,#45913,#45914,#45915,#45916,#45917,#45918,#45919,
#45920,#45921,#45922,#45923,#45924,#45925,#45926,#45927,#45928,#45929,#45930,
#45931,#45932,#45933,#45934,#45935,#45936,#45937,#45938,#45939,#45940,#45941,
#45942,#45943,#45944,#45945,#45946,#45947,#45948,#45949,#45950,#45951,#45952,
#45953,#45954,#45955,#45956,#45957,#45958,#45959,#45960,#45961,#45962,#45963,
#45964,#45965,#45966,#45967,#45968,#45969,#45970,#45971,#45972,#45973,#45974,
#45975,#45976,#45977,#45978,#45979,#45980,#45981,#45982,#45983,#45984,#45985,
#45986,#45987,#45988,#45989,#45990,#45991,#45992,#45993,#45994,#45995,#45996,
#45997,#45998,#45999,#46000,#46001,#46002,#46003,#46004),(#46005,#46006,
#46007,#46008,#46009,#46010,#46011,#46012,#46013,#46014,#46015,#46016,#46017,
#46018,#46019,#46020,#46021,#46022,#46023,#46024,#46025,#46026,#46027,#46028,
#46029,#46030,#46031,#46032,#46033,#46034,#46035,#46036,#46037,#46038,#46039,
#46040,#46041,#46042,#46043,#46044,#46045,#46046,#46047,#46048,#46049,#46050,
#46051,#46052,#46053,#46054,#46055,#46056,#46057,#46058,#46059,#46060,#46061,
#46062,#46063,#46064,#46065,#46066,#46067,#46068,#46069,#46070,#46071,#46072,
#46073,#46074,#46075,#46076,#46077,#46078,#46079,#46080,#46081,#46082,#46083,
#46084,#46085,#46086,#46087,#46088,#46089,#46090,#46091,#46092,#46093,#46094,
#46095,#46096,#46097,#46098,#46099,#46100,#46101,#46102,#46103,#46104,#46105,
#46106,#46107,#46108,#46109,#46110,#46111,#46112,#46113,#46114,#46115,#46116,
#46117,#46118,#46119,#46120,#46121,#46122,#46123,#46124,#46125,#46126,#46127,
#46128,#46129,#46130,#46131,#46132,#46133,#46134,#46135,#46136,#46137,#46138,
#46139,#46140,#46141,#46142,#46143,#46144,#46145,#46146,#46147,#46148),
(#46149,#46150,#46151,#46152,#46153,#46154,#46155,#46156,#46157,#46158,
#46159,#46160,#46161,#46162,#46163,#46164,#46165,#46166,#46167,#46168,#46169,
#46170,#46171,#46172,#46173,#46174,#46175,#46176,#46177,#46178,#46179,#46180,
#46181,#46182,#46183,#46184,#46185,#46186,#46187,#46188,#46189,#46190,#46191,
#46192,#46193,#46194,#46195,#46196,#46197,#46198,#46199,#46200,#46201,#46202,
#46203,#46204,#46205,#46206,#46207,#46208,#46209,#46210,#46211,#46212,#46213,
#46214,#46215,#46216,#46217,#46218,#46219,#46220,#46221,#46222,#46223,#46224,
#46225,#46226,#46227,#46228,#46229,#46230,#46231,#46232,#46233,#46234,#46235,
#46236,#46237,#46238,#46239,#46240,#46241,#46242,#46243,#46244,#46245,#46246,
#46247,#46248,#46249,#46250,#46251,#46252,#46253,#46254,#46255,#46256,#46257,
#46258,#46259,#46260,#46261,#46262,#46263,#46264,#46265,#46266,#46267,#46268,
#46269,#46270,#46271,#46272,#46273,#46274,#46275,#46276,#46277,#46278,#46279,
#46280,#46281,#46282,#46283,#46284,#46285,#46286,#46287,#46288,#46289,#46290,
#46291,#46292),(#46293,#46294,#46295,#46296,#46297,#46298,#46299,#46300,
#46301,#46302,#46303,#46304,#46305,#46306,#46307,#46308,#46309,#46310,#46311,
#46312,#46313,#46314,#46315,#46316,#46317,#46318,#46319,#46320,#46321,#46322,
#46323,#46324,#46325,#46326,#46327,#46328,#46329,#46330,#46331,#46332,#46333,
#46334,#46335,#46336,#46337,#46338,#46339,#46340,#46341,#46342,#46343,#46344,
#46345,#46346,#46347,#46348,#46349,#46350,#46351,#46352,#46353,#46354,#46355,
#46356,#46357,#46358,#46359,#46360,#46361,#46362,#46363,#46364,#46365,#46366,
#46367,#46368,#46369,#46370,#46371,#46372,#46373,#46374,#46375,#46376,#46377,
#46378,#46379,#46380,#46381,#46382,#46383,#46384,#46385,#46386,#46387,#46388,
#46389,#46390,#46391,#46392,#46393,#46394,#46395,#46396,#46397,#46398,#46399,
#46400,#46401,#46402,#46403,#46404,#46405,#46406,#46407,#46408,#46409,#46410,
#46411,#46412,#46413,#46414,#46415,#46416,#46417,#46418,#46419,#46420,#46421,
#46422,#46423,#46424,#46425,#46426,#46427,#46428,#46429,#46430,#46431,#46432,
#46433,#46434,#46435,#46436),(#46437,#46438,#46439,#46440,#46441,#46442,
#46443,#46444,#46445,#46446,#46447,#46448,#46449,#46450,#46451,#46452,#46453,
#46454,#46455,#46456,#46457,#46458,#46459,#46460,#46461,#46462,#46463,#46464,
#46465,#46466,#46467,#46468,#46469,#46470,#46471,#46472,#46473,#46474,#46475,
#46476,#46477,#46478,#46479,#46480,#46481,#46482,#46483,#46484,#46485,#46486,
#46487,#46488,#46489,#46490,#46491,#46492,#46493,#46494,#46495,#46496,#46497,
#46498,#46499,#46500,#46501,#46502,#46503,#46504,#46505,#46506,#46507,#46508,
#46509,#46510,#46511,#46512,#46513,#46514,#46515,#46516,#46517,#46518,#46519,
#46520,#46521,#46522,#46523,#46524,#46525,#46526,#46527,#46528,#46529,#46530,
#46531,#46532,#46533,#46534,#46535,#46536,#46537,#46538,#46539,#46540,#46541,
#46542,#46543,#46544,#46545,#46546,#46547,#46548,#46549,#46550,#46551,#46552,
#46553,#46554,#46555,#46556,#46557,#46558,#46559,#46560,#46561,#46562,#46563,
#46564,#46565,#46566,#46567,#46568,#46569,#46570,#46571,#46572,#46573,#46574,
#46575,#46576,#46577,#46578,#46579,#46580),(#46581,#46582,#46583,#46584,
#46585,#46586,#46587,#46588,#46589,#46590,#46591,#46592,#46593,#46594,#46595,
#46596,#46597,#46598,#46599,#46600,#46601,#46602,#46603,#46604,#46605,#46606,
#46607,#46608,#46609,#46610,#46611,#46612,#46613,#46614,#46615,#46616,#46617,
#46618,#46619,#46620,#46621,#46622,#46623,#46624,#46625,#46626,#46627,#46628,
#46629,#46630,#46631,#46632,#46633,#46634,#46635,#46636,#46637,#46638,#46639,
#46640,#46641,#46642,#46643,#46644,#46645,#46646,#46647,#46648,#46649,#46650,
#46651,#46652,#46653,#46654,#46655,#46656,#46657,#46658,#46659,#46660,#46661,
#46662,#46663,#46664,#46665,#46666,#46667,#46668,#46669,#46670,#46671,#46672,
#46673,#46674,#46675,#46676,#46677,#46678,#46679,#46680,#46681,#46682,#46683,
#46684,#46685,#46686,#46687,#46688,#46689,#46690,#46691,#46692,#46693,#46694,
#46695,#46696,#46697,#46698,#46699,#46700,#46701,#46702,#46703,#46704,#46705,
#46706,#46707,#46708,#46709,#46710,#46711,#46712,#46713,#46714,#46715,#46716,
#46717,#46718,#46719,#46720,#46721,#46722,#46723,#46724),(#46725,#46726,
#46727,#46728,#46729,#46730,#46731,#46732,#46733,#46734,#46735,#46736,#46737,
#46738,#46739,#46740,#46741,#46742,#46743,#46744,#46745,#46746,#46747,#46748,
#46749,#46750,#46751,#46752,#46753,#46754,#46755,#46756,#46757,#46758,#46759,
#46760,#46761,#46762,#46763,#46764,#46765,#46766,#46767,#46768,#46769,#46770,
#46771,#46772,#46773,#46774,#46775,#46776,#46777,#46778,#46779,#46780,#46781,
#46782,#46783,#46784,#46785,#46786,#46787,#46788,#46789,#46790,#46791,#46792,
#46793,#46794,#46795,#46796,#46797,#46798,#46799,#46800,#46801,#46802,#46803,
#46804,#46805,#46806,#46807,#46808,#46809,#46810,#46811,#46812,#46813,#46814,
#46815,#46816,#46817,#46818,#46819,#46820,#46821,#46822,#46823,#46824,#46825,
#46826,#46827,#46828,#46829,#46830,#46831,#46832,#46833,#46834,#46835,#46836,
#46837,#46838,#46839,#46840,#46841,#46842,#46843,#46844,#46845,#46846,#46847,
#46848,#46849,#46850,#46851,#46852,#46853,#46854,#46855,#46856,#46857,#46858,
#46859,#46860,#46861,#46862,#46863,#46864,#46865,#46866,#46867,#46868),
(#46869,#46870,#46871,#46872,#46873,#46874,#46875,#46876,#46877,#46878,
#46879,#46880,#46881,#46882,#46883,#46884,#46885,#46886,#46887,#46888,#46889,
#46890,#46891,#46892,#46893,#46894,#46895,#46896,#46897,#46898,#46899,#46900,
#46901,#46902,#46903,#46904,#46905,#46906,#46907,#46908,#46909,#46910,#46911,
#46912,#46913,#46914,#46915,#46916,#46917,#46918,#46919,#46920,#46921,#46922,
#46923,#46924,#46925,#46926,#46927,#46928,#46929,#46930,#46931,#46932,#46933,
#46934,#46935,#46936,#46937,#46938,#46939,#46940,#46941,#46942,#46943,#46944,
#46945,#46946,#46947,#46948,#46949,#46950,#46951,#46952,#46953,#46954,#46955,
#46956,#46957,#46958,#46959,#46960,#46961,#46962,#46963,#46964,#46965,#46966,
#46967,#46968,#46969,#46970,#46971,#46972,#46973,#46974,#46975,#46976,#46977,
#46978,#46979,#46980,#46981,#46982,#46983,#46984,#46985,#46986,#46987,#46988,
#46989,#46990,#46991,#46992,#46993,#46994,#46995,#46996,#46997,#46998,#46999,
#47000,#47001,#47002,#47003,#47004,#47005,#47006,#47007,#47008,#47009,#47010,
#47011,#47012),(#47013,#47014,#47015,#47016,#47017,#47018,#47019,#47020,
#47021,#47022,#47023,#47024,#47025,#47026,#47027,#47028,#47029,#47030,#47031,
#47032,#47033,#47034,#47035,#47036,#47037,#47038,#47039,#47040,#47041,#47042,
#47043,#47044,#47045,#47046,#47047,#47048,#47049,#47050,#47051,#47052,#47053,
#47054,#47055,#47056,#47057,#47058,#47059,#47060,#47061,#47062,#47063,#47064,
#47065,#47066,#47067,#47068,#47069,#47070,#47071,#47072,#47073,#47074,#47075,
#47076,#47077,#47078,#47079,#47080,#47081,#47082,#47083,#47084,#47085,#47086,
#47087,#47088,#47089,#47090,#47091,#47092,#47093,#47094,#47095,#47096,#47097,
#47098,#47099,#47100,#47101,#47102,#47103,#47104,#47105,#47106,#47107,#47108,
#47109,#47110,#47111,#47112,#47113,#47114,#47115,#47116,#47117,#47118,#47119,
#47120,#47121,#47122,#47123,#47124,#47125,#47126,#47127,#47128,#47129,#47130,
#47131,#47132,#47133,#47134,#47135,#47136,#47137,#47138,#47139,#47140,#47141,
#47142,#47143,#47144,#47145,#47146,#47147,#47148,#47149,#47150,#47151,#47152,
#47153,#47154,#47155,#47156),(#47157,#47158,#47159,#47160,#47161,#47162,
#47163,#47164,#47165,#47166,#47167,#47168,#47169,#47170,#47171,#47172,#47173,
#47174,#47175,#47176,#47177,#47178,#47179,#47180,#47181,#47182,#47183,#47184,
#47185,#47186,#47187,#47188,#47189,#47190,#47191,#47192,#47193,#47194,#47195,
#47196,#47197,#47198,#47199,#47200,#47201,#47202,#47203,#47204,#47205,#47206,
#47207,#47208,#47209,#47210,#47211,#47212,#47213,#47214,#47215,#47216,#47217,
#47218,#47219,#47220,#47221,#47222,#47223,#47224,#47225,#47226,#47227,#47228,
#47229,#47230,#47231,#47232,#47233,#47234,#47235,#47236,#47237,#47238,#47239,
#47240,#47241,#47242,#47243,#47244,#47245,#47246,#47247,#47248,#47249,#47250,
#47251,#47252,#47253,#47254,#47255,#47256,#47257,#47258,#47259,#47260,#47261,
#47262,#47263,#47264,#47265,#47266,#47267,#47268,#47269,#47270,#47271,#47272,
#47273,#47274,#47275,#47276,#47277,#47278,#47279,#47280,#47281,#47282,#47283,
#47284,#47285,#47286,#47287,#47288,#47289,#47290,#47291,#47292,#47293,#47294,
#47295,#47296,#47297,#47298,#47299,#47300),(#47301,#47302,#47303,#47304,
#47305,#47306,#47307,#47308,#47309,#47310,#47311,#47312,#47313,#47314,#47315,
#47316,#47317,#47318,#47319,#47320,#47321,#47322,#47323,#47324,#47325,#47326,
#47327,#47328,#47329,#47330,#47331,#47332,#47333,#47334,#47335,#47336,#47337,
#47338,#47339,#47340,#47341,#47342,#47343,#47344,#47345,#47346,#47347,#47348,
#47349,#47350,#47351,#47352,#47353,#47354,#47355,#47356,#47357,#47358,#47359,
#47360,#47361,#47362,#47363,#47364,#47365,#47366,#47367,#47368,#47369,#47370,
#47371,#47372,#47373,#47374,#47375,#47376,#47377,#47378,#47379,#47380,#47381,
#47382,#47383,#47384,#47385,#47386,#47387,#47388,#47389,#47390,#47391,#47392,
#47393,#47394,#47395,#47396,#47397,#47398,#47399,#47400,#47401,#47402,#47403,
#47404,#47405,#47406,#47407,#47408,#47409,#47410,#47411,#47412,#47413,#47414,
#47415,#47416,#47417,#47418,#47419,#47420,#47421,#47422,#47423,#47424,#47425,
#47426,#47427,#47428,#47429,#47430,#47431,#47432,#47433,#47434,#47435,#47436,
#47437,#47438,#47439,#47440,#47441,#47442,#47443,#47444),(#47445,#47446,
#47447,#47448,#47449,#47450,#47451,#47452,#47453,#47454,#47455,#47456,#47457,
#47458,#47459,#47460,#47461,#47462,#47463,#47464,#47465,#47466,#47467,#47468,
#47469,#47470,#47471,#47472,#47473,#47474,#47475,#47476,#47477,#47478,#47479,
#47480,#47481,#47482,#47483,#47484,#47485,#47486,#47487,#47488,#47489,#47490,
#47491,#47492,#47493,#47494,#47495,#47496,#47497,#47498,#47499,#47500,#47501,
#47502,#47503,#47504,#47505,#47506,#47507,#47508,#47509,#47510,#47511,#47512,
#47513,#47514,#47515,#47516,#47517,#47518,#47519,#47520,#47521,#47522,#47523,
#47524,#47525,#47526,#47527,#47528,#47529,#47530,#47531,#47532,#47533,#47534,
#47535,#47536,#47537,#47538,#47539,#47540,#47541,#47542,#47543,#47544,#47545,
#47546,#47547,#47548,#47549,#47550,#47551,#47552,#47553,#47554,#47555,#47556,
#47557,#47558,#47559,#47560,#47561,#47562,#47563,#47564,#47565,#47566,#47567,
#47568,#47569,#47570,#47571,#47572,#47573,#47574,#47575,#47576,#47577,#47578,
#47579,#47580,#47581,#47582,#47583,#47584,#47585,#47586,#47587,#47588),
(#47589,#47590,#47591,#47592,#47593,#47594,#47595,#47596,#47597,#47598,
#47599,#47600,#47601,#47602,#47603,#47604,#47605,#47606,#47607,#47608,#47609,
#47610,#47611,#47612,#47613,#47614,#47615,#47616,#47617,#47618,#47619,#47620,
#47621,#47622,#47623,#47624,#47625,#47626,#47627,#47628,#47629,#47630,#47631,
#47632,#47633,#47634,#47635,#47636,#47637,#47638,#47639,#47640,#47641,#47642,
#47643,#47644,#47645,#47646,#47647,#47648,#47649,#47650,#47651,#47652,#47653,
#47654,#47655,#47656,#47657,#47658,#47659,#47660,#47661,#47662,#47663,#47664,
#47665,#47666,#47667,#47668,#47669,#47670,#47671,#47672,#47673,#47674,#47675,
#47676,#47677,#47678,#47679,#47680,#47681,#47682,#47683,#47684,#47685,#47686,
#47687,#47688,#47689,#47690,#47691,#47692,#47693,#47694,#47695,#47696,#47697,
#47698,#47699,#47700,#47701,#47702,#47703,#47704,#47705,#47706,#47707,#47708,
#47709,#47710,#47711,#47712,#47713,#47714,#47715,#47716,#47717,#47718,#47719,
#47720,#47721,#47722,#47723,#47724,#47725,#47726,#47727,#47728,#47729,#47730,
#47731,#47732),(#47733,#47734,#47735,#47736,#47737,#47738,#47739,#47740,
#47741,#47742,#47743,#47744,#47745,#47746,#47747,#47748,#47749,#47750,#47751,
#47752,#47753,#47754,#47755,#47756,#47757,#47758,#47759,#47760,#47761,#47762,
#47763,#47764,#47765,#47766,#47767,#47768,#47769,#47770,#47771,#47772,#47773,
#47774,#47775,#47776,#47777,#47778,#47779,#47780,#47781,#47782,#47783,#47784,
#47785,#47786,#47787,#47788,#47789,#47790,#47791,#47792,#47793,#47794,#47795,
#47796,#47797,#47798,#47799,#47800,#47801,#47802,#47803,#47804,#47805,#47806,
#47807,#47808,#47809,#47810,#47811,#47812,#47813,#47814,#47815,#47816,#47817,
#47818,#47819,#47820,#47821,#47822,#47823,#47824,#47825,#47826,#47827,#47828,
#47829,#47830,#47831,#47832,#47833,#47834,#47835,#47836,#47837,#47838,#47839,
#47840,#47841,#47842,#47843,#47844,#47845,#47846,#47847,#47848,#47849,#47850,
#47851,#47852,#47853,#47854,#47855,#47856,#47857,#47858,#47859,#47860,#47861,
#47862,#47863,#47864,#47865,#47866,#47867,#47868,#47869,#47870,#47871,#47872,
#47873,#47874,#47875,#47876),(#47877,#47878,#47879,#47880,#47881,#47882,
#47883,#47884,#47885,#47886,#47887,#47888,#47889,#47890,#47891,#47892,#47893,
#47894,#47895,#47896,#47897,#47898,#47899,#47900,#47901,#47902,#47903,#47904,
#47905,#47906,#47907,#47908,#47909,#47910,#47911,#47912,#47913,#47914,#47915,
#47916,#47917,#47918,#47919,#47920,#47921,#47922,#47923,#47924,#47925,#47926,
#47927,#47928,#47929,#47930,#47931,#47932,#47933,#47934,#47935,#47936,#47937,
#47938,#47939,#47940,#47941,#47942,#47943,#47944,#47945,#47946,#47947,#47948,
#47949,#47950,#47951,#47952,#47953,#47954,#47955,#47956,#47957,#47958,#47959,
#47960,#47961,#47962,#47963,#47964,#47965,#47966,#47967,#47968,#47969,#47970,
#47971,#47972,#47973,#47974,#47975,#47976,#47977,#47978,#47979,#47980,#47981,
#47982,#47983,#47984,#47985,#47986,#47987,#47988,#47989,#47990,#47991,#47992,
#47993,#47994,#47995,#47996,#47997,#47998,#47999,#48000,#48001,#48002,#48003,
#48004,#48005,#48006,#48007,#48008,#48009,#48010,#48011,#48012,#48013,#48014,
#48015,#48016,#48017,#48018,#48019,#48020),(#48021,#48022,#48023,#48024,
#48025,#48026,#48027,#48028,#48029,#48030,#48031,#48032,#48033,#48034,#48035,
#48036,#48037,#48038,#48039,#48040,#48041,#48042,#48043,#48044,#48045,#48046,
#48047,#48048,#48049,#48050,#48051,#48052,#48053,#48054,#48055,#48056,#48057,
#48058,#48059,#48060,#48061,#48062,#48063,#48064,#48065,#48066,#48067,#48068,
#48069,#48070,#48071,#48072,#48073,#48074,#48075,#48076,#48077,#48078,#48079,
#48080,#48081,#48082,#48083,#48084,#48085,#48086,#48087,#48088,#48089,#48090,
#48091,#48092,#48093,#48094,#48095,#48096,#48097,#48098,#48099,#48100,#48101,
#48102,#48103,#48104,#48105,#48106,#48107,#48108,#48109,#48110,#48111,#48112,
#48113,#48114,#48115,#48116,#48117,#48118,#48119,#48120,#48121,#48122,#48123,
#48124,#48125,#48126,#48127,#48128,#48129,#48130,#48131,#48132,#48133,#48134,
#48135,#48136,#48137,#48138,#48139,#48140,#48141,#48142,#48143,#48144,#48145,
#48146,#48147,#48148,#48149,#48150,#48151,#48152,#48153,#48154,#48155,#48156,
#48157,#48158,#48159,#48160,#48161,#48162,#48163,#48164),(#48165,#48166,
#48167,#48168,#48169,#48170,#48171,#48172,#48173,#48174,#48175,#48176,#48177,
#48178,#48179,#48180,#48181,#48182,#48183,#48184,#48185,#48186,#48187,#48188,
#48189,#48190,#48191,#48192,#48193,#48194,#48195,#48196,#48197,#48198,#48199,
#48200,#48201,#48202,#48203,#48204,#48205,#48206,#48207,#48208,#48209,#48210,
#48211,#48212,#48213,#48214,#48215,#48216,#48217,#48218,#48219,#48220,#48221,
#48222,#48223,#48224,#48225,#48226,#48227,#48228,#48229,#48230,#48231,#48232,
#48233,#48234,#48235,#48236,#48237,#48238,#48239,#48240,#48241,#48242,#48243,
#48244,#48245,#48246,#48247,#48248,#48249,#48250,#48251,#48252,#48253,#48254,
#48255,#48256,#48257,#48258,#48259,#48260,#48261,#48262,#48263,#48264,#48265,
#48266,#48267,#48268,#48269,#48270,#48271,#48272,#48273,#48274,#48275,#48276,
#48277,#48278,#48279,#48280,#48281,#48282,#48283,#48284,#48285,#48286,#48287,
#48288,#48289,#48290,#48291,#48292,#48293,#48294,#48295,#48296,#48297,#48298,
#48299,#48300,#48301,#48302,#48303,#48304,#48305,#48306,#48307,#48308),
(#48309,#48310,#48311,#48312,#48313,#48314,#48315,#48316,#48317,#48318,
#48319,#48320,#48321,#48322,#48323,#48324,#48325,#48326,#48327,#48328,#48329,
#48330,#48331,#48332,#48333,#48334,#48335,#48336,#48337,#48338,#48339,#48340,
#48341,#48342,#48343,#48344,#48345,#48346,#48347,#48348,#48349,#48350,#48351,
#48352,#48353,#48354,#48355,#48356,#48357,#48358,#48359,#48360,#48361,#48362,
#48363,#48364,#48365,#48366,#48367,#48368,#48369,#48370,#48371,#48372,#48373,
#48374,#48375,#48376,#48377,#48378,#48379,#48380,#48381,#48382,#48383,#48384,
#48385,#48386,#48387,#48388,#48389,#48390,#48391,#48392,#48393,#48394,#48395,
#48396,#48397,#48398,#48399,#48400,#48401,#48402,#48403,#48404,#48405,#48406,
#48407,#48408,#48409,#48410,#48411,#48412,#48413,#48414,#48415,#48416,#48417,
#48418,#48419,#48420,#48421,#48422,#48423,#48424,#48425,#48426,#48427,#48428,
#48429,#48430,#48431,#48432,#48433,#48434,#48435,#48436,#48437,#48438,#48439,
#48440,#48441,#48442,#48443,#48444,#48445,#48446,#48447,#48448,#48449,#48450,
#48451,#48452),(#48453,#48454,#48455,#48456,#48457,#48458,#48459,#48460,
#48461,#48462,#48463,#48464,#48465,#48466,#48467,#48468,#48469,#48470,#48471,
#48472,#48473,#48474,#48475,#48476,#48477,#48478,#48479,#48480,#48481,#48482,
#48483,#48484,#48485,#48486,#48487,#48488,#48489,#48490,#48491,#48492,#48493,
#48494,#48495,#48496,#48497,#48498,#48499,#48500,#48501,#48502,#48503,#48504,
#48505,#48506,#48507,#48508,#48509,#48510,#48511,#48512,#48513,#48514,#48515,
#48516,#48517,#48518,#48519,#48520,#48521,#48522,#48523,#48524,#48525,#48526,
#48527,#48528,#48529,#48530,#48531,#48532,#48533,#48534,#48535,#48536,#48537,
#48538,#48539,#48540,#48541,#48542,#48543,#48544,#48545,#48546,#48547,#48548,
#48549,#48550,#48551,#48552,#48553,#48554,#48555,#48556,#48557,#48558,#48559,
#48560,#48561,#48562,#48563,#48564,#48565,#48566,#48567,#48568,#48569,#48570,
#48571,#48572,#48573,#48574,#48575,#48576,#48577,#48578,#48579,#48580,#48581,
#48582,#48583,#48584,#48585,#48586,#48587,#48588,#48589,#48590,#48591,#48592,
#48593,#48594,#48595,#48596),(#48597,#48598,#48599,#48600,#48601,#48602,
#48603,#48604,#48605,#48606,#48607,#48608,#48609,#48610,#48611,#48612,#48613,
#48614,#48615,#48616,#48617,#48618,#48619,#48620,#48621,#48622,#48623,#48624,
#48625,#48626,#48627,#48628,#48629,#48630,#48631,#48632,#48633,#48634,#48635,
#48636,#48637,#48638,#48639,#48640,#48641,#48642,#48643,#48644,#48645,#48646,
#48647,#48648,#48649,#48650,#48651,#48652,#48653,#48654,#48655,#48656,#48657,
#48658,#48659,#48660,#48661,#48662,#48663,#48664,#48665,#48666,#48667,#48668,
#48669,#48670,#48671,#48672,#48673,#48674,#48675,#48676,#48677,#48678,#48679,
#48680,#48681,#48682,#48683,#48684,#48685,#48686,#48687,#48688,#48689,#48690,
#48691,#48692,#48693,#48694,#48695,#48696,#48697,#48698,#48699,#48700,#48701,
#48702,#48703,#48704,#48705,#48706,#48707,#48708,#48709,#48710,#48711,#48712,
#48713,#48714,#48715,#48716,#48717,#48718,#48719,#48720,#48721,#48722,#48723,
#48724,#48725,#48726,#48727,#48728,#48729,#48730,#48731,#48732,#48733,#48734,
#48735,#48736,#48737,#48738,#48739,#48740),(#48741,#48742,#48743,#48744,
#48745,#48746,#48747,#48748,#48749,#48750,#48751,#48752,#48753,#48754,#48755,
#48756,#48757,#48758,#48759,#48760,#48761,#48762,#48763,#48764,#48765,#48766,
#48767,#48768,#48769,#48770,#48771,#48772,#48773,#48774,#48775,#48776,#48777,
#48778,#48779,#48780,#48781,#48782,#48783,#48784,#48785,#48786,#48787,#48788,
#48789,#48790,#48791,#48792,#48793,#48794,#48795,#48796,#48797,#48798,#48799,
#48800,#48801,#48802,#48803,#48804,#48805,#48806,#48807,#48808,#48809,#48810,
#48811,#48812,#48813,#48814,#48815,#48816,#48817,#48818,#48819,#48820,#48821,
#48822,#48823,#48824,#48825,#48826,#48827,#48828,#48829,#48830,#48831,#48832,
#48833,#48834,#48835,#48836,#48837,#48838,#48839,#48840,#48841,#48842,#48843,
#48844,#48845,#48846,#48847,#48848,#48849,#48850,#48851,#48852,#48853,#48854,
#48855,#48856,#48857,#48858,#48859,#48860,#48861,#48862,#48863,#48864,#48865,
#48866,#48867,#48868,#48869,#48870,#48871,#48872,#48873,#48874,#48875,#48876,
#48877,#48878,#48879,#48880,#48881,#48882,#48883,#48884),(#48885,#48886,
#48887,#48888,#48889,#48890,#48891,#48892,#48893,#48894,#48895,#48896,#48897,
#48898,#48899,#48900,#48901,#48902,#48903,#48904,#48905,#48906,#48907,#48908,
#48909,#48910,#48911,#48912,#48913,#48914,#48915,#48916,#48917,#48918,#48919,
#48920,#48921,#48922,#48923,#48924,#48925,#48926,#48927,#48928,#48929,#48930,
#48931,#48932,#48933,#48934,#48935,#48936,#48937,#48938,#48939,#48940,#48941,
#48942,#48943,#48944,#48945,#48946,#48947,#48948,#48949,#48950,#48951,#48952,
#48953,#48954,#48955,#48956,#48957,#48958,#48959,#48960,#48961,#48962,#48963,
#48964,#48965,#48966,#48967,#48968,#48969,#48970,#48971,#48972,#48973,#48974,
#48975,#48976,#48977,#48978,#48979,#48980,#48981,#48982,#48983,#48984,#48985,
#48986,#48987,#48988,#48989,#48990,#48991,#48992,#48993,#48994,#48995,#48996,
#48997,#48998,#48999,#49000,#49001,#49002,#49003,#49004,#49005,#49006,#49007,
#49008,#49009,#49010,#49011,#49012,#49013,#49014,#49015,#49016,#49017,#49018,
#49019,#49020,#49021,#49022,#49023,#49024,#49025,#49026,#49027,#49028),
(#49029,#49030,#49031,#49032,#49033,#49034,#49035,#49036,#49037,#49038,
#49039,#49040,#49041,#49042,#49043,#49044,#49045,#49046,#49047,#49048,#49049,
#49050,#49051,#49052,#49053,#49054,#49055,#49056,#49057,#49058,#49059,#49060,
#49061,#49062,#49063,#49064,#49065,#49066,#49067,#49068,#49069,#49070,#49071,
#49072,#49073,#49074,#49075,#49076,#49077,#49078,#49079,#49080,#49081,#49082,
#49083,#49084,#49085,#49086,#49087,#49088,#49089,#49090,#49091,#49092,#49093,
#49094,#49095,#49096,#49097,#49098,#49099,#49100,#49101,#49102,#49103,#49104,
#49105,#49106,#49107,#49108,#49109,#49110,#49111,#49112,#49113,#49114,#49115,
#49116,#49117,#49118,#49119,#49120,#49121,#49122,#49123,#49124,#49125,#49126,
#49127,#49128,#49129,#49130,#49131,#49132,#49133,#49134,#49135,#49136,#49137,
#49138,#49139,#49140,#49141,#49142,#49143,#49144,#49145,#49146,#49147,#49148,
#49149,#49150,#49151,#49152,#49153,#49154,#49155,#49156,#49157,#49158,#49159,
#49160,#49161,#49162,#49163,#49164,#49165,#49166,#49167,#49168,#49169,#49170,
#49171,#49172),(#49173,#49174,#49175,#49176,#49177,#49178,#49179,#49180,
#49181,#49182,#49183,#49184,#49185,#49186,#49187,#49188,#49189,#49190,#49191,
#49192,#49193,#49194,#49195,#49196,#49197,#49198,#49199,#49200,#49201,#49202,
#49203,#49204,#49205,#49206,#49207,#49208,#49209,#49210,#49211,#49212,#49213,
#49214,#49215,#49216,#49217,#49218,#49219,#49220,#49221,#49222,#49223,#49224,
#49225,#49226,#49227,#49228,#49229,#49230,#49231,#49232,#49233,#49234,#49235,
#49236,#49237,#49238,#49239,#49240,#49241,#49242,#49243,#49244,#49245,#49246,
#49247,#49248,#49249,#49250,#49251,#49252,#49253,#49254,#49255,#49256,#49257,
#49258,#49259,#49260,#49261,#49262,#49263,#49264,#49265,#49266,#49267,#49268,
#49269,#49270,#49271,#49272,#49273,#49274,#49275,#49276,#49277,#49278,#49279,
#49280,#49281,#49282,#49283,#49284,#49285,#49286,#49287,#49288,#49289,#49290,
#49291,#49292,#49293,#49294,#49295,#49296,#49297,#49298,#49299,#49300,#49301,
#49302,#49303,#49304,#49305,#49306,#49307,#49308,#49309,#49310,#49311,#49312,
#49313,#49314,#49315,#49316),(#49317,#49318,#49319,#49320,#49321,#49322,
#49323,#49324,#49325,#49326,#49327,#49328,#49329,#49330,#49331,#49332,#49333,
#49334,#49335,#49336,#49337,#49338,#49339,#49340,#49341,#49342,#49343,#49344,
#49345,#49346,#49347,#49348,#49349,#49350,#49351,#49352,#49353,#49354,#49355,
#49356,#49357,#49358,#49359,#49360,#49361,#49362,#49363,#49364,#49365,#49366,
#49367,#49368,#49369,#49370,#49371,#49372,#49373,#49374,#49375,#49376,#49377,
#49378,#49379,#49380,#49381,#49382,#49383,#49384,#49385,#49386,#49387,#49388,
#49389,#49390,#49391,#49392,#49393,#49394,#49395,#49396,#49397,#49398,#49399,
#49400,#49401,#49402,#49403,#49404,#49405,#49406,#49407,#49408,#49409,#49410,
#49411,#49412,#49413,#49414,#49415,#49416,#49417,#49418,#49419,#49420,#49421,
#49422,#49423,#49424,#49425,#49426,#49427,#49428,#49429,#49430,#49431,#49432,
#49433,#49434,#49435,#49436,#49437,#49438,#49439,#49440,#49441,#49442,#49443,
#49444,#49445,#49446,#49447,#49448,#49449,#49450,#49451,#49452,#49453,#49454,
#49455,#49456,#49457,#49458,#49459,#49460),(#49461,#49462,#49463,#49464,
#49465,#49466,#49467,#49468,#49469,#49470,#49471,#49472,#49473,#49474,#49475,
#49476,#49477,#49478,#49479,#49480,#49481,#49482,#49483,#49484,#49485,#49486,
#49487,#49488,#49489,#49490,#49491,#49492,#49493,#49494,#49495,#49496,#49497,
#49498,#49499,#49500,#49501,#49502,#49503,#49504,#49505,#49506,#49507,#49508,
#49509,#49510,#49511,#49512,#49513,#49514,#49515,#49516,#49517,#49518,#49519,
#49520,#49521,#49522,#49523,#49524,#49525,#49526,#49527,#49528,#49529,#49530,
#49531,#49532,#49533,#49534,#49535,#49536,#49537,#49538,#49539,#49540,#49541,
#49542,#49543,#49544,#49545,#49546,#49547,#49548,#49549,#49550,#49551,#49552,
#49553,#49554,#49555,#49556,#49557,#49558,#49559,#49560,#49561,#49562,#49563,
#49564,#49565,#49566,#49567,#49568,#49569,#49570,#49571,#49572,#49573,#49574,
#49575,#49576,#49577,#49578,#49579,#49580,#49581,#49582,#49583,#49584,#49585,
#49586,#49587,#49588,#49589,#49590,#49591,#49592,#49593,#49594,#49595,#49596,
#49597,#49598,#49599,#49600,#49601,#49602,#49603,#49604),(#49605,#49606,
#49607,#49608,#49609,#49610,#49611,#49612,#49613,#49614,#49615,#49616,#49617,
#49618,#49619,#49620,#49621,#49622,#49623,#49624,#49625,#49626,#49627,#49628,
#49629,#49630,#49631,#49632,#49633,#49634,#49635,#49636,#49637,#49638,#49639,
#49640,#49641,#49642,#49643,#49644,#49645,#49646,#49647,#49648,#49649,#49650,
#49651,#49652,#49653,#49654,#49655,#49656,#49657,#49658,#49659,#49660,#49661,
#49662,#49663,#49664,#49665,#49666,#49667,#49668,#49669,#49670,#49671,#49672,
#49673,#49674,#49675,#49676,#49677,#49678,#49679,#49680,#49681,#49682,#49683,
#49684,#49685,#49686,#49687,#49688,#49689,#49690,#49691,#49692,#49693,#49694,
#49695,#49696,#49697,#49698,#49699,#49700,#49701,#49702,#49703,#49704,#49705,
#49706,#49707,#49708,#49709,#49710,#49711,#49712,#49713,#49714,#49715,#49716,
#49717,#49718,#49719,#49720,#49721,#49722,#49723,#49724,#49725,#49726,#49727,
#49728,#49729,#49730,#49731,#49732,#49733,#49734,#49735,#49736,#49737,#49738,
#49739,#49740,#49741,#49742,#49743,#49744,#49745,#49746,#49747,#49748),
(#49749,#49750,#49751,#49752,#49753,#49754,#49755,#49756,#49757,#49758,
#49759,#49760,#49761,#49762,#49763,#49764,#49765,#49766,#49767,#49768,#49769,
#49770,#49771,#49772,#49773,#49774,#49775,#49776,#49777,#49778,#49779,#49780,
#49781,#49782,#49783,#49784,#49785,#49786,#49787,#49788,#49789,#49790,#49791,
#49792,#49793,#49794,#49795,#49796,#49797,#49798,#49799,#49800,#49801,#49802,
#49803,#49804,#49805,#49806,#49807,#49808,#49809,#49810,#49811,#49812,#49813,
#49814,#49815,#49816,#49817,#49818,#49819,#49820,#49821,#49822,#49823,#49824,
#49825,#49826,#49827,#49828,#49829,#49830,#49831,#49832,#49833,#49834,#49835,
#49836,#49837,#49838,#49839,#49840,#49841,#49842,#49843,#49844,#49845,#49846,
#49847,#49848,#49849,#49850,#49851,#49852,#49853,#49854,#49855,#49856,#49857,
#49858,#49859,#49860,#49861,#49862,#49863,#49864,#49865,#49866,#49867,#49868,
#49869,#49870,#49871,#49872,#49873,#49874,#49875,#49876,#49877,#49878,#49879,
#49880,#49881,#49882,#49883,#49884,#49885,#49886,#49887,#49888,#49889,#49890,
#49891,#49892),(#49893,#49894,#49895,#49896,#49897,#49898,#49899,#49900,
#49901,#49902,#49903,#49904,#49905,#49906,#49907,#49908,#49909,#49910,#49911,
#49912,#49913,#49914,#49915,#49916,#49917,#49918,#49919,#49920,#49921,#49922,
#49923,#49924,#49925,#49926,#49927,#49928,#49929,#49930,#49931,#49932,#49933,
#49934,#49935,#49936,#49937,#49938,#49939,#49940,#49941,#49942,#49943,#49944,
#49945,#49946,#49947,#49948,#49949,#49950,#49951,#49952,#49953,#49954,#49955,
#49956,#49957,#49958,#49959,#49960,#49961,#49962,#49963,#49964,#49965,#49966,
#49967,#49968,#49969,#49970,#49971,#49972,#49973,#49974,#49975,#49976,#49977,
#49978,#49979,#49980,#49981,#49982,#49983,#49984,#49985,#49986,#49987,#49988,
#49989,#49990,#49991,#49992,#49993,#49994,#49995,#49996,#49997,#49998,#49999,
#50000,#50001,#50002,#50003,#50004,#50005,#50006,#50007,#50008,#50009,#50010,
#50011,#50012,#50013,#50014,#50015,#50016,#50017,#50018,#50019,#50020,#50021,
#50022,#50023,#50024,#50025,#50026,#50027,#50028,#50029,#50030,#50031,#50032,
#50033,#50034,#50035,#50036),(#50037,#50038,#50039,#50040,#50041,#50042,
#50043,#50044,#50045,#50046,#50047,#50048,#50049,#50050,#50051,#50052,#50053,
#50054,#50055,#50056,#50057,#50058,#50059,#50060,#50061,#50062,#50063,#50064,
#50065,#50066,#50067,#50068,#50069,#50070,#50071,#50072,#50073,#50074,#50075,
#50076,#50077,#50078,#50079,#50080,#50081,#50082,#50083,#50084,#50085,#50086,
#50087,#50088,#50089,#50090,#50091,#50092,#50093,#50094,#50095,#50096,#50097,
#50098,#50099,#50100,#50101,#50102,#50103,#50104,#50105,#50106,#50107,#50108,
#50109,#50110,#50111,#50112,#50113,#50114,#50115,#50116,#50117,#50118,#50119,
#50120,#50121,#50122,#50123,#50124,#50125,#50126,#50127,#50128,#50129,#50130,
#50131,#50132,#50133,#50134,#50135,#50136,#50137,#50138,#50139,#50140,#50141,
#50142,#50143,#50144,#50145,#50146,#50147,#50148,#50149,#50150,#50151,#50152,
#50153,#50154,#50155,#50156,#50157,#50158,#50159,#50160,#50161,#50162,#50163,
#50164,#50165,#50166,#50167,#50168,#50169,#50170,#50171,#50172,#50173,#50174,
#50175,#50176,#50177,#50178,#50179,#50180),(#50181,#50182,#50183,#50184,
#50185,#50186,#50187,#50188,#50189,#50190,#50191,#50192,#50193,#50194,#50195,
#50196,#50197,#50198,#50199,#50200,#50201,#50202,#50203,#50204,#50205,#50206,
#50207,#50208,#50209,#50210,#50211,#50212,#50213,#50214,#50215,#50216,#50217,
#50218,#50219,#50220,#50221,#50222,#50223,#50224,#50225,#50226,#50227,#50228,
#50229,#50230,#50231,#50232,#50233,#50234,#50235,#50236,#50237,#50238,#50239,
#50240,#50241,#50242,#50243,#50244,#50245,#50246,#50247,#50248,#50249,#50250,
#50251,#50252,#50253,#50254,#50255,#50256,#50257,#50258,#50259,#50260,#50261,
#50262,#50263,#50264,#50265,#50266,#50267,#50268,#50269,#50270,#50271,#50272,
#50273,#50274,#50275,#50276,#50277,#50278,#50279,#50280,#50281,#50282,#50283,
#50284,#50285,#50286,#50287,#50288,#50289,#50290,#50291,#50292,#50293,#50294,
#50295,#50296,#50297,#50298,#50299,#50300,#50301,#50302,#50303,#50304,#50305,
#50306,#50307,#50308,#50309,#50310,#50311,#50312,#50313,#50314,#50315,#50316,
#50317,#50318,#50319,#50320,#50321,#50322,#50323,#50324),(#50325,#50326,
#50327,#50328,#50329,#50330,#50331,#50332,#50333,#50334,#50335,#50336,#50337,
#50338,#50339,#50340,#50341,#50342,#50343,#50344,#50345,#50346,#50347,#50348,
#50349,#50350,#50351,#50352,#50353,#50354,#50355,#50356,#50357,#50358,#50359,
#50360,#50361,#50362,#50363,#50364,#50365,#50366,#50367,#50368,#50369,#50370,
#50371,#50372,#50373,#50374,#50375,#50376,#50377,#50378,#50379,#50380,#50381,
#50382,#50383,#50384,#50385,#50386,#50387,#50388,#50389,#50390,#50391,#50392,
#50393,#50394,#50395,#50396,#50397,#50398,#50399,#50400,#50401,#50402,#50403,
#50404,#50405,#50406,#50407,#50408,#50409,#50410,#50411,#50412,#50413,#50414,
#50415,#50416,#50417,#50418,#50419,#50420,#50421,#50422,#50423,#50424,#50425,
#50426,#50427,#50428,#50429,#50430,#50431,#50432,#50433,#50434,#50435,#50436,
#50437,#50438,#50439,#50440,#50441,#50442,#50443,#50444,#50445,#50446,#50447,
#50448,#50449,#50450,#50451,#50452,#50453,#50454,#50455,#50456,#50457,#50458,
#50459,#50460,#50461,#50462,#50463,#50464,#50465,#50466,#50467,#50468),
(#50469,#50470,#50471,#50472,#50473,#50474,#50475,#50476,#50477,#50478,
#50479,#50480,#50481,#50482,#50483,#50484,#50485,#50486,#50487,#50488,#50489,
#50490,#50491,#50492,#50493,#50494,#50495,#50496,#50497,#50498,#50499,#50500,
#50501,#50502,#50503,#50504,#50505,#50506,#50507,#50508,#50509,#50510,#50511,
#50512,#50513,#50514,#50515,#50516,#50517,#50518,#50519,#50520,#50521,#50522,
#50523,#50524,#50525,#50526,#50527,#50528,#50529,#50530,#50531,#50532,#50533,
#50534,#50535,#50536,#50537,#50538,#50539,#50540,#50541,#50542,#50543,#50544,
#50545,#50546,#50547,#50548,#50549,#50550,#50551,#50552,#50553,#50554,#50555,
#50556,#50557,#50558,#50559,#50560,#50561,#50562,#50563,#50564,#50565,#50566,
#50567,#50568,#50569,#50570,#50571,#50572,#50573,#50574,#50575,#50576,#50577,
#50578,#50579,#50580,#50581,#50582,#50583,#50584,#50585,#50586,#50587,#50588,
#50589,#50590,#50591,#50592,#50593,#50594,#50595,#50596,#50597,#50598,#50599,
#50600,#50601,#50602,#50603,#50604,#50605,#50606,#50607,#50608,#50609,#50610,
#50611,#50612),(#50613,#50614,#50615,#50616,#50617,#50618,#50619,#50620,
#50621,#50622,#50623,#50624,#50625,#50626,#50627,#50628,#50629,#50630,#50631,
#50632,#50633,#50634,#50635,#50636,#50637,#50638,#50639,#50640,#50641,#50642,
#50643,#50644,#50645,#50646,#50647,#50648,#50649,#50650,#50651,#50652,#50653,
#50654,#50655,#50656,#50657,#50658,#50659,#50660,#50661,#50662,#50663,#50664,
#50665,#50666,#50667,#50668,#50669,#50670,#50671,#50672,#50673,#50674,#50675,
#50676,#50677,#50678,#50679,#50680,#50681,#50682,#50683,#50684,#50685,#50686,
#50687,#50688,#50689,#50690,#50691,#50692,#50693,#50694,#50695,#50696,#50697,
#50698,#50699,#50700,#50701,#50702,#50703,#50704,#50705,#50706,#50707,#50708,
#50709,#50710,#50711,#50712,#50713,#50714,#50715,#50716,#50717,#50718,#50719,
#50720,#50721,#50722,#50723,#50724,#50725,#50726,#50727,#50728,#50729,#50730,
#50731,#50732,#50733,#50734,#50735,#50736,#50737,#50738,#50739,#50740,#50741,
#50742,#50743,#50744,#50745,#50746,#50747,#50748,#50749,#50750,#50751,#50752,
#50753,#50754,#50755,#50756),(#50757,#50758,#50759,#50760,#50761,#50762,
#50763,#50764,#50765,#50766,#50767,#50768,#50769,#50770,#50771,#50772,#50773,
#50774,#50775,#50776,#50777,#50778,#50779,#50780,#50781,#50782,#50783,#50784,
#50785,#50786,#50787,#50788,#50789,#50790,#50791,#50792,#50793,#50794,#50795,
#50796,#50797,#50798,#50799,#50800,#50801,#50802,#50803,#50804,#50805,#50806,
#50807,#50808,#50809,#50810,#50811,#50812,#50813,#50814,#50815,#50816,#50817,
#50818,#50819,#50820,#50821,#50822,#50823,#50824,#50825,#50826,#50827,#50828,
#50829,#50830,#50831,#50832,#50833,#50834,#50835,#50836,#50837,#50838,#50839,
#50840,#50841,#50842,#50843,#50844,#50845,#50846,#50847,#50848,#50849,#50850,
#50851,#50852,#50853,#50854,#50855,#50856,#50857,#50858,#50859,#50860,#50861,
#50862,#50863,#50864,#50865,#50866,#50867,#50868,#50869,#50870,#50871,#50872,
#50873,#50874,#50875,#50876,#50877,#50878,#50879,#50880,#50881,#50882,#50883,
#50884,#50885,#50886,#50887,#50888,#50889,#50890,#50891,#50892,#50893,#50894,
#50895,#50896,#50897,#50898,#50899,#50900),(#50901,#50902,#50903,#50904,
#50905,#50906,#50907,#50908,#50909,#50910,#50911,#50912,#50913,#50914,#50915,
#50916,#50917,#50918,#50919,#50920,#50921,#50922,#50923,#50924,#50925,#50926,
#50927,#50928,#50929,#50930,#50931,#50932,#50933,#50934,#50935,#50936,#50937,
#50938,#50939,#50940,#50941,#50942,#50943,#50944,#50945,#50946,#50947,#50948,
#50949,#50950,#50951,#50952,#50953,#50954,#50955,#50956,#50957,#50958,#50959,
#50960,#50961,#50962,#50963,#50964,#50965,#50966,#50967,#50968,#50969,#50970,
#50971,#50972,#50973,#50974,#50975,#50976,#50977,#50978,#50979,#50980,#50981,
#50982,#50983,#50984,#50985,#50986,#50987,#50988,#50989,#50990,#50991,#50992,
#50993,#50994,#50995,#50996,#50997,#50998,#50999,#51000,#51001,#51002,#51003,
#51004,#51005,#51006,#51007,#51008,#51009,#51010,#51011,#51012,#51013,#51014,
#51015,#51016,#51017,#51018,#51019,#51020,#51021,#51022,#51023,#51024,#51025,
#51026,#51027,#51028,#51029,#51030,#51031,#51032,#51033,#51034,#51035,#51036,
#51037,#51038,#51039,#51040,#51041,#51042,#51043,#51044),(#51045,#51046,
#51047,#51048,#51049,#51050,#51051,#51052,#51053,#51054,#51055,#51056,#51057,
#51058,#51059,#51060,#51061,#51062,#51063,#51064,#51065,#51066,#51067,#51068,
#51069,#51070,#51071,#51072,#51073,#51074,#51075,#51076,#51077,#51078,#51079,
#51080,#51081,#51082,#51083,#51084,#51085,#51086,#51087,#51088,#51089,#51090,
#51091,#51092,#51093,#51094,#51095,#51096,#51097,#51098,#51099,#51100,#51101,
#51102,#51103,#51104,#51105,#51106,#51107,#51108,#51109,#51110,#51111,#51112,
#51113,#51114,#51115,#51116,#51117,#51118,#51119,#51120,#51121,#51122,#51123,
#51124,#51125,#51126,#51127,#51128,#51129,#51130,#51131,#51132,#51133,#51134,
#51135,#51136,#51137,#51138,#51139,#51140,#51141,#51142,#51143,#51144,#51145,
#51146,#51147,#51148,#51149,#51150,#51151,#51152,#51153,#51154,#51155,#51156,
#51157,#51158,#51159,#51160,#51161,#51162,#51163,#51164,#51165,#51166,#51167,
#51168,#51169,#51170,#51171,#51172,#51173,#51174,#51175,#51176,#51177,#51178,
#51179,#51180,#51181,#51182,#51183,#51184,#51185,#51186,#51187,#51188),
(#51189,#51190,#51191,#51192,#51193,#51194,#51195,#51196,#51197,#51198,
#51199,#51200,#51201,#51202,#51203,#51204,#51205,#51206,#51207,#51208,#51209,
#51210,#51211,#51212,#51213,#51214,#51215,#51216,#51217,#51218,#51219,#51220,
#51221,#51222,#51223,#51224,#51225,#51226,#51227,#51228,#51229,#51230,#51231,
#51232,#51233,#51234,#51235,#51236,#51237,#51238,#51239,#51240,#51241,#51242,
#51243,#51244,#51245,#51246,#51247,#51248,#51249,#51250,#51251,#51252,#51253,
#51254,#51255,#51256,#51257,#51258,#51259,#51260,#51261,#51262,#51263,#51264,
#51265,#51266,#51267,#51268,#51269,#51270,#51271,#51272,#51273,#51274,#51275,
#51276,#51277,#51278,#51279,#51280,#51281,#51282,#51283,#51284,#51285,#51286,
#51287,#51288,#51289,#51290,#51291,#51292,#51293,#51294,#51295,#51296,#51297,
#51298,#51299,#51300,#51301,#51302,#51303,#51304,#51305,#51306,#51307,#51308,
#51309,#51310,#51311,#51312,#51313,#51314,#51315,#51316,#51317,#51318,#51319,
#51320,#51321,#51322,#51323,#51324,#51325,#51326,#51327,#51328,#51329,#51330,
#51331,#51332),(#51333,#51334,#51335,#51336,#51337,#51338,#51339,#51340,
#51341,#51342,#51343,#51344,#51345,#51346,#51347,#51348,#51349,#51350,#51351,
#51352,#51353,#51354,#51355,#51356,#51357,#51358,#51359,#51360,#51361,#51362,
#51363,#51364,#51365,#51366,#51367,#51368,#51369,#51370,#51371,#51372,#51373,
#51374,#51375,#51376,#51377,#51378,#51379,#51380,#51381,#51382,#51383,#51384,
#51385,#51386,#51387,#51388,#51389,#51390,#51391,#51392,#51393,#51394,#51395,
#51396,#51397,#51398,#51399,#51400,#51401,#51402,#51403,#51404,#51405,#51406,
#51407,#51408,#51409,#51410,#51411,#51412,#51413,#51414,#51415,#51416,#51417,
#51418,#51419,#51420,#51421,#51422,#51423,#51424,#51425,#51426,#51427,#51428,
#51429,#51430,#51431,#51432,#51433,#51434,#51435,#51436,#51437,#51438,#51439,
#51440,#51441,#51442,#51443,#51444,#51445,#51446,#51447,#51448,#51449,#51450,
#51451,#51452,#51453,#51454,#51455,#51456,#51457,#51458,#51459,#51460,#51461,
#51462,#51463,#51464,#51465,#51466,#51467,#51468,#51469,#51470,#51471,#51472,
#51473,#51474,#51475,#51476),(#51477,#51478,#51479,#51480,#51481,#51482,
#51483,#51484,#51485,#51486,#51487,#51488,#51489,#51490,#51491,#51492,#51493,
#51494,#51495,#51496,#51497,#51498,#51499,#51500,#51501,#51502,#51503,#51504,
#51505,#51506,#51507,#51508,#51509,#51510,#51511,#51512,#51513,#51514,#51515,
#51516,#51517,#51518,#51519,#51520,#51521,#51522,#51523,#51524,#51525,#51526,
#51527,#51528,#51529,#51530,#51531,#51532,#51533,#51534,#51535,#51536,#51537,
#51538,#51539,#51540,#51541,#51542,#51543,#51544,#51545,#51546,#51547,#51548,
#51549,#51550,#51551,#51552,#51553,#51554,#51555,#51556,#51557,#51558,#51559,
#51560,#51561,#51562,#51563,#51564,#51565,#51566,#51567,#51568,#51569,#51570,
#51571,#51572,#51573,#51574,#51575,#51576,#51577,#51578,#51579,#51580,#51581,
#51582,#51583,#51584,#51585,#51586,#51587,#51588,#51589,#51590,#51591,#51592,
#51593,#51594,#51595,#51596,#51597,#51598,#51599,#51600,#51601,#51602,#51603,
#51604,#51605,#51606,#51607,#51608,#51609,#51610,#51611,#51612,#51613,#51614,
#51615,#51616,#51617,#51618,#51619,#51620),(#51621,#51622,#51623,#51624,
#51625,#51626,#51627,#51628,#51629,#51630,#51631,#51632,#51633,#51634,#51635,
#51636,#51637,#51638,#51639,#51640,#51641,#51642,#51643,#51644,#51645,#51646,
#51647,#51648,#51649,#51650,#51651,#51652,#51653,#51654,#51655,#51656,#51657,
#51658,#51659,#51660,#51661,#51662,#51663,#51664,#51665,#51666,#51667,#51668,
#51669,#51670,#51671,#51672,#51673,#51674,#51675,#51676,#51677,#51678,#51679,
#51680,#51681,#51682,#51683,#51684,#51685,#51686,#51687,#51688,#51689,#51690,
#51691,#51692,#51693,#51694,#51695,#51696,#51697,#51698,#51699,#51700,#51701,
#51702,#51703,#51704,#51705,#51706,#51707,#51708,#51709,#51710,#51711,#51712,
#51713,#51714,#51715,#51716,#51717,#51718,#51719,#51720,#51721,#51722,#51723,
#51724,#51725,#51726,#51727,#51728,#51729,#51730,#51731,#51732,#51733,#51734,
#51735,#51736,#51737,#51738,#51739,#51740,#51741,#51742,#51743,#51744,#51745,
#51746,#51747,#51748,#51749,#51750,#51751,#51752,#51753,#51754,#51755,#51756,
#51757,#51758,#51759,#51760,#51761,#51762,#51763,#51764),(#51765,#51766,
#51767,#51768,#51769,#51770,#51771,#51772,#51773,#51774,#51775,#51776,#51777,
#51778,#51779,#51780,#51781,#51782,#51783,#51784,#51785,#51786,#51787,#51788,
#51789,#51790,#51791,#51792,#51793,#51794,#51795,#51796,#51797,#51798,#51799,
#51800,#51801,#51802,#51803,#51804,#51805,#51806,#51807,#51808,#51809,#51810,
#51811,#51812,#51813,#51814,#51815,#51816,#51817,#51818,#51819,#51820,#51821,
#51822,#51823,#51824,#51825,#51826,#51827,#51828,#51829,#51830,#51831,#51832,
#51833,#51834,#51835,#51836,#51837,#51838,#51839,#51840,#51841,#51842,#51843,
#51844,#51845,#51846,#51847,#51848,#51849,#51850,#51851,#51852,#51853,#51854,
#51855,#51856,#51857,#51858,#51859,#51860,#51861,#51862,#51863,#51864,#51865,
#51866,#51867,#51868,#51869,#51870,#51871,#51872,#51873,#51874,#51875,#51876,
#51877,#51878,#51879,#51880,#51881,#51882,#51883,#51884,#51885,#51886,#51887,
#51888,#51889,#51890,#51891,#51892,#51893,#51894,#51895,#51896,#51897,#51898,
#51899,#51900,#51901,#51902,#51903,#51904,#51905,#51906,#51907,#51908),
(#51909,#51910,#51911,#51912,#51913,#51914,#51915,#51916,#51917,#51918,
#51919,#51920,#51921,#51922,#51923,#51924,#51925,#51926,#51927,#51928,#51929,
#51930,#51931,#51932,#51933,#51934,#51935,#51936,#51937,#51938,#51939,#51940,
#51941,#51942,#51943,#51944,#51945,#51946,#51947,#51948,#51949,#51950,#51951,
#51952,#51953,#51954,#51955,#51956,#51957,#51958,#51959,#51960,#51961,#51962,
#51963,#51964,#51965,#51966,#51967,#51968,#51969,#51970,#51971,#51972,#51973,
#51974,#51975,#51976,#51977,#51978,#51979,#51980,#51981,#51982,#51983,#51984,
#51985,#51986,#51987,#51988,#51989,#51990,#51991,#51992,#51993,#51994,#51995,
#51996,#51997,#51998,#51999,#52000,#52001,#52002,#52003,#52004,#52005,#52006,
#52007,#52008,#52009,#52010,#52011,#52012,#52013,#52014,#52015,#52016,#52017,
#52018,#52019,#52020,#52021,#52022,#52023,#52024,#52025,#52026,#52027,#52028,
#52029,#52030,#52031,#52032,#52033,#52034,#52035,#52036,#52037,#52038,#52039,
#52040,#52041,#52042,#52043,#52044,#52045,#52046,#52047,#52048,#52049,#52050,
#52051,#52052),(#52053,#52054,#52055,#52056,#52057,#52058,#52059,#52060,
#52061,#52062,#52063,#52064,#52065,#52066,#52067,#52068,#52069,#52070,#52071,
#52072,#52073,#52074,#52075,#52076,#52077,#52078,#52079,#52080,#52081,#52082,
#52083,#52084,#52085,#52086,#52087,#52088,#52089,#52090,#52091,#52092,#52093,
#52094,#52095,#52096,#52097,#52098,#52099,#52100,#52101,#52102,#52103,#52104,
#52105,#52106,#52107,#52108,#52109,#52110,#52111,#52112,#52113,#52114,#52115,
#52116,#52117,#52118,#52119,#52120,#52121,#52122,#52123,#52124,#52125,#52126,
#52127,#52128,#52129,#52130,#52131,#52132,#52133,#52134,#52135,#52136,#52137,
#52138,#52139,#52140,#52141,#52142,#52143,#52144,#52145,#52146,#52147,#52148,
#52149,#52150,#52151,#52152,#52153,#52154,#52155,#52156,#52157,#52158,#52159,
#52160,#52161,#52162,#52163,#52164,#52165,#52166,#52167,#52168,#52169,#52170,
#52171,#52172,#52173,#52174,#52175,#52176,#52177,#52178,#52179,#52180,#52181,
#52182,#52183,#52184,#52185,#52186,#52187,#52188,#52189,#52190,#52191,#52192,
#52193,#52194,#52195,#52196),(#52197,#52198,#52199,#52200,#52201,#52202,
#52203,#52204,#52205,#52206,#52207,#52208,#52209,#52210,#52211,#52212,#52213,
#52214,#52215,#52216,#52217,#52218,#52219,#52220,#52221,#52222,#52223,#52224,
#52225,#52226,#52227,#52228,#52229,#52230,#52231,#52232,#52233,#52234,#52235,
#52236,#52237,#52238,#52239,#52240,#52241,#52242,#52243,#52244,#52245,#52246,
#52247,#52248,#52249,#52250,#52251,#52252,#52253,#52254,#52255,#52256,#52257,
#52258,#52259,#52260,#52261,#52262,#52263,#52264,#52265,#52266,#52267,#52268,
#52269,#52270,#52271,#52272,#52273,#52274,#52275,#52276,#52277,#52278,#52279,
#52280,#52281,#52282,#52283,#52284,#52285,#52286,#52287,#52288,#52289,#52290,
#52291,#52292,#52293,#52294,#52295,#52296,#52297,#52298,#52299,#52300,#52301,
#52302,#52303,#52304,#52305,#52306,#52307,#52308,#52309,#52310,#52311,#52312,
#52313,#52314,#52315,#52316,#52317,#52318,#52319,#52320,#52321,#52322,#52323,
#52324,#52325,#52326,#52327,#52328,#52329,#52330,#52331,#52332,#52333,#52334,
#52335,#52336,#52337,#52338,#52339,#52340)),.UNSPECIFIED.,.F.,.F.,.F.,(4,
1,1,1,1,1,1,1,1,1,1,1,1,1,1,1,1,1,1,1,1,1,1,1,1,1,1,1,1,1,1,1,1,1,1,1,1,
1,1,1,1,1,1,1,1,1,1,1,1,1,1,1,1,1,1,1,1,1,1,1,1,1,1,1,1,1,1,1,1,1,1,1,4),
(4,2,1,1,2,1,1,1,2,1,1,1,1,2,1,1,1,1,2,1,1,1,1,1,1,1,2,1,1,1,1,1,1,1,2,
1,1,1,1,1,1,1,1,2,1,1,1,1,1,1,1,1,1,1,1,1,2,1,1,1,1,1,2,1,1,1,1,1,1,1,2,
1,1,1,1,2,1,1,1,1,1,1,1,1,1,1,2,1,1,1,1,1,2,1,1,1,1,2,1,1,1,1,1,1,1,1,1,
1,1,1,1,2,1,1,1,1,2,1,1,1,1,1,2,4),(0.0268156772007072,0.0437158964674566,
0.0606153077094141,0.0775147189513715,0.094414130193329,0.111313541435286,
0.115538394245776,0.119763247056265,0.128212952677244,0.145112363919201,
0.162011775161159,0.178911186403116,0.195810597645074,0.212710008887031,
0.229609420128989,0.238059125749968,0.246508831370946,0.263408242612904,
0.271857948233882,0.280307653854861,0.284532506665351,0.28875735947584,
0.297207065096819,0.308473339258124,0.319739613419429,0.331005887580734,
0.336639024661386,0.342272161742039,0.353538435903344,0.364804710064649,
0.387337258387259,0.398603532548564,0.409869806709869,0.421136080871174,
0.432402355032479,0.454934903355088,0.466201177516393,0.477467451677698,
0.500000000000308,0.511266274161613,0.522532548322918,0.545065096645528,
0.567597644968138,0.584497056210096,0.601396467452053,0.618295878694011,
0.635195289935968,0.643644995556947,0.652094701177926,0.668994112419883,
0.677443818040862,0.685893523661841,0.702792934903798,0.719692346145756,
0.728142051766734,0.736591757387713,0.75349116862967,0.770390579871628,
0.787289991113585,0.804189402355543,0.8210888135975,0.837988224839458,0.854887636081415,
0.871787047323373,0.880236752944352,0.884461605754841,0.88868645856533,
0.897136164186309,0.905585869807288,0.922485281049245,0.939384692291203,
0.95628410353316,0.973183514775118),(0.0960305811261704,0.0972154775043869,
0.109378606187391,0.121541734870394,0.145867992236401,0.151993923775347,
0.158119855314292,0.170371718392183,0.194875444547964,0.200989580746302,
0.207103716944641,0.219331989341318,0.231560261737996,0.243788534134673,
0.246827927163601,0.24986732019253,0.255946106250386,0.2681036783661,0.292418822597527,
0.293959106599555,0.295499390601583,0.29857995860564,0.304741094613752,
0.310902230621865,0.317063366629978,0.329385638646203,0.341707910662428,
0.344790082003921,0.347872253345414,0.354036596028399,0.36636528139437,
0.37869396676034,0.384858309443326,0.387940480784818,0.391022652126311,
0.392583125212554,0.394143598298796,0.397264544471281,0.403506436816251,
0.415990221506191,0.428474006196132,0.431594952368617,0.434715898541102,
0.440957790886072,0.442498863959882,0.444039937033693,0.447122083181315,
0.448663156255125,0.450204229328936,0.450974765865841,0.451745302402747,
0.452515838939652,0.452901107208105,0.453286375476557,0.465614960067043,
0.477943544657529,0.490272129248014,0.493311253959715,0.496350378671415,
0.502428628094816,0.514585126941617,0.526741625788419,0.53889812463522,
0.540417366609575,0.541936608583929,0.544975092532638,0.551052060430056,
0.563205996224891,0.575359932019726,0.581436899917144,0.587513867814562,
0.590576684581802,0.593639501349043,0.599765134883524,0.612016401952486,
0.636518936090411,0.642599511724338,0.645639799541302,0.648680087358265,
0.654760662992193,0.66084123862612,0.666921814260047,0.669962102077011,
0.673002389893974,0.676042677710938,0.679082965527902,0.685163541161829,
0.688226234079092,0.691288926996354,0.697414312830879,0.70966508449993,
0.72191585616898,0.734166627838031,0.737264704064826,0.740362780291622,
0.746558932745213,0.758951237652395,0.783735847466759,0.785338745832564,
0.78694164419837,0.790147440929981,0.796559034393203,0.809382221319647,
0.815793814782869,0.822205408246091,0.823808306611897,0.825411204977702,
0.828617001709314,0.830219900075119,0.831021349258022,0.831822798440925,
0.835028595172536,0.838457852551916,0.841887109931297,0.848745624690058,
0.86246265420758,0.889896713242625,0.893337440953794,0.896778168664963,
0.9036596240873,0.910541079509638,0.917422534931976,0.944948356621327,0.967478850977141),
 .UNSPECIFIED.);
#18853=B_SPLINE_SURFACE_WITH_KNOTS('',3,3,((#55216,#55217,#55218,#55219,
#55220,#55221,#55222,#55223,#55224,#55225,#55226,#55227,#55228,#55229,#55230,
#55231,#55232,#55233,#55234,#55235,#55236,#55237,#55238,#55239,#55240,#55241,
#55242,#55243,#55244,#55245,#55246,#55247,#55248,#55249,#55250,#55251,#55252,
#55253,#55254,#55255,#55256,#55257,#55258,#55259,#55260,#55261),(#55262,
#55263,#55264,#55265,#55266,#55267,#55268,#55269,#55270,#55271,#55272,#55273,
#55274,#55275,#55276,#55277,#55278,#55279,#55280,#55281,#55282,#55283,#55284,
#55285,#55286,#55287,#55288,#55289,#55290,#55291,#55292,#55293,#55294,#55295,
#55296,#55297,#55298,#55299,#55300,#55301,#55302,#55303,#55304,#55305,#55306,
#55307),(#55308,#55309,#55310,#55311,#55312,#55313,#55314,#55315,#55316,
#55317,#55318,#55319,#55320,#55321,#55322,#55323,#55324,#55325,#55326,#55327,
#55328,#55329,#55330,#55331,#55332,#55333,#55334,#55335,#55336,#55337,#55338,
#55339,#55340,#55341,#55342,#55343,#55344,#55345,#55346,#55347,#55348,#55349,
#55350,#55351,#55352,#55353),(#55354,#55355,#55356,#55357,#55358,#55359,
#55360,#55361,#55362,#55363,#55364,#55365,#55366,#55367,#55368,#55369,#55370,
#55371,#55372,#55373,#55374,#55375,#55376,#55377,#55378,#55379,#55380,#55381,
#55382,#55383,#55384,#55385,#55386,#55387,#55388,#55389,#55390,#55391,#55392,
#55393,#55394,#55395,#55396,#55397,#55398,#55399),(#55400,#55401,#55402,
#55403,#55404,#55405,#55406,#55407,#55408,#55409,#55410,#55411,#55412,#55413,
#55414,#55415,#55416,#55417,#55418,#55419,#55420,#55421,#55422,#55423,#55424,
#55425,#55426,#55427,#55428,#55429,#55430,#55431,#55432,#55433,#55434,#55435,
#55436,#55437,#55438,#55439,#55440,#55441,#55442,#55443,#55444,#55445),
(#55446,#55447,#55448,#55449,#55450,#55451,#55452,#55453,#55454,#55455,
#55456,#55457,#55458,#55459,#55460,#55461,#55462,#55463,#55464,#55465,#55466,
#55467,#55468,#55469,#55470,#55471,#55472,#55473,#55474,#55475,#55476,#55477,
#55478,#55479,#55480,#55481,#55482,#55483,#55484,#55485,#55486,#55487,#55488,
#55489,#55490,#55491)),.UNSPECIFIED.,.F.,.T.,.F.,(4,1,1,4),(4,2,1,2,1,1,
1,1,1,1,2,1,1,1,1,2,1,1,2,1,1,1,1,2,1,2,1,1,1,2,1,2,2,4),(-0.00142384579029664,
0.285714285714286,0.571428571428571,1.),(-9.19419977830157,-8.92020082022876,
-8.53897544224619,-8.15775006426363,-7.94884017932526,-7.73993029438688,
-7.32211052451013,-7.11320063957175,-6.79983581216419,-6.695380869695,-6.48647098475663,
-6.38692241757501,-6.28737385039339,-6.08827671603015,-5.73985673089448,
-5.69008244730366,-5.46391696776057,-5.23775148821748,-5.08697450185542,
-5.0692256166783,-5.01597896114694,-4.94498342043847,-4.80299233902153,
-4.51901017618764,-4.27069680674408,-3.85684119100481,-3.05948850905774,
-2.69705547180907,-1.68224296751281,-1.53726975261334,-1.28960453962952,
-0.876829184656479,-0.308773384377632,0.),.UNSPECIFIED.);
#18854=B_SPLINE_SURFACE_WITH_KNOTS('',3,3,((#55772,#55773,#55774,#55775,
#55776,#55777,#55778,#55779,#55780,#55781,#55782,#55783,#55784,#55785,#55786,
#55787,#55788,#55789,#55790,#55791,#55792,#55793,#55794,#55795,#55796,#55797,
#55798,#55799,#55800,#55801,#55802,#55803,#55804,#55805,#55806,#55807,#55808,
#55809),(#55810,#55811,#55812,#55813,#55814,#55815,#55816,#55817,#55818,
#55819,#55820,#55821,#55822,#55823,#55824,#55825,#55826,#55827,#55828,#55829,
#55830,#55831,#55832,#55833,#55834,#55835,#55836,#55837,#55838,#55839,#55840,
#55841,#55842,#55843,#55844,#55845,#55846,#55847),(#55848,#55849,#55850,
#55851,#55852,#55853,#55854,#55855,#55856,#55857,#55858,#55859,#55860,#55861,
#55862,#55863,#55864,#55865,#55866,#55867,#55868,#55869,#55870,#55871,#55872,
#55873,#55874,#55875,#55876,#55877,#55878,#55879,#55880,#55881,#55882,#55883,
#55884,#55885),(#55886,#55887,#55888,#55889,#55890,#55891,#55892,#55893,
#55894,#55895,#55896,#55897,#55898,#55899,#55900,#55901,#55902,#55903,#55904,
#55905,#55906,#55907,#55908,#55909,#55910,#55911,#55912,#55913,#55914,#55915,
#55916,#55917,#55918,#55919,#55920,#55921,#55922,#55923),(#55924,#55925,
#55926,#55927,#55928,#55929,#55930,#55931,#55932,#55933,#55934,#55935,#55936,
#55937,#55938,#55939,#55940,#55941,#55942,#55943,#55944,#55945,#55946,#55947,
#55948,#55949,#55950,#55951,#55952,#55953,#55954,#55955,#55956,#55957,#55958,
#55959,#55960,#55961)),.UNSPECIFIED.,.F.,.T.,.F.,(4,1,4),(4,2,2,2,1,2,2,
2,1,1,1,2,1,2,1,1,1,1,1,1,1,2,1,1,2,4),(0.,0.571428571428571,1.),(-9.1649736818217,
-8.85500373849296,-8.29205753853133,-7.63533633256183,-6.48172574214371,
-5.32811515172559,-4.66932841177279,-4.10834838496996,-4.03861769654365,
-3.96888700811733,-3.8294256312647,-3.55050287755944,-3.18769596354942,
-2.82488904953941,-2.76816872685197,-2.71144840416452,-2.59800775878964,
-2.37112646803988,-1.91736388654036,-1.46360130504084,-1.23672001429108,
-1.00983872354131,-0.824618171658037,-0.639397619774759,-0.268956516008204,
0.),.UNSPECIFIED.);
#18855=B_SPLINE_SURFACE_WITH_KNOTS('',3,3,((#55967,#55968,#55969,#55970,
#55971,#55972,#55973,#55974,#55975,#55976,#55977,#55978,#55979,#55980,#55981,
#55982,#55983),(#55984,#55985,#55986,#55987,#55988,#55989,#55990,#55991,
#55992,#55993,#55994,#55995,#55996,#55997,#55998,#55999,#56000),(#56001,
#56002,#56003,#56004,#56005,#56006,#56007,#56008,#56009,#56010,#56011,#56012,
#56013,#56014,#56015,#56016,#56017),(#56018,#56019,#56020,#56021,#56022,
#56023,#56024,#56025,#56026,#56027,#56028,#56029,#56030,#56031,#56032,#56033,
#56034),(#56035,#56036,#56037,#56038,#56039,#56040,#56041,#56042,#56043,
#56044,#56045,#56046,#56047,#56048,#56049,#56050,#56051)),.UNSPECIFIED.,
 .F.,.T.,.F.,(4,1,4),(4,1,1,2,1,1,1,1,1,1,1,2,4),(0.,0.571428571428571,
1.00001445338435),(-1.29174070129165,-1.21783674573549,-1.07002883462318,
-0.922220923510859,-0.795342097926536,-0.753049156065094,-0.668463272342212,
-0.583877388619329,-0.414705621173564,-0.330119737450682,-0.245533853727799,
-0.076362086282034,0.),.UNSPECIFIED.);
#18856=B_SPLINE_SURFACE_WITH_KNOTS('',3,3,((#56103,#56104,#56105,#56106,
#56107,#56108,#56109,#56110,#56111,#56112,#56113,#56114,#56115,#56116,#56117),
(#56118,#56119,#56120,#56121,#56122,#56123,#56124,#56125,#56126,#56127,
#56128,#56129,#56130,#56131,#56132),(#56133,#56134,#56135,#56136,#56137,
#56138,#56139,#56140,#56141,#56142,#56143,#56144,#56145,#56146,#56147),
(#56148,#56149,#56150,#56151,#56152,#56153,#56154,#56155,#56156,#56157,
#56158,#56159,#56160,#56161,#56162),(#56163,#56164,#56165,#56166,#56167,
#56168,#56169,#56170,#56171,#56172,#56173,#56174,#56175,#56176,#56177)),
 .UNSPECIFIED.,.F.,.T.,.F.,(4,1,4),(4,2,1,1,1,1,1,2,1,1,4),(0.,0.571428571428571,
1.),(-1.2915881661436,-1.18065640410841,-1.01148719643655,-0.842317988764689,
-0.757733384928759,-0.673148781092829,-0.50397957342097,-0.334810365749111,
-0.234367256024377,-0.133924146299644,0.),.UNSPECIFIED.);
#18857=B_SPLINE_SURFACE_WITH_KNOTS('',3,3,((#56183,#56184,#56185,#56186,
#56187,#56188,#56189,#56190,#56191,#56192,#56193,#56194,#56195,#56196,#56197,
#56198,#56199,#56200,#56201,#56202,#56203,#56204,#56205),(#56206,#56207,
#56208,#56209,#56210,#56211,#56212,#56213,#56214,#56215,#56216,#56217,#56218,
#56219,#56220,#56221,#56222,#56223,#56224,#56225,#56226,#56227,#56228),
(#56229,#56230,#56231,#56232,#56233,#56234,#56235,#56236,#56237,#56238,
#56239,#56240,#56241,#56242,#56243,#56244,#56245,#56246,#56247,#56248,#56249,
#56250,#56251),(#56252,#56253,#56254,#56255,#56256,#56257,#56258,#56259,
#56260,#56261,#56262,#56263,#56264,#56265,#56266,#56267,#56268,#56269,#56270,
#56271,#56272,#56273,#56274),(#56275,#56276,#56277,#56278,#56279,#56280,
#56281,#56282,#56283,#56284,#56285,#56286,#56287,#56288,#56289,#56290,#56291,
#56292,#56293,#56294,#56295,#56296,#56297)),.UNSPECIFIED.,.F.,.T.,.F.,(4,
1,4),(4,1,1,1,1,2,1,1,1,1,1,1,1,1,1,2,1,1,4),(0.,0.571428571428571,1.00007865727904),
(-1.29193145083568,-1.18863906797729,-1.0853466851189,-0.982054302260506,
-0.878761919402114,-0.775469536543723,-0.720593698815789,-0.665717861087855,
-0.555966185631988,-0.44621451017612,-0.336462834720253,-0.309024915856286,
-0.281586996992319,-0.254149078128352,-0.240430118696369,-0.226711159264386,
-0.181368927411508,-0.136026695558631,0.),.UNSPECIFIED.);
#18858=B_SPLINE_SURFACE_WITH_KNOTS('',3,3,((#56420,#56421,#56422,#56423,
#56424,#56425,#56426,#56427,#56428,#56429,#56430,#56431,#56432,#56433,#56434,
#56435,#56436,#56437,#56438),(#56439,#56440,#56441,#56442,#56443,#56444,
#56445,#56446,#56447,#56448,#56449,#56450,#56451,#56452,#56453,#56454,#56455,
#56456,#56457),(#56458,#56459,#56460,#56461,#56462,#56463,#56464,#56465,
#56466,#56467,#56468,#56469,#56470,#56471,#56472,#56473,#56474,#56475,#56476),
(#56477,#56478,#56479,#56480,#56481,#56482,#56483,#56484,#56485,#56486,
#56487,#56488,#56489,#56490,#56491,#56492,#56493,#56494,#56495),(#56496,
#56497,#56498,#56499,#56500,#56501,#56502,#56503,#56504,#56505,#56506,#56507,
#56508,#56509,#56510,#56511,#56512,#56513,#56514)),.UNSPECIFIED.,.F.,.T.,
 .F.,(4,1,4),(4,1,2,1,1,1,1,1,2,1,1,1,1,1,4),(0.,0.571428571428571,1.),
(-1.29158374785677,-1.19032888736264,-1.03844659662145,-0.983576456101594,
-0.928706315581737,-0.818966034542023,-0.709225753502309,-0.599485472462595,
-0.489745191422881,-0.440770672280593,-0.391796153138305,-0.293847114853729,
-0.195898076569152,-0.0979490382845762,0.),.UNSPECIFIED.);
#18859=B_SPLINE_SURFACE_WITH_KNOTS('',3,3,((#56520,#56521,#56522,#56523,
#56524,#56525,#56526,#56527),(#56528,#56529,#56530,#56531,#56532,#56533,
#56534,#56535),(#56536,#56537,#56538,#56539,#56540,#56541,#56542,#56543),
(#56544,#56545,#56546,#56547,#56548,#56549,#56550,#56551)),
 .UNSPECIFIED.,.F.,.F.,.F.,(4,4),(4,2,2,4),(0.,1.),(-0.32931292451793,-0.275040863381023,
0.328202711224253,0.329193263838381),.UNSPECIFIED.);
#18860=B_SPLINE_SURFACE_WITH_KNOTS('',3,3,((#56577,#56578,#56579,#56580,
#56581),(#56582,#56583,#56584,#56585,#56586),(#56587,#56588,#56589,#56590,
#56591),(#56592,#56593,#56594,#56595,#56596)),.UNSPECIFIED.,.F.,.F.,.F.,
(4,4),(4,1,4),(0.,1.),(-0.299498223131783,-0.0164065923085981,0.361048915455649),
 .UNSPECIFIED.);
#18861=B_SPLINE_SURFACE_WITH_KNOTS('',3,3,((#56607,#56608,#56609,#56610,
#56611,#56612,#56613,#56614,#56615,#56616,#56617,#56618,#56619,#56620,#56621,
#56622,#56623),(#56624,#56625,#56626,#56627,#56628,#56629,#56630,#56631,
#56632,#56633,#56634,#56635,#56636,#56637,#56638,#56639,#56640),(#56641,
#56642,#56643,#56644,#56645,#56646,#56647,#56648,#56649,#56650,#56651,#56652,
#56653,#56654,#56655,#56656,#56657),(#56658,#56659,#56660,#56661,#56662,
#56663,#56664,#56665,#56666,#56667,#56668,#56669,#56670,#56671,#56672,#56673,
#56674)),.UNSPECIFIED.,.F.,.F.,.F.,(4,4),(4,2,1,1,1,1,1,1,1,1,1,2,4),(0.,
1.),(-0.297794025374421,-0.296794638674619,-0.236399107412475,-0.17600357615033,
-0.115608044888186,-0.0552125136260416,0.00518301763610282,0.0655785488982472,
0.125974080160392,0.186369611422536,0.24676514268468,0.307160673946825,
0.361386326815235),.UNSPECIFIED.);
#18862=B_SPLINE_SURFACE_WITH_KNOTS('',3,3,((#56689,#56690,#56691,#56692,
#56693,#56694,#56695,#56696,#56697),(#56698,#56699,#56700,#56701,#56702,
#56703,#56704,#56705,#56706),(#56707,#56708,#56709,#56710,#56711,#56712,
#56713,#56714,#56715),(#56716,#56717,#56718,#56719,#56720,#56721,#56722,
#56723,#56724)),.UNSPECIFIED.,.F.,.F.,.F.,(4,4),(4,2,1,2,4),(-4.7316025546104E-6,
1.00000473160542),(-0.330176451776112,-0.314286281116363,-0.0628601143819659,
0.314279135719629,0.330169461918646),.UNSPECIFIED.);
#18863=B_SPLINE_SURFACE_WITH_KNOTS('',3,3,((#56727,#56728,#56729,#56730),
(#56731,#56732,#56733,#56734),(#56735,#56736,#56737,#56738),(#56739,#56740,
#56741,#56742),(#56743,#56744,#56745,#56746),(#56747,#56748,#56749,#56750)),
 .UNSPECIFIED.,.F.,.F.,.F.,(4,1,1,4),(4,4),(-0.799336073509661,-0.594771590871585,
-0.39020710823351,-0.0833603842763964),(-0.204000152442369,0.204),
 .UNSPECIFIED.);
#18864=B_SPLINE_SURFACE_WITH_KNOTS('',3,3,((#56753,#56754,#56755,#56756),
(#56757,#56758,#56759,#56760),(#56761,#56762,#56763,#56764),(#56765,#56766,
#56767,#56768),(#56769,#56770,#56771,#56772),(#56773,#56774,#56775,#56776)),
 .UNSPECIFIED.,.F.,.F.,.F.,(4,1,1,4),(4,4),(-1.96312962658784,-1.63061718285122,
-1.46436096098291,-0.799336073509661),(-0.204,0.204048008019707),
 .UNSPECIFIED.);
#18865=B_SPLINE_SURFACE_WITH_KNOTS('',3,3,((#56778,#56779,#56780,#56781),
(#56782,#56783,#56784,#56785),(#56786,#56787,#56788,#56789),(#56790,#56791,
#56792,#56793),(#56794,#56795,#56796,#56797),(#56798,#56799,#56800,#56801)),
 .UNSPECIFIED.,.F.,.F.,.F.,(4,1,1,4),(4,4),(-3.17329134625142,-3.0004111005852,
-2.65465060925274,-1.96312962658784),(-0.204,0.204),.UNSPECIFIED.);
#18866=B_SPLINE_SURFACE_WITH_KNOTS('',3,3,((#56805,#56806,#56807,#56808),
(#56809,#56810,#56811,#56812),(#56813,#56814,#56815,#56816),(#56817,#56818,
#56819,#56820),(#56821,#56822,#56823,#56824),(#56825,#56826,#56827,#56828)),
 .UNSPECIFIED.,.F.,.F.,.F.,(4,1,1,4),(4,4),(-4.08237667107798,-3.69276867472374,
-3.43303001048758,-3.17329134625142),(-0.204,0.204),.UNSPECIFIED.);
#18867=B_SPLINE_SURFACE_WITH_KNOTS('',3,3,((#56832,#56833,#56834,#56835),
(#56836,#56837,#56838,#56839),(#56840,#56841,#56842,#56843),(#56844,#56845,
#56846,#56847),(#56848,#56849,#56850,#56851),(#56852,#56853,#56854,#56855)),
 .UNSPECIFIED.,.F.,.F.,.F.,(4,1,1,4),(4,4),(-5.24964463690696,-5.08288401419063,
-4.74938156648641,-4.08236727834706),(-0.204,0.204009400954156),
 .UNSPECIFIED.);
#18868=B_SPLINE_SURFACE_WITH_KNOTS('',3,3,((#56857,#56858,#56859,#56860),
(#56861,#56862,#56863,#56864),(#56865,#56866,#56867,#56868),(#56869,#56870,
#56871,#56872),(#56873,#56874,#56875,#56876),(#56877,#56878,#56879,#56880),
(#56881,#56882,#56883,#56884)),.UNSPECIFIED.,.F.,.F.,.F.,(4,1,1,1,4),(4,
4),(-6.31492341312625,-6.01055536310239,-5.85837133809046,-5.5540032880666,
-5.24963523804274),(-0.204,0.204),.UNSPECIFIED.);
#18869=B_SPLINE_SURFACE_WITH_KNOTS('',3,3,((#56886,#56887,#56888,#56889),
(#56890,#56891,#56892,#56893),(#56894,#56895,#56896,#56897),(#56898,#56899,
#56900,#56901),(#56902,#56903,#56904,#56905),(#56906,#56907,#56908,#56909),
(#56910,#56911,#56912,#56913),(#56914,#56915,#56916,#56917),(#56918,#56919,
#56920,#56921),(#56922,#56923,#56924,#56925)),.UNSPECIFIED.,.F.,.F.,.F.,
(4,1,1,1,1,1,1,4),(4,4),(-7.69657954651299,-7.30181972429585,-7.10444046206193,
-6.90706119982801,-6.80837156871105,-6.70968193759409,-6.51230267536017,
-6.31492211537695),(-0.204,0.204001297749304),.UNSPECIFIED.);
#18870=B_SPLINE_SURFACE_WITH_KNOTS('',3,3,((#56927,#56928,#56929,#56930),
(#56931,#56932,#56933,#56934),(#56935,#56936,#56937,#56938),(#56939,#56940,
#56941,#56942),(#56943,#56944,#56945,#56946),(#56947,#56948,#56949,#56950),
(#56951,#56952,#56953,#56954),(#56955,#56956,#56957,#56958),(#56959,#56960,
#56961,#56962)),.UNSPECIFIED.,.F.,.F.,.F.,(4,1,1,1,1,1,4),(4,4),(-10.2944961530174,
-9.9233650238383,-9.5522338946592,-9.18110276548009,-8.43884050712189,-8.06770937794279,
-7.69657824876369),(-0.204,0.204),.UNSPECIFIED.);
#18871=B_SPLINE_SURFACE_WITH_KNOTS('',3,3,((#56964,#56965,#56966,#56967),
(#56968,#56969,#56970,#56971),(#56972,#56973,#56974,#56975),(#56976,#56977,
#56978,#56979),(#56980,#56981,#56982,#56983),(#56984,#56985,#56986,#56987),
(#56988,#56989,#56990,#56991),(#56992,#56993,#56994,#56995)),
 .UNSPECIFIED.,.F.,.F.,.F.,(4,1,1,1,1,4),(4,4),(-11.9813316832122,-11.8608434310554,
-11.7403551788986,-11.2584021702716,-10.7764491616445,-10.2944961530174),
(-0.204,0.204),.UNSPECIFIED.);
#18872=B_SPLINE_SURFACE_WITH_KNOTS('',3,3,((#56999,#57000,#57001,#57002),
(#57003,#57004,#57005,#57006),(#57007,#57008,#57009,#57010),(#57011,#57012,
#57013,#57014),(#57015,#57016,#57017,#57018),(#57019,#57020,#57021,#57022),
(#57023,#57024,#57025,#57026),(#57027,#57028,#57029,#57030),(#57031,#57032,
#57033,#57034),(#57035,#57036,#57037,#57038)),.UNSPECIFIED.,.F.,.F.,.F.,
(4,1,1,1,1,1,1,4),(4,4),(-16.6980910490008,-16.0242682824596,-14.6766227493771,
-14.0027999828359,-13.3289772162947,-12.6551544497534,-12.3182430664828,
-11.9813316832122),(-0.204,0.204),.UNSPECIFIED.);
#18873=B_SPLINE_SURFACE_WITH_KNOTS('',3,3,((#57042,#57043,#57044,#57045),
(#57046,#57047,#57048,#57049),(#57050,#57051,#57052,#57053),(#57054,#57055,
#57056,#57057),(#57058,#57059,#57060,#57061),(#57062,#57063,#57064,#57065),
(#57066,#57067,#57068,#57069),(#57070,#57071,#57072,#57073),(#57074,#57075,
#57076,#57077)),.UNSPECIFIED.,.F.,.F.,.F.,(4,1,1,1,1,1,4),(4,4),(-21.7463678506673,
-21.0251854504292,-19.5828206499531,-18.861638249715,-18.140455849477,-17.4192734492389,
-16.6980910490008),(-0.204,0.204),.UNSPECIFIED.);
#18874=B_SPLINE_SURFACE_WITH_KNOTS('',3,3,((#57081,#57082,#57083,#57084),
(#57085,#57086,#57087,#57088),(#57089,#57090,#57091,#57092),(#57093,#57094,
#57095,#57096),(#57097,#57098,#57099,#57100),(#57101,#57102,#57103,#57104),
(#57105,#57106,#57107,#57108)),.UNSPECIFIED.,.F.,.F.,.F.,(4,1,1,1,4),(4,
4),(-25.4580188592258,-24.3975168143727,-23.8672870216316,-22.8068274361495,
-21.7463253912963),(-0.204042459371017,0.204),.UNSPECIFIED.);
#18875=B_SPLINE_SURFACE_WITH_KNOTS('',3,3,((#57110,#57111,#57112,#57113),
(#57114,#57115,#57116,#57117),(#57118,#57119,#57120,#57121),(#57122,#57123,
#57124,#57125),(#57126,#57127,#57128,#57129)),.UNSPECIFIED.,.F.,.F.,.F.,
(4,1,4),(4,4),(-27.614177239717,-26.6900911654903,-25.4579763998548),(-0.204,
0.204044923106431),.UNSPECIFIED.);
#18876=B_SPLINE_SURFACE_WITH_KNOTS('',3,3,((#57131,#57132,#57133,#57134),
(#57135,#57136,#57137,#57138),(#57139,#57140,#57141,#57142),(#57143,#57144,
#57145,#57146),(#57147,#57148,#57149,#57150),(#57151,#57152,#57153,#57154),
(#57155,#57156,#57157,#57158),(#57159,#57160,#57161,#57162),(#57163,#57164,
#57165,#57166)),.UNSPECIFIED.,.F.,.F.,.F.,(4,1,1,1,1,1,4),(4,4),(4.87949017123957,
5.11201692992118,5.57705083698662,5.80956779051934,6.04208474405206,6.27460169758478,
6.507128569875),(-0.204009919306124,0.204),.UNSPECIFIED.);
#18877=B_SPLINE_SURFACE_WITH_KNOTS('',3,3,((#57171,#57172,#57173,#57174),
(#57175,#57176,#57177,#57178),(#57179,#57180,#57181,#57182),(#57183,#57184,
#57185,#57186),(#57187,#57188,#57189,#57190),(#57191,#57192,#57193,#57194),
(#57195,#57196,#57197,#57198)),.UNSPECIFIED.,.F.,.F.,.F.,(4,1,1,1,4),(4,
4),(2.69094642325915,3.62889794602885,4.25419896120866,4.56684946879856,
4.87949997638846),(-0.204,0.204),.UNSPECIFIED.);
#18878=B_SPLINE_SURFACE_WITH_KNOTS('',3,3,((#57200,#57201,#57202,#57203),
(#57204,#57205,#57206,#57207),(#57208,#57209,#57210,#57211),(#57212,#57213,
#57214,#57215),(#57216,#57217,#57218,#57219),(#57220,#57221,#57222,#57223),
(#57224,#57225,#57226,#57227),(#57228,#57229,#57230,#57231),(#57232,#57233,
#57234,#57235),(#57236,#57237,#57238,#57239)),.UNSPECIFIED.,.F.,.F.,.F.,
(4,1,1,1,1,1,1,4),(4,4),(1.28453619636216,1.68637707337851,1.88729094335464,
1.93751941084867,1.9877478783427,2.08820481333076,2.28911868330689,2.69095954767691),
(-0.204,0.204013137504486),.UNSPECIFIED.);
#18879=B_SPLINE_SURFACE_WITH_KNOTS('',3,3,((#57241,#57242,#57243,#57244),
(#57245,#57246,#57247,#57248),(#57249,#57250,#57251,#57252),(#57253,#57254,
#57255,#57256),(#57257,#57258,#57259,#57260),(#57261,#57262,#57263,#57264),
(#57265,#57266,#57267,#57268)),.UNSPECIFIED.,.F.,.F.,.F.,(4,1,1,1,4),(4,
4),(0.675577463735769,0.762573445120124,0.936565407888833,1.11055737065754,
1.28454933342625),(-0.204,0.204),.UNSPECIFIED.);
#18880=B_SPLINE_SURFACE_WITH_KNOTS('',3,3,((#57270,#57271,#57272,#57273),
(#57274,#57275,#57276,#57277),(#57278,#57279,#57280,#57281),(#57282,#57283,
#57284,#57285),(#57286,#57287,#57288,#57289),(#57290,#57291,#57292,#57293)),
 .UNSPECIFIED.,.F.,.F.,.F.,(4,1,1,4),(4,4),(0.0412699530886637,0.222500670416408,
0.403731387744152,0.675577463735769),(-0.204,0.204),.UNSPECIFIED.);
#18881=B_SPLINE_SURFACE_WITH_KNOTS('',3,3,((#57295,#57296,#57297,#57298),
(#57299,#57300,#57301,#57302),(#57303,#57304,#57305,#57306),(#57307,#57308,
#57309,#57310)),.UNSPECIFIED.,.F.,.F.,.F.,(4,4),(4,4),(0.,0.0412699530886637),
(-0.204,0.204),.UNSPECIFIED.);
#18882=B_SPLINE_SURFACE_WITH_KNOTS('',3,3,((#57312,#57313,#57314,#57315),
(#57316,#57317,#57318,#57319),(#57320,#57321,#57322,#57323),(#57324,#57325,
#57326,#57327),(#57328,#57329,#57330,#57331),(#57332,#57333,#57334,#57335)),
 .UNSPECIFIED.,.F.,.F.,.F.,(4,1,1,4),(4,4),(8.77692550510397,9.17723620667681,
9.97785760982251,11.5791004161139),(-0.204,0.204000856547217),
 .UNSPECIFIED.);
#18883=B_SPLINE_SURFACE_WITH_KNOTS('',3,3,((#57338,#57339,#57340,#57341),
(#57342,#57343,#57344,#57345),(#57346,#57347,#57348,#57349),(#57350,#57351,
#57352,#57353),(#57354,#57355,#57356,#57357)),.UNSPECIFIED.,.F.,.F.,.F.,
(4,1,4),(4,4),(6.63337020876143,7.5520367643368,8.77692550510397),(-0.204,
0.204),.UNSPECIFIED.);
#18884=B_SPLINE_SURFACE_WITH_KNOTS('',3,3,((#57359,#57360,#57361,#57362),
(#57363,#57364,#57365,#57366),(#57367,#57368,#57369,#57370),(#57371,#57372,
#57373,#57374),(#57375,#57376,#57377,#57378)),.UNSPECIFIED.,.F.,.F.,.F.,
(4,1,4),(4,4),(4.69944989998284,5.80455488046634,6.63338808485148),(-0.204017876090052,
0.204),.UNSPECIFIED.);
#18885=B_SPLINE_SURFACE_WITH_KNOTS('',3,3,((#57380,#57381,#57382,#57383),
(#57384,#57385,#57386,#57387),(#57388,#57389,#57390,#57391),(#57392,#57393,
#57394,#57395),(#57396,#57397,#57398,#57399),(#57400,#57401,#57402,#57403),
(#57404,#57405,#57406,#57407)),.UNSPECIFIED.,.F.,.F.,.F.,(4,1,1,1,4),(4,
4),(3.61161161838824,4.07783568596737,4.23324370849375,4.54405975354651,
4.69946777607289),(-0.204,0.204015895391734),.UNSPECIFIED.);
#18886=B_SPLINE_SURFACE_WITH_KNOTS('',3,3,((#57409,#57410,#57411,#57412),
(#57413,#57414,#57415,#57416),(#57417,#57418,#57419,#57420),(#57421,#57422,
#57423,#57424),(#57425,#57426,#57427,#57428),(#57429,#57430,#57431,#57432),
(#57433,#57434,#57435,#57436),(#57437,#57438,#57439,#57440),(#57441,#57442,
#57443,#57444),(#57445,#57446,#57447,#57448)),.UNSPECIFIED.,.F.,.F.,.F.,
(4,1,1,1,1,1,1,4),(4,4),(1.96419346040493,2.1995405412518,2.43488572077454,
2.67023090029728,2.90557607982002,3.14092125934276,3.3762664388655,3.61161352768816),
(-0.204001604230681,0.204001909299916),.UNSPECIFIED.);
#18887=B_SPLINE_SURFACE_WITH_KNOTS('',3,3,((#57452,#57453,#57454,#57455),
(#57456,#57457,#57458,#57459),(#57460,#57461,#57462,#57463),(#57464,#57465,
#57466,#57467),(#57468,#57469,#57470,#57471),(#57472,#57473,#57474,#57475),
(#57476,#57477,#57478,#57479),(#57480,#57481,#57482,#57483),(#57484,#57485,
#57486,#57487),(#57488,#57489,#57490,#57491),(#57492,#57493,#57494,#57495)),
 .UNSPECIFIED.,.F.,.F.,.F.,(4,1,1,1,1,1,1,1,4),(4,4),(-3.27331145294747E-6,
0.561198674779733,0.701498343474666,0.841798012169599,0.982097680864532,
1.12239734955947,1.40299668694933,1.6835960243392,1.96419863537987),(-0.204,
0.204003273650805),.UNSPECIFIED.);
#18888=B_SPLINE_SURFACE_WITH_KNOTS('',3,3,((#57497,#57498,#57499,#57500),
(#57501,#57502,#57503,#57504),(#57505,#57506,#57507,#57508),(#57509,#57510,
#57511,#57512),(#57513,#57514,#57515,#57516),(#57517,#57518,#57519,#57520),
(#57521,#57522,#57523,#57524),(#57525,#57526,#57527,#57528),(#57529,#57530,
#57531,#57532)),.UNSPECIFIED.,.F.,.F.,.F.,(4,1,1,1,1,1,4),(4,4),(-1.10870576037865,
-1.01091721837057,-0.913128676362484,-0.815340134354398,-0.766445863350356,
-0.619763050338228,-0.424185966322057),(-0.204,0.204),.UNSPECIFIED.);
#18889=B_SPLINE_SURFACE_WITH_KNOTS('',3,3,((#57537,#57538,#57539,#57540),
(#57541,#57542,#57543,#57544),(#57545,#57546,#57547,#57548),(#57549,#57550,
#57551,#57552),(#57553,#57554,#57555,#57556),(#57557,#57558,#57559,#57560),
(#57561,#57562,#57563,#57564),(#57565,#57566,#57567,#57568),(#57569,#57570,
#57571,#57572),(#57573,#57574,#57575,#57576)),.UNSPECIFIED.,.F.,.F.,.F.,
(4,1,1,1,1,1,1,4),(4,4),(-2.04907351897734,-1.91473526774895,-1.64605876529219,
-1.5117205140638,-1.37738226283542,-1.24304401160704,-1.17587488599285,
-1.10870576037865),(-0.204,0.204),.UNSPECIFIED.);
#18890=B_SPLINE_SURFACE_WITH_KNOTS('',3,3,((#57580,#57581,#57582,#57583),
(#57584,#57585,#57586,#57587),(#57588,#57589,#57590,#57591),(#57592,#57593,
#57594,#57595),(#57596,#57597,#57598,#57599),(#57600,#57601,#57602,#57603),
(#57604,#57605,#57606,#57607),(#57608,#57609,#57610,#57611),(#57612,#57613,
#57614,#57615),(#57616,#57617,#57618,#57619),(#57620,#57621,#57622,#57623)),
 .UNSPECIFIED.,.F.,.F.,.F.,(4,1,1,1,1,1,1,1,4),(4,4),(-3.79500150868533,
-3.54558322444133,-3.04674665595333,-2.92203751383133,-2.79732837170933,
-2.67261922958733,-2.54791008746534,-2.29849180322134,-2.04907351897734),
(-0.204,0.204),.UNSPECIFIED.);
#18891=B_SPLINE_SURFACE_WITH_KNOTS('',3,3,((#57627,#57628,#57629,#57630),
(#57631,#57632,#57633,#57634),(#57635,#57636,#57637,#57638),(#57639,#57640,
#57641,#57642),(#57643,#57644,#57645,#57646),(#57647,#57648,#57649,#57650),
(#57651,#57652,#57653,#57654),(#57655,#57656,#57657,#57658),(#57659,#57660,
#57661,#57662),(#57663,#57664,#57665,#57666),(#57667,#57668,#57669,#57670)),
 .UNSPECIFIED.,.F.,.F.,.F.,(4,1,1,1,1,1,1,1,4),(4,4),(-7.37894121078442,
-6.86694230253758,-5.84296203792017,-4.81898177330275,-4.56298670714839,
-4.46698855734051,-4.30699164099404,-4.05099657483969,-3.7949926101359),
(-0.204,0.204008898549431),.UNSPECIFIED.);
#18892=B_SPLINE_SURFACE_WITH_KNOTS('',3,3,((#57672,#57673,#57674,#57675),
(#57676,#57677,#57678,#57679),(#57680,#57681,#57682,#57683),(#57684,#57685,
#57686,#57687),(#57688,#57689,#57690,#57691),(#57692,#57693,#57694,#57695),
(#57696,#57697,#57698,#57699),(#57700,#57701,#57702,#57703)),
 .UNSPECIFIED.,.F.,.F.,.F.,(4,1,1,1,1,4),(4,4),(-13.6209874915031,-10.9458199140635,
-10.0540980442592,-9.16237617445491,-8.2706543046506,-7.3789298003802),
(-0.204,0.20400263446609),.UNSPECIFIED.);
#18893=B_SPLINE_SURFACE_WITH_KNOTS('',3,3,((#57705,#57706,#57707,#57708),
(#57709,#57710,#57711,#57712),(#57713,#57714,#57715,#57716),(#57717,#57718,
#57719,#57720),(#57721,#57722,#57723,#57724),(#57725,#57726,#57727,#57728),
(#57729,#57730,#57731,#57732),(#57733,#57734,#57735,#57736)),
 .UNSPECIFIED.,.F.,.F.,.F.,(4,1,1,1,1,4),(4,4),(-20.9230961620266,-17.7936201740765,
-15.7073028487765,-14.6641441861265,-14.1425648548015,-13.6209855234765),
(-0.204,0.204),.UNSPECIFIED.);
#18894=B_SPLINE_SURFACE_WITH_KNOTS('',3,3,((#57738,#57739,#57740,#57741),
(#57742,#57743,#57744,#57745),(#57746,#57747,#57748,#57749),(#57750,#57751,
#57752,#57753),(#57754,#57755,#57756,#57757),(#57758,#57759,#57760,#57761),
(#57762,#57763,#57764,#57765),(#57766,#57767,#57768,#57769)),
 .UNSPECIFIED.,.F.,.F.,.F.,(4,1,1,1,1,4),(4,4),(-29.2787346184417,-28.085071981811,
-25.6977467085495,-24.5040840719188,-23.310421435288,-20.9230961620266),
(-0.204,0.204),.UNSPECIFIED.);
#18895=B_SPLINE_SURFACE_WITH_KNOTS('',3,3,((#57771,#57772,#57773,#57774),
(#57775,#57776,#57777,#57778),(#57779,#57780,#57781,#57782),(#57783,#57784,
#57785,#57786),(#57787,#57788,#57789,#57790),(#57791,#57792,#57793,#57794),
(#57795,#57796,#57797,#57798)),.UNSPECIFIED.,.F.,.F.,.F.,(4,1,1,1,4),(4,
4),(-35.1303495878619,-33.4584584867811,-31.7865689394453,-30.9506241657775,
-29.2787331702972),(-0.204001840580079,0.204),.UNSPECIFIED.);
#18896=B_SPLINE_SURFACE_WITH_KNOTS('',3,3,((#57802,#57803,#57804,#57805),
(#57806,#57807,#57808,#57809),(#57810,#57811,#57812,#57813),(#57814,#57815,
#57816,#57817),(#57818,#57819,#57820,#57821),(#57822,#57823,#57824,#57825),
(#57826,#57827,#57828,#57829),(#57830,#57831,#57832,#57833),(#57834,#57835,
#57836,#57837)),.UNSPECIFIED.,.F.,.F.,.F.,(4,1,1,1,1,1,4),(4,4),(-40.4542048267256,
-38.9331028859802,-38.1725519156075,-37.4120009452349,-36.6514499748622,
-35.8908990044895,-35.1303480341168),(-0.204,0.204),.UNSPECIFIED.);
#18897=B_SPLINE_SURFACE_WITH_KNOTS('',3,3,((#57841,#57842,#57843,#57844),
(#57845,#57846,#57847,#57848),(#57849,#57850,#57851,#57852),(#57853,#57854,
#57855,#57856),(#57857,#57858,#57859,#57860),(#57861,#57862,#57863,#57864),
(#57865,#57866,#57867,#57868),(#57869,#57870,#57871,#57872)),
 .UNSPECIFIED.,.F.,.F.,.F.,(4,1,1,1,1,4),(4,4),(-52.0762703289969,-47.0953817384218,
-43.7747932825737,-42.1144990546496,-41.2843519406876,-40.4541989180265),
(-0.204,0.204005908699072),.UNSPECIFIED.);
#18898=B_SPLINE_SURFACE_WITH_KNOTS('',3,3,((#57874,#57875,#57876,#57877),
(#57878,#57879,#57880,#57881),(#57882,#57883,#57884,#57885),(#57886,#57887,
#57888,#57889),(#57890,#57891,#57892,#57893)),.UNSPECIFIED.,.F.,.F.,.F.,
(4,1,4),(4,4),(-66.1031756239825,-60.0916422517874,-52.076264422194),(-0.204,
0.204),.UNSPECIFIED.);
#18899=B_SPLINE_SURFACE_WITH_KNOTS('',3,3,((#57895,#57896,#57897,#57898),
(#57899,#57900,#57901,#57902),(#57903,#57904,#57905,#57906),(#57907,#57908,
#57909,#57910)),.UNSPECIFIED.,.F.,.F.,.F.,(4,4),(4,4),(-75.2949305236969,
-66.1031756239825),(-0.204,0.204),.UNSPECIFIED.);
#18900=B_SPLINE_SURFACE_WITH_KNOTS('',3,3,((#57912,#57913,#57914,#57915),
(#57916,#57917,#57918,#57919),(#57920,#57921,#57922,#57923),(#57924,#57925,
#57926,#57927)),.UNSPECIFIED.,.F.,.F.,.F.,(4,4),(4,4),(-76.3862538744791,
-75.2949305236969),(-0.204,0.204000226653285),.UNSPECIFIED.);
#18901=B_SPLINE_SURFACE_WITH_KNOTS('',3,3,((#57929,#57930,#57931,#57932),
(#57933,#57934,#57935,#57936),(#57937,#57938,#57939,#57940),(#57941,#57942,
#57943,#57944),(#57945,#57946,#57947,#57948),(#57949,#57950,#57951,#57952),
(#57953,#57954,#57955,#57956),(#57957,#57958,#57959,#57960)),
 .UNSPECIFIED.,.F.,.F.,.F.,(4,1,1,1,1,4),(4,4),(2.10086200096182,2.11383027239681,
2.12678492441379,2.13973957643076,2.15269422844774,2.19157180391669),(-0.204,
0.204013619418013),.UNSPECIFIED.);
#18902=B_SPLINE_SURFACE_WITH_KNOTS('',3,3,((#57965,#57966,#57967,#57968),
(#57969,#57970,#57971,#57972),(#57973,#57974,#57975,#57976),(#57977,#57978,
#57979,#57980),(#57981,#57982,#57983,#57984),(#57985,#57986,#57987,#57988),
(#57989,#57990,#57991,#57992),(#57993,#57994,#57995,#57996),(#57997,#57998,
#57999,#58000)),.UNSPECIFIED.,.F.,.F.,.F.,(4,1,1,1,1,1,4),(4,4),(2.03661045158091,
2.0549719283806,2.06415266678044,2.07333340518029,2.08251414358014,2.09169488197998,
2.10087562037983),(-0.204,0.204),.UNSPECIFIED.);
#18903=B_SPLINE_SURFACE_WITH_KNOTS('',3,3,((#58002,#58003,#58004,#58005),
(#58006,#58007,#58008,#58009),(#58010,#58011,#58012,#58013),(#58014,#58015,
#58016,#58017),(#58018,#58019,#58020,#58021),(#58022,#58023,#58024,#58025),
(#58026,#58027,#58028,#58029),(#58030,#58031,#58032,#58033)),
 .UNSPECIFIED.,.F.,.F.,.F.,(4,1,1,1,1,4),(4,4),(1.96650114296421,1.97401285460172,
1.97651675848088,1.98653237399755,2.00656360503089,2.03661045158091),(-0.204,
0.204),.UNSPECIFIED.);
#18904=B_SPLINE_SURFACE_WITH_KNOTS('',3,3,((#58035,#58036,#58037,#58038),
(#58039,#58040,#58041,#58042),(#58043,#58044,#58045,#58046),(#58047,#58048,
#58049,#58050)),.UNSPECIFIED.,.F.,.F.,.F.,(4,4),(4,4),(1.9008556588209,
1.96650114296421),(-0.204000199215518,0.204),.UNSPECIFIED.);
#18905=B_SPLINE_SURFACE_WITH_KNOTS('',3,3,((#58052,#58053,#58054,#58055),
(#58056,#58057,#58058,#58059),(#58060,#58061,#58062,#58063),(#58064,#58065,
#58066,#58067),(#58068,#58069,#58070,#58071),(#58072,#58073,#58074,#58075),
(#58076,#58077,#58078,#58079),(#58080,#58081,#58082,#58083),(#58084,#58085,
#58086,#58087)),.UNSPECIFIED.,.F.,.F.,.F.,(4,1,1,1,1,1,4),(4,4),(1.82758018188507,
1.83805116497033,1.84328487279121,1.85898599625385,1.87992082753738,1.89038824317914,
1.9008592262644),(-0.204,0.204003567443499),.UNSPECIFIED.);
#18906=B_SPLINE_SURFACE_WITH_KNOTS('',3,3,((#58089,#58090,#58091,#58092),
(#58093,#58094,#58095,#58096),(#58097,#58098,#58099,#58100),(#58101,#58102,
#58103,#58104),(#58105,#58106,#58107,#58108),(#58109,#58110,#58111,#58112)),
 .UNSPECIFIED.,.F.,.F.,.F.,(4,1,1,4),(4,4),(1.80197179046417,1.80928949299685,
1.8129483442632,1.82758374932857),(-0.204,0.204000646491389),
 .UNSPECIFIED.);
#18907=B_SPLINE_SURFACE_WITH_KNOTS('',3,3,((#58114,#58115,#58116,#58117),
(#58118,#58119,#58120,#58121),(#58122,#58123,#58124,#58125),(#58126,#58127,
#58128,#58129),(#58130,#58131,#58132,#58133),(#58134,#58135,#58136,#58137),
(#58138,#58139,#58140,#58141),(#58142,#58143,#58144,#58145),(#58146,#58147,
#58148,#58149),(#58150,#58151,#58152,#58153),(#58154,#58155,#58156,#58157),
(#58158,#58159,#58160,#58161)),.UNSPECIFIED.,.F.,.F.,.F.,(4,1,1,1,1,1,1,
1,1,4),(4,4),(1.56845471413357,1.60181606521468,1.66853464029784,1.70189392783942,
1.735253215381,1.7435930372664,1.75193285915179,1.76861250292259,1.78529214669338,
1.8019738540036),(-0.204001877008512,0.204002063539524),.UNSPECIFIED.);
#18908=B_SPLINE_SURFACE_WITH_KNOTS('',3,3,((#58163,#58164,#58165,#58166),
(#58167,#58168,#58169,#58170),(#58171,#58172,#58173,#58174),(#58175,#58176,
#58177,#58178),(#58179,#58180,#58181,#58182),(#58183,#58184,#58185,#58186),
(#58187,#58188,#58189,#58190)),.UNSPECIFIED.,.F.,.F.,.F.,(4,1,1,1,4),(4,
4),(1.43249195629979,1.45191550221026,1.4616272751655,1.4907625940312,1.56845677767309),
(-0.204,0.204),.UNSPECIFIED.);
#18909=B_SPLINE_SURFACE_WITH_KNOTS('',3,3,((#58192,#58193,#58194,#58195),
(#58196,#58197,#58198,#58199),(#58200,#58201,#58202,#58203),(#58204,#58205,
#58206,#58207),(#58208,#58209,#58210,#58211),(#58212,#58213,#58214,#58215),
(#58216,#58217,#58218,#58219),(#58220,#58221,#58222,#58223)),
 .UNSPECIFIED.,.F.,.F.,.F.,(4,1,1,1,1,4),(4,4),(1.26182357380732,1.33496716630409,
1.35934836380302,1.38372956130194,1.3959201600514,1.43249195629979),(-0.204,
0.204),.UNSPECIFIED.);
#18910=B_SPLINE_SURFACE_WITH_KNOTS('',3,3,((#58225,#58226,#58227,#58228),
(#58229,#58230,#58231,#58232),(#58233,#58234,#58235,#58236),(#58237,#58238,
#58239,#58240),(#58241,#58242,#58243,#58244),(#58245,#58246,#58247,#58248),
(#58249,#58250,#58251,#58252),(#58253,#58254,#58255,#58256),(#58257,#58258,
#58259,#58260),(#58261,#58262,#58263,#58264),(#58265,#58266,#58267,#58268),
(#58269,#58270,#58271,#58272),(#58273,#58274,#58275,#58276),(#58277,#58278,
#58279,#58280),(#58281,#58282,#58283,#58284),(#58285,#58286,#58287,#58288)),
 .UNSPECIFIED.,.F.,.F.,.F.,(4,1,1,1,1,1,1,1,1,1,1,1,1,4),(4,4),(0.756789029878484,
0.828970599685942,0.901112762039505,0.919148302627896,0.937183843216286,
0.973254924393068,1.00932600556985,1.02736154615824,1.03637931645244,1.04539708674663,
1.11753924910019,1.18968141145376,1.22575249263054,1.26186298126122),(-0.204039407453895,
0.204016158273927),.UNSPECIFIED.);
#18911=B_SPLINE_SURFACE_WITH_KNOTS('',3,3,((#58290,#58291,#58292,#58293),
(#58294,#58295,#58296,#58297),(#58298,#58299,#58300,#58301),(#58302,#58303,
#58304,#58305),(#58306,#58307,#58308,#58309),(#58310,#58311,#58312,#58313),
(#58314,#58315,#58316,#58317),(#58318,#58319,#58320,#58321),(#58322,#58323,
#58324,#58325),(#58326,#58327,#58328,#58329)),.UNSPECIFIED.,.F.,.F.,.F.,
(4,1,1,1,1,1,1,4),(4,4),(0.,0.21623669638068,0.324355044571019,0.432473392761359,
0.540591740951699,0.648710089142039,0.702769263237209,0.756836420205482),
(-0.204,0.204007982873103),.UNSPECIFIED.);
#18912=B_SPLINE_SURFACE_WITH_KNOTS('',3,3,((#58331,#58332,#58333,#58334),
(#58335,#58336,#58337,#58338),(#58339,#58340,#58341,#58342),(#58343,#58344,
#58345,#58346),(#58347,#58348,#58349,#58350),(#58351,#58352,#58353,#58354),
(#58355,#58356,#58357,#58358),(#58359,#58360,#58361,#58362),(#58363,#58364,
#58365,#58366)),.UNSPECIFIED.,.F.,.F.,.F.,(4,1,1,1,1,1,4),(4,4),(13.8978590689825,
14.2193450517567,14.862262798083,15.1837216712462,15.5051805444094,15.8266394175726,
16.1481253792677),(-0.204025631400802,0.204027109611016),.UNSPECIFIED.);
#18913=B_SPLINE_SURFACE_WITH_KNOTS('',3,3,((#58369,#58370,#58371,#58372),
(#58373,#58374,#58375,#58376),(#58377,#58378,#58379,#58380),(#58381,#58382,
#58383,#58384),(#58385,#58386,#58387,#58388),(#58389,#58390,#58391,#58392)),
 .UNSPECIFIED.,.F.,.F.,.F.,(4,1,1,4),(4,4),(12.3501192806041,13.0134488895805,
13.455667534087,13.8978877785644),(-0.204,0.204001642216694),
 .UNSPECIFIED.);
#18914=B_SPLINE_SURFACE_WITH_KNOTS('',3,3,((#58394,#58395,#58396,#58397),
(#58398,#58399,#58400,#58401),(#58402,#58403,#58404,#58405),(#58406,#58407,
#58408,#58409),(#58410,#58411,#58412,#58413),(#58414,#58415,#58416,#58417),
(#58418,#58419,#58420,#58421),(#58422,#58423,#58424,#58425),(#58426,#58427,
#58428,#58429)),.UNSPECIFIED.,.F.,.F.,.F.,(4,1,1,1,1,1,4),(4,4),(10.8793710892452,
11.0894782083274,11.2995853274097,11.5096924464919,11.7197995655741,11.9299066846563,
12.3501209228208),(-0.204,0.204),.UNSPECIFIED.);
#18915=B_SPLINE_SURFACE_WITH_KNOTS('',3,3,((#58431,#58432,#58433,#58434),
(#58435,#58436,#58437,#58438),(#58439,#58440,#58441,#58442),(#58443,#58444,
#58445,#58446),(#58447,#58448,#58449,#58450),(#58451,#58452,#58453,#58454),
(#58455,#58456,#58457,#58458),(#58459,#58460,#58461,#58462),(#58463,#58464,
#58465,#58466)),.UNSPECIFIED.,.F.,.F.,.F.,(4,1,1,1,1,1,4),(4,4),(7.9278984945301,
8.77117777664964,9.19281643916875,9.61445510168786,10.036093764207,10.4577324267261,
10.8793730468907),(-0.204,0.204031354795924),.UNSPECIFIED.);
#18916=B_SPLINE_SURFACE_WITH_KNOTS('',3,3,((#58468,#58469,#58470,#58471),
(#58472,#58473,#58474,#58475),(#58476,#58477,#58478,#58479),(#58480,#58481,
#58482,#58483)),.UNSPECIFIED.,.F.,.F.,.F.,(4,4),(4,4),(6.94071132372615,
7.92790045161141),(-0.204,0.20400038518575),.UNSPECIFIED.);
#18917=B_SPLINE_SURFACE_WITH_KNOTS('',3,3,((#58485,#58486,#58487,#58488),
(#58489,#58490,#58491,#58492),(#58493,#58494,#58495,#58496),(#58497,#58498,
#58499,#58500),(#58501,#58502,#58503,#58504),(#58505,#58506,#58507,#58508),
(#58509,#58510,#58511,#58512),(#58513,#58514,#58515,#58516),(#58517,#58518,
#58519,#58520),(#58521,#58522,#58523,#58524),(#58525,#58526,#58527,#58528),
(#58529,#58530,#58531,#58532)),.UNSPECIFIED.,.F.,.F.,.F.,(4,1,1,1,1,1,1,
1,1,4),(4,4),(4.48918216137468,4.66429138725693,4.75184600019805,4.83940061313917,
5.53983751666817,5.89005596843266,6.06516519431491,6.24027442019716,6.59049287196166,
6.94071132372615),(-0.204,0.204015052160367),.UNSPECIFIED.);
#18918=B_SPLINE_SURFACE_WITH_KNOTS('',3,3,((#58534,#58535,#58536,#58537),
(#58538,#58539,#58540,#58541),(#58542,#58543,#58544,#58545),(#58546,#58547,
#58548,#58549)),.UNSPECIFIED.,.F.,.F.,.F.,(4,4),(4,4),(3.57654770812807,
4.48918216137468),(-0.204,0.204),.UNSPECIFIED.);
#18919=B_SPLINE_SURFACE_WITH_KNOTS('',3,3,((#58551,#58552,#58553,#58554),
(#58555,#58556,#58557,#58558),(#58559,#58560,#58561,#58562),(#58563,#58564,
#58565,#58566),(#58567,#58568,#58569,#58570),(#58571,#58572,#58573,#58574)),
 .UNSPECIFIED.,.F.,.F.,.F.,(4,1,1,4),(4,4),(2.87518401914012,3.17576845727781,
3.37615808270294,3.57654770812807),(-0.204,0.204),.UNSPECIFIED.);
#18920=B_SPLINE_SURFACE_WITH_KNOTS('',3,3,((#58576,#58577,#58578,#58579),
(#58580,#58581,#58582,#58583),(#58584,#58585,#58586,#58587),(#58588,#58589,
#58590,#58591),(#58592,#58593,#58594,#58595),(#58596,#58597,#58598,#58599),
(#58600,#58601,#58602,#58603),(#58604,#58605,#58606,#58607)),
 .UNSPECIFIED.,.F.,.F.,.F.,(4,1,1,1,1,4),(4,4),(2.26956600807314,2.44259972552085,
2.5291165842447,2.61563344296856,2.70215030169241,2.87518401914012),(-0.204,
0.204),.UNSPECIFIED.);
#18921=B_SPLINE_SURFACE_WITH_KNOTS('',3,3,((#58609,#58610,#58611,#58612),
(#58613,#58614,#58615,#58616),(#58617,#58618,#58619,#58620),(#58621,#58622,
#58623,#58624),(#58625,#58626,#58627,#58628),(#58629,#58630,#58631,#58632),
(#58633,#58634,#58635,#58636),(#58637,#58638,#58639,#58640),(#58641,#58642,
#58643,#58644)),.UNSPECIFIED.,.F.,.F.,.F.,(4,1,1,1,1,1,4),(4,4),(1.46286168120391,
1.57811142102339,1.80859628337331,1.92383871454827,2.03908114572322,2.15432357689818,
2.26957331671767),(-0.204,0.204007308644527),.UNSPECIFIED.);
#18922=B_SPLINE_SURFACE_WITH_KNOTS('',3,3,((#58648,#58649,#58650,#58651),
(#58652,#58653,#58654,#58655),(#58656,#58657,#58658,#58659),(#58660,#58661,
#58662,#58663),(#58664,#58665,#58666,#58667),(#58668,#58669,#58670,#58671),
(#58672,#58673,#58674,#58675),(#58676,#58677,#58678,#58679),(#58680,#58681,
#58682,#58683)),.UNSPECIFIED.,.F.,.F.,.F.,(4,1,1,1,1,1,4),(4,4),(0.,0.208981284264062,
0.626943852792187,0.835925137056249,1.04490642132031,1.25388770558437,1.46286898984844),
(-0.204,0.204),.UNSPECIFIED.);
#18923=B_SPLINE_SURFACE_WITH_KNOTS('',3,3,((#58685,#58686,#58687,#58688),
(#58689,#58690,#58691,#58692),(#58693,#58694,#58695,#58696),(#58697,#58698,
#58699,#58700),(#58701,#58702,#58703,#58704),(#58705,#58706,#58707,#58708),
(#58709,#58710,#58711,#58712),(#58713,#58714,#58715,#58716)),
 .UNSPECIFIED.,.F.,.F.,.F.,(4,1,1,1,1,4),(4,4),(16.1480982907358,17.1122318399124,
17.4336096896379,17.7549875393634,17.9156764642262,18.3977432388145),(-0.204,
0.204),.UNSPECIFIED.);
#18924=B_SPLINE_SURFACE_WITH_KNOTS('',3,3,((#58717,#58718,#58719,#58720),
(#58721,#58722,#58723,#58724),(#58725,#58726,#58727,#58728),(#58729,#58730,
#58731,#58732),(#58733,#58734,#58735,#58736),(#58737,#58738,#58739,#58740),
(#58741,#58742,#58743,#58744),(#58745,#58746,#58747,#58748),(#58749,#58750,
#58751,#58752),(#58753,#58754,#58755,#58756),(#58757,#58758,#58759,#58760)),
 .UNSPECIFIED.,.F.,.F.,.F.,(4,1,1,1,1,1,1,1,4),(4,4),(2.19155818449868,
2.25090656855756,2.280580760587,2.31025495261644,2.32509204863116,2.33992914464588,
2.36960333667532,2.48830010479308,2.60699687291084),(-0.204,0.204),
 .UNSPECIFIED.);
#18925=B_SPLINE_SURFACE_WITH_KNOTS('',3,3,((#58761,#58762,#58763,#58764),
(#58765,#58766,#58767,#58768),(#58769,#58770,#58771,#58772),(#58773,#58774,
#58775,#58776)),.UNSPECIFIED.,.F.,.F.,.F.,(4,4),(4,4),(-0.424185966322057,
0.),(-0.204,0.204),.UNSPECIFIED.);
#18926=B_SPLINE_SURFACE_WITH_KNOTS('',3,3,((#58777,#58778,#58779,#58780),
(#58781,#58782,#58783,#58784),(#58785,#58786,#58787,#58788),(#58789,#58790,
#58791,#58792),(#58793,#58794,#58795,#58796),(#58797,#58798,#58799,#58800),
(#58801,#58802,#58803,#58804),(#58805,#58806,#58807,#58808),(#58809,#58810,
#58811,#58812),(#58813,#58814,#58815,#58816),(#58817,#58818,#58819,#58820),
(#58821,#58822,#58823,#58824),(#58825,#58826,#58827,#58828),(#58829,#58830,
#58831,#58832),(#58833,#58834,#58835,#58836),(#58837,#58838,#58839,#58840),
(#58841,#58842,#58843,#58844),(#58845,#58846,#58847,#58848)),
 .UNSPECIFIED.,.F.,.F.,.F.,(4,1,1,1,1,1,1,1,1,1,1,1,1,1,1,4),(4,4),(0.,
0.0536833715747986,0.107366743149597,0.161050114724396,0.214733486299194,
0.228154329192894,0.241575172086594,0.268416857873993,0.322100229448792,
0.37578360102359,0.429466972598389,0.509992029960587,0.590517087322785,
0.644200458897583,0.697883830472382,0.75156720204718),(-0.204,0.204),
 .UNSPECIFIED.);
#18927=B_SPLINE_SURFACE_WITH_KNOTS('',3,3,((#58850,#58851,#58852,#58853),
(#58854,#58855,#58856,#58857),(#58858,#58859,#58860,#58861),(#58862,#58863,
#58864,#58865)),.UNSPECIFIED.,.F.,.F.,.F.,(4,4),(4,4),(11.5791004161139,
11.7855397152994),(-0.204,0.20400006877991),.UNSPECIFIED.);
#18928=B_SPLINE_SURFACE_WITH_KNOTS('',3,3,((#58866,#58867,#58868,#58869),
(#58870,#58871,#58872,#58873),(#58874,#58875,#58876,#58877),(#58878,#58879,
#58880,#58881),(#58882,#58883,#58884,#58885),(#58886,#58887,#58888,#58889),
(#58890,#58891,#58892,#58893),(#58894,#58895,#58896,#58897),(#58898,#58899,
#58900,#58901),(#58902,#58903,#58904,#58905),(#58906,#58907,#58908,#58909),
(#58910,#58911,#58912,#58913),(#58914,#58915,#58916,#58917)),
 .UNSPECIFIED.,.F.,.F.,.F.,(4,1,1,1,1,1,1,1,1,1,4),(4,4),(6.50711619353453,
6.712779658626,6.91844066613449,6.96985591801162,7.02127116988874,7.22693217739724,
7.32976268115149,7.48400843678286,7.53542368865998,7.74108469616848,7.94674816125994),
(-0.204002457582968,0.204),.UNSPECIFIED.);
#18929=B_SPLINE_SURFACE_WITH_KNOTS('',3,3,((#58918,#58919,#58920,#58921,
#58922),(#58923,#58924,#58925,#58926,#58927),(#58928,#58929,#58930,#58931,
#58932),(#58933,#58934,#58935,#58936,#58937),(#58938,#58939,#58940,#58941,
#58942),(#58943,#58944,#58945,#58946,#58947),(#58948,#58949,#58950,#58951,
#58952),(#58953,#58954,#58955,#58956,#58957),(#58958,#58959,#58960,#58961,
#58962),(#58963,#58964,#58965,#58966,#58967),(#58968,#58969,#58970,#58971,
#58972),(#58973,#58974,#58975,#58976,#58977),(#58978,#58979,#58980,#58981,
#58982),(#58983,#58984,#58985,#58986,#58987),(#58988,#58989,#58990,#58991,
#58992),(#58993,#58994,#58995,#58996,#58997),(#58998,#58999,#59000,#59001,
#59002),(#59003,#59004,#59005,#59006,#59007),(#59008,#59009,#59010,#59011,
#59012),(#59013,#59014,#59015,#59016,#59017),(#59018,#59019,#59020,#59021,
#59022),(#59023,#59024,#59025,#59026,#59027),(#59028,#59029,#59030,#59031,
#59032),(#59033,#59034,#59035,#59036,#59037),(#59038,#59039,#59040,#59041,
#59042),(#59043,#59044,#59045,#59046,#59047)),.UNSPECIFIED.,.F.,.F.,.F.,
(4,1,1,1,1,1,1,1,1,1,1,1,1,1,1,1,1,1,1,1,1,1,1,4),(4,1,4),(0.,0.0539979975781232,
0.107995995156246,0.215991990312493,0.269989987890616,0.323987985468739,
0.377985983046862,0.431983980624985,0.458982979414047,0.472482478808578,
0.485981978203109,0.49948147759764,0.51298097699217,0.519730726689436,0.521418164113752,
0.526480476386701,0.529855351235334,0.533230226083967,0.536605100932599,
0.538292538356915,0.539979975781232,0.593977973359355,0.647975970937478,
0.755971966093725),(-0.204000260274416,-0.0291428571428571,0.204),
 .UNSPECIFIED.);
#18930=B_SPLINE_SURFACE_WITH_KNOTS('',3,3,((#59049,#59050,#59051,#59052),
(#59053,#59054,#59055,#59056),(#59057,#59058,#59059,#59060),(#59061,#59062,
#59063,#59064)),.UNSPECIFIED.,.F.,.F.,.F.,(4,4),(4,4),(-0.0833603842763964,
0.),(-0.204,0.204),.UNSPECIFIED.);
#18960=ADVANCED_FACE('',(#5026),#18849,.F.);
#18961=ADVANCED_FACE('',(#5027),#4554,.F.);
#18962=ADVANCED_FACE('',(#5028,#1694,#1695,#1696,#1697,#1698),#18850,.F.);
#18963=ADVANCED_FACE('',(#5029),#18851,.F.);
#18964=ADVANCED_FACE('',(#5030,#1699,#1700,#1701,#1702),#18852,.T.);
#18965=ADVANCED_FACE('',(#5031),#18853,.F.);
#18966=ADVANCED_FACE('',(#5032),#4555,.F.);
#18967=ADVANCED_FACE('',(#5033),#18854,.F.);
#18968=ADVANCED_FACE('',(#5034),#18855,.F.);
#18969=ADVANCED_FACE('',(#5035),#4556,.F.);
#18970=ADVANCED_FACE('',(#5036),#18856,.F.);
#18971=ADVANCED_FACE('',(#5037),#18857,.F.);
#18972=ADVANCED_FACE('',(#5038),#4557,.F.);
#18973=ADVANCED_FACE('',(#5039),#18858,.F.);
#18974=ADVANCED_FACE('',(#5040),#18859,.F.);
#18975=ADVANCED_FACE('',(#5041),#18860,.F.);
#18976=ADVANCED_FACE('',(#5042),#18861,.F.);
#18977=ADVANCED_FACE('',(#5043),#18862,.F.);
#18978=ADVANCED_FACE('',(#5044),#1363,.F.);
#18979=ADVANCED_FACE('',(#5045),#18863,.F.);
#18980=ADVANCED_FACE('',(#5046),#18864,.F.);
#18981=ADVANCED_FACE('',(#5047),#18865,.F.);
#18982=ADVANCED_FACE('',(#5048),#18866,.F.);
#18983=ADVANCED_FACE('',(#5049),#18867,.F.);
#18984=ADVANCED_FACE('',(#5050),#18868,.F.);
#18985=ADVANCED_FACE('',(#5051),#18869,.F.);
#18986=ADVANCED_FACE('',(#5052),#18870,.F.);
#18987=ADVANCED_FACE('',(#5053),#18871,.F.);
#18988=ADVANCED_FACE('',(#5054),#18872,.F.);
#18989=ADVANCED_FACE('',(#5055),#18873,.F.);
#18990=ADVANCED_FACE('',(#5056),#18874,.F.);
#18991=ADVANCED_FACE('',(#5057),#18875,.F.);
#18992=ADVANCED_FACE('',(#5058),#18876,.F.);
#18993=ADVANCED_FACE('',(#5059),#18877,.F.);
#18994=ADVANCED_FACE('',(#5060),#18878,.F.);
#18995=ADVANCED_FACE('',(#5061),#18879,.F.);
#18996=ADVANCED_FACE('',(#5062),#18880,.F.);
#18997=ADVANCED_FACE('',(#5063),#18881,.F.);
#18998=ADVANCED_FACE('',(#5064),#18882,.F.);
#18999=ADVANCED_FACE('',(#5065),#18883,.F.);
#19000=ADVANCED_FACE('',(#5066),#18884,.F.);
#19001=ADVANCED_FACE('',(#5067),#18885,.F.);
#19002=ADVANCED_FACE('',(#5068),#18886,.F.);
#19003=ADVANCED_FACE('',(#5069),#18887,.F.);
#19004=ADVANCED_FACE('',(#5070),#18888,.F.);
#19005=ADVANCED_FACE('',(#5071),#18889,.F.);
#19006=ADVANCED_FACE('',(#5072),#18890,.F.);
#19007=ADVANCED_FACE('',(#5073),#18891,.F.);
#19008=ADVANCED_FACE('',(#5074),#18892,.F.);
#19009=ADVANCED_FACE('',(#5075),#18893,.F.);
#19010=ADVANCED_FACE('',(#5076),#18894,.F.);
#19011=ADVANCED_FACE('',(#5077),#18895,.F.);
#19012=ADVANCED_FACE('',(#5078),#18896,.F.);
#19013=ADVANCED_FACE('',(#5079),#18897,.F.);
#19014=ADVANCED_FACE('',(#5080),#18898,.F.);
#19015=ADVANCED_FACE('',(#5081),#18899,.F.);
#19016=ADVANCED_FACE('',(#5082),#18900,.F.);
#19017=ADVANCED_FACE('',(#5083),#18901,.F.);
#19018=ADVANCED_FACE('',(#5084),#18902,.F.);
#19019=ADVANCED_FACE('',(#5085),#18903,.F.);
#19020=ADVANCED_FACE('',(#5086),#18904,.F.);
#19021=ADVANCED_FACE('',(#5087),#18905,.F.);
#19022=ADVANCED_FACE('',(#5088),#18906,.F.);
#19023=ADVANCED_FACE('',(#5089),#18907,.F.);
#19024=ADVANCED_FACE('',(#5090),#18908,.F.);
#19025=ADVANCED_FACE('',(#5091),#18909,.F.);
#19026=ADVANCED_FACE('',(#5092),#18910,.F.);
#19027=ADVANCED_FACE('',(#5093),#18911,.F.);
#19028=ADVANCED_FACE('',(#5094),#18912,.F.);
#19029=ADVANCED_FACE('',(#5095),#18913,.F.);
#19030=ADVANCED_FACE('',(#5096),#18914,.F.);
#19031=ADVANCED_FACE('',(#5097),#18915,.F.);
#19032=ADVANCED_FACE('',(#5098),#18916,.F.);
#19033=ADVANCED_FACE('',(#5099),#18917,.F.);
#19034=ADVANCED_FACE('',(#5100),#18918,.F.);
#19035=ADVANCED_FACE('',(#5101),#18919,.F.);
#19036=ADVANCED_FACE('',(#5102),#18920,.F.);
#19037=ADVANCED_FACE('',(#5103),#18921,.F.);
#19038=ADVANCED_FACE('',(#5104),#18922,.F.);
#19039=ADVANCED_FACE('',(#5105),#18923,.F.);
#19040=ADVANCED_FACE('',(#5106),#18924,.F.);
#19041=ADVANCED_FACE('',(#5107),#18925,.F.);
#19042=ADVANCED_FACE('',(#5108),#18926,.F.);
#19043=ADVANCED_FACE('',(#5109),#18927,.F.);
#19044=ADVANCED_FACE('',(#5110),#18928,.F.);
#19045=ADVANCED_FACE('',(#5111),#18929,.F.);
#19046=ADVANCED_FACE('',(#5112),#18930,.F.);
#20117=CLOSED_SHELL('',(#18960,#18961,#18962,#18963,#18964,#18965,#18966,
#18967,#18968,#18969,#18970,#18971,#18972,#18973,#18974,#18975,#18976,#18977,
#18978,#18979,#18980,#18981,#18982,#18983,#18984,#18985,#18986,#18987,#18988,
#18989,#18990,#18991,#18992,#18993,#18994,#18995,#18996,#18997,#18998,#18999,
#19000,#19001,#19002,#19003,#19004,#19005,#19006,#19007,#19008,#19009,#19010,
#19011,#19012,#19013,#19014,#19015,#19016,#19017,#19018,#19019,#19020,#19021,
#19022,#19023,#19024,#19025,#19026,#19027,#19028,#19029,#19030,#19031,#19032,
#19033,#19034,#19035,#19036,#19037,#19038,#19039,#19040,#19041,#19042,#19043,
#19044,#19045,#19046));
#20335=AXIS2_PLACEMENT_3D('',#28195,#22527,#22528);
#20336=AXIS2_PLACEMENT_3D('',#28807,#22529,#22530);
#20337=AXIS2_PLACEMENT_3D('',#40840,#22532,#22533);
#20338=AXIS2_PLACEMENT_3D('',#54981,#22534,#22535);
#20339=AXIS2_PLACEMENT_3D('',#55726,#22536,#22537);
#20340=AXIS2_PLACEMENT_3D('',#56080,#22539,#22540);
#20341=AXIS2_PLACEMENT_3D('',#56332,#22542,#22543);
#20342=AXIS2_PLACEMENT_3D('',#56726,#22549,#22550);
#22527=DIRECTION('axis',(0.,0.,1.));
#22528=DIRECTION('refdir',(1.,0.,0.));
#22529=DIRECTION('center_axis',(0.,1.,0.));
#22530=DIRECTION('ref_axis',(1.,0.,0.));
#22531=DIRECTION('',(0.,1.,0.));
#22532=DIRECTION('center_axis',(-0.0253793612844622,-0.999677881145026,
0.000148223423376537));
#22533=DIRECTION('ref_axis',(-0.178708422703468,0.00439108419345073,-0.983892279690437));
#22534=DIRECTION('center_axis',(0.0255908057683819,0.999672491941936,-0.000139695117279073));
#22535=DIRECTION('ref_axis',(0.172447171466502,-0.00427686176175424,0.985009482952664));
#22536=DIRECTION('center_axis',(0.,1.,0.));
#22537=DIRECTION('ref_axis',(1.,0.,0.));
#22538=DIRECTION('',(0.,1.,0.));
#22539=DIRECTION('center_axis',(0.,1.,0.));
#22540=DIRECTION('ref_axis',(1.,0.,0.));
#22541=DIRECTION('',(0.,1.,0.));
#22542=DIRECTION('center_axis',(0.,1.,0.));
#22543=DIRECTION('ref_axis',(1.,0.,0.));
#22544=DIRECTION('',(0.,1.,0.));
#22545=DIRECTION('',(0.,0.,1.));
#22546=DIRECTION('',(-1.,0.,0.));
#22547=DIRECTION('',(0.,0.,-1.));
#22548=DIRECTION('',(1.,0.,0.));
#22549=DIRECTION('center_axis',(0.,1.,0.));
#22550=DIRECTION('ref_axis',(0.,0.,1.));
#22551=DIRECTION('',(-0.00142981099856909,0.882946690327321,0.46947108290132));
#22552=DIRECTION('',(-0.00150687409113358,0.883971486149799,0.467538384525367));
#22553=DIRECTION('',(0.0093100859730185,0.921219118259289,0.388932717128236));
#22554=DIRECTION('',(0.11564262543821,0.977075605521038,0.178745753173203));
#22555=DIRECTION('',(0.11564262543821,0.977075605521038,0.178745753173203));
#22556=DIRECTION('',(0.312891528512139,0.948359943232815,0.0520798373345121));
#22557=DIRECTION('',(0.312891528512139,0.948359943232815,0.0520798373345121));
#22558=DIRECTION('',(0.373785927406222,0.925420377862593,0.0622993154836071));
#22559=DIRECTION('',(0.335603981569758,0.93950240830941,0.0685944045483549));
#22560=DIRECTION('',(0.300592335144719,0.950101339342829,0.0833768135107546));
#22561=DIRECTION('',(0.388156973132249,0.911806820751478,0.133949564537902));
#22562=DIRECTION('',(0.301315367899131,0.918801423299879,0.25497645697187));
#22563=DIRECTION('',(0.301315367899131,0.918801423299879,0.25497645697187));
#22564=DIRECTION('',(0.212309885750666,0.93297911113271,0.29064495626547));
#22565=DIRECTION('',(0.212309885750666,0.93297911113271,0.29064495626547));
#22566=DIRECTION('',(0.270714584418356,0.934862032394266,0.229666266941533));
#22567=DIRECTION('',(0.270714584418356,0.934862032394266,0.229666266941533));
#22568=DIRECTION('',(0.374046850555081,0.917657512959969,0.134140383546302));
#22569=DIRECTION('',(0.418654959254244,0.897085298745081,0.141301068174572));
#22570=DIRECTION('',(0.000960745570679864,0.997274324740366,0.0737766777619821));
#22571=DIRECTION('',(0.0202807143037105,0.975301639137796,0.219944095902709));
#22572=DIRECTION('',(0.000960745570679864,0.997274324740366,0.0737766777619821));
#22573=DIRECTION('',(0.0689297223974915,0.919692597369279,0.386541355762038));
#22574=DIRECTION('',(0.00418796611478942,0.889609932076628,0.456701904627557));
#22575=DIRECTION('',(-0.000115678535487473,0.883083285401883,0.469216258949211));
#22576=DIRECTION('',(0.000654370202600861,0.882947403819665,0.469471462271938));
#22577=DIRECTION('',(0.000647998298494371,0.882947407483268,0.469471464219905));
#22578=DIRECTION('',(-0.000654370203064388,0.882947403819657,0.469471462271951));
#22579=DIRECTION('',(0.000115678535825108,0.883083285401884,0.46921625894921));
#22580=DIRECTION('',(-0.00418796611441199,0.889609932076588,0.456701904627638));
#22581=DIRECTION('',(-0.0689297223978216,0.919692597369242,0.386541355762066));
#22582=DIRECTION('',(-0.0202807143037967,0.975301639137796,0.219944095902698));
#22583=DIRECTION('',(-0.000960745570720953,0.997274324740367,0.0737766777619683));
#22584=DIRECTION('',(-0.000960745570720953,0.997274324740367,0.0737766777619683));
#22585=DIRECTION('',(6.32891971479231E-15,0.999877709626058,-0.0156385994560964));
#22586=DIRECTION('',(-0.374046850567848,0.917657512954638,0.134140383547171));
#22587=DIRECTION('',(-0.270714584414742,0.934862032395629,0.229666266940246));
#22588=DIRECTION('',(-0.270714584414742,0.934862032395629,0.229666266940246));
#22589=DIRECTION('',(-0.21230988575075,0.932979111132764,0.290644956265237));
#22590=DIRECTION('',(-0.21230988575075,0.932979111132764,0.290644956265237));
#22591=DIRECTION('',(-0.301315367899016,0.918801423299914,0.254976456971879));
#22592=DIRECTION('',(-0.301315367899016,0.918801423299914,0.254976456971879));
#22593=DIRECTION('',(-0.38815697313222,0.911806820751496,0.133949564537858));
#22594=DIRECTION('',(-0.300592335144713,0.950101339342829,0.0833768135107739));
#22595=DIRECTION('',(-0.335603981569753,0.939502408309412,0.0685944045483639));
#22596=DIRECTION('',(-0.373785927406274,0.925420377862572,0.0622993154836042));
#22597=DIRECTION('',(-0.312891528512024,0.948359943232853,0.0520798373345141));
#22598=DIRECTION('',(-0.312891528512024,0.948359943232853,0.0520798373345141));
#22599=DIRECTION('',(-0.11564262543822,0.977075605521036,0.178745753173204));
#22600=DIRECTION('',(-0.11564262543822,0.977075605521036,0.178745753173204));
#22601=DIRECTION('',(-0.00931008597314742,0.921219118259316,0.38893271712817));
#22602=DIRECTION('',(0.00150687409148693,0.883971486149805,0.467538384525354));
#22603=DIRECTION('',(0.00142981099892595,0.882946690327321,0.469471082901318));
#22604=DIRECTION('',(0.00131186599430631,0.882946833085555,0.469471158807229));
#22605=DIRECTION('',(-0.215703315134032,0.969009134257414,-0.120388444486531));
#22606=DIRECTION('',(0.000191764460211616,0.999797893622117,-0.0201031125741501));
#22607=DIRECTION('',(-0.215703315134032,0.969009134257414,-0.120388444486531));
#22608=DIRECTION('',(-0.000711770826806861,0.99999974667456,-5.75375725464803E-6));
#22609=DIRECTION('',(0.0013619134070984,0.999999072594712,-1.25999984792182E-6));
#22610=DIRECTION('',(-0.00216662813574643,0.999997652852845,-3.36493555673733E-6));
#22611=DIRECTION('',(-0.0752475458844889,0.997164884342654,1.65004120863823E-5));
#22612=DIRECTION('',(-0.103899479420175,0.994587803073991,-1.23558909609556E-5));
#22613=DIRECTION('',(-0.137985609280151,0.990434122609957,-0.0004694693063891));
#22614=DIRECTION('',(-0.140950090121527,0.990013822946304,0.00238798450134629));
#22615=DIRECTION('',(-0.113368116257768,0.993551950546169,-0.00148046684130703));
#22616=DIRECTION('',(-0.481426420109111,0.851820335359678,0.206472076292778));
#22617=DIRECTION('',(-0.418654959263383,0.897085298741647,0.1413010681693));
#22618=DIRECTION('',(0.481426420119192,0.851820335353988,0.206472076292748));
#22619=DIRECTION('',(0.113368116259197,0.993551950546006,-0.00148046684129751));
#22620=DIRECTION('',(0.140950090121739,0.990013822946273,0.00238798450135761));
#22621=DIRECTION('',(0.13798560927957,0.990434122610038,-0.000469469306391179));
#22622=DIRECTION('',(0.103899479420036,0.994587803074006,-1.23558909597681E-5));
#22623=DIRECTION('',(0.0752475458845945,0.997164884342646,1.65004120770553E-5));
#22624=DIRECTION('',(0.00216662813568782,0.999997652852845,-3.36493555644336E-6));
#22625=DIRECTION('',(-0.00136191340713365,0.999999072594712,-1.25999984490252E-6));
#22626=DIRECTION('',(0.000711770826834646,0.99999974667456,-5.7537572588639E-6));
#22627=DIRECTION('',(-0.000191764460208702,0.999797893622118,-0.0201031125741359));
#22628=DIRECTION('',(0.215703315134029,0.969009134257416,-0.120388444486517));
#22629=DIRECTION('',(0.215703315134029,0.969009134257416,-0.120388444486517));
#22630=DIRECTION('',(-2.65900267047622E-15,0.999951816801407,-0.00981652054273898));
#22631=DIRECTION('',(-0.000647998298984417,0.882947407483259,0.46947146421992));
#22632=DIRECTION('',(-0.00131186599394202,0.882946833085558,0.469471158807223));
#28195=CARTESIAN_POINT('',(0.,0.,0.));
#28196=CARTESIAN_POINT('Ctrl Pts',(38.2828091153483,1.11761889124797,-6.97607757441136));
#28197=CARTESIAN_POINT('Ctrl Pts',(37.8234650542136,1.10267068721089,-6.34100646753079));
#28198=CARTESIAN_POINT('Ctrl Pts',(37.4119152099722,1.08893748353005,-5.66458394800673));
#28199=CARTESIAN_POINT('Ctrl Pts',(36.1750430818529,1.05272528345341,-3.19923902056362));
#28200=CARTESIAN_POINT('Ctrl Pts',(35.6552816803935,1.04017275782615,-1.28742952530723));
#28201=CARTESIAN_POINT('Ctrl Pts',(35.4024624085441,1.03362032558888,2.58828262498384));
#28202=CARTESIAN_POINT('Ctrl Pts',(35.6533597239508,1.03853511081772,4.49488675691593));
#28203=CARTESIAN_POINT('Ctrl Pts',(36.9684333541811,1.07241301784844,8.4308675114562));
#28204=CARTESIAN_POINT('Ctrl Pts',(38.166980981151,1.10654958981212,10.3494011670926));
#28205=CARTESIAN_POINT('Ctrl Pts',(42.4575040433213,1.31384645443024,14.7529942978924));
#28206=CARTESIAN_POINT('Ctrl Pts',(49.7427089282406,1.83976032664608,17.7051751379966));
#28207=CARTESIAN_POINT('Ctrl Pts',(57.4412528288424,3.05949378929588,14.9345604704364));
#28208=CARTESIAN_POINT('Ctrl Pts',(60.2987018294292,3.48165017466642,12.2915412726567));
#28209=CARTESIAN_POINT('Ctrl Pts',(62.2074133981106,3.75719846747112,10.3606273747238));
#28210=CARTESIAN_POINT('Ctrl Pts',(63.3952259577481,3.96815686996487,8.42841971454959));
#28211=CARTESIAN_POINT('Ctrl Pts',(64.3744913950824,4.11561648662927,5.51345108116818));
#28212=CARTESIAN_POINT('Ctrl Pts',(64.8255995379143,4.15696630959856,3.66330292048651));
#28213=CARTESIAN_POINT('Ctrl Pts',(64.9117544346393,4.15341185643901,1.72453429192862));
#28214=CARTESIAN_POINT('Ctrl Pts',(64.8223415702672,4.18106939249892,0.39897045654781));
#28215=CARTESIAN_POINT('Ctrl Pts',(64.7753392842092,4.17529785000113,-0.106728049613198));
#28216=CARTESIAN_POINT('Ctrl Pts',(64.576120105023,4.10463228263791,-1.47947502913099));
#28217=CARTESIAN_POINT('Ctrl Pts',(64.1132581733554,3.92494468696414,-3.21690424520401));
#28218=CARTESIAN_POINT('Ctrl Pts',(63.4924556791943,3.96423510196274,-4.61414496951605));
#28219=CARTESIAN_POINT('Ctrl Pts',(62.8174909867282,4.12437261502235,-5.90593483351001));
#28220=CARTESIAN_POINT('Ctrl Pts',(62.1074018466296,4.41790060200681,-7.02319446864059));
#28221=CARTESIAN_POINT('Ctrl Pts',(60.874042949834,4.65644789261152,-8.48467747835397));
#28222=CARTESIAN_POINT('Ctrl Pts',(59.5348713215518,4.62838251566496,-9.75493905450226));
#28223=CARTESIAN_POINT('Ctrl Pts',(58.4404096210695,4.46707972840779,-10.538993216145));
#28224=CARTESIAN_POINT('Ctrl Pts',(57.7265849587516,4.3804810495509,-10.9717881911377));
#28225=CARTESIAN_POINT('Ctrl Pts',(57.427631809086,4.34556285696451,-11.1495376426103));
#28226=CARTESIAN_POINT('Ctrl Pts',(56.8142079310565,4.28689339090294,-11.4851678734925));
#28227=CARTESIAN_POINT('Ctrl Pts',(56.019812652493,4.23179766652216,-11.8577285498697));
#28228=CARTESIAN_POINT('Ctrl Pts',(55.0368711190457,4.16394895128873,-12.244451574114));
#28229=CARTESIAN_POINT('Ctrl Pts',(53.0324279581537,4.02139112324784,-12.8739714647708));
#28230=CARTESIAN_POINT('Ctrl Pts',(50.8522420828372,3.64495098639604,-13.1243776858381));
#28231=CARTESIAN_POINT('Ctrl Pts',(49.0742420084695,3.08805349273552,-13.0189954266342));
#28232=CARTESIAN_POINT('Ctrl Pts',(47.74311273162,2.65858895657289,-12.8839029021203));
#28233=CARTESIAN_POINT('Ctrl Pts',(46.0943092484674,2.06945988764268,-12.5441901629219));
#28234=CARTESIAN_POINT('Ctrl Pts',(43.9349361397835,1.53425192497824,-11.7148070258463));
#28235=CARTESIAN_POINT('Ctrl Pts',(42.7080397066157,1.37629460379916,-11.0306022357214));
#28236=CARTESIAN_POINT('Ctrl Pts',(41.8420335216443,1.28598589888282,-10.4618812091461));
#28237=CARTESIAN_POINT('Ctrl Pts',(41.2944047225801,1.23959147323119,-10.0745090823477));
#28238=CARTESIAN_POINT('Ctrl Pts',(39.9171313864447,1.1643772887167,-8.95351967626449));
#28239=CARTESIAN_POINT('Ctrl Pts',(38.9330416908621,1.13877908473415,-7.87506366436157));
#28240=CARTESIAN_POINT('Ctrl Pts',(38.2828091153483,1.11761889124797,-6.97607757441134));
#28241=CARTESIAN_POINT('Ctrl Pts',(38.2843482333976,0.970543869916695,-6.97820549874059));
#28242=CARTESIAN_POINT('Ctrl Pts',(37.824791924162,0.955556555693735,-6.34307994854715));
#28243=CARTESIAN_POINT('Ctrl Pts',(37.4129921013726,0.941740302951165,-5.66650842402892));
#28244=CARTESIAN_POINT('Ctrl Pts',(36.1752804401636,0.905197105915887,-3.20024374312772));
#28245=CARTESIAN_POINT('Ctrl Pts',(35.6553911302101,0.892454629920639,-1.28819029786402));
#28246=CARTESIAN_POINT('Ctrl Pts',(35.4023984837046,0.885821644900872,2.5885372043277));
#28247=CARTESIAN_POINT('Ctrl Pts',(35.6534560236685,0.890838387074693,4.4954292042868));
#28248=CARTESIAN_POINT('Ctrl Pts',(36.9690538044905,0.925251214315146,8.43257933875382));
#28249=CARTESIAN_POINT('Ctrl Pts',(38.1687976685799,0.959829053301754,10.3518678931255));
#28250=CARTESIAN_POINT('Ctrl Pts',(42.4632009249305,1.16789187702483,14.7578885142237));
#28251=CARTESIAN_POINT('Ctrl Pts',(49.7618317204618,1.6931399112023,17.7090114279978));
#28252=CARTESIAN_POINT('Ctrl Pts',(57.4610310499495,2.90441419567966,14.9231238711394));
#28253=CARTESIAN_POINT('Ctrl Pts',(60.3097400224713,3.32399961368451,12.2809040971181));
#28254=CARTESIAN_POINT('Ctrl Pts',(62.2158010395199,3.59788612667688,10.3487350385468));
#28255=CARTESIAN_POINT('Ctrl Pts',(63.4002833408593,3.80723506974322,8.41753794372203));
#28256=CARTESIAN_POINT('Ctrl Pts',(64.3756536499245,3.95482640879122,5.50797169852747));
#28257=CARTESIAN_POINT('Ctrl Pts',(64.8253779982732,3.99801213031397,3.66556685127137));
#28258=CARTESIAN_POINT('Ctrl Pts',(64.9117753274102,3.99589965313243,1.72084989994536));
#28259=CARTESIAN_POINT('Ctrl Pts',(64.8222143508002,4.02098591528982,0.397822582894523));
#28260=CARTESIAN_POINT('Ctrl Pts',(64.7759267056921,4.01433363661953,-0.100391348441605));
#28261=CARTESIAN_POINT('Ctrl Pts',(64.5786238367047,3.94076580473302,-1.46658139432066));
#28262=CARTESIAN_POINT('Ctrl Pts',(64.117831181995,3.75607887428162,-3.2065576872073));
#28263=CARTESIAN_POINT('Ctrl Pts',(63.4888906171941,3.78991406306379,-4.62291834378092));
#28264=CARTESIAN_POINT('Ctrl Pts',(62.802436085822,3.94505235147423,-5.93252337080619));
#28265=CARTESIAN_POINT('Ctrl Pts',(62.0853063832136,4.23159609271163,-7.05224389309994));
#28266=CARTESIAN_POINT('Ctrl Pts',(60.866372023969,4.46084159502816,-8.49116591110996));
#28267=CARTESIAN_POINT('Ctrl Pts',(59.5475053704118,4.43416211348493,-9.74333222473352));
#28268=CARTESIAN_POINT('Ctrl Pts',(58.4568923922613,4.27445806559024,-10.5279602375712));
#28269=CARTESIAN_POINT('Ctrl Pts',(57.7426864679962,4.18653414690636,-10.9621830331791));
#28270=CARTESIAN_POINT('Ctrl Pts',(57.4419997351774,4.14960693218127,-11.1414507351609));
#28271=CARTESIAN_POINT('Ctrl Pts',(56.8262448121692,4.08791202738523,-11.4791825193719));
#28272=CARTESIAN_POINT('Ctrl Pts',(56.0302740120864,4.02944743362823,-11.8531328935142));
#28273=CARTESIAN_POINT('Ctrl Pts',(55.0487268897378,3.95898137161517,-12.2403796446246));
#28274=CARTESIAN_POINT('Ctrl Pts',(53.0526650913507,3.81294159687107,-12.8684207467596));
#28275=CARTESIAN_POINT('Ctrl Pts',(50.8995528671741,3.44390300519801,-13.1207367571065));
#28276=CARTESIAN_POINT('Ctrl Pts',(49.1290190995407,2.90117687030285,-13.0231451906789));
#28277=CARTESIAN_POINT('Ctrl Pts',(47.7994031066733,2.4821543279567,-12.8933016449541));
#28278=CARTESIAN_POINT('Ctrl Pts',(46.1394375535869,1.90575400846461,-12.5586946873949));
#28279=CARTESIAN_POINT('Ctrl Pts',(43.9556751935569,1.38157721032517,-11.7254914115979));
#28280=CARTESIAN_POINT('Ctrl Pts',(42.7203926546672,1.22604125597042,-11.0380186679154));
#28281=CARTESIAN_POINT('Ctrl Pts',(41.8510060573403,1.13609818750472,-10.4681041752686));
#28282=CARTESIAN_POINT('Ctrl Pts',(41.300244194319,1.09125622040995,-10.0790642159954));
#28283=CARTESIAN_POINT('Ctrl Pts',(39.9191713337688,1.01731653755015,-8.95575210737738));
#28284=CARTESIAN_POINT('Ctrl Pts',(38.9348812604486,0.991759426515284,-7.87726865688117));
#28285=CARTESIAN_POINT('Ctrl Pts',(38.2843482333976,0.970543869916693,-6.97820549874057));
#28286=CARTESIAN_POINT('Ctrl Pts',(38.2338763919957,0.676840453798634,-7.02118403389358));
#28287=CARTESIAN_POINT('Ctrl Pts',(37.7717920326072,0.661775302774764,-6.38309719311575));
#28288=CARTESIAN_POINT('Ctrl Pts',(37.3575860906707,0.647794127754478,-5.70323225274495));
#28289=CARTESIAN_POINT('Ctrl Pts',(36.1123525330349,0.610593091434165,-3.22412755712282));
#28290=CARTESIAN_POINT('Ctrl Pts',(35.5896785478952,0.597473572198639,-1.30297380755022));
#28291=CARTESIAN_POINT('Ctrl Pts',(35.3351252218906,0.590680455223746,2.59338985996385));
#28292=CARTESIAN_POINT('Ctrl Pts',(35.5877124163472,0.59589966460025,4.50953805245734));
#28293=CARTESIAN_POINT('Ctrl Pts',(36.9108449328443,0.631375350576928,8.46662689486421));
#28294=CARTESIAN_POINT('Ctrl Pts',(38.1185183684278,0.666829439106687,10.3959359859494));
#28295=CARTESIAN_POINT('Ctrl Pts',(42.4406442978422,0.876416661809782,14.8257561155249));
#28296=CARTESIAN_POINT('Ctrl Pts',(49.7958477126675,1.40034557220048,17.7894082437089));
#28297=CARTESIAN_POINT('Ctrl Pts',(57.5366834538322,2.59483636795635,14.9687982987776));
#28298=CARTESIAN_POINT('Ctrl Pts',(60.3846991062462,3.00931729041542,12.3153796590069));
#28299=CARTESIAN_POINT('Ctrl Pts',(62.2964901059904,3.2799066287722,10.3717454931349));
#28300=CARTESIAN_POINT('Ctrl Pts',(63.4820778102999,3.48606190817418,8.43271076666013));
#28301=CARTESIAN_POINT('Ctrl Pts',(64.4545411897986,3.63390851895106,5.51796931146853));
#28302=CARTESIAN_POINT('Ctrl Pts',(64.9020137172839,3.68073403490991,3.6805130487955));
#28303=CARTESIAN_POINT('Ctrl Pts',(64.9879632943044,3.68148987723326,1.71407508637896));
#28304=CARTESIAN_POINT('Ctrl Pts',(64.9001507314642,3.70147455415994,0.388961732509691));
#28305=CARTESIAN_POINT('Ctrl Pts',(64.8559236706679,3.69307183338057,-0.0971210585065526));
#28306=CARTESIAN_POINT('Ctrl Pts',(64.6648905108266,3.61376880717593,-1.45821181459786));
#28307=CARTESIAN_POINT('Ctrl Pts',(64.2100297152053,3.41916239249666,-3.21445917834352));
#28308=CARTESIAN_POINT('Ctrl Pts',(63.5663200101209,3.44220843949932,-4.67995598826193));
#28309=CARTESIAN_POINT('Ctrl Pts',(62.8598470037644,3.5875286692031,-6.03733781860483));
#28310=CARTESIAN_POINT('Ctrl Pts',(62.1313319346664,3.8603129866682,-7.17486204206737));
#28311=CARTESIAN_POINT('Ctrl Pts',(60.9366508193253,4.07112216165055,-8.58492853258466));
#28312=CARTESIAN_POINT('Ctrl Pts',(59.6468918463728,4.04720779460478,-9.81081719124648));
#28313=CARTESIAN_POINT('Ctrl Pts',(58.554757623092,3.89068939024514,-10.6017315018052));
#28314=CARTESIAN_POINT('Ctrl Pts',(57.8348859259373,3.80015936073672,-11.043412961638));
#28315=CARTESIAN_POINT('Ctrl Pts',(57.5294671083027,3.75925621283239,-11.22905794043));
#28316=CARTESIAN_POINT('Ctrl Pts',(56.9057049465525,3.69159213430375,-11.5768172191285));
#28317=CARTESIAN_POINT('Ctrl Pts',(56.1015735095258,3.62649446962661,-11.9604026832035));
#28318=CARTESIAN_POINT('Ctrl Pts',(55.1154738556396,3.55087990661318,-12.355403877143));
#28319=CARTESIAN_POINT('Ctrl Pts',(53.1194939160782,3.39800079265719,-12.9908439077088));
#28320=CARTESIAN_POINT('Ctrl Pts',(50.9985372139996,3.04359005396801,-13.2449422202065));
#28321=CARTESIAN_POINT('Ctrl Pts',(49.2292301319419,2.52884635192557,-13.1480799473144));
#28322=CARTESIAN_POINT('Ctrl Pts',(47.8934345339389,2.13048353986497,-13.0161964109135));
#28323=CARTESIAN_POINT('Ctrl Pts',(46.2037204788327,1.57914981460136,-12.672375554347));
#28324=CARTESIAN_POINT('Ctrl Pts',(43.9658914820892,1.07677302966014,-11.8125313821532));
#28325=CARTESIAN_POINT('Ctrl Pts',(42.7096093696835,0.926038355842821,-11.1128523513539));
#28326=CARTESIAN_POINT('Ctrl Pts',(41.8297177896006,0.836813474807447,-10.5373478547873));
#28327=CARTESIAN_POINT('Ctrl Pts',(41.2711074075715,0.795053392302155,-10.1418327999497));
#28328=CARTESIAN_POINT('Ctrl Pts',(39.8770164559302,0.723645794097905,-9.00776748871939));
#28329=CARTESIAN_POINT('Ctrl Pts',(38.8879880449638,0.698166193651579,-7.92443909907391));
#28330=CARTESIAN_POINT('Ctrl Pts',(38.2338763919957,0.676840453798629,-7.02118403389356));
#28331=CARTESIAN_POINT('Ctrl Pts',(37.9755726500682,0.260078906144198,-7.21719833326774));
#28332=CARTESIAN_POINT('Ctrl Pts',(37.5026155044898,0.244950287093724,-6.56501278076528));
#28333=CARTESIAN_POINT('Ctrl Pts',(37.0783378702849,0.230836545601503,-5.86997432036658));
#28334=CARTESIAN_POINT('Ctrl Pts',(35.8021634986244,0.19311352273868,-3.33429548649416));
#28335=CARTESIAN_POINT('Ctrl Pts',(35.2667422286841,0.17970731942181,-1.37011705125621));
#28336=CARTESIAN_POINT('Ctrl Pts',(35.0057829672195,0.172789861916432,2.61538435750336));
#28337=CARTESIAN_POINT('Ctrl Pts',(35.2647213031546,0.178164003071174,4.57492439960631));
#28338=CARTESIAN_POINT('Ctrl Pts',(36.6209929910503,0.214460834622622,8.62171290521318));
#28339=CARTESIAN_POINT('Ctrl Pts',(37.8591948792036,0.250608489038568,10.5949420714734));
#28340=CARTESIAN_POINT('Ctrl Pts',(42.2901085418755,0.461561258183715,15.125001674628));
#28341=CARTESIAN_POINT('Ctrl Pts',(49.8305121070811,0.985076187029921,18.1566364375623));
#28342=CARTESIAN_POINT('Ctrl Pts',(57.7671470310111,2.16867740413173,15.2701980250863));
#28343=CARTESIAN_POINT('Ctrl Pts',(60.6718156147976,2.57897979706842,12.5568347354958));
#28344=CARTESIAN_POINT('Ctrl Pts',(62.6293284960575,2.84736891467804,10.566014989906));
#28345=CARTESIAN_POINT('Ctrl Pts',(63.8429017716634,3.05132886188749,8.58195565622854));
#28346=CARTESIAN_POINT('Ctrl Pts',(64.8285820743521,3.19878966350941,5.60448525990243));
#28347=CARTESIAN_POINT('Ctrl Pts',(65.275485562142,3.24760181738135,3.73737513244731));
#28348=CARTESIAN_POINT('Ctrl Pts',(65.3581463113578,3.25021437519247,1.7067892570071));
#28349=CARTESIAN_POINT('Ctrl Pts',(65.278918050488,3.26706734456811,0.353980649115699));
#28350=CARTESIAN_POINT('Ctrl Pts',(65.2393269706764,3.25764677656883,-0.125349094041277));
#28351=CARTESIAN_POINT('Ctrl Pts',(65.0640319535867,3.17608139024397,-1.5076834973838));
#28352=CARTESIAN_POINT('Ctrl Pts',(64.6212457938457,2.97538186506718,-3.3249923897941));
#28353=CARTESIAN_POINT('Ctrl Pts',(63.9611889154096,2.99381204921896,-4.89182750593231));
#28354=CARTESIAN_POINT('Ctrl Pts',(63.2368536880495,3.14024319198427,-6.35014365680316));
#28355=CARTESIAN_POINT('Ctrl Pts',(62.50227653091,3.41141589189322,-7.54919924147722));
#28356=CARTESIAN_POINT('Ctrl Pts',(61.3187069374386,3.61275670087874,-8.97794668849745));
#28357=CARTESIAN_POINT('Ctrl Pts',(60.0237974951738,3.59088824799297,-10.2076024056545));
#28358=CARTESIAN_POINT('Ctrl Pts',(58.8982776603944,3.43605957167923,-11.0244640574304));
#28359=CARTESIAN_POINT('Ctrl Pts',(58.1538979147083,3.34499063864486,-11.4908234586531));
#28360=CARTESIAN_POINT('Ctrl Pts',(57.8375768250259,3.30338878993206,-11.6947038585483));
#28361=CARTESIAN_POINT('Ctrl Pts',(57.191461854579,3.23515093659049,-12.0730719345562));
#28362=CARTESIAN_POINT('Ctrl Pts',(56.3590794249149,3.17002756060386,-12.4899209447339));
#28363=CARTESIAN_POINT('Ctrl Pts',(55.3412124627408,3.09523089727471,-12.9153793174091));
#28364=CARTESIAN_POINT('Ctrl Pts',(53.2858637202805,2.94410587092508,-13.5928076231749));
#28365=CARTESIAN_POINT('Ctrl Pts',(51.1252252958554,2.59665348818909,-13.8437949847423));
#28366=CARTESIAN_POINT('Ctrl Pts',(49.3161008082114,2.09001896696724,-13.7034803700494));
#28367=CARTESIAN_POINT('Ctrl Pts',(47.9461640300902,1.69674609843365,-13.5322820821945));
#28368=CARTESIAN_POINT('Ctrl Pts',(46.2002895057426,1.14928126906623,-13.1183870449433));
#28369=CARTESIAN_POINT('Ctrl Pts',(43.8718153675593,0.653583390728654,-12.1628380118467));
#28370=CARTESIAN_POINT('Ctrl Pts',(42.57085577801,0.505460781225472,-11.4270867861695));
#28371=CARTESIAN_POINT('Ctrl Pts',(41.6631348373488,0.416355188800432,-10.8327479115071));
#28372=CARTESIAN_POINT('Ctrl Pts',(41.0877064851766,0.376568431697981,-10.41767437804));
#28373=CARTESIAN_POINT('Ctrl Pts',(39.6561155818029,0.306894436867863,-9.24753265543428));
#28374=CARTESIAN_POINT('Ctrl Pts',(38.6450754670143,0.281494489279973,-8.1404110781305));
#28375=CARTESIAN_POINT('Ctrl Pts',(37.9755726500682,0.260078906144189,-7.21719833326772));
#28376=CARTESIAN_POINT('Ctrl Pts',(37.6827349553876,0.123820476106236,-7.43200930537173));
#28377=CARTESIAN_POINT('Ctrl Pts',(37.1981115312996,0.108758167919931,-6.76415338866424));
#28378=CARTESIAN_POINT('Ctrl Pts',(36.7631614809068,0.0947959133819992,
-6.0524004348351));
#28379=CARTESIAN_POINT('Ctrl Pts',(35.4544728346314,0.0576802462121595,
-3.45532498536105));
#28380=CARTESIAN_POINT('Ctrl Pts',(34.9052399965703,0.0446571520855538,
-1.44349856127014));
#28381=CARTESIAN_POINT('Ctrl Pts',(34.6375668077913,0.0378911336842094,
2.6394105962902));
#28382=CARTESIAN_POINT('Ctrl Pts',(34.9031853275286,0.0430667657461748,
4.64681425938547));
#28383=CARTESIAN_POINT('Ctrl Pts',(36.2948564127528,0.0783236368819047,
8.79157409478439));
#28384=CARTESIAN_POINT('Ctrl Pts',(37.5644599252781,0.113661228931385,10.8124043557161));
#28385=CARTESIAN_POINT('Ctrl Pts',(42.1078998944315,0.323523601766359,15.4501968176738));
#28386=CARTESIAN_POINT('Ctrl Pts',(49.8287231859174,0.849796931774696,18.5588719405612));
#28387=CARTESIAN_POINT('Ctrl Pts',(57.9754329065988,2.0540989824616,15.6254681029825));
#28388=CARTESIAN_POINT('Ctrl Pts',(60.9594784171162,2.46870777859652,12.8441351803459));
#28389=CARTESIAN_POINT('Ctrl Pts',(62.971560441687,2.74096720090711,10.8037036380583));
#28390=CARTESIAN_POINT('Ctrl Pts',(64.2214654517206,2.9484923882698,8.76815175703241));
#28391=CARTESIAN_POINT('Ctrl Pts',(65.2308459020326,3.09443853654356,5.7106058750305));
#28392=CARTESIAN_POINT('Ctrl Pts',(65.6823520855425,3.13806676670926,3.79439575576531));
#28393=CARTESIAN_POINT('Ctrl Pts',(65.762315057619,3.13733886966709,1.70709534462677));
#28394=CARTESIAN_POINT('Ctrl Pts',(65.6900530491722,3.16070120932451,0.318603327590335));
#28395=CARTESIAN_POINT('Ctrl Pts',(65.6529204214975,3.15356930340056,-0.170262844993036));
#28396=CARTESIAN_POINT('Ctrl Pts',(65.4862706901961,3.08217960117338,-1.59024642585578));
#28397=CARTESIAN_POINT('Ctrl Pts',(65.0461514716187,2.89386831665398,-3.46667020680638));
#28398=CARTESIAN_POINT('Ctrl Pts',(64.3809104358716,2.92998396789142,-5.09288798615411));
#28399=CARTESIAN_POINT('Ctrl Pts',(63.6556566613573,3.10360208747441,-6.60774501667949));
#28400=CARTESIAN_POINT('Ctrl Pts',(62.9225440804532,3.40530745932964,-7.85255781394852));
#28401=CARTESIAN_POINT('Ctrl Pts',(61.7086950342478,3.63132384902911,-9.34491776509278));
#28402=CARTESIAN_POINT('Ctrl Pts',(60.3613536516037,3.60718414391209,-10.6218630745699));
#28403=CARTESIAN_POINT('Ctrl Pts',(59.1952457990793,3.44841050071065,-11.4638466082202));
#28404=CARTESIAN_POINT('Ctrl Pts',(58.4263692487142,3.36258353011487,-11.9491687552984));
#28405=CARTESIAN_POINT('Ctrl Pts',(58.101489891242,3.32884046917442,-12.164519725722));
#28406=CARTESIAN_POINT('Ctrl Pts',(57.4362450214768,3.27343367240952,-12.5627748724467));
#28407=CARTESIAN_POINT('Ctrl Pts',(56.5774664878876,3.223674244555,-13.0020133628729));
#28408=CARTESIAN_POINT('Ctrl Pts',(55.5238152782093,3.16231592704423,-13.4494879741627));
#28409=CARTESIAN_POINT('Ctrl Pts',(53.3899462310028,3.029985365176,-14.1614509406894));
#28410=CARTESIAN_POINT('Ctrl Pts',(51.1305329459546,2.66262149151837,-14.4130141023804));
#28411=CARTESIAN_POINT('Ctrl Pts',(49.2708165592316,2.10607072348422,-14.2349085336049));
#28412=CARTESIAN_POINT('Ctrl Pts',(47.8677938844659,1.67422453698365,-14.0303104653549));
#28413=CARTESIAN_POINT('Ctrl Pts',(46.0951831056431,1.0718027650261,-13.5585223739087));
#28414=CARTESIAN_POINT('Ctrl Pts',(43.7219341720429,0.532922359928608,-12.5251822886396));
#28415=CARTESIAN_POINT('Ctrl Pts',(42.388913557605,0.377751766345516,-11.7591450726125));
#28416=CARTESIAN_POINT('Ctrl Pts',(41.457679963294,0.286900595795112,-11.1471711579781));
#28417=CARTESIAN_POINT('Ctrl Pts',(40.8697916597159,0.243253833273792,-10.7154469863502));
#28418=CARTESIAN_POINT('Ctrl Pts',(39.4040717113082,0.170652973788299,-9.51115933805032));
#28419=CARTESIAN_POINT('Ctrl Pts',(38.3687521783392,0.145142191730392,-8.37740451026479));
#28420=CARTESIAN_POINT('Ctrl Pts',(37.6827349553875,0.123820476106226,-7.43200930537172));
#28421=CARTESIAN_POINT('Ctrl Pts',(37.5039656670749,0.118112959038132,-7.56143810282447));
#28422=CARTESIAN_POINT('Ctrl Pts',(37.0123775719425,0.10313359302091,-6.88405610335296));
#28423=CARTESIAN_POINT('Ctrl Pts',(36.5711306628854,0.0893498876773675,
-6.16220244562775));
#28424=CARTESIAN_POINT('Ctrl Pts',(35.2433527822817,0.0529585045549561,
-3.52820338776542));
#28425=CARTESIAN_POINT('Ctrl Pts',(34.6859738142494,0.0403720985573172,
-1.48759930416187));
#28426=CARTESIAN_POINT('Ctrl Pts',(34.4143703467061,0.0337848714443707,
2.65385351185261));
#28427=CARTESIAN_POINT('Ctrl Pts',(34.6839009903238,0.0387342423626621,
4.69008938372649));
#28428=CARTESIAN_POINT('Ctrl Pts',(36.0963099966431,0.0727670904719236,
8.89387566280885));
#28429=CARTESIAN_POINT('Ctrl Pts',(37.3842658146977,0.107170593364541,10.9433341336584));
#28430=CARTESIAN_POINT('Ctrl Pts',(41.9934716582436,0.315543736904061,15.6460641572062));
#28431=CARTESIAN_POINT('Ctrl Pts',(49.8196297154773,0.84468878067967,18.8009942746542));
#28432=CARTESIAN_POINT('Ctrl Pts',(58.0877581529129,2.07108377161561,15.8397172942412));
#28433=CARTESIAN_POINT('Ctrl Pts',(61.1210009956106,2.49061701093176,13.0173740492313));
#28434=CARTESIAN_POINT('Ctrl Pts',(63.1652907725653,2.76697733959494,10.9477133500425));
#28435=CARTESIAN_POINT('Ctrl Pts',(64.4366398118809,2.97827221081983,8.88139359080468));
#28436=CARTESIAN_POINT('Ctrl Pts',(65.4622821937629,3.12300989375844,5.77488389114306));
#28437=CARTESIAN_POINT('Ctrl Pts',(65.9190548938414,3.16143432460456,3.82648857040399));
#28438=CARTESIAN_POINT('Ctrl Pts',(65.998639811114,3.15704672469335,1.70925454566402));
#28439=CARTESIAN_POINT('Ctrl Pts',(65.928095335385,3.18715779039101,0.298800350813972));
#28440=CARTESIAN_POINT('Ctrl Pts',(65.891116073978,3.18243009548258,-0.199734967314633));
#28441=CARTESIAN_POINT('Ctrl Pts',(65.724890489484,3.12052200322572,-1.64464387487764));
#28442=CARTESIAN_POINT('Ctrl Pts',(65.2803917641197,2.94481678182075,-3.55221350711536));
#28443=CARTESIAN_POINT('Ctrl Pts',(64.6112886712169,2.99710209211733,-5.19738775518303));
#28444=CARTESIAN_POINT('Ctrl Pts',(63.8845078135012,3.19262492584513,-6.72720317525355));
#28445=CARTESIAN_POINT('Ctrl Pts',(63.1478922725819,3.51893245868478,-7.98720386840469));
#28446=CARTESIAN_POINT('Ctrl Pts',(61.9033465036304,3.76669114727106,-9.51925813077716));
#28447=CARTESIAN_POINT('Ctrl Pts',(60.5179602038555,3.74004538058918,-10.8316209977219));
#28448=CARTESIAN_POINT('Ctrl Pts',(59.3303434129858,3.57752994005544,-11.6868660023985));
#28449=CARTESIAN_POINT('Ctrl Pts',(58.5488026525572,3.49573255165253,-12.1790390892533));
#28450=CARTESIAN_POINT('Ctrl Pts',(58.2193592315412,3.46833531514964,-12.3964860812939));
#28451=CARTESIAN_POINT('Ctrl Pts',(57.5441918319574,3.42281957210131,-12.7988621720065));
#28452=CARTESIAN_POINT('Ctrl Pts',(56.6717264715229,3.38439221421136,-13.2427196483312));
#28453=CARTESIAN_POINT('Ctrl Pts',(55.5988183637806,3.33268751766902,-13.6954762514658));
#28454=CARTESIAN_POINT('Ctrl Pts',(53.4217095394243,3.21319086988362,-14.4173723958613));
#28455=CARTESIAN_POINT('Ctrl Pts',(51.1016444796743,2.83048256335952,-14.6743846054424));
#28456=CARTESIAN_POINT('Ctrl Pts',(49.2134657180401,2.23435274398341,-14.4914393185008));
#28457=CARTESIAN_POINT('Ctrl Pts',(47.793446484243,1.77072158723543,-14.281705766681));
#28458=CARTESIAN_POINT('Ctrl Pts',(46.0121640592379,1.12290576810707,-13.7965877390655));
#28459=CARTESIAN_POINT('Ctrl Pts',(43.6223924642014,0.543466278467186,-12.7346019515179));
#28460=CARTESIAN_POINT('Ctrl Pts',(42.2733193663373,0.381005068405684,-11.9542639561288));
#28461=CARTESIAN_POINT('Ctrl Pts',(41.3294951498055,0.288584763006973,-11.332814913621));
#28462=CARTESIAN_POINT('Ctrl Pts',(40.734984113935,0.240755869996147,-10.8931568499415));
#28463=CARTESIAN_POINT('Ctrl Pts',(39.2498617813692,0.164868595658534,-9.67023765817002));
#28464=CARTESIAN_POINT('Ctrl Pts',(38.1998418527826,0.139317264414103,-8.52031812194351));
#28465=CARTESIAN_POINT('Ctrl Pts',(37.5039656670749,0.118112959038122,-7.56143810282446));
#28466=CARTESIAN_POINT('',(37.5042795392924,0.11812305820763,-7.56121085790808));
#28467=CARTESIAN_POINT('',(38.2828091153483,1.11761889124797,-6.97607757441136));
#28468=CARTESIAN_POINT('Ctrl Pts',(37.5042795392924,0.118123058207631,-7.56121085790808));
#28469=CARTESIAN_POINT('Ctrl Pts',(37.6829406508519,0.123916213079733,-7.43185841697136));
#28470=CARTESIAN_POINT('Ctrl Pts',(37.9756374600947,0.26018347422652,-7.21714915205247));
#28471=CARTESIAN_POINT('Ctrl Pts',(38.2338763919957,0.676840453798634,-7.02118403389358));
#28472=CARTESIAN_POINT('Ctrl Pts',(38.2843482333976,0.970543869916695,-6.97820549874059));
#28473=CARTESIAN_POINT('Ctrl Pts',(38.2828091153483,1.11761889124797,-6.97607757441136));
#28474=CARTESIAN_POINT('',(35.495997940798,1.03592643542494,1.63217755032596));
#28475=CARTESIAN_POINT('Ctrl Pts',(38.2828091153483,1.11761889124797,-6.97607757441136));
#28476=CARTESIAN_POINT('Ctrl Pts',(37.8234650542136,1.10267068721089,-6.34100646753079));
#28477=CARTESIAN_POINT('Ctrl Pts',(37.4119152099722,1.08893748353005,-5.66458394800673));
#28478=CARTESIAN_POINT('Ctrl Pts',(36.1750430818529,1.05272528345341,-3.19923902056362));
#28479=CARTESIAN_POINT('Ctrl Pts',(35.6552816803935,1.04017275782615,-1.28742952530723));
#28480=CARTESIAN_POINT('Ctrl Pts',(35.5063406075951,1.03631258419414,0.995832827675688));
#28481=CARTESIAN_POINT('Ctrl Pts',(35.495996386627,1.03600036720019,1.31426374489689));
#28482=CARTESIAN_POINT('Ctrl Pts',(35.495997940798,1.03592643542494,1.63217755032596));
#28483=CARTESIAN_POINT('Ctrl Pts',(35.495997940798,1.03592643542494,1.63217755032596));
#28484=CARTESIAN_POINT('Ctrl Pts',(35.4960057101111,1.03555684987327,3.22143127459461));
#28485=CARTESIAN_POINT('Ctrl Pts',(35.7545552599904,1.04114203174067,4.79776233220028));
#28486=CARTESIAN_POINT('Ctrl Pts',(36.9684333541811,1.07241301784844,8.4308675114562));
#28487=CARTESIAN_POINT('Ctrl Pts',(38.166980981151,1.10654958981212,10.3494011670926));
#28488=CARTESIAN_POINT('Ctrl Pts',(42.4575040433213,1.31384645443024,14.7529942978924));
#28489=CARTESIAN_POINT('Ctrl Pts',(49.7427089282406,1.83976032664608,17.7051751379966));
#28490=CARTESIAN_POINT('Ctrl Pts',(57.4412528288424,3.05949378929588,14.9345604704364));
#28491=CARTESIAN_POINT('Ctrl Pts',(60.2987018294292,3.48165017466642,12.2915412726567));
#28492=CARTESIAN_POINT('Ctrl Pts',(62.2074133981106,3.75719846747112,10.3606273747238));
#28493=CARTESIAN_POINT('Ctrl Pts',(63.3952259577481,3.96815686996487,8.42841971454959));
#28494=CARTESIAN_POINT('Ctrl Pts',(64.3744913950824,4.11561648662927,5.51345108116818));
#28495=CARTESIAN_POINT('Ctrl Pts',(64.8255995379143,4.15696630959856,3.66330292048651));
#28496=CARTESIAN_POINT('Ctrl Pts',(64.9117544346393,4.15341185643901,1.72453429192862));
#28497=CARTESIAN_POINT('Ctrl Pts',(64.8223415702672,4.18106939249892,0.39897045654781));
#28498=CARTESIAN_POINT('Ctrl Pts',(64.7753392842092,4.17529785000113,-0.106728049613198));
#28499=CARTESIAN_POINT('Ctrl Pts',(64.576120105023,4.10463228263791,-1.47947502913099));
#28500=CARTESIAN_POINT('Ctrl Pts',(64.1132581733554,3.92494468696414,-3.21690424520401));
#28501=CARTESIAN_POINT('Ctrl Pts',(63.4924556791943,3.96423510196274,-4.61414496951605));
#28502=CARTESIAN_POINT('Ctrl Pts',(62.8174909867282,4.12437261502235,-5.90593483351001));
#28503=CARTESIAN_POINT('Ctrl Pts',(62.1074018466296,4.41790060200681,-7.02319446864059));
#28504=CARTESIAN_POINT('Ctrl Pts',(60.874042949834,4.65644789261152,-8.48467747835397));
#28505=CARTESIAN_POINT('Ctrl Pts',(59.5348713215518,4.62838251566496,-9.75493905450226));
#28506=CARTESIAN_POINT('Ctrl Pts',(58.4404096210695,4.46707972840779,-10.538993216145));
#28507=CARTESIAN_POINT('Ctrl Pts',(57.7265849587516,4.3804810495509,-10.9717881911377));
#28508=CARTESIAN_POINT('Ctrl Pts',(57.427631809086,4.34556285696451,-11.1495376426103));
#28509=CARTESIAN_POINT('Ctrl Pts',(56.8142079310565,4.28689339090294,-11.4851678734925));
#28510=CARTESIAN_POINT('Ctrl Pts',(56.019812652493,4.23179766652216,-11.8577285498697));
#28511=CARTESIAN_POINT('Ctrl Pts',(55.0368711190457,4.16394895128873,-12.244451574114));
#28512=CARTESIAN_POINT('Ctrl Pts',(53.0324279581537,4.02139112324784,-12.8739714647708));
#28513=CARTESIAN_POINT('Ctrl Pts',(50.8522420828372,3.64495098639604,-13.1243776858381));
#28514=CARTESIAN_POINT('Ctrl Pts',(49.0742420084695,3.08805349273552,-13.0189954266342));
#28515=CARTESIAN_POINT('Ctrl Pts',(47.74311273162,2.65858895657289,-12.8839029021203));
#28516=CARTESIAN_POINT('Ctrl Pts',(46.0943092484674,2.06945988764268,-12.5441901629219));
#28517=CARTESIAN_POINT('Ctrl Pts',(43.9349361397835,1.53425192497824,-11.7148070258463));
#28518=CARTESIAN_POINT('Ctrl Pts',(42.7080397066157,1.37629460379916,-11.0306022357214));
#28519=CARTESIAN_POINT('Ctrl Pts',(41.8420335216443,1.28598589888282,-10.4618812091461));
#28520=CARTESIAN_POINT('Ctrl Pts',(41.2944047225801,1.23959147323119,-10.0745090823477));
#28521=CARTESIAN_POINT('Ctrl Pts',(39.9171313864447,1.1643772887167,-8.95351967626449));
#28522=CARTESIAN_POINT('Ctrl Pts',(38.9330416908621,1.13877908473415,-7.87506366436157));
#28523=CARTESIAN_POINT('Ctrl Pts',(38.2828091153483,1.11761889124797,-6.97607757441134));
#28524=CARTESIAN_POINT('',(41.6354952640144,0.318620154457148,-11.5338206587945));
#28525=CARTESIAN_POINT('Ctrl Pts',(37.5042795392924,0.118123058207621,-7.56121085790808));
#28526=CARTESIAN_POINT('Ctrl Pts',(38.2001384150095,0.139327569664645,-8.52006720115489));
#28527=CARTESIAN_POINT('Ctrl Pts',(39.2501325334149,0.164878829687915,-9.66995835627672));
#28528=CARTESIAN_POINT('Ctrl Pts',(40.7352207990105,0.240760335453449,-10.8928448336842));
#28529=CARTESIAN_POINT('Ctrl Pts',(41.3297202060976,0.28858188757864,-11.3324889652665));
#28530=CARTESIAN_POINT('Ctrl Pts',(41.6342353020102,0.318400150449319,-11.5329923830209));
#28531=CARTESIAN_POINT('',(58.6306321623861,3.50423391942768,-12.126881567578));
#28532=CARTESIAN_POINT('Ctrl Pts',(41.6354952640144,0.318620154457148,-11.5338206587945));
#28533=CARTESIAN_POINT('Ctrl Pts',(41.6362878084932,0.318697950647469,-11.5343425540537));
#28534=CARTESIAN_POINT('Ctrl Pts',(41.6370804004481,0.318775798580112,-11.5348645371535));
#28535=CARTESIAN_POINT('Ctrl Pts',(41.6378730398733,0.318853698316649,-11.535386607734));
#28536=CARTESIAN_POINT('Ctrl Pts',(41.6805430916827,0.323047264379738,-11.5634911632345));
#28537=CARTESIAN_POINT('Ctrl Pts',(41.7233594774993,0.327272758560646,-11.5905980399423));
#28538=CARTESIAN_POINT('Ctrl Pts',(41.7663216672521,0.331560773468719,-11.617196229109));
#28539=CARTESIAN_POINT('Ctrl Pts',(41.8237490958923,0.33729254998102,-11.6527499478352));
#28540=CARTESIAN_POINT('Ctrl Pts',(41.8814372382824,0.343135341510576,-11.6873965783807));
#28541=CARTESIAN_POINT('Ctrl Pts',(41.9393805747972,0.349184541000843,-11.7224062258384));
#28542=CARTESIAN_POINT('Ctrl Pts',(41.9484915860832,0.350135717238561,-11.7279111434405));
#28543=CARTESIAN_POINT('Ctrl Pts',(41.9576088967413,0.351092041842586,-11.7334251279012));
#28544=CARTESIAN_POINT('Ctrl Pts',(41.966732473864,0.352053933362217,-11.7389531680816));
#28545=CARTESIAN_POINT('Ctrl Pts',(42.0678457344272,0.36271422444658,-11.800218410832));
#28546=CARTESIAN_POINT('Ctrl Pts',(42.1697316625997,0.374060704226699,-11.8632120074282));
#28547=CARTESIAN_POINT('Ctrl Pts',(42.2723599254288,0.386135829849839,-11.9261906774715));
#28548=CARTESIAN_POINT('Ctrl Pts',(42.2821197317413,0.387284157649918,-11.9321798621707));
#28549=CARTESIAN_POINT('Ctrl Pts',(42.2918862233456,0.388439054026203,-11.9381689411694));
#28550=CARTESIAN_POINT('Ctrl Pts',(42.3016593559583,0.389600542077846,-11.9441564539643));
#28551=CARTESIAN_POINT('Ctrl Pts',(42.3936906818806,0.400538006007943,-12.0005394749798));
#28552=CARTESIAN_POINT('Ctrl Pts',(42.4863130122695,0.412061738656644,-12.0567865043064));
#28553=CARTESIAN_POINT('Ctrl Pts',(42.5794710623517,0.424232517306317,-12.1124724443935));
#28554=CARTESIAN_POINT('Ctrl Pts',(42.616739429467,0.429101501214791,-12.1347498971364));
#28555=CARTESIAN_POINT('Ctrl Pts',(42.6540932478344,0.434073788916218,-12.1569371588301));
#28556=CARTESIAN_POINT('Ctrl Pts',(42.6915278434756,0.439152057304701,-12.1790052390936));
#28557=CARTESIAN_POINT('Ctrl Pts',(42.7750031529593,0.450476075051076,-12.2282147950712));
#28558=CARTESIAN_POINT('Ctrl Pts',(42.8588810395273,0.462329209534337,-12.2768344282141));
#28559=CARTESIAN_POINT('Ctrl Pts',(42.9430983303904,0.474720322453312,-12.3245056174194));
#28560=CARTESIAN_POINT('Ctrl Pts',(42.9739518538696,0.479259883028827,-12.3419702513485));
#28561=CARTESIAN_POINT('Ctrl Pts',(43.0048507962696,0.483871351127161,-12.3593072142871));
#28562=CARTESIAN_POINT('Ctrl Pts',(43.0357916073031,0.48855404931147,-12.3764975648787));
#28563=CARTESIAN_POINT('Ctrl Pts',(43.0688709401821,0.49356039939852,-12.394876053048));
#28564=CARTESIAN_POINT('Ctrl Pts',(43.1019981319312,0.498648178118461,-12.413086934805));
#28565=CARTESIAN_POINT('Ctrl Pts',(43.1351685474621,0.503815669246779,-12.4311044326627));
#28566=CARTESIAN_POINT('Ctrl Pts',(43.2619434026418,0.523565435083243,-12.4999659662025));
#28567=CARTESIAN_POINT('Ctrl Pts',(43.3894520501079,0.544650665563608,-12.5675782480188));
#28568=CARTESIAN_POINT('Ctrl Pts',(43.517587224881,0.567178250965569,-12.6339106825963));
#28569=CARTESIAN_POINT('Ctrl Pts',(43.5580986076791,0.574300601540666,-12.6548824310164));
#28570=CARTESIAN_POINT('Ctrl Pts',(43.5986725234741,0.581566783988415,-12.6757260768497));
#28571=CARTESIAN_POINT('Ctrl Pts',(43.639305355365,0.588979215694766,-12.6964402253611));
#28572=CARTESIAN_POINT('Ctrl Pts',(43.770820391591,0.612970805230051,-12.7634850722274));
#28573=CARTESIAN_POINT('Ctrl Pts',(43.902951595011,0.63849760106563,-12.8291686268927));
#28574=CARTESIAN_POINT('Ctrl Pts',(44.0355913256016,0.665605135682187,-12.8934021229607));
#28575=CARTESIAN_POINT('Ctrl Pts',(44.170902783624,0.693258690284793,-12.9589294575546));
#28576=CARTESIAN_POINT('Ctrl Pts',(44.3067430280389,0.722557229868377,-13.0229470822634));
#28577=CARTESIAN_POINT('Ctrl Pts',(44.442994733047,0.753494258239274,-13.0853521869752));
#28578=CARTESIAN_POINT('Ctrl Pts',(44.5847248842449,0.785675211192184,-13.1502664933744));
#28579=CARTESIAN_POINT('Ctrl Pts',(44.7268998030087,0.819628907971195,-13.2134353747213));
#28580=CARTESIAN_POINT('Ctrl Pts',(44.869391068584,0.855290801050117,-13.2747439186379));
#28581=CARTESIAN_POINT('Ctrl Pts',(44.9602833090406,0.878038787375999,-13.313851374756));
#28582=CARTESIAN_POINT('Ctrl Pts',(45.0513043719664,0.901480660320446,-13.3522019415445));
#28583=CARTESIAN_POINT('Ctrl Pts',(45.1424228228309,0.925589006286844,-13.3897675411456));
#28584=CARTESIAN_POINT('Ctrl Pts',(45.2989388033037,0.967000393011594,-13.4542947208534));
#28585=CARTESIAN_POINT('Ctrl Pts',(45.4557410008675,1.01038049562556,-13.5165049785781));
#28586=CARTESIAN_POINT('Ctrl Pts',(45.6126867596284,1.05554311938658,-13.5762731041656));
#28587=CARTESIAN_POINT('Ctrl Pts',(45.634793280895,1.06190447958204,-13.5846917154731));
#28588=CARTESIAN_POINT('Ctrl Pts',(45.6569026820318,1.0683011314888,-13.5930619004269));
#28589=CARTESIAN_POINT('Ctrl Pts',(45.6790145959132,1.07473248690174,-13.6013833344557));
#28590=CARTESIAN_POINT('Ctrl Pts',(45.7022331439354,1.0814857121225,-13.6101212309873));
#28591=CARTESIAN_POINT('Ctrl Pts',(45.725454460823,1.08827720199514,-13.6188053740536));
#28592=CARTESIAN_POINT('Ctrl Pts',(45.7486783960119,1.09510594231381,-13.6274355210719));
#28593=CARTESIAN_POINT('Ctrl Pts',(45.8897873508652,1.1365974639485,-13.6798724149958));
#28594=CARTESIAN_POINT('Ctrl Pts',(46.0310824355953,1.17949718829418,-13.730358540107));
#28595=CARTESIAN_POINT('Ctrl Pts',(46.1724531782968,1.22353169119453,-13.7788017971356));
#28596=CARTESIAN_POINT('Ctrl Pts',(46.32153255783,1.26996729905082,-13.8298865588224));
#28597=CARTESIAN_POINT('Ctrl Pts',(46.470696032981,1.31766399879709,-13.8786996052067));
#28598=CARTESIAN_POINT('Ctrl Pts',(46.6198588270415,1.36626728785705,-13.925153963532));
#28599=CARTESIAN_POINT('Ctrl Pts',(46.7838432849947,1.41970007625068,-13.9762242912066));
#28600=CARTESIAN_POINT('Ctrl Pts',(46.9478267103645,1.4742275693381,-14.0244438551355));
#28601=CARTESIAN_POINT('Ctrl Pts',(47.111751758602,1.52935338987879,-14.0697223547562));
#28602=CARTESIAN_POINT('Ctrl Pts',(47.2839815191092,1.58727197505886,-14.1172947375594));
#28603=CARTESIAN_POINT('Ctrl Pts',(47.4561473004127,1.64584955469103,-14.1616207839425));
#28604=CARTESIAN_POINT('Ctrl Pts',(47.6282383345528,1.70450420101496,-14.202620250181));
#28605=CARTESIAN_POINT('Ctrl Pts',(47.8063777312818,1.76522034095631,-14.2450606958348));
#28606=CARTESIAN_POINT('Ctrl Pts',(47.9844378704465,1.8260174434581,-14.2839370275261));
#28607=CARTESIAN_POINT('Ctrl Pts',(48.1624546904282,1.88626804703706,-14.3191803292874));
#28608=CARTESIAN_POINT('Ctrl Pts',(48.2845509541258,1.92759208362686,-14.3433526264101));
#28609=CARTESIAN_POINT('Ctrl Pts',(48.4066278478853,1.96865945200782,-14.3658162976994));
#28610=CARTESIAN_POINT('Ctrl Pts',(48.5287060210717,2.00927801867859,-14.3865528070135));
#28611=CARTESIAN_POINT('Ctrl Pts',(48.5795058047287,2.02618042101204,-14.395181787604));
#28612=CARTESIAN_POINT('Ctrl Pts',(48.6303058803714,2.04300521698769,-14.4035117170511));
#28613=CARTESIAN_POINT('Ctrl Pts',(48.6811080503884,2.0597445246276,-14.411546778321));
#28614=CARTESIAN_POINT('Ctrl Pts',(48.7698851510948,2.08899656641255,-14.4255880966996));
#28615=CARTESIAN_POINT('Ctrl Pts',(48.8586361317935,2.11796377610708,-14.4387002156688));
#28616=CARTESIAN_POINT('Ctrl Pts',(48.9476431695491,2.14671805951331,-14.4509851041558));
#28617=CARTESIAN_POINT('Ctrl Pts',(49.1289020390981,2.20527487744969,-14.4760027326024));
#28618=CARTESIAN_POINT('Ctrl Pts',(49.3112299792474,2.26296695841828,-14.4976102350092));
#28619=CARTESIAN_POINT('Ctrl Pts',(49.494313376004,2.3190836575616,-14.5153939546957));
#28620=CARTESIAN_POINT('Ctrl Pts',(49.6708418613708,2.37319121771753,-14.5325409661456));
#28621=CARTESIAN_POINT('Ctrl Pts',(49.848074175385,2.42583287289,-14.5461339316348));
#28622=CARTESIAN_POINT('Ctrl Pts',(50.0257615281202,2.47639372396407,-14.5558261649752));
#28623=CARTESIAN_POINT('Ctrl Pts',(50.1942980989071,2.52435072441977,-14.5650192546652));
#28624=CARTESIAN_POINT('Ctrl Pts',(50.3630915255812,2.5704970187266,-14.5708751277587));
#28625=CARTESIAN_POINT('Ctrl Pts',(50.5321948117733,2.61460905768064,-14.5734097802231));
#28626=CARTESIAN_POINT('Ctrl Pts',(50.6971710074472,2.65764450976398,-14.5758825726232));
#28627=CARTESIAN_POINT('Ctrl Pts',(50.8624427189907,2.69874393343093,-14.5751944305834));
#28628=CARTESIAN_POINT('Ctrl Pts',(51.0280432903485,2.73774622267041,-14.57135806409));
#28629=CARTESIAN_POINT('Ctrl Pts',(51.1178357570973,2.75889416757757,-14.5692778972888));
#28630=CARTESIAN_POINT('Ctrl Pts',(51.2077245811264,2.77942633997864,-14.5662720832095));
#28631=CARTESIAN_POINT('Ctrl Pts',(51.2977121284949,2.7993227910621,-14.5623421493354));
#28632=CARTESIAN_POINT('Ctrl Pts',(51.476572612791,2.83886925032923,-14.5545309588261));
#28633=CARTESIAN_POINT('Ctrl Pts',(51.6558242884339,2.8759015177138,-14.5430693891014));
#28634=CARTESIAN_POINT('Ctrl Pts',(51.8353539157248,2.91049258394627,-14.5279826127422));
#28635=CARTESIAN_POINT('Ctrl Pts',(52.0277244870162,2.94755779303254,-14.5118167473585));
#28636=CARTESIAN_POINT('Ctrl Pts',(52.2204143047013,2.98182029930665,-14.4914887915954));
#28637=CARTESIAN_POINT('Ctrl Pts',(52.4132556251568,3.01342421633923,-14.4670192086256));
#28638=CARTESIAN_POINT('Ctrl Pts',(52.6151364581437,3.0465095793782,-14.4414026043567));
#28639=CARTESIAN_POINT('Ctrl Pts',(52.8171832798044,3.07668189726131,-14.4112472444537));
#28640=CARTESIAN_POINT('Ctrl Pts',(53.0191731687535,3.10415715631786,-14.3765615055575));
#28641=CARTESIAN_POINT('Ctrl Pts',(53.23945350474,3.13412033580066,-14.3387349279118));
#28642=CARTESIAN_POINT('Ctrl Pts',(53.4596662303745,3.16087663619287,-14.2955208513539));
#28643=CARTESIAN_POINT('Ctrl Pts',(53.6794860987647,3.18475461457528,-14.2469064357038));
#28644=CARTESIAN_POINT('Ctrl Pts',(53.8355717274022,3.20170944806556,-14.2123872101072));
#28645=CARTESIAN_POINT('Ctrl Pts',(53.9914584891298,3.2172141704109,-14.1751446872917));
#28646=CARTESIAN_POINT('Ctrl Pts',(54.1470201860804,3.23139546016389,-14.1351660195684));
#28647=CARTESIAN_POINT('Ctrl Pts',(54.237177508032,3.23961436707358,-14.1119959867918));
#28648=CARTESIAN_POINT('Ctrl Pts',(54.3272254441774,3.24738868938361,-14.0879067247933));
#28649=CARTESIAN_POINT('Ctrl Pts',(54.4171337810238,3.25474330129036,-14.0628870997708));
#28650=CARTESIAN_POINT('Ctrl Pts',(54.4848782213328,3.26028487935518,-14.0440352273712));
#28651=CARTESIAN_POINT('Ctrl Pts',(54.5525599073258,3.26558501280704,-14.0246434861282));
#28652=CARTESIAN_POINT('Ctrl Pts',(54.6201763752903,3.27066606446067,-14.00471935415));
#28653=CARTESIAN_POINT('Ctrl Pts',(54.8212606123777,3.28577657564425,-13.9454670891459));
#28654=CARTESIAN_POINT('Ctrl Pts',(55.0217685357112,3.29894547064154,-13.8815092378663));
#28655=CARTESIAN_POINT('Ctrl Pts',(55.2216267544097,3.31081104799838,-13.8129634769434));
#28656=CARTESIAN_POINT('Ctrl Pts',(55.406937860943,3.32181296367628,-13.7494069672962));
#28657=CARTESIAN_POINT('Ctrl Pts',(55.5916903573697,3.33169575577238,-13.6819049981657));
#28658=CARTESIAN_POINT('Ctrl Pts',(55.7758214214221,3.34100312231682,-13.6105321875762));
#28659=CARTESIAN_POINT('Ctrl Pts',(56.0257234664947,3.35363504809027,-13.5136652552054));
#28660=CARTESIAN_POINT('Ctrl Pts',(56.2744888438065,3.36519900722206,-13.4096494123916));
#28661=CARTESIAN_POINT('Ctrl Pts',(56.5208818625146,3.37649328426046,-13.298125861323));
#28662=CARTESIAN_POINT('Ctrl Pts',(56.5403976007538,3.37738785568719,-13.2892925573537));
#28663=CARTESIAN_POINT('Ctrl Pts',(56.5598984329187,3.37828073365513,-13.2804121394665));
#28664=CARTESIAN_POINT('Ctrl Pts',(56.5793837321424,3.37917231069026,-13.2714844240186));
#28665=CARTESIAN_POINT('Ctrl Pts',(56.7011413747803,3.38474350140081,-13.2156978756783));
#28666=CARTESIAN_POINT('Ctrl Pts',(56.8222678009723,3.39029559284719,-13.158134882614));
#28667=CARTESIAN_POINT('Ctrl Pts',(56.9427407283792,3.39596934234435,-13.0987731088611));
#28668=CARTESIAN_POINT('Ctrl Pts',(57.0022426840281,3.39877162496676,-13.069454143139));
#28669=CARTESIAN_POINT('Ctrl Pts',(57.0615852070991,3.40160350710119,-13.0396962421641));
#28670=CARTESIAN_POINT('Ctrl Pts',(57.1207634691196,3.40448790678842,-13.0095138025368));
#28671=CARTESIAN_POINT('Ctrl Pts',(57.2394457744615,3.41027258502532,-12.948982766418));
#28672=CARTESIAN_POINT('Ctrl Pts',(57.3574683316654,3.41626782467713,-12.8867410811329));
#28673=CARTESIAN_POINT('Ctrl Pts',(57.4747616997881,3.42264482405701,-12.8229308281502));
#28674=CARTESIAN_POINT('Ctrl Pts',(57.524842042396,3.42536758936647,-12.7956859857314));
#28675=CARTESIAN_POINT('Ctrl Pts',(57.5747892882394,3.42816006754099,-12.7681557937622));
#28676=CARTESIAN_POINT('Ctrl Pts',(57.6245972805189,3.43103602860081,-12.7403541019914));
#28677=CARTESIAN_POINT('Ctrl Pts',(57.6968840889615,3.43520993798171,-12.7000052448014));
#28678=CARTESIAN_POINT('Ctrl Pts',(57.768876811572,3.43957742139646,-12.6591218520253));
#28679=CARTESIAN_POINT('Ctrl Pts',(57.8405471761051,3.44417469677127,-12.6177486205741));
#28680=CARTESIAN_POINT('Ctrl Pts',(57.9103178844631,3.44865011923504,-12.5774720057666));
#28681=CARTESIAN_POINT('Ctrl Pts',(57.979782361742,3.45334489481511,-12.5367356281187));
#28682=CARTESIAN_POINT('Ctrl Pts',(58.0489530044697,3.45817075099943,-12.4952150159453));
#28683=CARTESIAN_POINT('Ctrl Pts',(58.1158780081092,3.46283993477397,-12.4550423789532));
#28684=CARTESIAN_POINT('Ctrl Pts',(58.1825279258874,3.46763181259156,-12.4141355213333));
#28685=CARTESIAN_POINT('Ctrl Pts',(58.2489206708859,3.47244908344074,-12.3721579743786));
#28686=CARTESIAN_POINT('Ctrl Pts',(58.2905482136799,3.47546946086947,-12.3458385002812));
#28687=CARTESIAN_POINT('Ctrl Pts',(58.3320756067246,3.47849784936122,-12.3190926740185));
#28688=CARTESIAN_POINT('Ctrl Pts',(58.3734322388319,3.4817278052044,-12.2924709828604));
#28689=CARTESIAN_POINT('Ctrl Pts',(58.3766957722737,3.48198268739313,-12.2903702126828));
#28690=CARTESIAN_POINT('Ctrl Pts',(58.3799582378835,3.48223883340623,-12.2882702406214));
#28691=CARTESIAN_POINT('Ctrl Pts',(58.3832195986403,3.48249634281616,-12.2861713501478));
#28692=CARTESIAN_POINT('Ctrl Pts',(58.4107742785886,3.48467199583441,-12.2684381830568));
#28693=CARTESIAN_POINT('Ctrl Pts',(58.4382726399568,3.48687721189157,-12.2505993231288));
#28694=CARTESIAN_POINT('Ctrl Pts',(58.4657016549427,3.48916124785644,-12.2327797434489));
#28695=CARTESIAN_POINT('Ctrl Pts',(58.492300617373,3.49137616468266,-12.2154994170984));
#28696=CARTESIAN_POINT('Ctrl Pts',(58.5188344931624,3.49366487702235,-12.1982362815353));
#28697=CARTESIAN_POINT('Ctrl Pts',(58.5452842975648,3.49609103963997,-12.1811518796883));
#28698=CARTESIAN_POINT('Ctrl Pts',(58.5688654567635,3.49825406988614,-12.165920387098));
#28699=CARTESIAN_POINT('Ctrl Pts',(58.5923797907988,3.5005263639239,-12.150830927202));
#28700=CARTESIAN_POINT('Ctrl Pts',(58.6158074637682,3.50296975356874,-12.1360415899455));
#28701=CARTESIAN_POINT('Ctrl Pts',(58.6186574373906,3.50326699162759,-12.1342424688323));
#28702=CARTESIAN_POINT('Ctrl Pts',(58.6215061199422,3.50356678411242,-12.1324478482872));
#28703=CARTESIAN_POINT('Ctrl Pts',(58.624353468298,3.5038692616587,-12.1306580639657));
#28704=CARTESIAN_POINT('Ctrl Pts',(58.6261974023257,3.50406514518629,-12.1294990051502));
#28705=CARTESIAN_POINT('Ctrl Pts',(58.6280412554071,3.50426063077623,-12.128338325465));
#28706=CARTESIAN_POINT('Ctrl Pts',(58.6298850303881,3.50445571262044,-12.1271760060145));
#28707=CARTESIAN_POINT('',(64.2981106326832,3.0811123562608,-5.85555843435015));
#28708=CARTESIAN_POINT('Ctrl Pts',(58.6309985074851,3.50412516642371,-12.1267371940558));
#28709=CARTESIAN_POINT('Ctrl Pts',(59.3307183820628,3.57738713031641,-11.6860335001487));
#28710=CARTESIAN_POINT('Ctrl Pts',(60.517944889496,3.73981722935225,-10.8310066664578));
#28711=CARTESIAN_POINT('Ctrl Pts',(61.9030047025891,3.76645360291022,-9.51895198440983));
#28712=CARTESIAN_POINT('Ctrl Pts',(63.1474965884414,3.51873308138032,-7.98696741401787));
#28713=CARTESIAN_POINT('Ctrl Pts',(63.8841059835174,3.19246873749153,-6.72699339972162));
#28714=CARTESIAN_POINT('Ctrl Pts',(64.2977768285069,3.08120206602316,-5.85626119470832));
#28715=CARTESIAN_POINT('',(65.9408742037128,3.18204282773931,0.563892468411459));
#28716=CARTESIAN_POINT('Ctrl Pts',(64.2990162441269,3.08086897348378,-5.8536518439966));
#28717=CARTESIAN_POINT('Ctrl Pts',(64.6116198958172,2.99692695046148,-5.19539506303037));
#28718=CARTESIAN_POINT('Ctrl Pts',(65.2801899672622,2.94481025351616,-3.5511642822986));
#28719=CARTESIAN_POINT('Ctrl Pts',(65.7244715160515,3.1204547806088,-1.64454837118901));
#28720=CARTESIAN_POINT('Ctrl Pts',(65.8904051975644,3.18227049415762,-0.202227005722761));
#28721=CARTESIAN_POINT('Ctrl Pts',(65.9273187549476,3.18706519524341,0.294007279412763));
#28722=CARTESIAN_POINT('Ctrl Pts',(65.9407606432144,3.18152655267827,0.560435122518436));
#28723=CARTESIAN_POINT('',(65.1820057808194,3.08346314704612,6.62245362259951));
#28724=CARTESIAN_POINT('Ctrl Pts',(65.9410186585186,3.18269955622032,0.568290390542557));
#28725=CARTESIAN_POINT('Ctrl Pts',(65.9482910538458,3.17968929367419,0.713809495459604));
#28726=CARTESIAN_POINT('Ctrl Pts',(65.9538461064654,3.17693067006538,0.860231473819412));
#28727=CARTESIAN_POINT('Ctrl Pts',(65.9576971484804,3.17445963453872,1.00728204069835));
#28728=CARTESIAN_POINT('Ctrl Pts',(65.9616531303433,3.17192126396582,1.15833969554288));
#28729=CARTESIAN_POINT('Ctrl Pts',(65.9638107706592,3.1696861756633,1.31006037972726));
#28730=CARTESIAN_POINT('Ctrl Pts',(65.9641614268585,3.1677446692947,1.46216354030635));
#28731=CARTESIAN_POINT('Ctrl Pts',(65.9645256747771,3.16572790856114,1.62016234302247));
#28732=CARTESIAN_POINT('Ctrl Pts',(65.9629399442982,3.16402755556653,1.77857356369251));
#28733=CARTESIAN_POINT('Ctrl Pts',(65.9593729998557,3.16258514975214,1.93710510064369));
#28734=CARTESIAN_POINT('Ctrl Pts',(65.9554990511008,3.16101859711898,2.10928133161282));
#28735=CARTESIAN_POINT('Ctrl Pts',(65.949288022404,3.15975582648078,2.28159897580233));
#28736=CARTESIAN_POINT('Ctrl Pts',(65.9406774857124,3.15867302061577,2.45371636122117));
#28737=CARTESIAN_POINT('Ctrl Pts',(65.9315288686373,3.15752254921307,2.63658952088078));
#28738=CARTESIAN_POINT('Ctrl Pts',(65.9196710752013,3.15657393498886,2.81923624761305));
#28739=CARTESIAN_POINT('Ctrl Pts',(65.9050093929959,3.15564006925673,3.00128898965019));
#28740=CARTESIAN_POINT('Ctrl Pts',(65.8893468159611,3.15464245221901,3.19576974954009));
#28741=CARTESIAN_POINT('Ctrl Pts',(65.8704837728399,3.15365958243021,3.38957235660907));
#28742=CARTESIAN_POINT('Ctrl Pts',(65.8482914544987,3.15244777519672,3.58230111020626));
#28743=CARTESIAN_POINT('Ctrl Pts',(65.8465233851039,3.15235123011075,3.59765587420649));
#28744=CARTESIAN_POINT('Ctrl Pts',(65.8447341805535,3.15225323446883,3.61300384904705));
#28745=CARTESIAN_POINT('Ctrl Pts',(65.8429237746156,3.15215366756841,3.6283448484288));
#28746=CARTESIAN_POINT('Ctrl Pts',(65.8267524394948,3.15126429260558,3.76537734312529));
#28747=CARTESIAN_POINT('Ctrl Pts',(65.8088894100432,3.150249141841,3.90185211718944));
#28748=CARTESIAN_POINT('Ctrl Pts',(65.7892859174208,3.14902631932301,4.03765352495476));
#28749=CARTESIAN_POINT('Ctrl Pts',(65.7625155923028,3.14735644564292,4.2231025113866));
#28750=CARTESIAN_POINT('Ctrl Pts',(65.7326172305382,3.14530962026868,4.4073328552257));
#28751=CARTESIAN_POINT('Ctrl Pts',(65.6994834206641,3.14270630129762,4.59044913856515));
#28752=CARTESIAN_POINT('Ctrl Pts',(65.6665345207502,3.14011751067718,4.77254350426792));
#28753=CARTESIAN_POINT('Ctrl Pts',(65.6303858121898,3.13697775158381,4.95353676926838));
#28754=CARTESIAN_POINT('Ctrl Pts',(65.5909440728671,3.1331492459991,5.13356289950103));
#28755=CARTESIAN_POINT('Ctrl Pts',(65.5796974902167,3.13205756989086,5.18489630385011));
#28756=CARTESIAN_POINT('Ctrl Pts',(65.5681832582793,3.13091016593668,5.23615126812696));
#28757=CARTESIAN_POINT('Ctrl Pts',(65.5563993018479,3.12970444792706,5.28733236991622));
#28758=CARTESIAN_POINT('Ctrl Pts',(65.5191527539497,3.12589343302229,5.449104807754));
#28759=CARTESIAN_POINT('Ctrl Pts',(65.4792102515102,3.12149696871513,5.61014156713253));
#28760=CARTESIAN_POINT('Ctrl Pts',(65.4365166245822,3.11646139895575,5.77056709721706));
#28761=CARTESIAN_POINT('Ctrl Pts',(65.4268592190441,3.1153223404409,5.80685575466259));
#28762=CARTESIAN_POINT('Ctrl Pts',(65.4170611155533,3.11415073489286,5.84311301303454));
#28763=CARTESIAN_POINT('Ctrl Pts',(65.4071218074921,3.11294623328413,5.87934008699024));
#28764=CARTESIAN_POINT('Ctrl Pts',(65.3803078629663,3.10969676771581,5.9770723179869));
#28765=CARTESIAN_POINT('Ctrl Pts',(65.3524660048671,3.10620755069197,6.07458048656183));
#28766=CARTESIAN_POINT('Ctrl Pts',(65.3235898025028,3.10247597339671,6.17180190452008));
#28767=CARTESIAN_POINT('Ctrl Pts',(65.3157399434555,3.10146156175691,6.19823108719857));
#28768=CARTESIAN_POINT('Ctrl Pts',(65.3078136652226,3.10042926681887,6.22463937508606));
#28769=CARTESIAN_POINT('Ctrl Pts',(65.2998108818847,3.09937909657588,6.25102616952741));
#28770=CARTESIAN_POINT('Ctrl Pts',(65.2810472815969,3.09691683140615,6.31289355277077));
#28771=CARTESIAN_POINT('Ctrl Pts',(65.2618630666386,3.09435625429473,6.37464772926933));
#28772=CARTESIAN_POINT('Ctrl Pts',(65.2422565977204,3.09169651310013,6.43643476558113));
#28773=CARTESIAN_POINT('Ctrl Pts',(65.2226501288021,3.08903677190554,6.49822180189292));
#28774=CARTESIAN_POINT('Ctrl Pts',(65.2026214010512,3.08627786254871,6.56004163681742));
#28775=CARTESIAN_POINT('Ctrl Pts',(65.1821694348226,3.08341966011011,6.62198291902686));
#28776=CARTESIAN_POINT('',(61.488060455579,2.54023853025181,12.6451667603895));
#28777=CARTESIAN_POINT('Ctrl Pts',(65.1820057808194,3.08346314704612,6.62245362259951));
#28778=CARTESIAN_POINT('Ctrl Pts',(64.4364313250544,2.978243913911,8.88068192566307));
#28779=CARTESIAN_POINT('Ctrl Pts',(63.1655278864518,2.76702770395235,10.9465222144682));
#28780=CARTESIAN_POINT('Ctrl Pts',(61.4888775365941,2.54034899309264,12.6443394503259));
#28781=CARTESIAN_POINT('',(39.0575084607384,0.182814626998845,12.6499766640859));
#28782=CARTESIAN_POINT('Ctrl Pts',(61.4877351764846,2.54019455511082,12.6454961116574));
#28783=CARTESIAN_POINT('Ctrl Pts',(61.1207173898856,2.49057863416769,13.0170698848163));
#28784=CARTESIAN_POINT('Ctrl Pts',(58.0875609241164,2.07105403856995,15.8393411259143));
#28785=CARTESIAN_POINT('Ctrl Pts',(49.8202147709309,0.844782240165095,18.8003653400802));
#28786=CARTESIAN_POINT('Ctrl Pts',(41.9948217404251,0.31563552772145,15.6461834941947));
#28787=CARTESIAN_POINT('Ctrl Pts',(39.0575084607384,0.182814626998845,12.6499766640859));
#28788=CARTESIAN_POINT('',(35.3362746312916,0.0544533848017485,6.63054475574935));
#28789=CARTESIAN_POINT('Ctrl Pts',(39.0562952757742,0.182759773910686,12.6487390081575));
#28790=CARTESIAN_POINT('Ctrl Pts',(37.384582188262,0.10718206711949,10.9431042532932));
#28791=CARTESIAN_POINT('Ctrl Pts',(36.0966585928923,0.0727769246540845,
8.89369604654459));
#28792=CARTESIAN_POINT('Ctrl Pts',(35.3362746312916,0.0544533848017485,
6.63054475574935));
#28793=CARTESIAN_POINT('',(34.5486968133484,0.0370407268214907,0.611571110133481));
#28794=CARTESIAN_POINT('Ctrl Pts',(35.3362641803865,0.0544531329586211,
6.63051365033307));
#28795=CARTESIAN_POINT('Ctrl Pts',(34.6842831176538,0.0387418751808522,
4.68999164416651));
#28796=CARTESIAN_POINT('Ctrl Pts',(34.4147629385807,0.0337921773623382,
2.65381724310736));
#28797=CARTESIAN_POINT('Ctrl Pts',(34.5486787314775,0.0370402882573318,
0.611846760577837));
#28798=CARTESIAN_POINT('',(36.1904970298096,0.0789173535423179,-5.40625271964083));
#28799=CARTESIAN_POINT('Ctrl Pts',(34.548710378627,0.0370410558386067,0.611364313220442));
#28800=CARTESIAN_POINT('Ctrl Pts',(34.6864441828166,0.0403816294309185,
-1.48783449464834));
#28801=CARTESIAN_POINT('Ctrl Pts',(35.2437959696896,0.0529688610259415,
-3.52821928318576));
#28802=CARTESIAN_POINT('Ctrl Pts',(36.1903620723292,0.0789136543077262,
-5.40598500767172));
#28803=CARTESIAN_POINT('Ctrl Pts',(36.1906166903305,0.0789206334815761,
-5.40649008739235));
#28804=CARTESIAN_POINT('Ctrl Pts',(36.5716643422744,0.089365667141814,-6.1623311541711));
#28805=CARTESIAN_POINT('Ctrl Pts',(37.0128131431011,0.103146882444921,-6.88399642848073));
#28806=CARTESIAN_POINT('Ctrl Pts',(37.5042795392924,0.118123058207631,-7.56121085790809));
#28807=CARTESIAN_POINT('Origin',(50.184,-32.64,1.632));
#28808=CARTESIAN_POINT('',(35.4961269461781,3.11629570184638,1.63325416304923));
#28809=CARTESIAN_POINT('',(35.496,-32.64,1.632));
#28810=CARTESIAN_POINT('',(45.4957186312967,4.13505468146236,-12.2876753485083));
#28811=CARTESIAN_POINT('Ctrl Pts',(45.4957186312967,4.13505468146236,-12.2876753485083));
#28812=CARTESIAN_POINT('Ctrl Pts',(46.5747881377784,4.51315986439798,-12.6511164012708));
#28813=CARTESIAN_POINT('Ctrl Pts',(48.7315111185874,5.55100447935154,-13.1127068857499));
#28814=CARTESIAN_POINT('Ctrl Pts',(52.2255324170519,6.61037667463491,-13.0603457351622));
#28815=CARTESIAN_POINT('Ctrl Pts',(55.7352401406832,6.78357937642121,-12.1273823391115));
#28816=CARTESIAN_POINT('Ctrl Pts',(57.8454449537772,6.76763575867449,-10.9565650346632));
#28817=CARTESIAN_POINT('Ctrl Pts',(58.9417818399741,6.90315486069136,-10.1604688849966));
#28818=CARTESIAN_POINT('Ctrl Pts',(59.1869377879013,6.93283823797164,-9.9764403477307));
#28819=CARTESIAN_POINT('Ctrl Pts',(59.6656000071998,6.98501272405032,-9.59287808094242));
#28820=CARTESIAN_POINT('Ctrl Pts',(60.4698386743377,7.03851518962114,-8.88527771072978));
#28821=CARTESIAN_POINT('Ctrl Pts',(61.935425590422,6.93159705832345,-7.32309238219473));
#28822=CARTESIAN_POINT('Ctrl Pts',(62.898870223949,6.33243798646893,-5.81981710521227));
#28823=CARTESIAN_POINT('Ctrl Pts',(63.6271064539284,6.1172012971021,-4.30394126827215));
#28824=CARTESIAN_POINT('Ctrl Pts',(63.9964631920437,6.08157109535702,-3.43096909542246));
#28825=CARTESIAN_POINT('Ctrl Pts',(64.4196909334568,6.16095583450854,-2.0750183342162));
#28826=CARTESIAN_POINT('Ctrl Pts',(64.7075353735302,6.25611577526355,-0.705188274299797));
#28827=CARTESIAN_POINT('Ctrl Pts',(64.8131179042321,6.27855936375402,0.234551382385882));
#28828=CARTESIAN_POINT('Ctrl Pts',(64.8578334301675,6.26126913644566,0.94307726867782));
#28829=CARTESIAN_POINT('Ctrl Pts',(64.8763131687878,6.25212971761612,1.41873044327074));
#28830=CARTESIAN_POINT('Ctrl Pts',(64.8669425474595,6.24148249015893,2.37159989960793));
#28831=CARTESIAN_POINT('Ctrl Pts',(64.7293383040315,6.23744524570034,4.02825143678288));
#28832=CARTESIAN_POINT('Ctrl Pts',(64.4090264396697,6.21556997011337,5.41180556034465));
#28833=CARTESIAN_POINT('Ctrl Pts',(63.392616944205,6.06901676370829,8.4362633730038));
#28834=CARTESIAN_POINT('Ctrl Pts',(62.2029128798603,5.85755777132363,10.3600282958658));
#28835=CARTESIAN_POINT('Ctrl Pts',(57.9137758164067,5.23547967962912,14.7285512014021));
#28836=CARTESIAN_POINT('Ctrl Pts',(50.2340493278717,3.97178337193033,17.9121952059345));
#28837=CARTESIAN_POINT('Ctrl Pts',(42.4627846177445,3.39626629188669,14.7465965189029));
#28838=CARTESIAN_POINT('Ctrl Pts',(38.1616839203783,3.18800029201627,10.3559731559896));
#28839=CARTESIAN_POINT('Ctrl Pts',(36.9711393616719,3.15313406811575,8.42495263430108));
#28840=CARTESIAN_POINT('Ctrl Pts',(35.7546310141604,3.1216063944377,4.80652569193013));
#28841=CARTESIAN_POINT('Ctrl Pts',(35.4967618613831,3.11596821566591,3.22213036278666));
#28842=CARTESIAN_POINT('Ctrl Pts',(35.4961269461781,3.11629570184638,1.63325416304923));
#28843=CARTESIAN_POINT('Ctrl Pts',(35.4961269461781,3.11629570184638,1.63325416304923));
#28844=CARTESIAN_POINT('Ctrl Pts',(35.4959999928206,3.11636118377183,1.31555320625316));
#28845=CARTESIAN_POINT('Ctrl Pts',(35.5061575990416,3.11666518074569,0.997673098419422));
#28846=CARTESIAN_POINT('Ctrl Pts',(35.6531385708734,3.12046556629585,-1.27776505111417));
#28847=CARTESIAN_POINT('Ctrl Pts',(36.175035699066,3.13335329444264,-3.19875344300605));
#28848=CARTESIAN_POINT('Ctrl Pts',(37.619750560802,3.17534463244499,-6.07811908458911));
#28849=CARTESIAN_POINT('Ctrl Pts',(39.0211463611516,3.22647042745986,-8.16085205297379));
#28850=CARTESIAN_POINT('Ctrl Pts',(40.9332506662835,3.2798490343456,-9.84541367809451));
#28851=CARTESIAN_POINT('Ctrl Pts',(42.2378053070641,3.41504440953276,-10.725652165237));
#28852=CARTESIAN_POINT('Ctrl Pts',(42.8038448826665,3.4807437957151,-11.0806258189848));
#28853=CARTESIAN_POINT('Ctrl Pts',(43.981345015687,3.67284868940879,-11.7113672365034));
#28854=CARTESIAN_POINT('Ctrl Pts',(44.8918845743013,3.92347165996875,-12.0842981943491));
#28855=CARTESIAN_POINT('Ctrl Pts',(45.4957186312967,4.13505468146236,-12.2876753485083));
#28856=CARTESIAN_POINT('Ctrl Pts',(-79.0674188627527,5.01522288740334,24.8190563538896));
#28857=CARTESIAN_POINT('Ctrl Pts',(-79.0681685301284,5.01561150558399,24.7698112319613));
#28858=CARTESIAN_POINT('Ctrl Pts',(-79.0689540583035,5.01601910927839,24.720540203059));
#28859=CARTESIAN_POINT('Ctrl Pts',(-79.0782218386017,5.02082390331305,24.1661600265106));
#28860=CARTESIAN_POINT('Ctrl Pts',(-79.0927115085079,5.02499992560426,23.175201774565));
#28861=CARTESIAN_POINT('Ctrl Pts',(-79.1310390764956,5.03563895843973,21.1518987112308));
#28862=CARTESIAN_POINT('Ctrl Pts',(-79.1918027806567,5.0685749771201,19.6199982936506));
#28863=CARTESIAN_POINT('Ctrl Pts',(-79.2833423745251,5.13810264877128,18.333204648019));
#28864=CARTESIAN_POINT('Ctrl Pts',(-79.3271997238556,5.16402211160836,17.8495119052833));
#28865=CARTESIAN_POINT('Ctrl Pts',(-79.4350333727236,5.21929371286925,16.8471015925371));
#28866=CARTESIAN_POINT('Ctrl Pts',(-79.6597754282508,5.33693138686091,15.0668568651258));
#28867=CARTESIAN_POINT('Ctrl Pts',(-79.8528862432256,5.52342881968698,13.4624410469408));
#28868=CARTESIAN_POINT('Ctrl Pts',(-79.9478677581679,5.77956933135521,12.0840553347989));
#28869=CARTESIAN_POINT('Ctrl Pts',(-79.987251247416,5.88971937931585,11.5496610322703));
#28870=CARTESIAN_POINT('Ctrl Pts',(-80.0644593134605,6.14288539486632,10.4849494061586));
#28871=CARTESIAN_POINT('Ctrl Pts',(-80.1868754301937,6.65297538854495,8.65255241882749));
#28872=CARTESIAN_POINT('Ctrl Pts',(-80.2380448998663,7.15195302098414,7.11347352122868));
#28873=CARTESIAN_POINT('Ctrl Pts',(-80.2204406795539,7.50474337783514,5.96584700843978));
#28874=CARTESIAN_POINT('Ctrl Pts',(-80.2096612212723,7.59336289588965,5.67864593273452));
#28875=CARTESIAN_POINT('Ctrl Pts',(-80.1847401855017,7.77374083996654,5.13331455388711));
#28876=CARTESIAN_POINT('Ctrl Pts',(-80.1261994373432,8.1062734462045,4.1910399007512));
#28877=CARTESIAN_POINT('Ctrl Pts',(-79.9741038356724,8.78915237629665,2.39877332558468));
#28878=CARTESIAN_POINT('Ctrl Pts',(-79.83947806308,9.27574137610065,0.998413592090816));
#28879=CARTESIAN_POINT('Ctrl Pts',(-79.7762751651938,9.47255640374571,0.106471325025258));
#28880=CARTESIAN_POINT('Ctrl Pts',(-79.7671955870895,9.49782362033992,-0.0121281782206109));
#28881=CARTESIAN_POINT('Ctrl Pts',(-79.7492052491573,9.54450055919095,-0.242617706451281));
#28882=CARTESIAN_POINT('Ctrl Pts',(-79.7157711688734,9.62061509733319,-0.650089358255339));
#28883=CARTESIAN_POINT('Ctrl Pts',(-79.6641805384973,9.71223607414345,-1.23187966460342));
#28884=CARTESIAN_POINT('Ctrl Pts',(-79.596965198778,9.79990417771364,-1.93470237003412));
#28885=CARTESIAN_POINT('Ctrl Pts',(-79.502992870302,9.89209711001119,-2.87653830176489));
#28886=CARTESIAN_POINT('Ctrl Pts',(-79.3825611224459,9.97162253608378,-4.06583643950883));
#28887=CARTESIAN_POINT('Ctrl Pts',(-79.2987282925754,10.0151797765619,-5.03298138339086));
#28888=CARTESIAN_POINT('Ctrl Pts',(-79.2557159682984,10.0403140537843,-5.64265285224522));
#28889=CARTESIAN_POINT('Ctrl Pts',(-79.2392565381024,10.0469385074052,-5.86265283336235));
#28890=CARTESIAN_POINT('Ctrl Pts',(-79.2076279337785,10.0536787811717,-6.32229182536503));
#28891=CARTESIAN_POINT('Ctrl Pts',(-79.1565003952743,10.0478001857035,-7.13344029341454));
#28892=CARTESIAN_POINT('Ctrl Pts',(-79.0957089826259,10.0015429336662,-8.33665236197077));
#28893=CARTESIAN_POINT('Ctrl Pts',(-79.0509111925855,9.93743960636052,-9.58843110743809));
#28894=CARTESIAN_POINT('Ctrl Pts',(-79.0268836059977,9.90337528247544,-10.4912277578721));
#28895=CARTESIAN_POINT('Ctrl Pts',(-79.0150770197293,9.89016083945574,-11.0141122843214));
#28896=CARTESIAN_POINT('Ctrl Pts',(-79.0097812960411,9.88618631938345,-11.2780557265188));
#28897=CARTESIAN_POINT('Ctrl Pts',(-79.006009248494,9.88440003313119,-11.477499488386));
#28898=CARTESIAN_POINT('Ctrl Pts',(-79.0036660448527,9.88335825035133,-11.6033946515416));
#28899=CARTESIAN_POINT('Ctrl Pts',(-78.9997418352511,9.88164895132235,-11.8592855042488));
#28900=CARTESIAN_POINT('Ctrl Pts',(-78.9947630668099,9.87966515108148,-12.3037147121711));
#28901=CARTESIAN_POINT('Ctrl Pts',(-78.9906403941104,9.87901424697721,-13.4432992984675));
#28902=CARTESIAN_POINT('Ctrl Pts',(-79.0055407029075,9.88809071261166,-14.6957989450663));
#28903=CARTESIAN_POINT('Ctrl Pts',(-79.0211143843459,9.89743215908292,-15.9454740463632));
#28904=CARTESIAN_POINT('Ctrl Pts',(-79.0275077450161,9.90133084380334,-16.5699512235593));
#28905=CARTESIAN_POINT('Ctrl Pts',(-79.0308484282295,9.90348313569322,-17.0700172931005));
#28906=CARTESIAN_POINT('Ctrl Pts',(-79.0317719310497,9.90415043469421,-17.3202164975421));
#28907=CARTESIAN_POINT('Ctrl Pts',(-79.0321242967022,9.9044653528448,-17.5072310514656));
#28908=CARTESIAN_POINT('Ctrl Pts',(-79.0323391539848,9.90466318448756,-17.6318736318689));
#28909=CARTESIAN_POINT('Ctrl Pts',(-79.0327007960053,9.90501350062777,-17.8806948619788));
#28910=CARTESIAN_POINT('Ctrl Pts',(-79.0329656912022,9.90529980852707,-18.1298687447505));
#28911=CARTESIAN_POINT('Ctrl Pts',(-79.0331441220501,9.90552904669751,-18.3791056565332));
#28912=CARTESIAN_POINT('Ctrl Pts',(-79.0332219147693,9.90564971859517,-18.5349686127661));
#28913=CARTESIAN_POINT('Ctrl Pts',(-79.0332651945694,9.90573358901976,-18.6596927977821));
#28914=CARTESIAN_POINT('Ctrl Pts',(-79.0332962921471,9.90580926151893,-18.784447455142));
#28915=CARTESIAN_POINT('Ctrl Pts',(-79.0333334879728,9.90598436409335,-19.1276271558624));
#28916=CARTESIAN_POINT('Ctrl Pts',(-79.033150149307,9.90610435638902,-19.6898219898101));
#28917=CARTESIAN_POINT('Ctrl Pts',(-79.0323557181868,9.90598203971701,-20.6911245536626));
#28918=CARTESIAN_POINT('Ctrl Pts',(-79.0309067855052,9.90546320762363,-21.9464416288123));
#28919=CARTESIAN_POINT('Ctrl Pts',(-79.0301647578065,9.90521322820462,-22.9549301708349));
#28920=CARTESIAN_POINT('Ctrl Pts',(-79.0301129783275,9.90528407108641,-23.5849311303309));
#28921=CARTESIAN_POINT('Ctrl Pts',(-79.0301033887371,9.90531333336311,-23.8340998786223));
#28922=CARTESIAN_POINT('Ctrl Pts',(-79.0301224332957,9.90537495702407,-24.3333441865812));
#28923=CARTESIAN_POINT('Ctrl Pts',(-79.0302414377352,9.90548775645281,-25.2087899694315));
#28924=CARTESIAN_POINT('Ctrl Pts',(-79.0305728693895,9.90564301980743,-26.4634885419102));
#28925=CARTESIAN_POINT('Ctrl Pts',(-79.0309607127377,9.90576143657678,-27.9717423759188));
#28926=CARTESIAN_POINT('Ctrl Pts',(-79.0310348337779,9.90575248186518,-28.9764101349217));
#28927=CARTESIAN_POINT('Ctrl Pts',(-79.030974280901,9.90571219648468,-29.5405779895657));
#28928=CARTESIAN_POINT('Ctrl Pts',(-79.0309568887622,9.90570176770536,-29.6659328550826));
#28929=CARTESIAN_POINT('Ctrl Pts',(-79.0309075280054,9.90567508984067,-29.9167097800688));
#28930=CARTESIAN_POINT('Ctrl Pts',(-79.0307858008553,9.90561395783502,-30.3557101965222));
#28931=CARTESIAN_POINT('Ctrl Pts',(-79.0304240360459,9.90544214485433,-31.2341706185155));
#28932=CARTESIAN_POINT('Ctrl Pts',(-79.0298462642804,9.9051666773888,-32.2385881451622));
#28933=CARTESIAN_POINT('Ctrl Pts',(-79.0293158017111,9.90488352664045,-33.2423420548747));
#28934=CARTESIAN_POINT('Ctrl Pts',(-79.0289945391947,9.90468490150068,-33.9945417552978));
#28935=CARTESIAN_POINT('Ctrl Pts',(-79.0288029824139,9.90451656743563,-34.7458244521028));
#28936=CARTESIAN_POINT('Ctrl Pts',(-79.0287969944716,9.9044364311933,-35.2458865326991));
#28937=CARTESIAN_POINT('Ctrl Pts',(-79.0288514758595,9.90439296894784,-35.621556386843));
#28938=CARTESIAN_POINT('Ctrl Pts',(-79.0289076082456,9.90434486162714,-35.8728434773854));
#28939=CARTESIAN_POINT('Ctrl Pts',(-79.0290895293272,9.9041887700443,-36.3750481796481));
#28940=CARTESIAN_POINT('Ctrl Pts',(-79.0295684482691,9.90379477628602,-37.2525756949588));
#28941=CARTESIAN_POINT('Ctrl Pts',(-79.030982819889,9.90286430485681,-39.0047230445932));
#28942=CARTESIAN_POINT('Ctrl Pts',(-79.0323534352322,9.90290751671525,-40.5079837793973));
#28943=CARTESIAN_POINT('Ctrl Pts',(-79.0328296458239,9.90448811011299,-41.641571295867));
#28944=CARTESIAN_POINT('Ctrl Pts',(-79.032917209571,9.90467855354968,-41.8894380420173));
#28945=CARTESIAN_POINT('Ctrl Pts',(-79.0330029087558,9.90459602900717,-42.2635358200489));
#28946=CARTESIAN_POINT('Ctrl Pts',(-79.0330513003446,9.90424331849555,-42.6380823834483));
#28947=CARTESIAN_POINT('Ctrl Pts',(-79.033076820358,9.90354620635817,-43.1388767357607));
#28948=CARTESIAN_POINT('Ctrl Pts',(-79.0330556176558,9.90250041232264,-43.7667436589721));
#28949=CARTESIAN_POINT('Ctrl Pts',(-79.0330088168266,9.90177277904131,-44.5229039800781));
#28950=CARTESIAN_POINT('Ctrl Pts',(-79.0330042982439,9.90228299286789,-45.1548080059856));
#28951=CARTESIAN_POINT('Ctrl Pts',(-79.0330513266589,9.90377740689026,-45.6611391413736));
#28952=CARTESIAN_POINT('Ctrl Pts',(-79.0331199231839,9.90554179418347,-46.0412449734119));
#28953=CARTESIAN_POINT('Ctrl Pts',(-79.0332294274041,9.90805317817079,-46.4216226721883));
#28954=CARTESIAN_POINT('Ctrl Pts',(-79.0334393286454,9.91254096860848,-46.9291402371028));
#28955=CARTESIAN_POINT('Ctrl Pts',(-79.0336816691687,9.91733189681885,-47.3099063411295));
#28956=CARTESIAN_POINT('Ctrl Pts',(-79.0339932833495,9.92331761422917,-47.6920768195153));
#28957=CARTESIAN_POINT('Ctrl Pts',(-79.0341735360946,9.92905486580875,-47.9610826353062));
#28958=CARTESIAN_POINT('Ctrl Pts',(-79.0345816125781,9.94535060407697,-48.4859414578514));
#28959=CARTESIAN_POINT('Ctrl Pts',(-79.0354059618012,9.98418172594247,-49.3951141832148));
#28960=CARTESIAN_POINT('Ctrl Pts',(-79.0371418804509,10.0534002757256,-50.6525346836543));
#28961=CARTESIAN_POINT('Ctrl Pts',(-79.0401273111891,10.1136514222037,-52.0997107598098));
#28962=CARTESIAN_POINT('Ctrl Pts',(-79.0422552206141,10.1120993389653,-53.0204920365356));
#28963=CARTESIAN_POINT('Ctrl Pts',(-79.0433045273899,10.0910469989791,-53.5823614484353));
#28964=CARTESIAN_POINT('Ctrl Pts',(-79.0434992845639,10.0797687358586,-53.7813889812428));
#28965=CARTESIAN_POINT('Ctrl Pts',(-79.0438680271245,10.0422770526706,-54.212352393059));
#28966=CARTESIAN_POINT('Ctrl Pts',(-79.0447540348028,9.94210946172304,-54.9970852215659));
#28967=CARTESIAN_POINT('Ctrl Pts',(-79.0490457006217,9.64640250166675,-56.7186062687235));
#28968=CARTESIAN_POINT('Ctrl Pts',(-79.0601766148963,9.39237875326479,-58.4313538319398));
#28969=CARTESIAN_POINT('Ctrl Pts',(-79.059766483128,9.47133330665219,-59.7671833797846));
#28970=CARTESIAN_POINT('Ctrl Pts',(-79.0598456780188,9.48084926379622,-59.9090085149049));
#28971=CARTESIAN_POINT('Ctrl Pts',(-79.0598234432279,9.50446791144338,-60.2030434562208));
#28972=CARTESIAN_POINT('Ctrl Pts',(-79.0596010942571,9.55558462025953,-60.7092328461816));
#28973=CARTESIAN_POINT('Ctrl Pts',(-79.0583387852863,9.69606554450088,-61.7148620605895));
#28974=CARTESIAN_POINT('Ctrl Pts',(-79.0556754227878,9.93263311243084,-62.8348748135968));
#28975=CARTESIAN_POINT('Ctrl Pts',(-79.0526696717474,10.2253808836434,-63.9269816046484));
#28976=CARTESIAN_POINT('Ctrl Pts',(-79.0509784410456,10.407659808702,-64.5298437089376));
#28977=CARTESIAN_POINT('Ctrl Pts',(-79.0499019636937,10.5350891047172,-64.9270005875748));
#28978=CARTESIAN_POINT('Ctrl Pts',(-79.0492009980767,10.6215251528287,-65.190447030245));
#28979=CARTESIAN_POINT('Ctrl Pts',(-79.0485251631571,10.7100790764068,-65.4520343939561));
#28980=CARTESIAN_POINT('Ctrl Pts',(-79.0479683208569,10.789141711712,-65.679125068285));
#28981=CARTESIAN_POINT('Ctrl Pts',(-79.0476607288907,10.8347393551293,-65.8083832714137));
#28982=CARTESIAN_POINT('Ctrl Pts',(-79.0472089442676,10.9035486536729,-66.0017870771877));
#28983=CARTESIAN_POINT('Ctrl Pts',(-79.0468583397703,10.96168030133,-66.1618627778113));
#28984=CARTESIAN_POINT('Ctrl Pts',(-79.0462811031981,11.0590539390145,-66.4261205989256));
#28985=CARTESIAN_POINT('Ctrl Pts',(-79.0439321978173,11.1763724490973,-66.7305525791315));
#28986=CARTESIAN_POINT('Ctrl Pts',(-79.0403369548941,11.4183562660455,-67.3072646266245));
#28987=CARTESIAN_POINT('Ctrl Pts',(-79.0340712069395,11.8774962769686,-68.2955742233012));
#28988=CARTESIAN_POINT('Ctrl Pts',(-79.0255132854485,12.8785149007951,-70.1534980895664));
#28989=CARTESIAN_POINT('Ctrl Pts',(-79.0268467610113,13.7541588492713,-71.6137842113818));
#28990=CARTESIAN_POINT('Ctrl Pts',(-79.0322812395531,14.3082343257534,-72.6661621417369));
#28991=CARTESIAN_POINT('Ctrl Pts',(-79.0318056712663,14.4438933775396,-72.9238448997369));
#28992=CARTESIAN_POINT('Ctrl Pts',(-79.031841873977,14.708725048567,-73.4254194790639));
#28993=CARTESIAN_POINT('Ctrl Pts',(-79.0315212396219,15.043288618854,-74.0571626127364));
#28994=CARTESIAN_POINT('Ctrl Pts',(-79.0314066683176,15.4439701285256,-74.8110570613112));
#28995=CARTESIAN_POINT('Ctrl Pts',(-79.0311527797013,16.2470909827666,-76.3186256623566));
#28996=CARTESIAN_POINT('Ctrl Pts',(-79.0311874647941,16.916487221391,-77.5711817650315));
#28997=CARTESIAN_POINT('Ctrl Pts',(-79.0314527933477,17.8844235621115,-79.3917431634465));
#28998=CARTESIAN_POINT('Ctrl Pts',(-79.0313374840439,18.3217664730177,-80.2144024929943));
#28999=CARTESIAN_POINT('Ctrl Pts',(-79.0313374840529,18.7582880604105,-81.0353801950843));
#29000=CARTESIAN_POINT('Ctrl Pts',(-78.1311770603316,4.8823848963277,24.8296314554803));
#29001=CARTESIAN_POINT('Ctrl Pts',(-78.1317596137954,4.88248902134106,24.7807222946484));
#29002=CARTESIAN_POINT('Ctrl Pts',(-78.132370290488,4.88259794481086,24.7317992370537));
#29003=CARTESIAN_POINT('Ctrl Pts',(-78.13957093287,4.88389587870922,24.1812167240996));
#29004=CARTESIAN_POINT('Ctrl Pts',(-78.1492429359712,4.88177210313678,23.1890789298898));
#29005=CARTESIAN_POINT('Ctrl Pts',(-78.1745369969141,4.87447718530254,21.1752495239669));
#29006=CARTESIAN_POINT('Ctrl Pts',(-78.2220508241846,4.88324527193882,19.6543634614215));
#29007=CARTESIAN_POINT('Ctrl Pts',(-78.3018347246677,4.91934124068949,18.3802224980497));
#29008=CARTESIAN_POINT('Ctrl Pts',(-78.3395077877287,4.93035417118105,17.9047186839576));
#29009=CARTESIAN_POINT('Ctrl Pts',(-78.4321792272901,4.94791278160678,16.9119065362627));
#29010=CARTESIAN_POINT('Ctrl Pts',(-78.62756606031,4.98365609259776,15.1385193686742));
#29011=CARTESIAN_POINT('Ctrl Pts',(-78.8098045608793,5.0898424320682,13.5202511675539));
#29012=CARTESIAN_POINT('Ctrl Pts',(-78.9141089484633,5.30595955448313,12.1229954701847));
#29013=CARTESIAN_POINT('Ctrl Pts',(-78.9585942274942,5.39913458638839,11.5903097961193));
#29014=CARTESIAN_POINT('Ctrl Pts',(-79.0492247135416,5.62075234576258,10.5216532651304));
#29015=CARTESIAN_POINT('Ctrl Pts',(-79.2018299524198,6.08316844415622,8.68166918251728));
#29016=CARTESIAN_POINT('Ctrl Pts',(-79.2830197421236,6.5635056595323,7.13011322696838));
#29017=CARTESIAN_POINT('Ctrl Pts',(-79.2878553005376,6.92316466988806,5.96944845900976));
#29018=CARTESIAN_POINT('Ctrl Pts',(-79.282984356692,7.0138990759062,5.68124408516632));
#29019=CARTESIAN_POINT('Ctrl Pts',(-79.2712479403953,7.2005591058413,5.13353015132918));
#29020=CARTESIAN_POINT('Ctrl Pts',(-79.2395729487823,7.54899370284812,4.18865635750972));
#29021=CARTESIAN_POINT('Ctrl Pts',(-79.1505290853445,8.27795044988715,2.39178151093953));
#29022=CARTESIAN_POINT('Ctrl Pts',(-79.070707980315,8.8246826800187,0.980147970971698));
#29023=CARTESIAN_POINT('Ctrl Pts',(-79.0228189077969,9.05591664951878,0.073019789545241));
#29024=CARTESIAN_POINT('Ctrl Pts',(-79.0149196694937,9.08588467337942,-0.0495288919925896));
#29025=CARTESIAN_POINT('Ctrl Pts',(-78.9990833022964,9.14173945834025,-0.286403911574409));
#29026=CARTESIAN_POINT('Ctrl Pts',(-78.9680083406107,9.23421776089135,-0.704916515177581));
#29027=CARTESIAN_POINT('Ctrl Pts',(-78.9167273956261,9.34909347519021,-1.29979756167584));
#29028=CARTESIAN_POINT('Ctrl Pts',(-78.8452758655552,9.46363978108595,-2.01421880695577));
#29029=CARTESIAN_POINT('Ctrl Pts',(-78.7408117788548,9.5901344998305,-2.96551425791824));
#29030=CARTESIAN_POINT('Ctrl Pts',(-78.5987783229652,9.70979958345411,-4.15435211288435));
#29031=CARTESIAN_POINT('Ctrl Pts',(-78.4950291376993,9.78175376820644,-5.10676453931961));
#29032=CARTESIAN_POINT('Ctrl Pts',(-78.4416371914842,9.82093148750338,-5.70314222326153));
#29033=CARTESIAN_POINT('Ctrl Pts',(-78.4207385059252,9.83260546240869,-5.92375435343461));
#29034=CARTESIAN_POINT('Ctrl Pts',(-78.3787166419865,9.84940723412515,-6.38078537772061));
#29035=CARTESIAN_POINT('Ctrl Pts',(-78.3063535050851,9.86034282260037,-7.18824112077948));
#29036=CARTESIAN_POINT('Ctrl Pts',(-78.2100675688258,9.83680828851061,-8.38360330684038));
#29037=CARTESIAN_POINT('Ctrl Pts',(-78.1312694080627,9.79254174665709,-9.62622235018801));
#29038=CARTESIAN_POINT('Ctrl Pts',(-78.0885083689964,9.7701710701754,-10.5210983780358));
#29039=CARTESIAN_POINT('Ctrl Pts',(-78.0681948463961,9.7628635691047,-11.0392011890184));
#29040=CARTESIAN_POINT('Ctrl Pts',(-78.0594913209939,9.76154320795425,-11.3006542720142));
#29041=CARTESIAN_POINT('Ctrl Pts',(-78.0535143369238,9.76161962452868,-11.4981602742583));
#29042=CARTESIAN_POINT('Ctrl Pts',(-78.0498065810985,9.76166029727339,-11.6217337400378));
#29043=CARTESIAN_POINT('Ctrl Pts',(-78.0435536653433,9.76183376963696,-11.8737775867398));
#29044=CARTESIAN_POINT('Ctrl Pts',(-78.0355242686166,9.76230016272006,-12.3116979655568));
#29045=CARTESIAN_POINT('Ctrl Pts',(-78.0282969034116,9.76406885016096,-13.437552775809));
#29046=CARTESIAN_POINT('Ctrl Pts',(-78.0502938289893,9.76693538421329,-14.6828676178628));
#29047=CARTESIAN_POINT('Ctrl Pts',(-78.0734333686552,9.76987668609478,-15.933933506998));
#29048=CARTESIAN_POINT('Ctrl Pts',(-78.0829759820323,9.77115854627909,-16.5611813088061));
#29049=CARTESIAN_POINT('Ctrl Pts',(-78.0879258747467,9.7719474833457,-17.0647077884012));
#29050=CARTESIAN_POINT('Ctrl Pts',(-78.0892801788362,9.77223811665514,-17.3170550822814));
#29051=CARTESIAN_POINT('Ctrl Pts',(-78.0897800630712,9.77240945302464,-17.5057890556041));
#29052=CARTESIAN_POINT('Ctrl Pts',(-78.0900870788457,9.77251532184126,-17.6302578973462));
#29053=CARTESIAN_POINT('Ctrl Pts',(-78.0906097519498,9.77270161694823,-17.8794826814823));
#29054=CARTESIAN_POINT('Ctrl Pts',(-78.0910083271607,9.77285036145401,-18.128758230635));
#29055=CARTESIAN_POINT('Ctrl Pts',(-78.0912885826298,9.77296663833634,-18.378228578358));
#29056=CARTESIAN_POINT('Ctrl Pts',(-78.091419685695,9.77302624849281,-18.5341964256989));
#29057=CARTESIAN_POINT('Ctrl Pts',(-78.0914988424284,9.77306672386026,-18.6590126744284));
#29058=CARTESIAN_POINT('Ctrl Pts',(-78.0915617440567,9.77310249825838,-18.7838528491809));
#29059=CARTESIAN_POINT('Ctrl Pts',(-78.0916723951705,9.77318196154698,-19.1272582738206));
#29060=CARTESIAN_POINT('Ctrl Pts',(-78.0915289923989,9.77321686059154,-19.689756310114));
#29061=CARTESIAN_POINT('Ctrl Pts',(-78.0906521378086,9.77309075816399,-20.6914139713249));
#29062=CARTESIAN_POINT('Ctrl Pts',(-78.0889259165822,9.77273700661441,-21.9468387332845));
#29063=CARTESIAN_POINT('Ctrl Pts',(-78.0880620482322,9.77256370885544,-22.9550493642093));
#29064=CARTESIAN_POINT('Ctrl Pts',(-78.0880383400088,9.77258901260607,-23.584773435821));
#29065=CARTESIAN_POINT('Ctrl Pts',(-78.0880395768243,9.7726007016267,-23.8339778576478));
#29066=CARTESIAN_POINT('Ctrl Pts',(-78.0880838000811,9.77262872959416,-24.3332133497713));
#29067=CARTESIAN_POINT('Ctrl Pts',(-78.088252906136,9.77268781310717,-25.2086881057995));
#29068=CARTESIAN_POINT('Ctrl Pts',(-78.0886628495693,9.77278573745366,-26.4634121522126));
#29069=CARTESIAN_POINT('Ctrl Pts',(-78.0891059208895,9.77287353184222,-27.971732488491));
#29070=CARTESIAN_POINT('Ctrl Pts',(-78.0891685459406,9.77287523721471,-28.9764534880619));
#29071=CARTESIAN_POINT('Ctrl Pts',(-78.0890765294099,9.772850268981,-29.5406571874715));
#29072=CARTESIAN_POINT('Ctrl Pts',(-78.0890507139456,9.77284358851919,-29.6660260140938));
#29073=CARTESIAN_POINT('Ctrl Pts',(-78.0889803736452,9.77282615857097,-29.916825941177));
#29074=CARTESIAN_POINT('Ctrl Pts',(-78.088811812522,9.77278558263809,-30.3558648188687));
#29075=CARTESIAN_POINT('Ctrl Pts',(-78.0883217064956,9.77267012835526,-31.2343865202128));
#29076=CARTESIAN_POINT('Ctrl Pts',(-78.0875465805831,9.77248607740738,-32.2388423203145));
#29077=CARTESIAN_POINT('Ctrl Pts',(-78.0868248669926,9.77230352837888,-33.2426016030373));
#29078=CARTESIAN_POINT('Ctrl Pts',(-78.0863774008031,9.77218073775463,-33.9947891081215));
#29079=CARTESIAN_POINT('Ctrl Pts',(-78.0860922922939,9.77208530274799,-34.7460433265988));
#29080=CARTESIAN_POINT('Ctrl Pts',(-78.0860550148545,9.77204885682753,-35.2460752767603));
#29081=CARTESIAN_POINT('Ctrl Pts',(-78.0861012732241,9.77203522768628,-35.6217188758795));
#29082=CARTESIAN_POINT('Ctrl Pts',(-78.086156285324,9.77200742994158,-35.8730071688202));
#29083=CARTESIAN_POINT('Ctrl Pts',(-78.0863516097015,9.77189278779233,-36.3752035941687));
#29084=CARTESIAN_POINT('Ctrl Pts',(-78.0868905139398,9.77157418955388,-37.252721497337));
#29085=CARTESIAN_POINT('Ctrl Pts',(-78.0885311437836,9.77079498681596,-39.0048450605797));
#29086=CARTESIAN_POINT('Ctrl Pts',(-78.0901452019584,9.77095530779979,-40.5080843164705));
#29087=CARTESIAN_POINT('Ctrl Pts',(-78.0906952190281,9.77259474634693,-41.641655016873));
#29088=CARTESIAN_POINT('Ctrl Pts',(-78.0907954655095,9.77279710383975,-41.8895200313038));
#29089=CARTESIAN_POINT('Ctrl Pts',(-78.0908911052138,9.77273076278161,-42.2636138212415));
#29090=CARTESIAN_POINT('Ctrl Pts',(-78.0909420739841,9.77239246210273,-42.6381563810303));
#29091=CARTESIAN_POINT('Ctrl Pts',(-78.0909635138741,9.77171257470949,-43.1389446717454));
#29092=CARTESIAN_POINT('Ctrl Pts',(-78.09092742472,9.77068485525827,-43.7668031474549));
#29093=CARTESIAN_POINT('Ctrl Pts',(-78.0908608932792,9.76997472163853,-44.5229517102528));
#29094=CARTESIAN_POINT('Ctrl Pts',(-78.0908498770293,9.77049710604355,-45.1548446000755));
#29095=CARTESIAN_POINT('Ctrl Pts',(-78.0909045527291,9.77200019178347,-45.6611661948043));
#29096=CARTESIAN_POINT('Ctrl Pts',(-78.0909870418411,9.77377081982469,-46.0412644517004));
#29097=CARTESIAN_POINT('Ctrl Pts',(-78.0911203204094,9.77628831072,-46.4216341649118));
#29098=CARTESIAN_POINT('Ctrl Pts',(-78.0913773835638,9.78078426220737,-46.9291405924077));
#29099=CARTESIAN_POINT('Ctrl Pts',(-78.0916751194715,9.78558159104817,-47.309897565456));
#29100=CARTESIAN_POINT('Ctrl Pts',(-78.092059060611,9.79157418755964,-47.6920585341438));
#29101=CARTESIAN_POINT('Ctrl Pts',(-78.0922909438206,9.79731541699787,-47.9610555557877));
#29102=CARTESIAN_POINT('Ctrl Pts',(-78.0928141854849,9.81361750367893,-48.4858996937119));
#29103=CARTESIAN_POINT('Ctrl Pts',(-78.0938702749711,9.85245636632907,-49.3950493909296));
#29104=CARTESIAN_POINT('Ctrl Pts',(-78.0960173981978,9.92168064086134,-50.6524469583706));
#29105=CARTESIAN_POINT('Ctrl Pts',(-78.0996054393462,9.98194546203058,-52.0996113003008));
#29106=CARTESIAN_POINT('Ctrl Pts',(-78.1021972194949,9.98041340611272,-53.0203965476282));
#29107=CARTESIAN_POINT('Ctrl Pts',(-78.103552984138,9.95937932560721,-53.5822721788142));
#29108=CARTESIAN_POINT('Ctrl Pts',(-78.1038796236689,9.9481109296527,-53.7812907141171));
#29109=CARTESIAN_POINT('Ctrl Pts',(-78.1045403781411,9.91063986083384,-54.2122458319189));
#29110=CARTESIAN_POINT('Ctrl Pts',(-78.1059994025237,9.81051140989646,-54.9969674720916));
#29111=CARTESIAN_POINT('Ctrl Pts',(-78.1115865709136,9.51488524279427,-56.7184898916356));
#29112=CARTESIAN_POINT('Ctrl Pts',(-78.1237638739996,9.26090797288462,-58.4312663199397));
#29113=CARTESIAN_POINT('Ctrl Pts',(-78.1237581974326,9.33988986088882,-59.7671397332803));
#29114=CARTESIAN_POINT('Ctrl Pts',(-78.1238844942955,9.34940969623997,-59.9089694744354));
#29115=CARTESIAN_POINT('Ctrl Pts',(-78.1239493445652,9.373035887766,-60.2030134747147));
#29116=CARTESIAN_POINT('Ctrl Pts',(-78.1238612804463,9.42416601746271,-60.7092172675734));
#29117=CARTESIAN_POINT('Ctrl Pts',(-78.1228017468007,9.5646735653548,-61.7148701901171));
#29118=CARTESIAN_POINT('Ctrl Pts',(-78.1202496321837,9.80126907269193,-62.8348983317338));
#29119=CARTESIAN_POINT('Ctrl Pts',(-78.1172942048821,10.0940392374588,-63.9270100056403));
#29120=CARTESIAN_POINT('Ctrl Pts',(-78.1156194824633,10.2763284006957,-64.5298711124851));
#29121=CARTESIAN_POINT('Ctrl Pts',(-78.1145537042295,10.4037633690798,-64.9270258410423));
#29122=CARTESIAN_POINT('Ctrl Pts',(-78.1138600882166,10.4902028980212,-65.1904704483085));
#29123=CARTESIAN_POINT('Ctrl Pts',(-78.1131924031274,10.5787598112662,-65.4520554048202));
#29124=CARTESIAN_POINT('Ctrl Pts',(-78.11264417627,10.6578246392337,-65.6791434485292));
#29125=CARTESIAN_POINT('Ctrl Pts',(-78.1123420474851,10.7034234087329,-65.8084000006324));
#29126=CARTESIAN_POINT('Ctrl Pts',(-78.1118990542037,10.7722342721755,-66.0018011861481));
#29127=CARTESIAN_POINT('Ctrl Pts',(-78.1115571420184,10.830366944376,-66.1618743867873));
#29128=CARTESIAN_POINT('Ctrl Pts',(-78.1109967335477,10.9277419669287,-66.4261277626537));
#29129=CARTESIAN_POINT('Ctrl Pts',(-78.1086634949448,11.0450638269318,-66.7305607142113));
#29130=CARTESIAN_POINT('Ctrl Pts',(-78.1050916349302,11.2870517329945,-67.3072716081194));
#29131=CARTESIAN_POINT('Ctrl Pts',(-78.0988486279178,11.7461964110975,-68.2955809227801));
#29132=CARTESIAN_POINT('Ctrl Pts',(-78.0902789114672,12.7472140896651,-70.153503416737));
#29133=CARTESIAN_POINT('Ctrl Pts',(-78.0915604899259,13.6228503189759,-71.6137900378666));
#29134=CARTESIAN_POINT('Ctrl Pts',(-78.0969926351875,14.1769257016773,-72.6661684679193));
#29135=CARTESIAN_POINT('Ctrl Pts',(-78.0965172414921,14.312584819131,-72.9238511155437));
#29136=CARTESIAN_POINT('Ctrl Pts',(-78.0965534003352,14.5774165362549,-73.4254256092325));
#29137=CARTESIAN_POINT('Ctrl Pts',(-78.0962328851151,14.9119801351456,-74.0571686215522));
#29138=CARTESIAN_POINT('Ctrl Pts',(-78.0961183673416,15.3126616085308,-74.8110629718493));
#29139=CARTESIAN_POINT('Ctrl Pts',(-78.0958646287455,16.1157823228879,-76.3186314304018));
#29140=CARTESIAN_POINT('Ctrl Pts',(-78.0958993832867,16.7851783804717,-77.5711876354937));
#29141=CARTESIAN_POINT('Ctrl Pts',(-78.0961645973801,17.7531148016156,-79.3917492952415));
#29142=CARTESIAN_POINT('Ctrl Pts',(-78.0960493444548,18.1904576864469,-80.2144085738812));
#29143=CARTESIAN_POINT('Ctrl Pts',(-78.0960493444647,18.626979273838,-81.0353862759772));
#29144=CARTESIAN_POINT('Ctrl Pts',(-76.2590042273726,4.61859600327472,24.8393189079396));
#29145=CARTESIAN_POINT('Ctrl Pts',(-76.2592681779219,4.61842447839424,24.7907142206875));
#29146=CARTESIAN_POINT('Ctrl Pts',(-76.2595448957426,4.61824498946315,24.7421095860943));
#29147=CARTESIAN_POINT('Ctrl Pts',(-76.2628180829915,4.61612282665744,24.1948927869701));
#29148=CARTESIAN_POINT('Ctrl Pts',(-76.2639562409209,4.60859831660333,23.1986363414545));
#29149=CARTESIAN_POINT('Ctrl Pts',(-76.2656140569439,4.58719755532069,21.1946693625333));
#29150=CARTESIAN_POINT('Ctrl Pts',(-76.2875114488552,4.57291627906073,19.688273194824));
#29151=CARTESIAN_POINT('Ctrl Pts',(-76.3407775511093,4.57211762926454,18.4315980029145));
#29152=CARTESIAN_POINT('Ctrl Pts',(-76.364795847461,4.56784519050253,17.9582353576507));
#29153=CARTESIAN_POINT('Ctrl Pts',(-76.4225713932389,4.54820072480068,16.9721940539584));
#29154=CARTESIAN_POINT('Ctrl Pts',(-76.5461514281704,4.50383717090078,15.2086150227548));
#29155=CARTESIAN_POINT('Ctrl Pts',(-76.6816334750586,4.51394771962339,13.6041032982031));
#29156=CARTESIAN_POINT('Ctrl Pts',(-76.7973140293964,4.6407009319777,12.217831420693));
#29157=CARTESIAN_POINT('Ctrl Pts',(-76.8482852102344,4.69590094579638,11.6963573236253));
#29158=CARTESIAN_POINT('Ctrl Pts',(-76.9619015909896,4.83491484815665,10.6384382958421));
#29159=CARTESIAN_POINT('Ctrl Pts',(-77.1773119360269,5.14739349753966,8.80323245732017));
#29160=CARTESIAN_POINT('Ctrl Pts',(-77.3359788946946,5.52637907226672,7.23241034151302));
#29161=CARTESIAN_POINT('Ctrl Pts',(-77.3978387797282,5.84607073042359,6.05183159679405));
#29162=CARTESIAN_POINT('Ctrl Pts',(-77.4104442325175,5.92294187553072,5.77136070217919));
#29163=CARTESIAN_POINT('Ctrl Pts',(-77.4347135540794,6.08613441821857,5.22885965815191));
#29164=CARTESIAN_POINT('Ctrl Pts',(-77.4719372792818,6.39735474942925,4.29054300823768));
#29165=CARTESIAN_POINT('Ctrl Pts',(-77.5145028871782,7.08180232375017,2.48801694228043));
#29166=CARTESIAN_POINT('Ctrl Pts',(-77.4910547207249,7.65143594580301,1.04581578691076));
#29167=CARTESIAN_POINT('Ctrl Pts',(-77.4563842398442,7.93937105777638,0.058709180579072));
#29168=CARTESIAN_POINT('Ctrl Pts',(-77.4493290402009,7.97629023793011,-0.0741410539284971));
#29169=CARTESIAN_POINT('Ctrl Pts',(-77.4352767501426,8.04762452283956,-0.330701773943114));
#29170=CARTESIAN_POINT('Ctrl Pts',(-77.4064452562596,8.1709111311268,-0.782749843811338));
#29171=CARTESIAN_POINT('Ctrl Pts',(-77.3563225287767,8.3397651769347,-1.42166221717552));
#29172=CARTESIAN_POINT('Ctrl Pts',(-77.2826938433032,8.53037197955925,-2.1802328912742));
#29173=CARTESIAN_POINT('Ctrl Pts',(-77.1698668107121,8.76522842254609,-3.17513515057689));
#29174=CARTESIAN_POINT('Ctrl Pts',(-77.0078569636857,9.01658055161386,-4.38307664684124));
#29175=CARTESIAN_POINT('Ctrl Pts',(-76.8810657628304,9.16472129690078,-5.30418238519797));
#29176=CARTESIAN_POINT('Ctrl Pts',(-76.8143618657502,9.23977927721158,-5.86669715931559));
#29177=CARTESIAN_POINT('Ctrl Pts',(-76.787607335228,9.26692705674221,-6.0982486037313));
#29178=CARTESIAN_POINT('Ctrl Pts',(-76.7305226862092,9.31381581727877,-6.56031291945888));
#29179=CARTESIAN_POINT('Ctrl Pts',(-76.6238236505912,9.37791596242654,-7.37656475134554));
#29180=CARTESIAN_POINT('Ctrl Pts',(-76.4588581176365,9.43436852869042,-8.55885890551735));
#29181=CARTESIAN_POINT('Ctrl Pts',(-76.3083560520247,9.47478587372195,-9.77012430061687));
#29182=CARTESIAN_POINT('Ctrl Pts',(-76.2268873631626,9.5027481596305,-10.6328071100525));
#29183=CARTESIAN_POINT('Ctrl Pts',(-76.1889655386322,9.51944302308452,-11.1295121211793));
#29184=CARTESIAN_POINT('Ctrl Pts',(-76.1732056728746,9.52823085883001,-11.3791648455793));
#29185=CARTESIAN_POINT('Ctrl Pts',(-76.1626504799191,9.5350719083413,-11.5673289815983));
#29186=CARTESIAN_POINT('Ctrl Pts',(-76.1561052967098,9.53898042037542,-11.6835151432893));
#29187=CARTESIAN_POINT('Ctrl Pts',(-76.144917308345,9.54587543167022,-11.9221807076453));
#29188=CARTESIAN_POINT('Ctrl Pts',(-76.13015184916,9.55494455746776,-12.3381370441309));
#29189=CARTESIAN_POINT('Ctrl Pts',(-76.1141485418874,9.5648471517035,-13.4170096797781));
#29190=CARTESIAN_POINT('Ctrl Pts',(-76.1462425759041,9.54491458592689,-14.6383048247315));
#29191=CARTESIAN_POINT('Ctrl Pts',(-76.1814626115458,9.52362292145339,-15.8942208802503));
#29192=CARTESIAN_POINT('Ctrl Pts',(-76.1958857385209,9.51493327790932,-16.5310031582579));
#29193=CARTESIAN_POINT('Ctrl Pts',(-76.2032145185471,9.51049482727055,-17.0463829734709));
#29194=CARTESIAN_POINT('Ctrl Pts',(-76.205081939314,9.50932336185469,-17.3060972556637));
#29195=CARTESIAN_POINT('Ctrl Pts',(-76.2056636418833,9.50892238711838,-17.5007252514251));
#29196=CARTESIAN_POINT('Ctrl Pts',(-76.2060215327765,9.50866985368353,-17.6246102520673));
#29197=CARTESIAN_POINT('Ctrl Pts',(-76.2066358525459,9.50821590728096,-17.8752338247666));
#29198=CARTESIAN_POINT('Ctrl Pts',(-76.2071030890251,9.50783307899538,-18.1248776552823));
#29199=CARTESIAN_POINT('Ctrl Pts',(-76.2074424999087,9.50751558146185,-18.3751638083415));
#29200=CARTESIAN_POINT('Ctrl Pts',(-76.2076034773988,9.50734240481563,-18.5315011597223));
#29201=CARTESIAN_POINT('Ctrl Pts',(-76.20770398336,9.50721831212379,-18.6566403311446));
#29202=CARTESIAN_POINT('Ctrl Pts',(-76.2077861285719,9.50710348714328,-18.781780869533));
#29203=CARTESIAN_POINT('Ctrl Pts',(-76.2079378679436,9.50682437559786,-19.1259787747093));
#29204=CARTESIAN_POINT('Ctrl Pts',(-76.2078153736874,9.50655555146275,-19.6895413001364));
#29205=CARTESIAN_POINT('Ctrl Pts',(-76.2068710997451,9.50646064275388,-20.6924449732618));
#29206=CARTESIAN_POINT('Ctrl Pts',(-76.2049542636278,9.50677431622997,-21.9482338168688));
#29207=CARTESIAN_POINT('Ctrl Pts',(-76.2039576717217,9.50690444115847,-22.9554522656082));
#29208=CARTESIAN_POINT('Ctrl Pts',(-76.2039275481492,9.50676784822903,-23.584208861743));
#29209=CARTESIAN_POINT('Ctrl Pts',(-76.2039300299676,9.50671629310398,-23.8335354558114));
#29210=CARTESIAN_POINT('Ctrl Pts',(-76.2039812982234,9.50662403516601,-24.3327382201223));
#29211=CARTESIAN_POINT('Ctrl Pts',(-76.2041739461635,9.50648909669583,-25.2083157606351));
#29212=CARTESIAN_POINT('Ctrl Pts',(-76.2046250598341,9.50636536455388,-26.4631392496011));
#29213=CARTESIAN_POINT('Ctrl Pts',(-76.2050816179087,9.50631559527858,-27.9716990325924));
#29214=CARTESIAN_POINT('Ctrl Pts',(-76.2050810711752,9.50634384078493,-28.9766011891009));
#29215=CARTESIAN_POINT('Ctrl Pts',(-76.2049293321848,9.50637549694148,-29.5409280424476));
#29216=CARTESIAN_POINT('Ctrl Pts',(-76.2048890852193,9.50638340512734,-29.6663460964825));
#29217=CARTESIAN_POINT('Ctrl Pts',(-76.2047833071876,9.50640205542425,-29.9172266777127));
#29218=CARTESIAN_POINT('Ctrl Pts',(-76.2045369353503,9.50644212052786,-30.3564002919477));
#29219=CARTESIAN_POINT('Ctrl Pts',(-76.2038391993363,9.50654997929938,-31.2351354934128));
#29220=CARTESIAN_POINT('Ctrl Pts',(-76.2027556621548,9.50672807600084,-32.2397232658103));
#29221=CARTESIAN_POINT('Ctrl Pts',(-76.2017504713315,9.50694345656999,-33.2434999211817));
#29222=CARTESIAN_POINT('Ctrl Pts',(-76.2011267950556,9.50711892763534,-33.9956442736657));
#29223=CARTESIAN_POINT('Ctrl Pts',(-76.2007236174732,9.50730363354043,-34.7467985689858));
#29224=CARTESIAN_POINT('Ctrl Pts',(-76.2006625756323,9.50742961952989,-35.2467251488447));
#29225=CARTESIAN_POINT('Ctrl Pts',(-76.2007175157305,9.50752450792639,-35.6222768028191));
#29226=CARTESIAN_POINT('Ctrl Pts',(-76.2007869898762,9.50756951397982,-35.8735693745529));
#29227=CARTESIAN_POINT('Ctrl Pts',(-76.2010421551002,9.50760093948215,-36.3757368169703));
#29228=CARTESIAN_POINT('Ctrl Pts',(-76.2017564177825,9.50753643027774,-37.2532219117906));
#29229=CARTESIAN_POINT('Ctrl Pts',(-76.2039537667349,9.50725174813394,-39.0052625360082));
#29230=CARTESIAN_POINT('Ctrl Pts',(-76.2061267775844,9.50776518387426,-40.5084306038123));
#29231=CARTESIAN_POINT('Ctrl Pts',(-76.2068678449123,9.50959628166372,-41.6419436757499));
#29232=CARTESIAN_POINT('Ctrl Pts',(-76.2070030478336,9.50983925074399,-41.8898029062589));
#29233=CARTESIAN_POINT('Ctrl Pts',(-76.2071324330694,9.50982923114487,-42.2638831022705));
#29234=CARTESIAN_POINT('Ctrl Pts',(-76.207201903782,9.50954278151185,-42.6384119642511));
#29235=CARTESIAN_POINT('Ctrl Pts',(-76.2072321498816,9.50892629007431,-43.1391794608419));
#29236=CARTESIAN_POINT('Ctrl Pts',(-76.2071857905377,9.50796757481491,-43.7670087702537));
#29237=CARTESIAN_POINT('Ctrl Pts',(-76.2070998926126,9.50732523819983,-44.5231165636665));
#29238=CARTESIAN_POINT('Ctrl Pts',(-76.2070893748377,9.50789273229008,-45.1549708187902));
#29239=CARTESIAN_POINT('Ctrl Pts',(-76.2071679695818,9.50942615111586,-45.661258620098));
#29240=CARTESIAN_POINT('Ctrl Pts',(-76.2072835240516,9.51121663437992,-46.0413300661524));
#29241=CARTESIAN_POINT('Ctrl Pts',(-76.2074683755412,9.5137512927683,-46.4216714909197));
#29242=CARTESIAN_POINT('Ctrl Pts',(-76.2078233899365,9.51826680586861,-46.9291382069745));
#29243=CARTESIAN_POINT('Ctrl Pts',(-76.2082324872451,9.52307518220736,-47.3098630957302));
#29244=CARTESIAN_POINT('Ctrl Pts',(-76.2087601881983,9.52907686736878,-47.6919901090945));
#29245=CARTESIAN_POINT('Ctrl Pts',(-76.2090940373854,9.53482117044283,-47.9609548438845));
#29246=CARTESIAN_POINT('Ctrl Pts',(-76.2098426948961,9.55112122915765,-48.4857456976199));
#29247=CARTESIAN_POINT('Ctrl Pts',(-76.2113481950911,9.58993737722253,-49.3948125759944));
#29248=CARTESIAN_POINT('Ctrl Pts',(-76.2142847700669,9.65909517046485,-50.6521313604828));
#29249=CARTESIAN_POINT('Ctrl Pts',(-76.2190279326259,9.71927703522356,-52.0992603167427));
#29250=CARTESIAN_POINT('Ctrl Pts',(-76.2225103933654,9.7177164037998,-53.0200657704971));
#29251=CARTESIAN_POINT('Ctrl Pts',(-76.2244565286584,9.69667881139509,-53.5819669884308));
#29252=CARTESIAN_POINT('Ctrl Pts',(-76.2250365305548,9.68541555942535,-53.7809570880999));
#29253=CARTESIAN_POINT('Ctrl Pts',(-76.2262583643598,9.64795122297238,-54.2118867929367));
#29254=CARTESIAN_POINT('Ctrl Pts',(-76.2288182517556,9.54783231147705,-54.9965727500687));
#29255=CARTESIAN_POINT('Ctrl Pts',(-76.2368998477477,9.25220215107105,-56.7180955616072));
#29256=CARTESIAN_POINT('Ctrl Pts',(-76.2511002172696,8.99816735527023,-58.4309623918978));
#29257=CARTESIAN_POINT('Ctrl Pts',(-76.25188003066,9.07715834511537,-59.7669855301454));
#29258=CARTESIAN_POINT('Ctrl Pts',(-76.2520979227219,9.08668132659362,-59.9088313263526));
#29259=CARTESIAN_POINT('Ctrl Pts',(-76.2523324143239,9.11031486210005,-60.2029067217604));
#29260=CARTESIAN_POINT('Ctrl Pts',(-76.252506727489,9.16146287136278,-60.7091604595888));
#29261=CARTESIAN_POINT('Ctrl Pts',(-76.2518467397678,9.30202067976079,-61.7148952707414));
#29262=CARTESIAN_POINT('Ctrl Pts',(-76.2495214391804,9.53869245490255,-62.8349751129574));
#29263=CARTESIAN_POINT('Ctrl Pts',(-76.2466756002566,9.83153216625402,-63.927101247565));
#29264=CARTESIAN_POINT('Ctrl Pts',(-76.2450394130943,10.0138543095137,-64.5299574543569));
#29265=CARTESIAN_POINT('Ctrl Pts',(-76.243998371472,10.1413072002774,-64.9271037524503));
#29266=CARTESIAN_POINT('Ctrl Pts',(-76.2433215730166,10.2277575008871,-65.1905413693236));
#29267=CARTESIAN_POINT('Ctrl Pts',(-76.2426720314166,10.3163233362897,-65.4521173384831));
#29268=CARTESIAN_POINT('Ctrl Pts',(-76.2421423804406,10.3953940639647,-65.6791957451958));
#29269=CARTESIAN_POINT('Ctrl Pts',(-76.2418518498307,10.4409956334978,-65.8084462860989));
#29270=CARTESIAN_POINT('Ctrl Pts',(-76.2414273462054,10.5098101142562,-66.0018379677946));
#29271=CARTESIAN_POINT('Ctrl Pts',(-76.2411033296708,10.5679445458857,-66.1619021679868));
#29272=CARTESIAN_POINT('Ctrl Pts',(-76.2405770538302,10.6653207752972,-66.4261396223808));
#29273=CARTESIAN_POINT('Ctrl Pts',(-76.238274380634,10.7826504114359,-66.7305752876175));
#29274=CARTESIAN_POINT('Ctrl Pts',(-76.2347483816778,11.0246467256038,-67.3072812057032));
#29275=CARTESIAN_POINT('Ctrl Pts',(-76.2285488107215,11.4838013522539,-68.2955882718413));
#29276=CARTESIAN_POINT('Ctrl Pts',(-76.2199525136906,12.484816163397,-70.153505038466));
#29277=CARTESIAN_POINT('Ctrl Pts',(-76.2211307523171,13.3604372158861,-71.6137934851493));
#29278=CARTESIAN_POINT('Ctrl Pts',(-76.2265609927081,13.914514542038,-72.6661742394984));
#29279=CARTESIAN_POINT('Ctrl Pts',(-76.2260858005073,14.0501737272878,-72.9238564325828));
#29280=CARTESIAN_POINT('Ctrl Pts',(-76.2261219886509,14.315005652721,-73.4254306124565));
#29281=CARTESIAN_POINT('Ctrl Pts',(-76.2258016137887,14.6495692888486,-74.0571731456247));
#29282=CARTESIAN_POINT('Ctrl Pts',(-76.2256871554553,15.0502506125563,-74.8110671326668));
#29283=CARTESIAN_POINT('Ctrl Pts',(-76.2254335074589,15.8533707573767,-76.3186350678062));
#29284=CARTESIAN_POINT('Ctrl Pts',(-76.2254681352656,16.5227663100739,-77.5711916489216));
#29285=CARTESIAN_POINT('Ctrl Pts',(-76.2257331671865,17.4907032123627,-79.3917542521962));
#29286=CARTESIAN_POINT('Ctrl Pts',(-76.2256179522378,17.9280460112828,-80.2144133326538));
#29287=CARTESIAN_POINT('Ctrl Pts',(-76.2256179522404,18.3645675986696,-81.0353910347614));
#29288=CARTESIAN_POINT('Ctrl Pts',(-73.4534503626178,4.22530732157714,24.8335657884132));
#29289=CARTESIAN_POINT('Ctrl Pts',(-73.4535264544043,4.22524571942005,24.7847806310169));
#29290=CARTESIAN_POINT('Ctrl Pts',(-73.4536065022151,4.22518103548679,24.7359973542828));
#29291=CARTESIAN_POINT('Ctrl Pts',(-73.4545515468872,4.22442734723246,24.1865265021468));
#29292=CARTESIAN_POINT('Ctrl Pts',(-73.4518396848519,4.22214509836896,23.1833993556362));
#29293=CARTESIAN_POINT('Ctrl Pts',(-73.4432875794321,4.21564386815076,21.1771447988208));
#29294=CARTESIAN_POINT('Ctrl Pts',(-73.4496482516278,4.21095932290573,19.6752901912072));
#29295=CARTESIAN_POINT('Ctrl Pts',(-73.480366066804,4.20940202828548,18.4259537128077));
#29296=CARTESIAN_POINT('Ctrl Pts',(-73.4934057763347,4.20716972644692,17.9326902717968));
#29297=CARTESIAN_POINT('Ctrl Pts',(-73.5231642093913,4.19898916407945,16.9350263710404));
#29298=CARTESIAN_POINT('Ctrl Pts',(-73.5876243829913,4.1820002035377,15.1776787075357));
#29299=CARTESIAN_POINT('Ctrl Pts',(-73.6730050953354,4.18371648075477,13.6462338534787));
#29300=CARTESIAN_POINT('Ctrl Pts',(-73.770746955575,4.21638770933198,12.3551078553633));
#29301=CARTESIAN_POINT('Ctrl Pts',(-73.8141207398876,4.22931004378227,11.8605695054897));
#29302=CARTESIAN_POINT('Ctrl Pts',(-73.914564301458,4.25858480531431,10.8516404283782));
#29303=CARTESIAN_POINT('Ctrl Pts',(-74.1168742425506,4.32647223867873,9.07410082103936));
#29304=CARTESIAN_POINT('Ctrl Pts',(-74.3029354570517,4.44250222456322,7.50899014168587));
#29305=CARTESIAN_POINT('Ctrl Pts',(-74.4141498819098,4.58646403629438,6.31642002121918));
#29306=CARTESIAN_POINT('Ctrl Pts',(-74.4407921161309,4.61616424599026,6.06973783334977));
#29307=CARTESIAN_POINT('Ctrl Pts',(-74.4971526282043,4.68062536381783,5.56172614019332));
#29308=CARTESIAN_POINT('Ctrl Pts',(-74.6016775943766,4.80347816750837,4.66722272176758));
#29309=CARTESIAN_POINT('Ctrl Pts',(-74.8082980429265,5.10837144424391,2.83336893354753));
#29310=CARTESIAN_POINT('Ctrl Pts',(-74.8896400752098,5.48503136133549,1.22545544900277));
#29311=CARTESIAN_POINT('Ctrl Pts',(-74.8560557702692,5.79782244142089,0.0737981143452186));
#29312=CARTESIAN_POINT('Ctrl Pts',(-74.8501359070869,5.83828255520455,-0.0741007103992069));
#29313=CARTESIAN_POINT('Ctrl Pts',(-74.8368000578546,5.9210901625713,-0.360514162164227));
#29314=CARTESIAN_POINT('Ctrl Pts',(-74.8077814370417,6.07422021650526,-0.857581343451014));
#29315=CARTESIAN_POINT('Ctrl Pts',(-74.7543904219924,6.30982751967589,-1.54628406476854));
#29316=CARTESIAN_POINT('Ctrl Pts',(-74.679453194965,6.60760255077807,-2.34684941248347));
#29317=CARTESIAN_POINT('Ctrl Pts',(-74.573252692236,7.00990006796143,-3.38247221632282));
#29318=CARTESIAN_POINT('Ctrl Pts',(-74.4409550234082,7.49588827955719,-4.62234798923736));
#29319=CARTESIAN_POINT('Ctrl Pts',(-74.3475267879606,7.80738658039865,-5.54684366132469));
#29320=CARTESIAN_POINT('Ctrl Pts',(-74.2938158486148,7.96133936928322,-6.09887709999131));
#29321=CARTESIAN_POINT('Ctrl Pts',(-74.2647795208492,8.03246017297698,-6.36322142372142));
#29322=CARTESIAN_POINT('Ctrl Pts',(-74.204142684526,8.16462655538642,-6.86450096167411));
#29323=CARTESIAN_POINT('Ctrl Pts',(-74.0823125138115,8.38762892071749,-7.74660662064083));
#29324=CARTESIAN_POINT('Ctrl Pts',(-73.8765358143582,8.67004701957717,-8.96897404996482));
#29325=CARTESIAN_POINT('Ctrl Pts',(-73.6612700003148,8.90659532438443,-10.1368517690802));
#29326=CARTESIAN_POINT('Ctrl Pts',(-73.536969782202,9.04056414474881,-10.9203308539594));
#29327=CARTESIAN_POINT('Ctrl Pts',(-73.4783977708949,9.10574841489709,-11.3597552080612));
#29328=CARTESIAN_POINT('Ctrl Pts',(-73.4540544265507,9.13408310685853,-11.5766197293273));
#29329=CARTESIAN_POINT('Ctrl Pts',(-73.4378784149944,9.15358518982697,-11.7387516496819));
#29330=CARTESIAN_POINT('Ctrl Pts',(-73.4277303903028,9.16489463380208,-11.8419689709694));
#29331=CARTESIAN_POINT('Ctrl Pts',(-73.4094360385693,9.18538739815458,-12.0534230548263));
#29332=CARTESIAN_POINT('Ctrl Pts',(-73.3828123696777,9.21382618350268,-12.4260876551212));
#29333=CARTESIAN_POINT('Ctrl Pts',(-73.3396234882099,9.25366459642119,-13.4097636359682));
#29334=CARTESIAN_POINT('Ctrl Pts',(-73.3513981969414,9.21041323300678,-14.5798442111602));
#29335=CARTESIAN_POINT('Ctrl Pts',(-73.3724414765133,9.15254517746251,-15.8391606330428));
#29336=CARTESIAN_POINT('Ctrl Pts',(-73.3809203128667,9.12816037948757,-16.4913836601658));
#29337=CARTESIAN_POINT('Ctrl Pts',(-73.3838080244589,9.11594801097321,-17.0271640927407));
#29338=CARTESIAN_POINT('Ctrl Pts',(-73.3834874083303,9.1132209118,-17.299854671422));
#29339=CARTESIAN_POINT('Ctrl Pts',(-73.382418156735,9.11276418517905,-17.5049038677841));
#29340=CARTESIAN_POINT('Ctrl Pts',(-73.3817366061404,9.11251885643354,-17.6264660402337));
#29341=CARTESIAN_POINT('Ctrl Pts',(-73.3805006647101,9.11203801180432,-17.8778403861542));
#29342=CARTESIAN_POINT('Ctrl Pts',(-73.3794378907323,9.11162404567047,-18.1262672036762));
#29343=CARTESIAN_POINT('Ctrl Pts',(-73.3785363964569,9.11125305690329,-18.3764169410916));
#29344=CARTESIAN_POINT('Ctrl Pts',(-73.3780354933547,9.1110426695193,-18.5324456069998));
#29345=CARTESIAN_POINT('Ctrl Pts',(-73.3776706912338,9.11088503822815,-18.6574338010098));
#29346=CARTESIAN_POINT('Ctrl Pts',(-73.3773289910963,9.11073495961537,-18.7824033715676));
#29347=CARTESIAN_POINT('Ctrl Pts',(-73.3764811288779,9.11035186572385,-19.1261708202472));
#29348=CARTESIAN_POINT('Ctrl Pts',(-73.3755667743369,9.10987842611151,-19.6891481817991));
#29349=CARTESIAN_POINT('Ctrl Pts',(-73.3749290409688,9.10936330232155,-20.6913688187418));
#29350=CARTESIAN_POINT('Ctrl Pts',(-73.3753285425777,9.10914109344479,-21.9470230877658));
#29351=CARTESIAN_POINT('Ctrl Pts',(-73.3754911264308,9.1089481309495,-22.9548469969399));
#29352=CARTESIAN_POINT('Ctrl Pts',(-73.3750955098072,9.10868038336673,-23.5842034053044));
#29353=CARTESIAN_POINT('Ctrl Pts',(-73.3749590412318,9.10857862176442,-23.8334635528237));
#29354=CARTESIAN_POINT('Ctrl Pts',(-73.3747576605167,9.10838989357654,-24.3327079378256));
#29355=CARTESIAN_POINT('Ctrl Pts',(-73.3745712186291,9.10809920532248,-25.2082707662882));
#29356=CARTESIAN_POINT('Ctrl Pts',(-73.3746578913938,9.10781325001986,-26.4631303759716));
#29357=CARTESIAN_POINT('Ctrl Pts',(-73.3749594298408,9.1076815981057,-27.9717572086069));
#29358=CARTESIAN_POINT('Ctrl Pts',(-73.3750307630492,9.10775043370461,-28.9767346163479));
#29359=CARTESIAN_POINT('Ctrl Pts',(-73.3749624986682,9.10782891690429,-29.5411160077894));
#29360=CARTESIAN_POINT('Ctrl Pts',(-73.3749426806809,9.10784793838067,-29.6665553412422));
#29361=CARTESIAN_POINT('Ctrl Pts',(-73.3748857815024,9.10789385649037,-29.917471271486));
#29362=CARTESIAN_POINT('Ctrl Pts',(-73.374745037268,9.10799489240151,-30.3567031022437));
#29363=CARTESIAN_POINT('Ctrl Pts',(-73.3743338055719,9.10826809090815,-31.2355308044657));
#29364=CARTESIAN_POINT('Ctrl Pts',(-73.373725112351,9.1087165407114,-32.2401731925551));
#29365=CARTESIAN_POINT('Ctrl Pts',(-73.3732937113373,9.1092241789564,-33.2439555370028));
#29366=CARTESIAN_POINT('Ctrl Pts',(-73.3731380822152,9.10961721873692,-33.9960806734612));
#29367=CARTESIAN_POINT('Ctrl Pts',(-73.373228976467,9.11001401755442,-34.7471878425551));
#29368=CARTESIAN_POINT('Ctrl Pts',(-73.3735069059235,9.11026772494588,-35.2470654367572));
#29369=CARTESIAN_POINT('Ctrl Pts',(-73.3738173886319,9.11044931268916,-35.6225752381303));
#29370=CARTESIAN_POINT('Ctrl Pts',(-73.3740685305789,9.11055357666728,-35.8738693081829));
#29371=CARTESIAN_POINT('Ctrl Pts',(-73.374722824881,9.11070510342909,-36.3760234464305));
#29372=CARTESIAN_POINT('Ctrl Pts',(-73.3762152519728,9.11086472772307,-37.2534889948367));
#29373=CARTESIAN_POINT('Ctrl Pts',(-73.3801684951591,9.11102366189834,-39.0054883315695));
#29374=CARTESIAN_POINT('Ctrl Pts',(-73.3837862952099,9.11189706598561,-40.5086064003644));
#29375=CARTESIAN_POINT('Ctrl Pts',(-73.3851750408898,9.11390494751553,-41.6420878899218));
#29376=CARTESIAN_POINT('Ctrl Pts',(-73.3854407772297,9.11418248909649,-41.8899452427818));
#29377=CARTESIAN_POINT('Ctrl Pts',(-73.385733110362,9.11421968779635,-42.2640193550185));
#29378=CARTESIAN_POINT('Ctrl Pts',(-73.3859371191632,9.11397489948023,-42.6385422942363));
#29379=CARTESIAN_POINT('Ctrl Pts',(-73.3861147834151,9.11340819415011,-43.1393000783977));
#29380=CARTESIAN_POINT('Ctrl Pts',(-73.3862039006377,9.11250144203186,-43.7671153050967));
#29381=CARTESIAN_POINT('Ctrl Pts',(-73.3862380108539,9.1119094287437,-44.5232019750015));
#29382=CARTESIAN_POINT('Ctrl Pts',(-73.3863216238271,9.11251236292798,-45.1550347080314));
#29383=CARTESIAN_POINT('Ctrl Pts',(-73.3864899830379,9.11407079904804,-45.6613051540447));
#29384=CARTESIAN_POINT('Ctrl Pts',(-73.3866844229875,9.11587953351574,-46.0413623597674));
#29385=CARTESIAN_POINT('Ctrl Pts',(-73.3869641726572,9.11843226101216,-46.4216884857227));
#29386=CARTESIAN_POINT('Ctrl Pts',(-73.3874731185593,9.12297234782612,-46.929134069437));
#29387=CARTESIAN_POINT('Ctrl Pts',(-73.3880347312395,9.12780023573987,-47.3098400721596));
#29388=CARTESIAN_POINT('Ctrl Pts',(-73.3887494498632,9.13382343347493,-47.6919484285281));
#29389=CARTESIAN_POINT('Ctrl Pts',(-73.3892094710157,9.13958046724949,-47.9608936712186));
#29390=CARTESIAN_POINT('Ctrl Pts',(-73.3902174338838,9.15590174806547,-48.4856540481513));
#29391=CARTESIAN_POINT('Ctrl Pts',(-73.3921986559709,9.19474692453655,-49.3946750318828));
#29392=CARTESIAN_POINT('Ctrl Pts',(-73.3959037699135,9.26393051387892,-50.6519564944643));
#29393=CARTESIAN_POINT('Ctrl Pts',(-73.4017847293707,9.32416468844298,-52.0990813594302));
#29394=CARTESIAN_POINT('Ctrl Pts',(-73.4062151490616,9.32266230323621,-53.0199070893121));
#29395=CARTESIAN_POINT('Ctrl Pts',(-73.4088284950924,9.30167781654893,-53.5818275823233));
#29396=CARTESIAN_POINT('Ctrl Pts',(-73.4096944558121,9.29044001726773,-53.7808119396728));
#29397=CARTESIAN_POINT('Ctrl Pts',(-73.4115556097283,9.25303083248528,-54.2117380381064));
#29398=CARTESIAN_POINT('Ctrl Pts',(-73.4153845540563,9.15301827167226,-54.9964148469323));
#29399=CARTESIAN_POINT('Ctrl Pts',(-73.4264161666536,8.85763669586025,-56.717925261362));
#29400=CARTESIAN_POINT('Ctrl Pts',(-73.4430808803201,8.60377450161111,-58.4308174042122));
#29401=CARTESIAN_POINT('Ctrl Pts',(-73.4448411697547,8.68284947729184,-59.7669033675985));
#29402=CARTESIAN_POINT('Ctrl Pts',(-73.4451747928894,8.69238433878198,-59.9087562831018));
#29403=CARTESIAN_POINT('Ctrl Pts',(-73.44562669213,8.71604056254549,-60.2028453790664));
#29404=CARTESIAN_POINT('Ctrl Pts',(-73.4461463667916,8.76722777315182,-60.709121236243));
#29405=CARTESIAN_POINT('Ctrl Pts',(-73.4460480073186,8.90786001593109,-61.7148920567937));
#29406=CARTESIAN_POINT('Ctrl Pts',(-73.4441197541151,9.1446054406115,-62.8349928689661));
#29407=CARTESIAN_POINT('Ctrl Pts',(-73.4415286901041,9.43750309762013,-63.9271205524142));
#29408=CARTESIAN_POINT('Ctrl Pts',(-73.4400020622522,9.61985202168433,-64.5299710521792));
#29409=CARTESIAN_POINT('Ctrl Pts',(-73.4390282344758,9.74732007330091,-64.9271112513151));
#29410=CARTESIAN_POINT('Ctrl Pts',(-73.4383952854194,9.83377984100711,-65.190544158916));
#29411=CARTESIAN_POINT('Ctrl Pts',(-73.437788842033,9.92235401522777,-65.452114631555));
#29412=CARTESIAN_POINT('Ctrl Pts',(-73.4372978605278,10.0014312044763,-65.6791874758265));
#29413=CARTESIAN_POINT('Ctrl Pts',(-73.4370298932181,10.0470362112387,-65.8084346445781));
#29414=CARTESIAN_POINT('Ctrl Pts',(-73.4366398093427,10.1158556040005,-66.0018210798071));
#29415=CARTESIAN_POINT('Ctrl Pts',(-73.4363458444488,10.1739935695649,-66.1618805005531));
#29416=CARTESIAN_POINT('Ctrl Pts',(-73.4358723151197,10.2713750523792,-66.4261097053089));
#29417=CARTESIAN_POINT('Ctrl Pts',(-73.4336120537652,10.3887106230506,-66.7305448161038));
#29418=CARTESIAN_POINT('Ctrl Pts',(-73.4301494517863,10.6307143027596,-67.3072459876494));
#29419=CARTESIAN_POINT('Ctrl Pts',(-73.424002389511,11.0898739110199,-68.2955486969726));
#29420=CARTESIAN_POINT('Ctrl Pts',(-73.4153433621308,12.0908752150646,-70.1534603463187));
#29421=CARTESIAN_POINT('Ctrl Pts',(-73.4163678681088,12.9664745957069,-71.6137496655871));
#29422=CARTESIAN_POINT('Ctrl Pts',(-73.4218155619401,13.5205584289329,-72.6661329169973));
#29423=CARTESIAN_POINT('Ctrl Pts',(-73.4213395272406,13.6562172198672,-72.9238147174108));
#29424=CARTESIAN_POINT('Ctrl Pts',(-73.4213765239796,13.9210493472121,-73.4253887032415));
#29425=CARTESIAN_POINT('Ctrl Pts',(-73.4210556809956,14.2556126777563,-74.0571308465917));
#29426=CARTESIAN_POINT('Ctrl Pts',(-73.4209409401286,14.6562937916129,-74.8110246011275));
#29427=CARTESIAN_POINT('Ctrl Pts',(-73.4206859365661,15.4594132840169,-76.318592205801));
#29428=CARTESIAN_POINT('Ctrl Pts',(-73.4207190966181,16.1288082739189,-77.571148953329));
#29429=CARTESIAN_POINT('Ctrl Pts',(-73.4209847269192,17.0967455638613,-79.3917120442865));
#29430=CARTESIAN_POINT('Ctrl Pts',(-73.420869138286,17.5340881419541,-80.2143709597686));
#29431=CARTESIAN_POINT('Ctrl Pts',(-73.4208691382803,17.9706097293417,-81.0353486618712));
#29432=CARTESIAN_POINT('Ctrl Pts',(-70.6494620665907,3.83081083471652,24.8276526399532));
#29433=CARTESIAN_POINT('Ctrl Pts',(-70.6496326998556,3.8309065566531,24.7786797052078));
#29434=CARTESIAN_POINT('Ctrl Pts',(-70.6498117133617,3.83100671102027,24.7297060068776));
#29435=CARTESIAN_POINT('Ctrl Pts',(-70.6519248484191,3.83219465222234,24.1780050135636));
#29436=CARTESIAN_POINT('Ctrl Pts',(-70.6530399902727,3.83471417259306,23.1723496464166));
#29437=CARTESIAN_POINT('Ctrl Pts',(-70.6553282802904,3.84151496701024,21.1618903863707));
#29438=CARTESIAN_POINT('Ctrl Pts',(-70.6694181592974,3.84933667283851,19.6579544149711));
#29439=CARTESIAN_POINT('Ctrl Pts',(-70.7017966351779,3.85799915528513,18.4074357876463));
#29440=CARTESIAN_POINT('Ctrl Pts',(-70.7166803709366,3.86261513924192,17.8992952787561));
#29441=CARTESIAN_POINT('Ctrl Pts',(-70.7528589610518,3.87486424445333,16.8915795958476));
#29442=CARTESIAN_POINT('Ctrl Pts',(-70.8302083467482,3.9004793077478,15.138016287893));
#29443=CARTESIAN_POINT('Ctrl Pts',(-70.9112744147464,3.91699381429674,13.6541787391245));
#29444=CARTESIAN_POINT('Ctrl Pts',(-70.9763140518782,3.91434651444167,12.4237745483885));
#29445=CARTESIAN_POINT('Ctrl Pts',(-71.0030618549083,3.91054737427746,11.9395233575876));
#29446=CARTESIAN_POINT('Ctrl Pts',(-71.0592521782506,3.894231013442,10.9566785715773));
#29447=CARTESIAN_POINT('Ctrl Pts',(-71.1632499017295,3.8509303468373,9.21600694973984));
#29448=CARTESIAN_POINT('Ctrl Pts',(-71.2580814374877,3.81527639561953,7.68018356218295));
#29449=CARTESIAN_POINT('Ctrl Pts',(-71.3272860059582,3.82213905637395,6.5082419323708));
#29450=CARTESIAN_POINT('Ctrl Pts',(-71.3427494575123,3.82225001371945,6.282526518141));
#29451=CARTESIAN_POINT('Ctrl Pts',(-71.3749139807024,3.81715308070013,5.80195460366119));
#29452=CARTESIAN_POINT('Ctrl Pts',(-71.4340129269757,3.79815273347038,4.94708162916697));
#29453=CARTESIAN_POINT('Ctrl Pts',(-71.5592342028308,3.74889431869233,3.13847244276675));
#29454=CARTESIAN_POINT('Ctrl Pts',(-71.6637008083176,3.81595423074781,1.43529809209986));
#29455=CARTESIAN_POINT('Ctrl Pts',(-71.6955799842735,4.05978002256819,0.17780386520389));
#29456=CARTESIAN_POINT('Ctrl Pts',(-71.6999728057474,4.08946262178212,0.0303556410748098));
#29457=CARTESIAN_POINT('Ctrl Pts',(-71.7086627700793,4.15430584581213,-0.263209799828586));
#29458=CARTESIAN_POINT('Ctrl Pts',(-71.7241795640316,4.2801082104513,-0.770234211702012));
#29459=CARTESIAN_POINT('Ctrl Pts',(-71.7446745302739,4.49143615920851,-1.47731101502265));
#29460=CARTESIAN_POINT('Ctrl Pts',(-71.7621594414976,4.78057190184174,-2.29733031108985));
#29461=CARTESIAN_POINT('Ctrl Pts',(-71.7719402743552,5.19615381873767,-3.35702259704706));
#29462=CARTESIAN_POINT('Ctrl Pts',(-71.7559940767548,5.73883787559449,-4.62551909003516));
#29463=CARTESIAN_POINT('Ctrl Pts',(-71.7136494335196,6.14233732235438,-5.60373018086587));
#29464=CARTESIAN_POINT('Ctrl Pts',(-71.6746530735446,6.36894140367775,-6.21041210479194));
#29465=CARTESIAN_POINT('Ctrl Pts',(-71.6454234832357,6.47958429679363,-6.50916202445099));
#29466=CARTESIAN_POINT('Ctrl Pts',(-71.5852869298051,6.69927064532406,-7.06348618753471));
#29467=CARTESIAN_POINT('Ctrl Pts',(-71.4592692103757,7.10401392951411,-8.02462301779982));
#29468=CARTESIAN_POINT('Ctrl Pts',(-71.2502864953223,7.68573763210261,-9.31372037528634));
#29469=CARTESIAN_POINT('Ctrl Pts',(-71.0413582371967,8.17269012460668,-10.4897486187166));
#29470=CARTESIAN_POINT('Ctrl Pts',(-70.9194484447363,8.41683088542299,-11.22389491883));
#29471=CARTESIAN_POINT('Ctrl Pts',(-70.8610061829472,8.52564011599825,-11.6150582453415));
#29472=CARTESIAN_POINT('Ctrl Pts',(-70.8363829293454,8.569358881547,-11.8004074281031));
#29473=CARTESIAN_POINT('Ctrl Pts',(-70.8199032162588,8.59828192577974,-11.9363061091416));
#29474=CARTESIAN_POINT('Ctrl Pts',(-70.8088878911491,8.61784484280418,-12.0351367520892));
#29475=CARTESIAN_POINT('Ctrl Pts',(-70.787732704196,8.65261205359186,-12.2300795541281));
#29476=CARTESIAN_POINT('Ctrl Pts',(-70.7529154929867,8.70419486900887,-12.5775059987084));
#29477=CARTESIAN_POINT('Ctrl Pts',(-70.674627889547,8.79351300847224,-13.4950550826304));
#29478=CARTESIAN_POINT('Ctrl Pts',(-70.6249383740797,8.77853835100137,-14.6202155928646));
#29479=CARTESIAN_POINT('Ctrl Pts',(-70.5943086444658,8.73281849448334,-15.8659974403439));
#29480=CARTESIAN_POINT('Ctrl Pts',(-70.5807074443851,8.71427141760064,-16.5189898372744));
#29481=CARTESIAN_POINT('Ctrl Pts',(-70.5696295443514,8.7084393082528,-17.0599664971091));
#29482=CARTESIAN_POINT('Ctrl Pts',(-70.5636960856804,8.710000548671,-17.3368382446092));
#29483=CARTESIAN_POINT('Ctrl Pts',(-70.5590378482671,8.71328878005061,-17.5453595325233));
#29484=CARTESIAN_POINT('Ctrl Pts',(-70.5561697720275,8.71501732932909,-17.66218208993));
#29485=CARTESIAN_POINT('Ctrl Pts',(-70.5510382949045,8.71822189311693,-17.9085187419594));
#29486=CARTESIAN_POINT('Ctrl Pts',(-70.5468139861943,8.72072632138071,-18.1508169083625));
#29487=CARTESIAN_POINT('Ctrl Pts',(-70.5434014822654,8.7226857771753,-18.3960892577941));
#29488=CARTESIAN_POINT('Ctrl Pts',(-70.5415889576892,8.72367630379317,-18.5490737482143));
#29489=CARTESIAN_POINT('Ctrl Pts',(-70.5403198577929,8.72434263374008,-18.6718055273237));
#29490=CARTESIAN_POINT('Ctrl Pts',(-70.539167663306,8.7249251220034,-18.7945738239458));
#29491=CARTESIAN_POINT('Ctrl Pts',(-70.5364628645629,8.72620000910083,-19.1326061304726));
#29492=CARTESIAN_POINT('Ctrl Pts',(-70.5344079682884,8.72660365685414,-19.6878742855126));
#29493=CARTESIAN_POINT('Ctrl Pts',(-70.5355608609243,8.72395856068241,-20.6811225067078));
#29494=CARTESIAN_POINT('Ctrl Pts',(-70.542387528159,8.7170164050489,-21.9344562421943));
#29495=CARTESIAN_POINT('Ctrl Pts',(-70.5458632611026,8.71339189514063,-22.9497488309881));
#29496=CARTESIAN_POINT('Ctrl Pts',(-70.5450374514181,8.7135098723975,-23.5865408257813));
#29497=CARTESIAN_POINT('Ctrl Pts',(-70.5447471842888,8.71355843775048,-23.8349075051346));
#29498=CARTESIAN_POINT('Ctrl Pts',(-70.5442924475687,8.71366924240936,-24.3345135506893));
#29499=CARTESIAN_POINT('Ctrl Pts',(-70.543800864288,8.71388643206869,-25.2095712506264));
#29500=CARTESIAN_POINT('Ctrl Pts',(-70.5437828030668,8.71422173656197,-26.4642473457495));
#29501=CARTESIAN_POINT('Ctrl Pts',(-70.5443151186548,8.714485394657,-27.972125838861));
#29502=CARTESIAN_POINT('Ctrl Pts',(-70.544657365899,8.71450179715225,-28.9765670388092));
#29503=CARTESIAN_POINT('Ctrl Pts',(-70.544753185945,8.71442826770179,-29.540599925421));
#29504=CARTESIAN_POINT('Ctrl Pts',(-70.5447725146452,8.71440819195271,-29.6659124473631));
#29505=CARTESIAN_POINT('Ctrl Pts',(-70.5448015365278,8.71435600444617,-29.9166176840538));
#29506=CARTESIAN_POINT('Ctrl Pts',(-70.5448305077078,8.71423710213987,-30.3554939541661));
#29507=CARTESIAN_POINT('Ctrl Pts',(-70.5448321347687,8.71389907695821,-31.2337491285771));
#29508=CARTESIAN_POINT('Ctrl Pts',(-70.5448349164206,8.71336869028112,-32.2380147384793));
#29509=CARTESIAN_POINT('Ctrl Pts',(-70.5451063262961,8.71283065278324,-33.2417295013175));
#29510=CARTESIAN_POINT('Ctrl Pts',(-70.5455105362915,8.71245869625278,-33.9939611185162));
#29511=CARTESIAN_POINT('Ctrl Pts',(-70.546176741767,8.71216609792829,-34.7453143056492));
#29512=CARTESIAN_POINT('Ctrl Pts',(-70.5468406439546,8.71204454454721,-35.2454583991906));
#29513=CARTESIAN_POINT('Ctrl Pts',(-70.5474393800059,8.71198876986363,-35.6212034339876));
#29514=CARTESIAN_POINT('Ctrl Pts',(-70.5478930911235,8.71193803468518,-35.8724848760286));
#29515=CARTESIAN_POINT('Ctrl Pts',(-70.5489856262303,8.71179501958184,-36.3747125556351));
#29516=CARTESIAN_POINT('Ctrl Pts',(-70.5513128995724,8.71147840408229,-37.252252911644));
#29517=CARTESIAN_POINT('Ctrl Pts',(-70.5571101664544,8.71082696437478,-39.0044582742178));
#29518=CARTESIAN_POINT('Ctrl Pts',(-70.5621980028138,8.71119560410614,-40.5077353732109));
#29519=CARTESIAN_POINT('Ctrl Pts',(-70.5642506312549,8.71287280584407,-41.6413572595022));
#29520=CARTESIAN_POINT('Ctrl Pts',(-70.5646509318823,8.71307821510131,-41.8892302310715));
#29521=CARTESIAN_POINT('Ctrl Pts',(-70.5651111355399,8.71300711616514,-42.2633393490989));
#29522=CARTESIAN_POINT('Ctrl Pts',(-70.5654537720773,8.7126560517315,-42.6378979443855));
#29523=CARTESIAN_POINT('Ctrl Pts',(-70.5657827919375,8.71195170856678,-43.1387093024551));
#29524=CARTESIAN_POINT('Ctrl Pts',(-70.5660093931435,8.7108842783085,-43.7665993987514));
#29525=CARTESIAN_POINT('Ctrl Pts',(-70.5661603846999,8.7101283917312,-44.5227897914755));
#29526=CARTESIAN_POINT('Ctrl Pts',(-70.5663301874602,8.71062807138128,-45.1547197983672));
#29527=CARTESIAN_POINT('Ctrl Pts',(-70.5665785295845,8.71212986471067,-45.6610761158928));
#29528=CARTESIAN_POINT('Ctrl Pts',(-70.5668426229271,8.71391030213836,-46.0412011432084));
#29529=CARTESIAN_POINT('Ctrl Pts',(-70.5672060860399,8.71645036476586,-46.4215986512285));
#29530=CARTESIAN_POINT('Ctrl Pts',(-70.5678510624984,8.72099633974999,-46.9291444376783));
#29531=CARTESIAN_POINT('Ctrl Pts',(-70.5685490049604,8.72585625964623,-47.3099306692449));
#29532=CARTESIAN_POINT('Ctrl Pts',(-70.5694315859434,8.73193307009486,-47.6921242948781));
#29533=CARTESIAN_POINT('Ctrl Pts',(-70.5700028112621,8.73773568313054,-47.9611506235088));
#29534=CARTESIAN_POINT('Ctrl Pts',(-70.5712340825493,8.75417753941003,-48.4860451568485));
#29535=CARTESIAN_POINT('Ctrl Pts',(-70.5736142010392,8.79330423740066,-49.3952751998665));
#29536=CARTESIAN_POINT('Ctrl Pts',(-70.5779570100187,8.86304416439338,-50.6527583617862));
#29537=CARTESIAN_POINT('Ctrl Pts',(-70.5848238355766,8.92405748189299,-52.0999793978263));
#29538=CARTESIAN_POINT('Ctrl Pts',(-70.5901323883384,8.92307983476999,-53.0207592136404));
#29539=CARTESIAN_POINT('Ctrl Pts',(-70.5933835869417,8.90240786789031,-53.5826175741996));
#29540=CARTESIAN_POINT('Ctrl Pts',(-70.5945272935145,8.89128748430115,-53.7816791081091));
#29541=CARTESIAN_POINT('Ctrl Pts',(-70.5970120911207,8.85415045768397,-54.2126751468643));
#29542=CARTESIAN_POINT('Ctrl Pts',(-70.6020877584862,8.75468433042563,-54.9974481723177));
#29543=CARTESIAN_POINT('Ctrl Pts',(-70.6160278517372,8.4606177040147,-56.7189510136224));
#29544=CARTESIAN_POINT('Ctrl Pts',(-70.6351143486718,8.20797974704676,-58.4315982466486));
#29545=CARTESIAN_POINT('Ctrl Pts',(-70.6378400431479,8.28745191915634,-59.7672962513482));
#29546=CARTESIAN_POINT('Ctrl Pts',(-70.6382882810371,8.29702776371256,-59.9091079122869));
#29547=CARTESIAN_POINT('Ctrl Pts',(-70.6389559396657,8.3207566747499,-60.203116134479));
#29548=CARTESIAN_POINT('Ctrl Pts',(-70.6398204929652,8.37204147372282,-60.7092633605087));
#29549=CARTESIAN_POINT('Ctrl Pts',(-70.6402897909106,8.51277007689702,-61.7148227459977));
#29550=CARTESIAN_POINT('Ctrl Pts',(-70.6387760021451,8.74946254134713,-62.8347878524703));
#29551=CARTESIAN_POINT('Ctrl Pts',(-70.63645635019,9.04226083934355,-63.9268742425419));
#29552=CARTESIAN_POINT('Ctrl Pts',(-70.6350467453139,9.22455565865073,-64.5297348535941));
#29553=CARTESIAN_POINT('Ctrl Pts',(-70.6341437471854,9.35199658562109,-64.9268950821234));
#29554=CARTESIAN_POINT('Ctrl Pts',(-70.6335566103036,9.43844111080219,-65.1903448912955));
#29555=CARTESIAN_POINT('Ctrl Pts',(-70.6329946828321,9.52700517591339,-65.451937409211));
#29556=CARTESIAN_POINT('Ctrl Pts',(-70.6325428578251,9.60607928875794,-65.6790341699771));
#29557=CARTESIAN_POINT('Ctrl Pts',(-70.6322975262368,9.65168438950241,-65.8082963195497));
#29558=CARTESIAN_POINT('Ctrl Pts',(-70.6319417515286,9.72050584533726,-66.0017064990561));
#29559=CARTESIAN_POINT('Ctrl Pts',(-70.6316773393184,9.77864984379035,-66.1617885164817));
#29560=CARTESIAN_POINT('Ctrl Pts',(-70.6312550527681,9.87604754909493,-66.4260578348278));
#29561=CARTESIAN_POINT('Ctrl Pts',(-70.6290388968904,9.99337956946595,-66.7304847584415));
#29562=CARTESIAN_POINT('Ctrl Pts',(-70.6256406643102,10.235385949348,-67.307196970974));
#29563=CARTESIAN_POINT('Ctrl Pts',(-70.6195478587563,10.6945412135849,-68.2955031148334));
#29564=CARTESIAN_POINT('Ctrl Pts',(-70.6108253052356,11.6955285102401,-70.1534276569231));
#29565=CARTESIAN_POINT('Ctrl Pts',(-70.6116939852769,12.5711088080986,-71.6137122958572));
#29566=CARTESIAN_POINT('Ctrl Pts',(-70.6171589562653,13.1251918432522,-72.6660905861456));
#29567=CARTESIAN_POINT('Ctrl Pts',(-70.6166820361121,13.2608502284483,-72.9237734197364));
#29568=CARTESIAN_POINT('Ctrl Pts',(-70.6167197576935,13.5256819745422,-73.4253481708406));
#29569=CARTESIAN_POINT('Ctrl Pts',(-70.6163984323959,13.8602451411829,-74.0570914180674));
#29570=CARTESIAN_POINT('Ctrl Pts',(-70.6162833700721,14.2609265969471,-74.8109860525134));
#29571=CARTESIAN_POINT('Ctrl Pts',(-70.6160270030381,15.0640473305046,-76.3185549282437));
#29572=CARTESIAN_POINT('Ctrl Pts',(-70.6160590352253,15.7334436640084,-77.5711107024718));
#29573=CARTESIAN_POINT('Ctrl Pts',(-70.6163255657832,16.7013800620162,-79.3916714201663));
#29574=CARTESIAN_POINT('Ctrl Pts',(-70.6162096418444,17.1387228581873,-80.2143307870197));
#29575=CARTESIAN_POINT('Ctrl Pts',(-70.6162096418429,17.5752444455778,-81.0353084891142));
#29576=CARTESIAN_POINT('Ctrl Pts',(-67.8429979490876,3.43540937587766,24.8291468061157));
#29577=CARTESIAN_POINT('Ctrl Pts',(-67.843255199307,3.43548039997282,24.7802219150478));
#29578=CARTESIAN_POINT('Ctrl Pts',(-67.8435249642338,3.43555466825619,24.7312970013852));
#29579=CARTESIAN_POINT('Ctrl Pts',(-67.8467076136049,3.43643894377634,24.1801610961006));
#29580=CARTESIAN_POINT('Ctrl Pts',(-67.8504237539074,3.43796780523234,23.1756926839324));
#29581=CARTESIAN_POINT('Ctrl Pts',(-67.8599419168608,3.44198305776693,21.1660006053159));
#29582=CARTESIAN_POINT('Ctrl Pts',(-67.8810374140118,3.44791190792428,19.6612635225141));
#29583=CARTESIAN_POINT('Ctrl Pts',(-67.9194104989257,3.45625007158521,18.4096589917386));
#29584=CARTESIAN_POINT('Ctrl Pts',(-67.9382125535026,3.46076834152602,17.9030504603971));
#29585=CARTESIAN_POINT('Ctrl Pts',(-67.9860602467786,3.47303181360074,16.8965429211016));
#29586=CARTESIAN_POINT('Ctrl Pts',(-68.0882538963617,3.49935505131162,15.1438911469587));
#29587=CARTESIAN_POINT('Ctrl Pts',(-68.1787023358157,3.51729839131463,13.6549281187412));
#29588=CARTESIAN_POINT('Ctrl Pts',(-68.2236661968178,3.51554813699857,12.416125634103));
#29589=CARTESIAN_POINT('Ctrl Pts',(-68.240294156464,3.5132479046786,11.9218528873524));
#29590=CARTESIAN_POINT('Ctrl Pts',(-68.2689151704927,3.50367771304502,10.9290940226273));
#29591=CARTESIAN_POINT('Ctrl Pts',(-68.3084503585006,3.47762876365091,9.18311221725741));
#29592=CARTESIAN_POINT('Ctrl Pts',(-68.3301235588637,3.45152683070009,7.6704450302173));
#29593=CARTESIAN_POINT('Ctrl Pts',(-68.3456628288656,3.44053057254519,6.52970039108954));
#29594=CARTESIAN_POINT('Ctrl Pts',(-68.3481621521419,3.43698218092217,6.2958605672267));
#29595=CARTESIAN_POINT('Ctrl Pts',(-68.3499178243137,3.42562356289472,5.81106989728593));
#29596=CARTESIAN_POINT('Ctrl Pts',(-68.3461693060382,3.39691433075224,4.95317410772437));
#29597=CARTESIAN_POINT('Ctrl Pts',(-68.3238707383516,3.3264308083201,3.17678700344086));
#29598=CARTESIAN_POINT('Ctrl Pts',(-68.3243575733678,3.30825572512503,1.5672747065012));
#29599=CARTESIAN_POINT('Ctrl Pts',(-68.3814826358144,3.39780225920189,0.387491389599531));
#29600=CARTESIAN_POINT('Ctrl Pts',(-68.3892510774313,3.40656307744178,0.265861555568177));
#29601=CARTESIAN_POINT('Ctrl Pts',(-68.4077487811753,3.42556704012703,0.0101690127921557));
#29602=CARTESIAN_POINT('Ctrl Pts',(-68.4474830193355,3.45999959830791,-0.435805451239607));
#29603=CARTESIAN_POINT('Ctrl Pts',(-68.5214053738539,3.51863065866942,-1.08807657225968));
#29604=CARTESIAN_POINT('Ctrl Pts',(-68.6244249906881,3.61485033990705,-1.88625004060008));
#29605=CARTESIAN_POINT('Ctrl Pts',(-68.762100742499,3.78900570837791,-2.97208690411789));
#29606=CARTESIAN_POINT('Ctrl Pts',(-68.8980921258,4.10565455346679,-4.35855017453348));
#29607=CARTESIAN_POINT('Ctrl Pts',(-68.9128972361772,4.46292517231313,-5.48743317652969));
#29608=CARTESIAN_POINT('Ctrl Pts',(-68.8835351541264,4.71911664935449,-6.20457641486434));
#29609=CARTESIAN_POINT('Ctrl Pts',(-68.8610406882809,4.84466478657557,-6.5358207313883));
#29610=CARTESIAN_POINT('Ctrl Pts',(-68.810269153138,5.111352077503,-7.14389354421227));
#29611=CARTESIAN_POINT('Ctrl Pts',(-68.7008986449468,5.6308280985943,-8.16490507596953));
#29612=CARTESIAN_POINT('Ctrl Pts',(-68.5263328009642,6.43604072547312,-9.48848437606004));
#29613=CARTESIAN_POINT('Ctrl Pts',(-68.3742509965807,7.15026503593484,-10.6834425942453));
#29614=CARTESIAN_POINT('Ctrl Pts',(-68.2960383802098,7.5095388116318,-11.4168829107783));
#29615=CARTESIAN_POINT('Ctrl Pts',(-68.2603561980416,7.66556287853389,-11.7970284531808));
#29616=CARTESIAN_POINT('Ctrl Pts',(-68.2455289714394,7.72624062966262,-11.97182504539));
#29617=CARTESIAN_POINT('Ctrl Pts',(-68.2353427298046,7.76560735334509,-12.097787494051));
#29618=CARTESIAN_POINT('Ctrl Pts',(-68.2257690214525,7.79765559041035,-12.2057348844777));
#29619=CARTESIAN_POINT('Ctrl Pts',(-68.2071477696638,7.8534301152825,-12.4091866131882));
#29620=CARTESIAN_POINT('Ctrl Pts',(-68.1716358694143,7.94179346169686,-12.7737393881953));
#29621=CARTESIAN_POINT('Ctrl Pts',(-68.0704929322039,8.1155169155222,-13.7174848416372));
#29622=CARTESIAN_POINT('Ctrl Pts',(-67.9379388540401,8.19410547769043,-14.8288865432328));
#29623=CARTESIAN_POINT('Ctrl Pts',(-67.827047180042,8.24470200634281,-16.0333715681186));
#29624=CARTESIAN_POINT('Ctrl Pts',(-67.7795672382218,8.26978736748521,-16.6593610065802));
#29625=CARTESIAN_POINT('Ctrl Pts',(-67.7480131276514,8.29424328490067,-17.1744632202735));
#29626=CARTESIAN_POINT('Ctrl Pts',(-67.73458059527,8.30876634793277,-17.4370136882304));
#29627=CARTESIAN_POINT('Ctrl Pts',(-67.7255258325098,8.32073410293769,-17.6343112047601));
#29628=CARTESIAN_POINT('Ctrl Pts',(-67.7200862703883,8.32680648549444,-17.7435073503106));
#29629=CARTESIAN_POINT('Ctrl Pts',(-67.7104146454208,8.33824536339626,-17.9755230869486));
#29630=CARTESIAN_POINT('Ctrl Pts',(-67.7026777620944,8.34715217005881,-18.2044889428511));
#29631=CARTESIAN_POINT('Ctrl Pts',(-67.6966341645092,8.3541764453997,-18.4375568529196));
#29632=CARTESIAN_POINT('Ctrl Pts',(-67.6935353376028,8.3577232053768,-18.5833563338914));
#29633=CARTESIAN_POINT('Ctrl Pts',(-67.6914358025922,8.36011433549464,-18.7006166844035));
#29634=CARTESIAN_POINT('Ctrl Pts',(-67.6895828416986,8.36220414098241,-18.8180952792904));
#29635=CARTESIAN_POINT('Ctrl Pts',(-67.6854660405954,8.36676764207297,-19.1423216763214));
#29636=CARTESIAN_POINT('Ctrl Pts',(-67.6837255962329,8.36814152476923,-19.6791089082259));
#29637=CARTESIAN_POINT('Ctrl Pts',(-67.6906843160803,8.35814000473539,-20.651093751224));
#29638=CARTESIAN_POINT('Ctrl Pts',(-67.710406632541,8.33191835568154,-21.899623813537));
#29639=CARTESIAN_POINT('Ctrl Pts',(-67.7210624318957,8.31774556571313,-22.9339497328628));
#29640=CARTESIAN_POINT('Ctrl Pts',(-67.7207994578438,8.31808112582329,-23.5892652088098));
#29641=CARTESIAN_POINT('Ctrl Pts',(-67.720733117923,8.31821360280331,-23.8355542489468));
#29642=CARTESIAN_POINT('Ctrl Pts',(-67.7207273213582,8.31850430364268,-24.3362847484307));
#29643=CARTESIAN_POINT('Ctrl Pts',(-67.7210039430532,8.31904808417056,-25.2105437686112));
#29644=CARTESIAN_POINT('Ctrl Pts',(-67.7219552216887,8.31985387668672,-26.4655180104148));
#29645=CARTESIAN_POINT('Ctrl Pts',(-67.7231943423994,8.32050740196497,-27.9726806839646));
#29646=CARTESIAN_POINT('Ctrl Pts',(-67.7235155311288,8.32051519025861,-28.9767684556765));
#29647=CARTESIAN_POINT('Ctrl Pts',(-67.7233971219608,8.32032151698294,-29.5405267267874));
#29648=CARTESIAN_POINT('Ctrl Pts',(-67.7233593675948,8.32027011766274,-29.6657703361541));
#29649=CARTESIAN_POINT('Ctrl Pts',(-67.723241014596,8.32013958929522,-29.9163521225107));
#29650=CARTESIAN_POINT('Ctrl Pts',(-67.7229297492033,8.31984426995699,-30.3550203608265));
#29651=CARTESIAN_POINT('Ctrl Pts',(-67.7219636671122,8.31901320679915,-31.2329310628976));
#29652=CARTESIAN_POINT('Ctrl Pts',(-67.720400340325,8.31768767781877,-32.2369480939191));
#29653=CARTESIAN_POINT('Ctrl Pts',(-67.7190338173315,8.31628904161721,-33.2405997552514));
#29654=CARTESIAN_POINT('Ctrl Pts',(-67.718271679738,8.31528342970505,-33.9928850424582));
#29655=CARTESIAN_POINT('Ctrl Pts',(-67.7179342080551,8.31441764247642,-34.7443623717059));
#29656=CARTESIAN_POINT('Ctrl Pts',(-67.7181023937929,8.31398381050784,-35.2446500331208));
#29657=CARTESIAN_POINT('Ctrl Pts',(-67.7184178356948,8.31372988048811,-35.6205257014851));
#29658=CARTESIAN_POINT('Ctrl Pts',(-67.7186970170676,8.31355042220773,-35.8717973937954));
#29659=CARTESIAN_POINT('Ctrl Pts',(-67.7194958221841,8.31316150286721,-36.3740651607934));
#29660=CARTESIAN_POINT('Ctrl Pts',(-67.7214436471302,8.31245406754501,-37.2516350499055));
#29661=CARTESIAN_POINT('Ctrl Pts',(-67.7268950573798,8.31112798346429,-39.0039525846174));
#29662=CARTESIAN_POINT('Ctrl Pts',(-67.7320219606896,8.31110091035574,-40.5072829288273));
#29663=CARTESIAN_POINT('Ctrl Pts',(-67.733879661603,8.31250535114878,-41.6409687968382));
#29664=CARTESIAN_POINT('Ctrl Pts',(-67.7342268248544,8.3126486066805,-41.8888478011433));
#29665=CARTESIAN_POINT('Ctrl Pts',(-67.734585193687,8.31248482742067,-42.2629729327167));
#29666=CARTESIAN_POINT('Ctrl Pts',(-67.7348093430965,8.31204199054457,-42.637548579422));
#29667=CARTESIAN_POINT('Ctrl Pts',(-67.7349662316575,8.31121885167147,-43.1383864958984));
#29668=CARTESIAN_POINT('Ctrl Pts',(-67.7349656602,8.31001211263342,-43.7663158642005));
#29669=CARTESIAN_POINT('Ctrl Pts',(-67.7348717584322,8.30911406018918,-44.5225635854086));
#29670=CARTESIAN_POINT('Ctrl Pts',(-67.7348996531857,8.30952467107504,-45.1545490110695));
#29671=CARTESIAN_POINT('Ctrl Pts',(-67.7350952479235,8.31097630696777,-45.6609588687116));
#29672=CARTESIAN_POINT('Ctrl Pts',(-67.7353560076653,8.3127316819013,-46.0411264962276));
#29673=CARTESIAN_POINT('Ctrl Pts',(-67.7357582008244,8.31526032504559,-46.421569382839));
#29674=CARTESIAN_POINT('Ctrl Pts',(-67.7365189774708,8.31981101030796,-46.9291804544779));
#29675=CARTESIAN_POINT('Ctrl Pts',(-67.7373839436146,8.32469869153759,-47.3100174825679));
#29676=CARTESIAN_POINT('Ctrl Pts',(-67.7385002254718,8.33082229499641,-47.6922674992038));
#29677=CARTESIAN_POINT('Ctrl Pts',(-67.739244988589,8.33666447214043,-47.9613494799267));
#29678=CARTESIAN_POINT('Ctrl Pts',(-67.7408837362312,8.35320967438326,-48.4863334714169));
#29679=CARTESIAN_POINT('Ctrl Pts',(-67.7441271193585,8.3925774158339,-49.3956976463571));
#29680=CARTESIAN_POINT('Ctrl Pts',(-67.75007447448,8.46278740267436,-50.6532900551304));
#29681=CARTESIAN_POINT('Ctrl Pts',(-67.759310281912,8.52447858594555,-52.1005349938358));
#29682=CARTESIAN_POINT('Ctrl Pts',(-67.7663979457576,8.52396820704625,-53.0212590273571));
#29683=CARTESIAN_POINT('Ctrl Pts',(-67.7707986217468,8.50358566761648,-53.5830646349072));
#29684=CARTESIAN_POINT('Ctrl Pts',(-67.7724421193683,8.49258175718754,-53.7821557918875));
#29685=CARTESIAN_POINT('Ctrl Pts',(-67.776029352105,8.45571054118338,-54.2131754916418));
#29686=CARTESIAN_POINT('Ctrl Pts',(-67.7832589050826,8.35677044352376,-54.9979892349162));
#29687=CARTESIAN_POINT('Ctrl Pts',(-67.8019983761006,8.06391832573667,-56.7195146620943));
#29688=CARTESIAN_POINT('Ctrl Pts',(-67.8248629176182,7.81231491994759,-58.4320640413801));
#29689=CARTESIAN_POINT('Ctrl Pts',(-67.8290231786131,7.89213968485429,-59.7675454191527));
#29690=CARTESIAN_POINT('Ctrl Pts',(-67.829637938248,7.90175378771661,-59.9093328492615));
#29691=CARTESIAN_POINT('Ctrl Pts',(-67.8306102124591,7.92555044535696,-60.2032942620685));
#29692=CARTESIAN_POINT('Ctrl Pts',(-67.8319358606205,7.97692831211166,-60.7093669674856));
#29693=CARTESIAN_POINT('Ctrl Pts',(-67.8330666988999,8.11775658317007,-61.7148057960873));
#29694=CARTESIAN_POINT('Ctrl Pts',(-67.8318365893804,8.3544189694753,-62.8347014563645));
#29695=CARTESIAN_POINT('Ctrl Pts',(-67.8295768244033,8.64714320487281,-63.9267786658913));
#29696=CARTESIAN_POINT('Ctrl Pts',(-67.8281626669886,8.82939642463849,-64.5296542650456));
#29697=CARTESIAN_POINT('Ctrl Pts',(-67.8272594889568,8.95681621745233,-64.9268322635415));
#29698=CARTESIAN_POINT('Ctrl Pts',(-67.8266742594514,9.04324888375184,-65.1902959131685));
#29699=CARTESIAN_POINT('Ctrl Pts',(-67.8261190407547,9.13180490501319,-65.4519052012751));
#29700=CARTESIAN_POINT('Ctrl Pts',(-67.8256806306326,9.21087657959977,-65.6790191260735));
#29701=CARTESIAN_POINT('Ctrl Pts',(-67.8254455665297,9.25648173733892,-65.8082917862273));
#29702=CARTESIAN_POINT('Ctrl Pts',(-67.8251080419102,9.32530480735155,-66.0017184022138));
#29703=CARTESIAN_POINT('Ctrl Pts',(-67.8248651643453,9.38345347502709,-66.1618155768751));
#29704=CARTESIAN_POINT('Ctrl Pts',(-67.8244897857844,9.48086408035106,-66.4261113164743));
#29705=CARTESIAN_POINT('Ctrl Pts',(-67.8223265957053,9.59820115895211,-66.7305377189812));
#29706=CARTESIAN_POINT('Ctrl Pts',(-67.8190059950224,9.8402199531971,-67.3072625970374));
#29707=CARTESIAN_POINT('Ctrl Pts',(-67.8129978099209,10.2993889138899,-68.2955787840444));
#29708=CARTESIAN_POINT('Ctrl Pts',(-67.8042650502226,11.300383254939,-70.1535168902183));
#29709=CARTESIAN_POINT('Ctrl Pts',(-67.8049715146091,12.1759405893878,-71.6137976724565));
#29710=CARTESIAN_POINT('Ctrl Pts',(-67.8104043429099,12.7300091438892,-72.6661690854145));
#29711=CARTESIAN_POINT('Ctrl Pts',(-67.8099292386307,12.865668301269,-72.9238530002178));
#29712=CARTESIAN_POINT('Ctrl Pts',(-67.8099657471829,13.1304995285569,-73.4254283169777));
#29713=CARTESIAN_POINT('Ctrl Pts',(-67.8096453736191,13.4650631962054,-74.0571725682281));
#29714=CARTESIAN_POINT('Ctrl Pts',(-67.8095307834107,13.8657451167143,-74.81106786658));
#29715=CARTESIAN_POINT('Ctrl Pts',(-67.8092764976037,14.6688673763839,-76.318637675562));
#29716=CARTESIAN_POINT('Ctrl Pts',(-67.8093100673287,15.3382645987951,-77.5711925792361));
#29717=CARTESIAN_POINT('Ctrl Pts',(-67.8095751893663,16.3061996227081,-79.3917515175623));
#29718=CARTESIAN_POINT('Ctrl Pts',(-67.8094597961512,16.743542771233,-80.2144112531435));
#29719=CARTESIAN_POINT('Ctrl Pts',(-67.8094597961536,17.1800643586234,-81.0353889552398));
#29720=CARTESIAN_POINT('Ctrl Pts',(-65.0350898325616,3.04280014736699,24.8318418817188));
#29721=CARTESIAN_POINT('Ctrl Pts',(-65.035302902329,3.04280068956435,24.7830007108261));
#29722=CARTESIAN_POINT('Ctrl Pts',(-65.0355263318473,3.0428012433223,24.7341611475317));
#29723=CARTESIAN_POINT('Ctrl Pts',(-65.0381652998135,3.04281055487639,24.1840050646084));
#29724=CARTESIAN_POINT('Ctrl Pts',(-65.0405012624098,3.04221819256434,23.1805167946382));
#29725=CARTESIAN_POINT('Ctrl Pts',(-65.046136422076,3.04039629670115,21.1726954882089));
#29726=CARTESIAN_POINT('Ctrl Pts',(-65.0636892145831,3.04050003718048,19.668687863039));
#29727=CARTESIAN_POINT('Ctrl Pts',(-65.0993528390164,3.04373154009752,18.4175940393545));
#29728=CARTESIAN_POINT('Ctrl Pts',(-65.1167624047629,3.04513799530223,17.916739559878));
#29729=CARTESIAN_POINT('Ctrl Pts',(-65.1610420261281,3.04848022156998,16.914221109985));
#29730=CARTESIAN_POINT('Ctrl Pts',(-65.2560901491897,3.05590136084768,15.1605997557044));
#29731=CARTESIAN_POINT('Ctrl Pts',(-65.3426276974946,3.06567624187454,13.6528135161078));
#29732=CARTESIAN_POINT('Ctrl Pts',(-65.3898854169488,3.07637962508634,12.3899242765431));
#29733=CARTESIAN_POINT('Ctrl Pts',(-65.4085188963124,3.08135345362665,11.8852540838332));
#29734=CARTESIAN_POINT('Ctrl Pts',(-65.4441924276268,3.09334441748007,10.8780247911361));
#29735=CARTESIAN_POINT('Ctrl Pts',(-65.5009212372911,3.11769138469222,9.11918270865987));
#29736=CARTESIAN_POINT('Ctrl Pts',(-65.5344759686303,3.13759494396961,7.61787678554747));
#29737=CARTESIAN_POINT('Ctrl Pts',(-65.5471823475504,3.14577486589797,6.4941358079782));
#29738=CARTESIAN_POINT('Ctrl Pts',(-65.5490064258502,3.14719343720313,6.24591568025131));
#29739=CARTESIAN_POINT('Ctrl Pts',(-65.5493650130214,3.14901199750275,5.7479323737717));
#29740=CARTESIAN_POINT('Ctrl Pts',(-65.5427232865531,3.15003714353534,4.87351085584839));
#29741=CARTESIAN_POINT('Ctrl Pts',(-65.5123332075237,3.1473687997001,3.11538441955382));
#29742=CARTESIAN_POINT('Ctrl Pts',(-65.4950406104052,3.15243776668915,1.59718257170604));
#29743=CARTESIAN_POINT('Ctrl Pts',(-65.5195969730143,3.16718209086072,0.529985838135656));
#29744=CARTESIAN_POINT('Ctrl Pts',(-65.5229264725584,3.168044097656,0.428401865576983));
#29745=CARTESIAN_POINT('Ctrl Pts',(-65.5308531279283,3.16715647935709,0.20693437589857));
#29746=CARTESIAN_POINT('Ctrl Pts',(-65.5479649445266,3.15891659841762,-0.182152293832136));
#29747=CARTESIAN_POINT('Ctrl Pts',(-65.5803536258395,3.1312880024813,-0.769064702460121));
#29748=CARTESIAN_POINT('Ctrl Pts',(-65.6288080052194,3.08514072014695,-1.51529846596412));
#29749=CARTESIAN_POINT('Ctrl Pts',(-65.7009443438072,3.02971820738691,-2.57286938657852));
#29750=CARTESIAN_POINT('Ctrl Pts',(-65.7958702426753,3.02141716607343,-4.01464059995897));
#29751=CARTESIAN_POINT('Ctrl Pts',(-65.8339671111026,3.21413230294904,-5.28558894656125));
#29752=CARTESIAN_POINT('Ctrl Pts',(-65.8290177318522,3.43646413138794,-6.09719401145983));
#29753=CARTESIAN_POINT('Ctrl Pts',(-65.8247331963601,3.54288486877194,-6.43980777047141));
#29754=CARTESIAN_POINT('Ctrl Pts',(-65.8126150415913,3.78785976564052,-7.07974275656304));
#29755=CARTESIAN_POINT('Ctrl Pts',(-65.7825405638733,4.28935048702146,-8.13424291300961));
#29756=CARTESIAN_POINT('Ctrl Pts',(-65.7262822211076,5.10673621212295,-9.47955334379582));
#29757=CARTESIAN_POINT('Ctrl Pts',(-65.6776040037731,5.87382394656201,-10.6881581647769));
#29758=CARTESIAN_POINT('Ctrl Pts',(-65.6530788862006,6.29690400402921,-11.4492892101479));
#29759=CARTESIAN_POINT('Ctrl Pts',(-65.6402560174144,6.4939315689468,-11.8545382815407));
#29760=CARTESIAN_POINT('Ctrl Pts',(-65.6338099852804,6.57563946285295,-12.0455045702372));
#29761=CARTESIAN_POINT('Ctrl Pts',(-65.6284734069914,6.63058551780554,-12.1854030496931));
#29762=CARTESIAN_POINT('Ctrl Pts',(-65.6190428236937,6.67764656971381,-12.3120037968729));
#29763=CARTESIAN_POINT('Ctrl Pts',(-65.6011861723993,6.76260038308683,-12.546849040613));
#29764=CARTESIAN_POINT('Ctrl Pts',(-65.5631649581857,6.90664395919742,-12.9665027856001));
#29765=CARTESIAN_POINT('Ctrl Pts',(-65.4439714345449,7.23556311786381,-14.0348885563294));
#29766=CARTESIAN_POINT('Ctrl Pts',(-65.2467963721198,7.50697144292392,-15.2036317173101));
#29767=CARTESIAN_POINT('Ctrl Pts',(-65.0613545935836,7.72730267070285,-16.3447670932083));
#29768=CARTESIAN_POINT('Ctrl Pts',(-64.9821956515023,7.82439148941587,-16.9129981157234));
#29769=CARTESIAN_POINT('Ctrl Pts',(-64.9318219661531,7.8931744738948,-17.3665625853196));
#29770=CARTESIAN_POINT('Ctrl Pts',(-64.9119293832766,7.92424621796352,-17.5936131468181));
#29771=CARTESIAN_POINT('Ctrl Pts',(-64.8993383270352,7.94603558521596,-17.7629146706841));
#29772=CARTESIAN_POINT('Ctrl Pts',(-64.8917663759709,7.95771535157678,-17.8627678181602));
#29773=CARTESIAN_POINT('Ctrl Pts',(-64.87829843768,7.97934358488809,-18.0718376780894));
#29774=CARTESIAN_POINT('Ctrl Pts',(-64.8675416986687,7.99634477320552,-18.2813039514666));
#29775=CARTESIAN_POINT('Ctrl Pts',(-64.8591829295582,8.00964496385992,-18.4954415917632));
#29776=CARTESIAN_POINT('Ctrl Pts',(-64.8549247713441,8.0163398028745,-18.6303160118129));
#29777=CARTESIAN_POINT('Ctrl Pts',(-64.8520602728037,8.02081409894711,-18.7391625487916));
#29778=CARTESIAN_POINT('Ctrl Pts',(-64.8495487097806,8.02469632094482,-18.8485295460239));
#29779=CARTESIAN_POINT('Ctrl Pts',(-64.8440461098093,8.03303268000617,-19.1515639158718));
#29780=CARTESIAN_POINT('Ctrl Pts',(-64.8422307342923,8.03444083547476,-19.660002172546));
#29781=CARTESIAN_POINT('Ctrl Pts',(-64.8535639039286,8.01101137755237,-20.5996246908767));
#29782=CARTESIAN_POINT('Ctrl Pts',(-64.8837685193248,7.95104762462188,-21.8412729116947));
#29783=CARTESIAN_POINT('Ctrl Pts',(-64.9003385408341,7.91656250618651,-22.9055157959435));
#29784=CARTESIAN_POINT('Ctrl Pts',(-64.9002603399163,7.91612971996068,-23.5899652055116));
#29785=CARTESIAN_POINT('Ctrl Pts',(-64.9002853704511,7.91597419274655,-23.8329246327572));
#29786=CARTESIAN_POINT('Ctrl Pts',(-64.9005209396592,7.91570372462549,-24.3354228327737));
#29787=CARTESIAN_POINT('Ctrl Pts',(-64.9013496705288,7.91533419006428,-25.2086189396213));
#29788=CARTESIAN_POINT('Ctrl Pts',(-64.9032377813096,7.91505426902946,-26.4649260715607));
#29789=CARTESIAN_POINT('Ctrl Pts',(-64.9051420818175,7.91497359547895,-27.9727284482595));
#29790=CARTESIAN_POINT('Ctrl Pts',(-64.9051740451273,7.91509119634508,-28.977928229516));
#29791=CARTESIAN_POINT('Ctrl Pts',(-64.9045909343935,7.91517658969557,-29.542350523228));
#29792=CARTESIAN_POINT('Ctrl Pts',(-64.9044396788063,7.9151974629864,-29.6678590219361));
#29793=CARTESIAN_POINT('Ctrl Pts',(-64.9040502584897,7.91524698093661,-29.9188765931247));
#29794=CARTESIAN_POINT('Ctrl Pts',(-64.9031570090159,7.91535731016294,-30.3582616791647));
#29795=CARTESIAN_POINT('Ctrl Pts',(-64.9006542075357,7.91565738205601,-31.2372934259634));
#29796=CARTESIAN_POINT('Ctrl Pts',(-64.896738035002,7.91617210820649,-32.241954517403));
#29797=CARTESIAN_POINT('Ctrl Pts',(-64.8929410178614,7.91678557699602,-33.2456522570364));
#29798=CARTESIAN_POINT('Ctrl Pts',(-64.8904447143674,7.91727679017316,-33.9976902843502));
#29799=CARTESIAN_POINT('Ctrl Pts',(-64.8885837756887,7.91779832763919,-34.7485988495637));
#29800=CARTESIAN_POINT('Ctrl Pts',(-64.8879625001898,7.91814877453707,-35.2483027153575));
#29801=CARTESIAN_POINT('Ctrl Pts',(-64.8878017993677,7.91840737253542,-35.6236749304173));
#29802=CARTESIAN_POINT('Ctrl Pts',(-64.8877802039006,7.91856704600513,-35.8749658786825));
#29803=CARTESIAN_POINT('Ctrl Pts',(-64.8880462852168,7.9188457091825,-36.3770736455709));
#29804=CARTESIAN_POINT('Ctrl Pts',(-64.8892204145641,7.91926455578023,-37.2544471887489));
#29805=CARTESIAN_POINT('Ctrl Pts',(-64.8936647430139,7.9200396565448,-39.0063061870146));
#29806=CARTESIAN_POINT('Ctrl Pts',(-64.8984157168729,7.92143147742256,-40.509206742286));
#29807=CARTESIAN_POINT('Ctrl Pts',(-64.8998413822583,7.92366309995064,-41.6425605863139));
#29808=CARTESIAN_POINT('Ctrl Pts',(-64.9000866589177,7.92398502833008,-41.8904057678773));
#29809=CARTESIAN_POINT('Ctrl Pts',(-64.9002737319323,7.92407597064351,-42.2644534304189));
#29810=CARTESIAN_POINT('Ctrl Pts',(-64.9003153064097,7.92387393480418,-42.6389519048891));
#29811=CARTESIAN_POINT('Ctrl Pts',(-64.9002215464106,7.92335187953369,-43.1396736261026));
#29812=CARTESIAN_POINT('Ctrl Pts',(-64.8999102341496,7.92248272763674,-43.7674421035051));
#29813=CARTESIAN_POINT('Ctrl Pts',(-64.899497759237,7.92192117742467,-44.5234680179482));
#29814=CARTESIAN_POINT('Ctrl Pts',(-64.899347390088,7.92254946999201,-45.1552451948918));
#29815=CARTESIAN_POINT('Ctrl Pts',(-64.8994781936819,7.92413700201671,-45.6614762962492));
#29816=CARTESIAN_POINT('Ctrl Pts',(-64.8997354762577,7.92597313553899,-46.0415025358713));
#29817=CARTESIAN_POINT('Ctrl Pts',(-64.9001857038644,7.92856083162908,-46.421796828405));
#29818=CARTESIAN_POINT('Ctrl Pts',(-64.9010872471559,7.93316033089061,-46.929200310135));
#29819=CARTESIAN_POINT('Ctrl Pts',(-64.9021548477992,7.9380492543922,-47.3098695287838));
#29820=CARTESIAN_POINT('Ctrl Pts',(-64.9035504526263,7.94414913770834,-47.6919428942751));
#29821=CARTESIAN_POINT('Ctrl Pts',(-64.9045064456491,7.94995809963907,-47.9608562576491));
#29822=CARTESIAN_POINT('Ctrl Pts',(-64.9066519832131,7.96638697291171,-48.4855609721244));
#29823=CARTESIAN_POINT('Ctrl Pts',(-64.9109876462315,8.00543160879661,-49.3944875787079));
#29824=CARTESIAN_POINT('Ctrl Pts',(-64.9189903444601,8.0749488016112,-50.6516519938867));
#29825=CARTESIAN_POINT('Ctrl Pts',(-64.9311863309774,8.13570078670839,-52.0986881422973));
#29826=CARTESIAN_POINT('Ctrl Pts',(-64.9404083729074,8.13464902825682,-53.0195058759792));
#29827=CARTESIAN_POINT('Ctrl Pts',(-64.9461372024873,8.11398242139807,-53.5814415216747));
#29828=CARTESIAN_POINT('Ctrl Pts',(-64.9483487490898,8.1028928551161,-53.7803715381629));
#29829=CARTESIAN_POINT('Ctrl Pts',(-64.9531816256131,8.06580685780084,-54.2112458480708));
#29830=CARTESIAN_POINT('Ctrl Pts',(-64.9628262208506,7.96642573989521,-54.9958597311264));
#29831=CARTESIAN_POINT('Ctrl Pts',(-64.9868870921632,7.672416767481,-56.7174028589548));
#29832=CARTESIAN_POINT('Ctrl Pts',(-65.0139477942561,7.41958191668347,-58.4304548950946));
#29833=CARTESIAN_POINT('Ctrl Pts',(-65.0196865912844,7.49908850817287,-59.7667398161207));
#29834=CARTESIAN_POINT('Ctrl Pts',(-65.020481436181,7.50867553992863,-59.9086131229831));
#29835=CARTESIAN_POINT('Ctrl Pts',(-65.0217813215993,7.53242952457539,-60.2027427012463));
#29836=CARTESIAN_POINT('Ctrl Pts',(-65.023594649291,7.58377340038694,-60.7090829018234));
#29837=CARTESIAN_POINT('Ctrl Pts',(-65.0253943628937,7.72466231531237,-61.7149615900748));
#29838=CARTESIAN_POINT('Ctrl Pts',(-65.0243823691169,7.96159119512331,-62.8351398823737));
#29839=CARTESIAN_POINT('Ctrl Pts',(-65.0220992216398,8.25460190105227,-63.9273046292012));
#29840=CARTESIAN_POINT('Ctrl Pts',(-65.0206361906803,8.43699629962348,-64.530160675701));
#29841=CARTESIAN_POINT('Ctrl Pts',(-65.0197085039787,8.56449059280231,-64.9272980267861));
#29842=CARTESIAN_POINT('Ctrl Pts',(-65.0191104802244,8.65096692107261,-65.1907272591478));
#29843=CARTESIAN_POINT('Ctrl Pts',(-65.018550261451,8.73955692474373,-65.4522913336752));
#29844=CARTESIAN_POINT('Ctrl Pts',(-65.018117988003,8.81864760344354,-65.6793561212113));
#29845=CARTESIAN_POINT('Ctrl Pts',(-65.0178900129609,8.86426034018339,-65.8085979580986));
#29846=CARTESIAN_POINT('Ctrl Pts',(-65.0175669761628,8.93309138951526,-66.0019756870505));
#29847=CARTESIAN_POINT('Ctrl Pts',(-65.0173448198335,8.99123936368044,-66.1620262154104));
#29848=CARTESIAN_POINT('Ctrl Pts',(-65.0170182798613,9.08863836597457,-66.4262390909692));
#29849=CARTESIAN_POINT('Ctrl Pts',(-65.0149069291614,9.20600383637598,-66.7306832709554));
#29850=CARTESIAN_POINT('Ctrl Pts',(-65.0116654762018,9.44804813625744,-67.3073862996916));
#29851=CARTESIAN_POINT('Ctrl Pts',(-65.0057472173816,9.90725703304797,-68.2956966704029));
#29852=CARTESIAN_POINT('Ctrl Pts',(-64.9970218138309,10.9082659234554,-70.1536088847422));
#29853=CARTESIAN_POINT('Ctrl Pts',(-64.9975725442118,11.7837973669017,-71.6138988712409));
#29854=CARTESIAN_POINT('Ctrl Pts',(-65.0029615035976,12.3378656929601,-72.6662798162345));
#29855=CARTESIAN_POINT('Ctrl Pts',(-65.0024890581818,12.4735259545828,-72.9239616761582));
#29856=CARTESIAN_POINT('Ctrl Pts',(-65.0025241219137,12.7383580418874,-73.4255354309714));
#29857=CARTESIAN_POINT('Ctrl Pts',(-65.0022053822186,13.0729224209133,-74.057277442144));
#29858=CARTESIAN_POINT('Ctrl Pts',(-65.0020916724498,13.4736037880218,-74.8111709421753));
#29859=CARTESIAN_POINT('Ctrl Pts',(-65.0018405734174,14.2767237520025,-76.3187381452471));
#29860=CARTESIAN_POINT('Ctrl Pts',(-65.0018764663666,14.9461187817725,-77.5712949176202));
#29861=CARTESIAN_POINT('Ctrl Pts',(-65.002139456689,15.914055900774,-79.3918586263518));
#29862=CARTESIAN_POINT('Ctrl Pts',(-65.0020250127354,16.3513988662646,-80.214517422021));
#29863=CARTESIAN_POINT('Ctrl Pts',(-65.0020250127364,16.7879204536536,-81.0354951241211));
#29864=CARTESIAN_POINT('Ctrl Pts',(-62.2324116460955,2.65110845064529,24.8313037818064));
#29865=CARTESIAN_POINT('Ctrl Pts',(-62.2325721397915,2.65111459129155,24.7824460238289));
#29866=CARTESIAN_POINT('Ctrl Pts',(-62.2327405043154,2.65112099191732,24.73358971044));
#29867=CARTESIAN_POINT('Ctrl Pts',(-62.2347287307477,2.6511997461256,24.1832352226466));
#29868=CARTESIAN_POINT('Ctrl Pts',(-62.2357093212771,2.65089278229138,23.1793101976511));
#29869=CARTESIAN_POINT('Ctrl Pts',(-62.2376383378861,2.64989439785791,21.1712233896418));
#29870=CARTESIAN_POINT('Ctrl Pts',(-62.2508930908442,2.65046521052102,19.6674111041318));
#29871=CARTESIAN_POINT('Ctrl Pts',(-62.2817163866741,2.65351012755467,18.4166246433661));
#29872=CARTESIAN_POINT('Ctrl Pts',(-62.2963498662037,2.65475210555508,17.9154924339037));
#29873=CARTESIAN_POINT('Ctrl Pts',(-62.3328704055141,2.65747355900587,16.9126547008369));
#29874=CARTESIAN_POINT('Ctrl Pts',(-62.4114012635184,2.66334020002405,15.1583826347409));
#29875=CARTESIAN_POINT('Ctrl Pts',(-62.4886607515688,2.67186631265648,13.6513035950692));
#29876=CARTESIAN_POINT('Ctrl Pts',(-62.5416546928848,2.68272729508388,12.3900260632852));
#29877=CARTESIAN_POINT('Ctrl Pts',(-62.5639055963637,2.68778477047206,11.8862901822519));
#29878=CARTESIAN_POINT('Ctrl Pts',(-62.6111307572197,2.70009687692735,10.8805271797224));
#29879=CARTESIAN_POINT('Ctrl Pts',(-62.6965536074913,2.72558808356462,9.12351965611986));
#29880=CARTESIAN_POINT('Ctrl Pts',(-62.7597622091768,2.74792172877984,7.62112790962481));
#29881=CARTESIAN_POINT('Ctrl Pts',(-62.7870470844756,2.75842119570929,6.49441772086995));
#29882=CARTESIAN_POINT('Ctrl Pts',(-62.7926887858624,2.76084923498194,6.24239217728173));
#29883=CARTESIAN_POINT('Ctrl Pts',(-62.8024673870572,2.76583093688162,5.73982653503197));
#29884=CARTESIAN_POINT('Ctrl Pts',(-62.8158649336197,2.77467005108555,4.85939849009647));
#29885=CARTESIAN_POINT('Ctrl Pts',(-62.8293424671233,2.79097056893532,3.10187317395191));
#29886=CARTESIAN_POINT('Ctrl Pts',(-62.8245365118151,2.79542564198213,1.60674978984311));
#29887=CARTESIAN_POINT('Ctrl Pts',(-62.8215989110629,2.79042377416418,0.562687943733352));
#29888=CARTESIAN_POINT('Ctrl Pts',(-62.8210181295631,2.78909536304729,0.458688210000553));
#29889=CARTESIAN_POINT('Ctrl Pts',(-62.819099431748,2.78353737887463,0.235639356286997));
#29890=CARTESIAN_POINT('Ctrl Pts',(-62.8139133497516,2.76682228410439,-0.156856655635209));
#29891=CARTESIAN_POINT('Ctrl Pts',(-62.8023804930994,2.7264976388699,-0.744805113266516));
#29892=CARTESIAN_POINT('Ctrl Pts',(-62.7849338452555,2.66393700041982,-1.4860279378941));
#29893=CARTESIAN_POINT('Ctrl Pts',(-62.7601070118959,2.58128821569208,-2.52537755151352));
#29894=CARTESIAN_POINT('Ctrl Pts',(-62.7319192302486,2.51604604164048,-3.91937798362081));
#29895=CARTESIAN_POINT('Ctrl Pts',(-62.7291090615613,2.61098576196056,-5.14442232357788));
#29896=CARTESIAN_POINT('Ctrl Pts',(-62.7362675602417,2.75758588449044,-5.93636656089618));
#29897=CARTESIAN_POINT('Ctrl Pts',(-62.7417753230037,2.82176011428813,-6.2451480087076));
#29898=CARTESIAN_POINT('Ctrl Pts',(-62.7599177726702,2.97657823602182,-6.85273841030402));
#29899=CARTESIAN_POINT('Ctrl Pts',(-62.8061257130493,3.30597747396704,-7.8806422937015));
#29900=CARTESIAN_POINT('Ctrl Pts',(-62.886404686147,3.89707297725855,-9.25228695764434));
#29901=CARTESIAN_POINT('Ctrl Pts',(-62.9397838682818,4.52675217606724,-10.5119105373165));
#29902=CARTESIAN_POINT('Ctrl Pts',(-62.9483184928025,4.9285398956449,-11.3479111829804));
#29903=CARTESIAN_POINT('Ctrl Pts',(-62.9426336815654,5.1384643004547,-11.8136597118286));
#29904=CARTESIAN_POINT('Ctrl Pts',(-62.9358884122851,5.23527166805804,-12.0423095827426));
#29905=CARTESIAN_POINT('Ctrl Pts',(-62.9289577891853,5.30491065956518,-12.2140201328765));
#29906=CARTESIAN_POINT('Ctrl Pts',(-62.9178577373982,5.36388019644879,-12.3629837700079));
#29907=CARTESIAN_POINT('Ctrl Pts',(-62.8961711642207,5.47660176938199,-12.638967148117));
#29908=CARTESIAN_POINT('Ctrl Pts',(-62.8501277346565,5.68011028976417,-13.1247575937463));
#29909=CARTESIAN_POINT('Ctrl Pts',(-62.7055635225399,6.20984207111696,-14.3304093147106));
#29910=CARTESIAN_POINT('Ctrl Pts',(-62.4912627490231,6.78243277690134,-15.5747311231459));
#29911=CARTESIAN_POINT('Ctrl Pts',(-62.2993265658437,7.20732218206552,-16.6805172535131));
#29912=CARTESIAN_POINT('Ctrl Pts',(-62.2163843982636,7.37604048928846,-17.1955856354033));
#29913=CARTESIAN_POINT('Ctrl Pts',(-62.1634884800495,7.48082183634278,-17.5834150637111));
#29914=CARTESIAN_POINT('Ctrl Pts',(-62.1425816155528,7.52290086798551,-17.7693030685432));
#29915=CARTESIAN_POINT('Ctrl Pts',(-62.1294522822413,7.55032238942497,-17.9052459033932));
#29916=CARTESIAN_POINT('Ctrl Pts',(-62.1211689409812,7.56758257430452,-17.9980979081998));
#29917=CARTESIAN_POINT('Ctrl Pts',(-62.1060500048589,7.5981531301875,-18.1847897844285));
#29918=CARTESIAN_POINT('Ctrl Pts',(-62.0930999650027,7.62314067975387,-18.3759185051838));
#29919=CARTESIAN_POINT('Ctrl Pts',(-62.0822251853017,7.64282104746964,-18.5711850893019));
#29920=CARTESIAN_POINT('Ctrl Pts',(-62.0762634979292,7.65299423254032,-18.6951881969995));
#29921=CARTESIAN_POINT('Ctrl Pts',(-62.0719773774967,7.65989572394792,-18.7955493623822));
#29922=CARTESIAN_POINT('Ctrl Pts',(-62.0680067906211,7.66598680920003,-18.8967172340001));
#29923=CARTESIAN_POINT('Ctrl Pts',(-62.0583511170679,7.6794882188253,-19.1781798294307));
#29924=CARTESIAN_POINT('Ctrl Pts',(-62.049173484007,7.68432097683299,-19.6572751966255));
#29925=CARTESIAN_POINT('Ctrl Pts',(-62.0471367134705,7.65430605731816,-20.5627028716984));
#29926=CARTESIAN_POINT('Ctrl Pts',(-62.0621562669111,7.56706421088203,-21.7946503974307));
#29927=CARTESIAN_POINT('Ctrl Pts',(-62.0707069159192,7.51367694952985,-22.8859623592707));
#29928=CARTESIAN_POINT('Ctrl Pts',(-62.0669229094418,7.51418611686719,-23.597568395228));
#29929=CARTESIAN_POINT('Ctrl Pts',(-62.065605431171,7.51428478253497,-23.8360696907441));
#29930=CARTESIAN_POINT('Ctrl Pts',(-62.0636147430115,7.51423124901991,-24.3384868425194));
#29931=CARTESIAN_POINT('Ctrl Pts',(-62.0616369095894,7.51353706611234,-25.2077394126351));
#29932=CARTESIAN_POINT('Ctrl Pts',(-62.0621090978214,7.51150180454813,-26.4627222976647));
#29933=CARTESIAN_POINT('Ctrl Pts',(-62.0648367787779,7.50912327519382,-27.9703278206264));
#29934=CARTESIAN_POINT('Ctrl Pts',(-62.0659098354568,7.50876672027581,-28.977760419241));
#29935=CARTESIAN_POINT('Ctrl Pts',(-62.0656790575361,7.50920693270786,-29.5438819590241));
#29936=CARTESIAN_POINT('Ctrl Pts',(-62.0656177966565,7.50931408197146,-29.6694987037349));
#29937=CARTESIAN_POINT('Ctrl Pts',(-62.0654621999351,7.5095788375689,-29.9208665818703));
#29938=CARTESIAN_POINT('Ctrl Pts',(-62.0651093215757,7.51016803327878,-30.3607331353584));
#29939=CARTESIAN_POINT('Ctrl Pts',(-62.0641551731755,7.51178083024612,-31.240593906287));
#29940=CARTESIAN_POINT('Ctrl Pts',(-62.0628134847873,7.51438388641435,-32.2457143097902));
#29941=CARTESIAN_POINT('Ctrl Pts',(-62.0618681293102,7.51721372304941,-33.2494668011189));
#29942=CARTESIAN_POINT('Ctrl Pts',(-62.0615205358396,7.51932631930793,-34.0013374152957));
#29943=CARTESIAN_POINT('Ctrl Pts',(-62.0616936586103,7.52133866738401,-34.7518363686095));
#29944=CARTESIAN_POINT('Ctrl Pts',(-62.0622663291613,7.52252721087467,-35.2511136693746));
#29945=CARTESIAN_POINT('Ctrl Pts',(-62.0629101197002,7.52333089608969,-35.6261195896978));
#29946=CARTESIAN_POINT('Ctrl Pts',(-62.0634331347508,7.52385463467722,-35.877425253617));
#29947=CARTESIAN_POINT('Ctrl Pts',(-62.0648031724192,7.52484270348859,-36.3794168797089));
#29948=CARTESIAN_POINT('Ctrl Pts',(-62.0679373960044,7.52647752632453,-37.256631961613));
#29949=CARTESIAN_POINT('Ctrl Pts',(-62.0762769369191,7.52947490759239,-39.0081317353124));
#29950=CARTESIAN_POINT('Ctrl Pts',(-62.0839209340646,7.53243636888415,-40.5106582147728));
#29951=CARTESIAN_POINT('Ctrl Pts',(-62.0868630236698,7.53555378748421,-41.643760836828));
#29952=CARTESIAN_POINT('Ctrl Pts',(-62.0874273668624,7.53606057387757,-41.8915881473257));
#29953=CARTESIAN_POINT('Ctrl Pts',(-62.0880498730019,7.53641673401846,-42.2655841484734));
#29954=CARTESIAN_POINT('Ctrl Pts',(-62.0884866387515,7.53646362757138,-42.6400314646002));
#29955=CARTESIAN_POINT('Ctrl Pts',(-62.0888701132174,7.53625336732302,-43.140671625036));
#29956=CARTESIAN_POINT('Ctrl Pts',(-62.0890699171536,7.53573296320779,-43.7683224820626));
#29957=CARTESIAN_POINT('Ctrl Pts',(-62.0891578668796,7.53552039690406,-44.524175919851));
#29958=CARTESIAN_POINT('Ctrl Pts',(-62.0893502736129,7.536377762892,-45.1557818376054));
#29959=CARTESIAN_POINT('Ctrl Pts',(-62.0897244006286,7.53810558976392,-45.6618674023183));
#29960=CARTESIAN_POINT('Ctrl Pts',(-62.0901508967091,7.54002629110324,-46.0417759029264));
#29961=CARTESIAN_POINT('Ctrl Pts',(-62.0907601063011,7.54267683770331,-46.4219444887662));
#29962=CARTESIAN_POINT('Ctrl Pts',(-62.0918650416074,7.54733023970297,-46.9291720541025));
#29963=CARTESIAN_POINT('Ctrl Pts',(-62.0930765605595,7.5522247703068,-47.3096923642799));
#29964=CARTESIAN_POINT('Ctrl Pts',(-62.0946204356517,7.55830553645758,-47.6916126248667));
#29965=CARTESIAN_POINT('Ctrl Pts',(-62.0956611667417,7.56408453136268,-47.9603797374788));
#29966=CARTESIAN_POINT('Ctrl Pts',(-62.0979298173075,7.58040451923821,-48.484847683365));
#29967=CARTESIAN_POINT('Ctrl Pts',(-62.1023740335685,7.61914468203589,-49.3934143881785));
#29968=CARTESIAN_POINT('Ctrl Pts',(-62.1103226825369,7.6879833924317,-50.6502627707064));
#29969=CARTESIAN_POINT('Ctrl Pts',(-62.1224187636886,7.74780400354067,-52.0972031986658));
#29970=CARTESIAN_POINT('Ctrl Pts',(-62.1317313561632,7.74616485099686,-53.0181336935282));
#29971=CARTESIAN_POINT('Ctrl Pts',(-62.1376297068955,7.72518476543617,-53.5801910295628));
#29972=CARTESIAN_POINT('Ctrl Pts',(-62.1399046696861,7.71398366576932,-53.7790286012338));
#29973=CARTESIAN_POINT('Ctrl Pts',(-62.1448964229361,7.67663304624389,-54.2098230859811));
#29974=CARTESIAN_POINT('Ctrl Pts',(-62.1548922339695,7.57671267544599,-54.9943108853671));
#29975=CARTESIAN_POINT('Ctrl Pts',(-62.1800038589513,7.2814270625882,-56.7158084727673));
#29976=CARTESIAN_POINT('Ctrl Pts',(-62.2081937086557,7.02731042184774,-58.429179473639));
#29977=CARTESIAN_POINT('Ctrl Pts',(-62.2144449752503,7.10646103808188,-59.766067468225));
#29978=CARTESIAN_POINT('Ctrl Pts',(-62.2153030164495,7.11601834418123,-59.9080059625841));
#29979=CARTESIAN_POINT('Ctrl Pts',(-62.2167297222136,7.13972355599113,-60.2022626238786));
#29980=CARTESIAN_POINT('Ctrl Pts',(-62.2187665552171,7.19102217448749,-60.7088053903155));
#29981=CARTESIAN_POINT('Ctrl Pts',(-62.2210163954321,7.33194976055543,-61.715014065663));
#29982=CARTESIAN_POINT('Ctrl Pts',(-62.2205026710733,7.56912629243654,-62.8353909891454));
#29983=CARTESIAN_POINT('Ctrl Pts',(-62.2186612717354,7.8624139680061,-63.9275925239715));
#29984=CARTESIAN_POINT('Ctrl Pts',(-62.2174192902535,8.04494851939812,-64.5304136453842));
#29985=CARTESIAN_POINT('Ctrl Pts',(-62.2166251202074,8.17251782148038,-64.9275067360983));
#29986=CARTESIAN_POINT('Ctrl Pts',(-62.216112444219,8.25903875171922,-65.1909008318996));
#29987=CARTESIAN_POINT('Ctrl Pts',(-62.2156312875442,8.34766383541202,-65.4524219722881));
#29988=CARTESIAN_POINT('Ctrl Pts',(-62.2152629695985,8.42677531857576,-65.6794422088368));
#29989=CARTESIAN_POINT('Ctrl Pts',(-62.2150699342168,8.47239682514454,-65.8086566631671));
#29990=CARTESIAN_POINT('Ctrl Pts',(-62.2147976898575,8.5412378240164,-66.0019914631938));
#29991=CARTESIAN_POINT('Ctrl Pts',(-62.2146142754426,8.5993869780191,-66.162002122305));
#29992=CARTESIAN_POINT('Ctrl Pts',(-62.2143468843432,8.69677781918142,-66.4261453563042));
#29993=CARTESIAN_POINT('Ctrl Pts',(-62.2122663839657,8.81415583938044,-66.7305933363832));
#29994=CARTESIAN_POINT('Ctrl Pts',(-62.2090735544206,9.05620581596369,-67.3072656757735));
#29995=CARTESIAN_POINT('Ctrl Pts',(-62.2031748317925,9.5154173411655,-68.2955530744696));
#29996=CARTESIAN_POINT('Ctrl Pts',(-62.1943357086957,10.5163936607581,-70.153431298556));
#29997=CARTESIAN_POINT('Ctrl Pts',(-62.1947416310962,11.3919028550599,-71.6137289819733));
#29998=CARTESIAN_POINT('Ctrl Pts',(-62.2001962725638,11.9460021900826,-72.6661254193472));
#29999=CARTESIAN_POINT('Ctrl Pts',(-62.1997204158704,12.0816609576166,-72.9238046059287));
#30000=CARTESIAN_POINT('Ctrl Pts',(-62.1997582965951,12.3464942952452,-73.4253768077921));
#30001=CARTESIAN_POINT('Ctrl Pts',(-62.1994376115016,12.6810575192846,-74.0571160945943));
#30002=CARTESIAN_POINT('Ctrl Pts',(-62.1993228596895,13.0817376901225,-74.8110077756463));
#30003=CARTESIAN_POINT('Ctrl Pts',(-62.1990669571479,13.8848537478945,-76.3185723843615));
#30004=CARTESIAN_POINT('Ctrl Pts',(-62.199097855418,14.5542456499623,-77.5711307629764));
#30005=CARTESIAN_POINT('Ctrl Pts',(-62.1993629968978,15.5221856398195,-79.3916987431088));
#30006=CARTESIAN_POINT('Ctrl Pts',(-62.1992471601886,15.9595275657022,-80.2143563979817));
#30007=CARTESIAN_POINT('Ctrl Pts',(-62.1992471601874,16.3960491530911,-81.0353341000812));
#30008=CARTESIAN_POINT('Ctrl Pts',(-59.4327183968758,2.25265122839169,24.8301364387822));
#30009=CARTESIAN_POINT('Ctrl Pts',(-59.4328841937094,2.25268691728004,24.7812415405472));
#30010=CARTESIAN_POINT('Ctrl Pts',(-59.4330580820664,2.25272429091666,24.7323473839837));
#30011=CARTESIAN_POINT('Ctrl Pts',(-59.4351118929449,2.25316729281828,24.181557485228));
#30012=CARTESIAN_POINT('Ctrl Pts',(-59.4365199278218,2.25376169001701,23.1771798534974));
#30013=CARTESIAN_POINT('Ctrl Pts',(-59.4396851090642,2.25528174738086,21.1682661339047));
#30014=CARTESIAN_POINT('Ctrl Pts',(-59.4533606108111,2.2582303591568,19.6641194136807));
#30015=CARTESIAN_POINT('Ctrl Pts',(-59.4831968696484,2.2632273018724,18.4131228363522));
#30016=CARTESIAN_POINT('Ctrl Pts',(-59.497368126688,2.26566892316074,17.9095299972916));
#30017=CARTESIAN_POINT('Ctrl Pts',(-59.5326978095034,2.27187083435169,16.9049738880677));
#30018=CARTESIAN_POINT('Ctrl Pts',(-59.6084620857887,2.28508910550582,15.1511096465538));
#30019=CARTESIAN_POINT('Ctrl Pts',(-59.6821606761099,2.29665137446202,13.6519191726693));
#30020=CARTESIAN_POINT('Ctrl Pts',(-59.7316230694136,2.30215371628457,12.400859407766));
#30021=CARTESIAN_POINT('Ctrl Pts',(-59.7521813816238,2.30419407380517,11.9013091163657));
#30022=CARTESIAN_POINT('Ctrl Pts',(-59.7951806640273,2.3076825131878,10.9016060004854));
#30023=CARTESIAN_POINT('Ctrl Pts',(-59.8719170049596,2.31235757963235,9.15030985240725));
#30024=CARTESIAN_POINT('Ctrl Pts',(-59.9284132374623,2.31423800236438,7.6443731963254));
#30025=CARTESIAN_POINT('Ctrl Pts',(-59.9544516997608,2.31509003621762,6.51126513178353));
#30026=CARTESIAN_POINT('Ctrl Pts',(-59.9599724708233,2.31518615800477,6.26176931787532));
#30027=CARTESIAN_POINT('Ctrl Pts',(-59.9701066362838,2.31511912260337,5.76118798583747));
#30028=CARTESIAN_POINT('Ctrl Pts',(-59.985437551415,2.31443601950404,4.8834987973579));
#30029=CARTESIAN_POINT('Ctrl Pts',(-60.0066383182567,2.31167052195812,3.1220569861816));
#30030=CARTESIAN_POINT('Ctrl Pts',(-60.0081640503809,2.31040451558357,1.61015252279124));
#30031=CARTESIAN_POINT('Ctrl Pts',(-60.0000054475934,2.31150617065875,0.547312270279649));
#30032=CARTESIAN_POINT('Ctrl Pts',(-59.9987719429314,2.3111616664216,0.432624314911944));
#30033=CARTESIAN_POINT('Ctrl Pts',(-59.9952824755793,2.30882437674471,0.194796398774891));
#30034=CARTESIAN_POINT('Ctrl Pts',(-59.9867324525885,2.30077823544184,-0.22188029869997));
#30035=CARTESIAN_POINT('Ctrl Pts',(-59.968749323234,2.280413820143,-0.830816811594355));
#30036=CARTESIAN_POINT('Ctrl Pts',(-59.9419776451423,2.24997017244242,-1.58054524315636));
#30037=CARTESIAN_POINT('Ctrl Pts',(-59.9045143667982,2.21331131315166,-2.60838361836337));
#30038=CARTESIAN_POINT('Ctrl Pts',(-59.8638638844383,2.1982498490195,-3.94729265834799));
#30039=CARTESIAN_POINT('Ctrl Pts',(-59.8547815312505,2.27162886589833,-5.07663826581443));
#30040=CARTESIAN_POINT('Ctrl Pts',(-59.8613065919288,2.36144504095905,-5.79808564937288));
#30041=CARTESIAN_POINT('Ctrl Pts',(-59.8668073479993,2.3953383972358,-6.05856085757831));
#30042=CARTESIAN_POINT('Ctrl Pts',(-59.8857885375052,2.47309818412149,-6.59755722116751));
#30043=CARTESIAN_POINT('Ctrl Pts',(-59.9370211914893,2.6300323610067,-7.53693441067443));
#30044=CARTESIAN_POINT('Ctrl Pts',(-60.0379558361062,2.9292811235094,-8.89353202373783));
#30045=CARTESIAN_POINT('Ctrl Pts',(-60.1099319053602,3.331710665947,-10.2468365016121));
#30046=CARTESIAN_POINT('Ctrl Pts',(-60.1185712193049,3.65741659751785,-11.1941046587181));
#30047=CARTESIAN_POINT('Ctrl Pts',(-60.1089528756095,3.85487089909554,-11.7360668264736));
#30048=CARTESIAN_POINT('Ctrl Pts',(-60.098819916929,3.95714002352826,-12.0071712114592));
#30049=CARTESIAN_POINT('Ctrl Pts',(-60.0888815169619,4.03583095585652,-12.2124781488849));
#30050=CARTESIAN_POINT('Ctrl Pts',(-60.0770949409152,4.10160480095275,-12.3804934812964));
#30051=CARTESIAN_POINT('Ctrl Pts',(-60.0533580255542,4.23333443500919,-12.6916634318784));
#30052=CARTESIAN_POINT('Ctrl Pts',(-60.0048392844905,4.48159518374812,-13.2286868483013));
#30053=CARTESIAN_POINT('Ctrl Pts',(-59.8591850430779,5.17319095150817,-14.520799126474));
#30054=CARTESIAN_POINT('Ctrl Pts',(-59.6737622709758,6.00239532719331,-15.7921178849206));
#30055=CARTESIAN_POINT('Ctrl Pts',(-59.5263695708326,6.61087952197628,-16.8978869745208));
#30056=CARTESIAN_POINT('Ctrl Pts',(-59.4652314700135,6.84135119363707,-17.3943244839072));
#30057=CARTESIAN_POINT('Ctrl Pts',(-59.4268061379572,6.97398181241572,-17.749766802165));
#30058=CARTESIAN_POINT('Ctrl Pts',(-59.4114107075389,7.02319302665999,-17.9115482795378));
#30059=CARTESIAN_POINT('Ctrl Pts',(-59.4014828487707,7.05388792561121,-18.0266474181241));
#30060=CARTESIAN_POINT('Ctrl Pts',(-59.3941817272012,7.07706386164247,-18.1188593896414));
#30061=CARTESIAN_POINT('Ctrl Pts',(-59.3804739949598,7.11648356283556,-18.29613591791));
#30062=CARTESIAN_POINT('Ctrl Pts',(-59.3672224174604,7.15029696899006,-18.4802941344704));
#30063=CARTESIAN_POINT('Ctrl Pts',(-59.3547804174123,7.17765498290196,-18.6669857253199));
#30064=CARTESIAN_POINT('Ctrl Pts',(-59.3472910192631,7.19246010955654,-18.7859857007086));
#30065=CARTESIAN_POINT('Ctrl Pts',(-59.3415001550889,7.20287995318006,-18.8822616582977));
#30066=CARTESIAN_POINT('Ctrl Pts',(-59.3358379461214,7.2124026048674,-18.9794207952203));
#30067=CARTESIAN_POINT('Ctrl Pts',(-59.3208037727125,7.23494416667871,-19.2500086791216));
#30068=CARTESIAN_POINT('Ctrl Pts',(-59.2992833716582,7.25249328063318,-19.7128242023755));
#30069=CARTESIAN_POINT('Ctrl Pts',(-59.2695945378286,7.23965402392194,-20.5959818589974));
#30070=CARTESIAN_POINT('Ctrl Pts',(-59.2466024375903,7.16395890440845,-21.8137011452256));
#30071=CARTESIAN_POINT('Ctrl Pts',(-59.2332940311674,7.11826912985185,-22.9079220046133));
#30072=CARTESIAN_POINT('Ctrl Pts',(-59.2225001191569,7.12827400914735,-23.6256217875921));
#30073=CARTESIAN_POINT('Ctrl Pts',(-59.2188039915616,7.13106784266876,-23.8586323041846));
#30074=CARTESIAN_POINT('Ctrl Pts',(-59.2130082602853,7.13573882821156,-24.3552887653573));
#30075=CARTESIAN_POINT('Ctrl Pts',(-59.2068812440707,7.14041873824705,-25.2138947714959));
#30076=CARTESIAN_POINT('Ctrl Pts',(-59.2070806050236,7.13979394289298,-26.4598831298544));
#30077=CARTESIAN_POINT('Ctrl Pts',(-59.2140897177481,7.1334418088711,-27.9631595619088));
#30078=CARTESIAN_POINT('Ctrl Pts',(-59.2182024954926,7.13023119006006,-28.9727175728279));
#30079=CARTESIAN_POINT('Ctrl Pts',(-59.2190175697542,7.12994002465576,-29.5412710567716));
#30080=CARTESIAN_POINT('Ctrl Pts',(-59.2192156653274,7.1298651627011,-29.6660415425381));
#30081=CARTESIAN_POINT('Ctrl Pts',(-59.2196582329829,7.12967351296968,-29.9165645862029));
#30082=CARTESIAN_POINT('Ctrl Pts',(-59.220554426431,7.12924881482313,-30.3546981134225));
#30083=CARTESIAN_POINT('Ctrl Pts',(-59.2228155884173,7.12806430740016,-31.231997036665));
#30084=CARTESIAN_POINT('Ctrl Pts',(-59.2263611472526,7.12624875019509,-32.235374646439));
#30085=CARTESIAN_POINT('Ctrl Pts',(-59.2306671790479,7.12438665706793,-33.2388778049522));
#30086=CARTESIAN_POINT('Ctrl Pts',(-59.2342226046425,7.1230697283121,-33.991252883038));
#30087=CARTESIAN_POINT('Ctrl Pts',(-59.2380309975618,7.12198989860983,-34.7429353412321));
#30088=CARTESIAN_POINT('Ctrl Pts',(-59.2407050015639,7.12147796415094,-35.2434716876348));
#30089=CARTESIAN_POINT('Ctrl Pts',(-59.2427536630326,7.12118948900547,-35.6195827369635));
#30090=CARTESIAN_POINT('Ctrl Pts',(-59.2442150573129,7.12099128564165,-35.8708339979703));
#30091=CARTESIAN_POINT('Ctrl Pts',(-59.2474467172818,7.12058821018909,-36.3731721058981));
#30092=CARTESIAN_POINT('Ctrl Pts',(-59.2537730541113,7.11993596026141,-37.2507570133435));
#30093=CARTESIAN_POINT('Ctrl Pts',(-59.2681644576381,7.11887801881393,-39.0032249173688));
#30094=CARTESIAN_POINT('Ctrl Pts',(-59.2800034741358,7.11923691355807,-40.5065455567628));
#30095=CARTESIAN_POINT('Ctrl Pts',(-59.2852313137663,7.12076542512632,-41.6403302586037));
#30096=CARTESIAN_POINT('Ctrl Pts',(-59.2862818754551,7.12092781263791,-41.888235467488));
#30097=CARTESIAN_POINT('Ctrl Pts',(-59.2875768563654,7.12078174250143,-42.2624016805809));
#30098=CARTESIAN_POINT('Ctrl Pts',(-59.2886310108195,7.12034618952707,-42.6370212228559));
#30099=CARTESIAN_POINT('Ctrl Pts',(-59.2897658837102,7.1195230928026,-43.1379181986253));
#30100=CARTESIAN_POINT('Ctrl Pts',(-59.2907736735576,7.11830360101143,-43.7659242265376));
#30101=CARTESIAN_POINT('Ctrl Pts',(-59.2916324835984,7.11738837896993,-44.5222636835069));
#30102=CARTESIAN_POINT('Ctrl Pts',(-59.2923109462295,7.11779890753617,-45.1543211423264));
#30103=CARTESIAN_POINT('Ctrl Pts',(-59.2929838888716,7.11926813498271,-45.6607996901971));
#30104=CARTESIAN_POINT('Ctrl Pts',(-59.2935916966502,7.12104796186459,-46.0410174981501));
#30105=CARTESIAN_POINT('Ctrl Pts',(-59.294340782817,7.12361458503253,-46.4215103632799));
#30106=CARTESIAN_POINT('Ctrl Pts',(-59.2955772293489,7.12823787347396,-46.9291911154372));
#30107=CARTESIAN_POINT('Ctrl Pts',(-59.2968324788671,7.13320605115335,-47.3100738833494));
#30108=CARTESIAN_POINT('Ctrl Pts',(-59.298380648924,7.13943526843574,-47.6923777956218));
#30109=CARTESIAN_POINT('Ctrl Pts',(-59.2993850683031,7.14535407475583,-47.9615186873962));
#30110=CARTESIAN_POINT('Ctrl Pts',(-59.3014603118004,7.16207268876626,-48.4866017625764));
#30111=CARTESIAN_POINT('Ctrl Pts',(-59.3052865602591,7.2017946763055,-49.396129784678));
#30112=CARTESIAN_POINT('Ctrl Pts',(-59.3118230764063,7.2726255534233,-50.6539095926112));
#30113=CARTESIAN_POINT('Ctrl Pts',(-59.322062828193,7.33518684047928,-52.1012995183051));
#30114=CARTESIAN_POINT('Ctrl Pts',(-59.3304629246601,7.33527504366464,-53.0220195395743));
#30115=CARTESIAN_POINT('Ctrl Pts',(-59.3360027967414,7.31527076853847,-53.5837864300138));
#30116=CARTESIAN_POINT('Ctrl Pts',(-59.3381330872285,7.30441091804775,-53.7829838756593));
#30117=CARTESIAN_POINT('Ctrl Pts',(-59.3428400672686,7.26786582493259,-54.214103866335));
#30118=CARTESIAN_POINT('Ctrl Pts',(-59.3523721996777,7.16957046701241,-54.9990388970232));
#30119=CARTESIAN_POINT('Ctrl Pts',(-59.3768268915765,6.87830936594744,-56.7204910521529));
#30120=CARTESIAN_POINT('Ctrl Pts',(-59.4048338955237,6.62818379471605,-58.4327351631704));
#30121=CARTESIAN_POINT('Ctrl Pts',(-59.4111517886009,6.70854270234599,-59.7678509567132));
#30122=CARTESIAN_POINT('Ctrl Pts',(-59.4120270987402,6.71821730117235,-59.9096006552835));
#30123=CARTESIAN_POINT('Ctrl Pts',(-59.4135033187453,6.74212534097523,-60.2034871715157));
#30124=CARTESIAN_POINT('Ctrl Pts',(-59.4156714996854,6.79367095362047,-60.7094406835807));
#30125=CARTESIAN_POINT('Ctrl Pts',(-59.418332233718,6.93474046783409,-61.714678385153));
#30126=CARTESIAN_POINT('Ctrl Pts',(-59.4185131411126,7.17151387462809,-62.8344252992925));
#30127=CARTESIAN_POINT('Ctrl Pts',(-59.4173708025752,7.46427674420058,-63.926424678659));
#30128=CARTESIAN_POINT('Ctrl Pts',(-59.4164873159989,7.64654168063073,-64.5292836353808));
#30129=CARTESIAN_POINT('Ctrl Pts',(-59.4159032525969,7.77397218102938,-64.9264627282968));
#30130=CARTESIAN_POINT('Ctrl Pts',(-59.4155220490055,7.86041325133793,-65.1899303784133));
#30131=CARTESIAN_POINT('Ctrl Pts',(-59.4151581240536,7.94898035286396,-65.4515487293264));
#30132=CARTESIAN_POINT('Ctrl Pts',(-59.4148775961833,8.02806528514184,-65.6786752745147));
#30133=CARTESIAN_POINT('Ctrl Pts',(-59.4147301846656,8.07367923751936,-65.8079565364368));
#30134=CARTESIAN_POINT('Ctrl Pts',(-59.4145216542839,8.14251677800326,-66.0013974175857));
#30135=CARTESIAN_POINT('Ctrl Pts',(-59.4143812193172,8.20068053593941,-66.1615094745568));
#30136=CARTESIAN_POINT('Ctrl Pts',(-59.4141694508199,8.29812039206658,-66.4258331073802));
#30137=CARTESIAN_POINT('Ctrl Pts',(-59.4121184531506,8.41545564797318,-66.7302393110289));
#30138=CARTESIAN_POINT('Ctrl Pts',(-59.4089645320295,8.65747843166566,-67.306955770546));
#30139=CARTESIAN_POINT('Ctrl Pts',(-59.4030611647312,9.11662704675057,-68.295250550469));
#30140=CARTESIAN_POINT('Ctrl Pts',(-59.3940478050956,10.1175438970205,-70.1531811722962));
#30141=CARTESIAN_POINT('Ctrl Pts',(-59.3943023247525,10.9930421956565,-71.6134584512388));
#30142=CARTESIAN_POINT('Ctrl Pts',(-59.3998704182841,11.5471501024684,-72.6658363506855));
#30143=CARTESIAN_POINT('Ctrl Pts',(-59.399388093542,11.6828060367678,-72.9235197213246));
#30144=CARTESIAN_POINT('Ctrl Pts',(-59.3994301178304,11.9476378029523,-73.4250952435116));
#30145=CARTESIAN_POINT('Ctrl Pts',(-59.3991056883216,12.282199468326,-74.056839118302));
#30146=CARTESIAN_POINT('Ctrl Pts',(-59.398988815121,12.6828808223937,-74.8107345944885));
#30147=CARTESIAN_POINT('Ctrl Pts',(-59.3987246047287,13.486001590597,-76.3183046987169));
#30148=CARTESIAN_POINT('Ctrl Pts',(-59.3987492158294,14.1553988360136,-77.5708588961577));
#30149=CARTESIAN_POINT('Ctrl Pts',(-59.3990199465909,15.1233351729319,-79.3914165419536));
#30150=CARTESIAN_POINT('Ctrl Pts',(-59.3989018465541,15.5606776339371,-80.2140760951489));
#30151=CARTESIAN_POINT('Ctrl Pts',(-59.3989018465536,15.9971992213268,-81.0350537972465));
#30152=CARTESIAN_POINT('Ctrl Pts',(-56.6218988576096,1.85135975369098,24.830305945651));
#30153=CARTESIAN_POINT('Ctrl Pts',(-56.6220771208639,1.8513926526504,24.7814164126151));
#30154=CARTESIAN_POINT('Ctrl Pts',(-56.6222640626647,1.85142711473754,24.7325276510878));
#30155=CARTESIAN_POINT('Ctrl Pts',(-56.6244716173778,1.85183533087296,24.1818026226272));
#30156=CARTESIAN_POINT('Ctrl Pts',(-56.6263912846077,1.85233538215404,23.1775909603722));
#30157=CARTESIAN_POINT('Ctrl Pts',(-56.6310064059174,1.85360104451151,21.1687551199745));
#30158=CARTESIAN_POINT('Ctrl Pts',(-56.6456879014065,1.85632152046014,19.6645215090319));
#30159=CARTESIAN_POINT('Ctrl Pts',(-56.6756899000187,1.86116117020704,18.4133896817507));
#30160=CARTESIAN_POINT('Ctrl Pts',(-56.6901377902638,1.86357831767313,17.9098159767833));
#30161=CARTESIAN_POINT('Ctrl Pts',(-56.7265081026977,1.86981384748473,16.9053246703197));
#30162=CARTESIAN_POINT('Ctrl Pts',(-56.8044350008068,1.88316004226665,15.1517241446086));
#30163=CARTESIAN_POINT('Ctrl Pts',(-56.8773927397668,1.89448873086831,13.6526002138188));
#30164=CARTESIAN_POINT('Ctrl Pts',(-56.9212630953127,1.8991353139138,12.4013088335406));
#30165=CARTESIAN_POINT('Ctrl Pts',(-56.9389604936624,1.90075751887008,11.9016148655307));
#30166=CARTESIAN_POINT('Ctrl Pts',(-56.9743053171184,1.90317356758234,10.9016120674607));
#30167=CARTESIAN_POINT('Ctrl Pts',(-57.0340146008934,1.90550527661059,9.14974790695198));
#30168=CARTESIAN_POINT('Ctrl Pts',(-57.0746626133434,1.90517739105699,7.64372859243564));
#30169=CARTESIAN_POINT('Ctrl Pts',(-57.0928894575461,1.90471487948243,6.51107083885909));
#30170=CARTESIAN_POINT('Ctrl Pts',(-57.0965664867556,1.9045157299458,6.26177103197025));
#30171=CARTESIAN_POINT('Ctrl Pts',(-57.1026094896939,1.90371984972078,5.76145104809821));
#30172=CARTESIAN_POINT('Ctrl Pts',(-57.1100269856796,1.90147186159325,4.88416698235186));
#30173=CARTESIAN_POINT('Ctrl Pts',(-57.114427530443,1.89495357174928,3.12305916100058));
#30174=CARTESIAN_POINT('Ctrl Pts',(-57.1081396707823,1.89053916476324,1.61151271554119));
#30175=CARTESIAN_POINT('Ctrl Pts',(-57.1069515118366,1.89320029256016,0.546521062953796));
#30176=CARTESIAN_POINT('Ctrl Pts',(-57.1067193922639,1.89325977797126,0.426774852984043));
#30177=CARTESIAN_POINT('Ctrl Pts',(-57.1059218532478,1.89254980474384,0.182314358857985));
#30178=CARTESIAN_POINT('Ctrl Pts',(-57.1037245963224,1.88931843331046,-0.245591088774696));
#30179=CARTESIAN_POINT('Ctrl Pts',(-57.0987044091975,1.88041735632271,-0.864386774086259));
#30180=CARTESIAN_POINT('Ctrl Pts',(-57.0909665484324,1.86725052592357,-1.61725556496489));
#30181=CARTESIAN_POINT('Ctrl Pts',(-57.0799859241427,1.85266601275522,-2.6357887229553));
#30182=CARTESIAN_POINT('Ctrl Pts',(-57.0681882866568,1.85141583259298,-3.93733134415447));
#30183=CARTESIAN_POINT('Ctrl Pts',(-57.0686338134797,1.8975336049876,-5.01284013637244));
#30184=CARTESIAN_POINT('Ctrl Pts',(-57.0741377233594,1.95117898364246,-5.69407277102527));
#30185=CARTESIAN_POINT('Ctrl Pts',(-57.0782624923922,1.968341193729,-5.92460777169142));
#30186=CARTESIAN_POINT('Ctrl Pts',(-57.0907813565385,2.00329563169115,-6.42030539819386));
#30187=CARTESIAN_POINT('Ctrl Pts',(-57.1223386706861,2.06395766073599,-7.29948928425403));
#30188=CARTESIAN_POINT('Ctrl Pts',(-57.1805994014943,2.17680783090116,-8.6327922182843));
#30189=CARTESIAN_POINT('Ctrl Pts',(-57.2188178486793,2.39767782185249,-10.0481485710067));
#30190=CARTESIAN_POINT('Ctrl Pts',(-57.2135095031993,2.65106102057314,-11.075169803635));
#30191=CARTESIAN_POINT('Ctrl Pts',(-57.1984185480159,2.82983507690918,-11.6693836511967));
#30192=CARTESIAN_POINT('Ctrl Pts',(-57.1864698978013,2.93142771294683,-11.968374134992));
#30193=CARTESIAN_POINT('Ctrl Pts',(-57.1755793884883,3.01319812834117,-12.1949580577661));
#30194=CARTESIAN_POINT('Ctrl Pts',(-57.1646573280793,3.08090027626859,-12.3737171427022));
#30195=CARTESIAN_POINT('Ctrl Pts',(-57.1424559875788,3.22031535553374,-12.7050150981405));
#30196=CARTESIAN_POINT('Ctrl Pts',(-57.0984492701348,3.48882118432202,-13.269768853707));
#30197=CARTESIAN_POINT('Ctrl Pts',(-56.971450424072,4.25779705956758,-14.6036767810547));
#30198=CARTESIAN_POINT('Ctrl Pts',(-56.821616693217,5.2117115170756,-15.8850776230598));
#30199=CARTESIAN_POINT('Ctrl Pts',(-56.7124849345261,5.92568874830589,-16.9994620802121));
#30200=CARTESIAN_POINT('Ctrl Pts',(-56.6705149547657,6.19751789378465,-17.4954244417774));
#30201=CARTESIAN_POINT('Ctrl Pts',(-56.6457436004024,6.35273777337066,-17.8450298557747));
#30202=CARTESIAN_POINT('Ctrl Pts',(-56.6361124070848,6.40938624849264,-18.0006668464923));
#30203=CARTESIAN_POINT('Ctrl Pts',(-56.6297990083521,6.44435211093092,-18.1098859771711));
#30204=CARTESIAN_POINT('Ctrl Pts',(-56.6238224116994,6.47364854166899,-18.2061271424651));
#30205=CARTESIAN_POINT('Ctrl Pts',(-56.6127470082692,6.52310520343213,-18.3863532881278));
#30206=CARTESIAN_POINT('Ctrl Pts',(-56.6010901193704,6.5673566044715,-18.5744851958529));
#30207=CARTESIAN_POINT('Ctrl Pts',(-56.5895322765753,6.60454437832707,-18.763467941586));
#30208=CARTESIAN_POINT('Ctrl Pts',(-56.58224180853,6.62550800540167,-18.8837829985038));
#30209=CARTESIAN_POINT('Ctrl Pts',(-56.5764278031212,6.6407926052895,-18.980842173998));
#30210=CARTESIAN_POINT('Ctrl Pts',(-56.5706154103516,6.65517482885583,-19.078680320108));
#30211=CARTESIAN_POINT('Ctrl Pts',(-56.5546691104267,6.69101365753071,-19.3505992028544));
#30212=CARTESIAN_POINT('Ctrl Pts',(-56.5290614864106,6.73029436785628,-19.8128903368675));
#30213=CARTESIAN_POINT('Ctrl Pts',(-56.4869367980868,6.7568518830943,-20.6888973291557));
#30214=CARTESIAN_POINT('Ctrl Pts',(-56.4440732140486,6.73201820804871,-21.8900996704012));
#30215=CARTESIAN_POINT('Ctrl Pts',(-56.4209020797944,6.72003372304772,-22.9645758384404));
#30216=CARTESIAN_POINT('Ctrl Pts',(-56.4084698223593,6.74461303690916,-23.6666494407614));
#30217=CARTESIAN_POINT('Ctrl Pts',(-56.4044520571116,6.75153694503519,-23.8933220995226));
#30218=CARTESIAN_POINT('Ctrl Pts',(-56.398617957031,6.76311230502334,-24.3786928060929));
#30219=CARTESIAN_POINT('Ctrl Pts',(-56.3939455464681,6.77486749362624,-25.2203664442027));
#30220=CARTESIAN_POINT('Ctrl Pts',(-56.3991641106537,6.77404460420982,-26.4506971606171));
#30221=CARTESIAN_POINT('Ctrl Pts',(-56.4128090599345,6.75952574652236,-27.9490394394889));
#30222=CARTESIAN_POINT('Ctrl Pts',(-56.4186020964461,6.75163853710771,-28.964769856858));
#30223=CARTESIAN_POINT('Ctrl Pts',(-56.4185413807569,6.75071680998041,-29.5392213230429));
#30224=CARTESIAN_POINT('Ctrl Pts',(-56.41850077081,6.75047701527422,-29.6630482265954));
#30225=CARTESIAN_POINT('Ctrl Pts',(-56.4183418667709,6.7498682969808,-29.9130092974894));
#30226=CARTESIAN_POINT('Ctrl Pts',(-56.4178679759819,6.74849085107283,-30.3496443283428));
#30227=CARTESIAN_POINT('Ctrl Pts',(-56.4162669443321,6.74460365616335,-31.2249500551174));
#30228=CARTESIAN_POINT('Ctrl Pts',(-56.4135345404153,6.7382792574658,-32.2268944758849));
#30229=CARTESIAN_POINT('Ctrl Pts',(-56.4110627833574,6.73139160220425,-33.2302213512026));
#30230=CARTESIAN_POINT('Ctrl Pts',(-56.4096388148828,6.72630365081552,-33.9829942708887));
#30231=CARTESIAN_POINT('Ctrl Pts',(-56.4089564710274,6.72171147475502,-34.7356406759868));
#30232=CARTESIAN_POINT('Ctrl Pts',(-56.4091943917731,6.71921902154299,-35.2372017854706));
#30233=CARTESIAN_POINT('Ctrl Pts',(-56.4097070974696,6.71764854985147,-35.6142149941863));
#30234=CARTESIAN_POINT('Ctrl Pts',(-56.4101658912545,6.71661412342689,-35.865417217711));
#30235=CARTESIAN_POINT('Ctrl Pts',(-56.4114906099971,6.71457458211718,-36.368036988799));
#30236=CARTESIAN_POINT('Ctrl Pts',(-56.4147583547514,6.71118598106391,-37.2459301139164));
#30237=CARTESIAN_POINT('Ctrl Pts',(-56.4239222246451,6.70512592455748,-38.9992306282585));
#30238=CARTESIAN_POINT('Ctrl Pts',(-56.4325797483113,6.70211084427062,-40.503204307213));
#30239=CARTESIAN_POINT('Ctrl Pts',(-56.4356597418105,6.70158386685987,-41.637518018572));
#30240=CARTESIAN_POINT('Ctrl Pts',(-56.436227148003,6.70129977242393,-41.8854637139816));
#30241=CARTESIAN_POINT('Ctrl Pts',(-56.4367999559624,6.70050414418084,-42.2597454053479));
#30242=CARTESIAN_POINT('Ctrl Pts',(-56.4371408314556,6.69944454592799,-42.6344827075468));
#30243=CARTESIAN_POINT('Ctrl Pts',(-56.4373510800416,6.69782878260777,-43.135565630316));
#30244=CARTESIAN_POINT('Ctrl Pts',(-56.4372757430818,6.69570282927745,-43.7638437316683));
#30245=CARTESIAN_POINT('Ctrl Pts',(-56.4370272452715,6.69386923707254,-44.520581936709));
#30246=CARTESIAN_POINT('Ctrl Pts',(-56.4370066578341,6.69368485012211,-45.153030469146));
#30247=CARTESIAN_POINT('Ctrl Pts',(-56.4372951630701,6.69479554136445,-45.6598675472249));
#30248=CARTESIAN_POINT('Ctrl Pts',(-56.4377102385364,6.69637061949979,-46.0403728670534));
#30249=CARTESIAN_POINT('Ctrl Pts',(-56.4383715762544,6.69880078721367,-46.4211725489629));
#30250=CARTESIAN_POINT('Ctrl Pts',(-56.4396469866395,6.70333891093526,-46.9292908559997));
#30251=CARTESIAN_POINT('Ctrl Pts',(-56.4411106225019,6.70835911318831,-47.3105250847255));
#30252=CARTESIAN_POINT('Ctrl Pts',(-56.4430182769622,6.71472635597951,-47.6932085369429));
#30253=CARTESIAN_POINT('Ctrl Pts',(-56.4443202971396,6.72078385397459,-47.9627015428219));
#30254=CARTESIAN_POINT('Ctrl Pts',(-56.4471805957533,6.73791561249716,-48.488363057411));
#30255=CARTESIAN_POINT('Ctrl Pts',(-56.452839064889,6.7786876824453,-49.3987692580904));
#30256=CARTESIAN_POINT('Ctrl Pts',(-56.4630087305302,6.8516965935292,-50.6573205793611));
#30257=CARTESIAN_POINT('Ctrl Pts',(-56.478554955567,6.91734142697298,-52.1049636847472));
#30258=CARTESIAN_POINT('Ctrl Pts',(-56.4906652637739,6.91946551340035,-53.0254034352169));
#30259=CARTESIAN_POINT('Ctrl Pts',(-56.4984723795404,6.90065827744901,-53.5868753803797));
#30260=CARTESIAN_POINT('Ctrl Pts',(-56.5016002918511,6.89025157491666,-53.7863134357493));
#30261=CARTESIAN_POINT('Ctrl Pts',(-56.5084824846647,6.85476627102659,-54.2176424541867));
#30262=CARTESIAN_POINT('Ctrl Pts',(-56.5222064261297,6.75859620610259,-55.002900407287));
#30263=CARTESIAN_POINT('Ctrl Pts',(-56.5557188725619,6.47235329506978,-56.7244566461801));
#30264=CARTESIAN_POINT('Ctrl Pts',(-56.5905103920183,6.22672792184383,-58.4359110328748));
#30265=CARTESIAN_POINT('Ctrl Pts',(-56.5993085295866,6.3084712124735,-59.7694917049779));
#30266=CARTESIAN_POINT('Ctrl Pts',(-56.6004698795833,6.31828583588924,-59.9110750466561));
#30267=CARTESIAN_POINT('Ctrl Pts',(-56.6024562371235,6.3424334183536,-60.2046373889052));
#30268=CARTESIAN_POINT('Ctrl Pts',(-56.6053617926738,6.39427272691221,-60.7100762799175));
#30269=CARTESIAN_POINT('Ctrl Pts',(-56.6089382009559,6.5355130961319,-61.7144784683024));
#30270=CARTESIAN_POINT('Ctrl Pts',(-56.6091698803726,6.77181605987139,-62.8337296048277));
#30271=CARTESIAN_POINT('Ctrl Pts',(-56.6076626515125,7.06395772219953,-63.9256374359719));
#30272=CARTESIAN_POINT('Ctrl Pts',(-56.6065228937132,7.24589964597599,-64.5285821372516));
#30273=CARTESIAN_POINT('Ctrl Pts',(-56.6057887546143,7.37315981700677,-64.9258717139614));
#30274=CARTESIAN_POINT('Ctrl Pts',(-56.6053161341454,7.45950133603607,-65.1894268522663));
#30275=CARTESIAN_POINT('Ctrl Pts',(-56.6048767227722,7.54799334393313,-65.451152914096));
#30276=CARTESIAN_POINT('Ctrl Pts',(-56.6045524245517,7.62703929608164,-65.678391165162));
#30277=CARTESIAN_POINT('Ctrl Pts',(-56.6043872291298,7.6726394260606,-65.8077411904003));
#30278=CARTESIAN_POINT('Ctrl Pts',(-56.6041598697884,7.74146499495084,-66.0012899423398));
#30279=CARTESIAN_POINT('Ctrl Pts',(-56.6040204700608,7.79963823627409,-66.1615022228199));
#30280=CARTESIAN_POINT('Ctrl Pts',(-56.6038401398609,7.89712205512293,-66.4260012968152));
#30281=CARTESIAN_POINT('Ctrl Pts',(-56.6018613301423,8.014442436703,-66.7303952892477));
#30282=CARTESIAN_POINT('Ctrl Pts',(-56.598807991678,8.256476084168,-67.307186300956));
#30283=CARTESIAN_POINT('Ctrl Pts',(-56.5930422710428,8.71563585450053,-68.2955341954575));
#30284=CARTESIAN_POINT('Ctrl Pts',(-56.5841020241658,9.71659757217878,-70.1535468005837));
#30285=CARTESIAN_POINT('Ctrl Pts',(-56.5841667701637,10.5920789188348,-71.6137998228524));
#30286=CARTESIAN_POINT('Ctrl Pts',(-56.589609187159,11.1461190431333,-72.6661384045627));
#30287=CARTESIAN_POINT('Ctrl Pts',(-56.589132916731,11.2817778728624,-72.9238283541102));
#30288=CARTESIAN_POINT('Ctrl Pts',(-56.5891691531417,11.5466066026176,-73.4254076537761));
#30289=CARTESIAN_POINT('Ctrl Pts',(-56.5888472189315,11.8811705517907,-74.0571578520545));
#30290=CARTESIAN_POINT('Ctrl Pts',(-56.5887317976132,12.2818546867643,-74.811057703383));
#30291=CARTESIAN_POINT('Ctrl Pts',(-56.5884758996885,13.0849847332041,-76.3186339768239));
#30292=CARTESIAN_POINT('Ctrl Pts',(-56.5885073839689,13.7543894226819,-77.5711826827783));
#30293=CARTESIAN_POINT('Ctrl Pts',(-56.5887725216993,14.7223187302815,-79.3917286320565));
#30294=CARTESIAN_POINT('Ctrl Pts',(-56.5886560510561,15.1596634720437,-80.2143905730094));
#30295=CARTESIAN_POINT('Ctrl Pts',(-56.5886560510566,15.5961850594335,-81.035368275107));
#30296=CARTESIAN_POINT('Ctrl Pts',(-53.7934016121151,1.46777263035546,24.8308339314903));
#30297=CARTESIAN_POINT('Ctrl Pts',(-53.7935673789398,1.46778911572206,24.7819610087646));
#30298=CARTESIAN_POINT('Ctrl Pts',(-53.7937412291651,1.46780639203802,24.7330891581798));
#30299=CARTESIAN_POINT('Ctrl Pts',(-53.7957940605583,1.4680113567613,24.182559255354));
#30300=CARTESIAN_POINT('Ctrl Pts',(-53.7974505746972,1.46806870936156,23.1785615709389));
#30301=CARTESIAN_POINT('Ctrl Pts',(-53.8013623765295,1.46812178194841,21.170090874394));
#30302=CARTESIAN_POINT('Ctrl Pts',(-53.8150194711945,1.46949731762704,19.6659938923605));
#30303=CARTESIAN_POINT('Ctrl Pts',(-53.8435681586524,1.47291723683062,18.4149444354279));
#30304=CARTESIAN_POINT('Ctrl Pts',(-53.8573208660153,1.47453448565679,17.9124519807325));
#30305=CARTESIAN_POINT('Ctrl Pts',(-53.8919646968564,1.47856781673371,16.9087225712457));
#30306=CARTESIAN_POINT('Ctrl Pts',(-53.9662720517638,1.48726824488107,15.154985516567));
#30307=CARTESIAN_POINT('Ctrl Pts',(-54.0360759968836,1.49596967969934,13.6523955194275));
#30308=CARTESIAN_POINT('Ctrl Pts',(-54.0783783253391,1.50214118899151,12.3965940749575));
#30309=CARTESIAN_POINT('Ctrl Pts',(-54.0955196430407,1.50475066335151,11.8950813235525));
#30310=CARTESIAN_POINT('Ctrl Pts',(-54.1299654040665,1.51034842817017,10.8924208756531));
#30311=CARTESIAN_POINT('Ctrl Pts',(-54.1885203186833,1.52060781579293,9.13802848610798));
#30312=CARTESIAN_POINT('Ctrl Pts',(-54.2283839579081,1.52835861779018,7.63360627521497));
#30313=CARTESIAN_POINT('Ctrl Pts',(-54.2457520045372,1.53183396510449,6.50373537823322));
#30314=CARTESIAN_POINT('Ctrl Pts',(-54.2492240717393,1.53257118037915,6.25319826017849));
#30315=CARTESIAN_POINT('Ctrl Pts',(-54.2548282374031,1.53394380346214,5.75188483012969));
#30316=CARTESIAN_POINT('Ctrl Pts',(-54.2614203310286,1.53607147592114,4.87331849088099));
#30317=CARTESIAN_POINT('Ctrl Pts',(-54.2642706333787,1.53913741979663,3.11388667514309));
#30318=CARTESIAN_POINT('Ctrl Pts',(-54.2573573900383,1.53962861673724,1.61024224287674));
#30319=CARTESIAN_POINT('Ctrl Pts',(-54.2557011205212,1.53829310187352,0.55436693754337));
#30320=CARTESIAN_POINT('Ctrl Pts',(-54.2554390849759,1.53794051723846,0.433325589773345));
#30321=CARTESIAN_POINT('Ctrl Pts',(-54.2546681386206,1.53649044292413,0.18795312726425));
#30322=CARTESIAN_POINT('Ctrl Pts',(-54.252728235578,1.53219001729857,-0.241485578503602));
#30323=CARTESIAN_POINT('Ctrl Pts',(-54.2485647358662,1.52204724154832,-0.859857757289458));
#30324=CARTESIAN_POINT('Ctrl Pts',(-54.2423653025322,1.50685522503959,-1.60940139514622));
#30325=CARTESIAN_POINT('Ctrl Pts',(-54.2337702553029,1.48741416699455,-2.61949206742553));
#30326=CARTESIAN_POINT('Ctrl Pts',(-54.2248290290242,1.47379740438393,-3.90374360005717));
#30327=CARTESIAN_POINT('Ctrl Pts',(-54.2237546998493,1.49469271641052,-4.95634090943278));
#30328=CARTESIAN_POINT('Ctrl Pts',(-54.2262898829685,1.52395867016253,-5.62053571048191));
#30329=CARTESIAN_POINT('Ctrl Pts',(-54.2285279466657,1.53131804401625,-5.83575830669255));
#30330=CARTESIAN_POINT('Ctrl Pts',(-54.2359652395121,1.54110790073169,-6.30995058400631));
#30331=CARTESIAN_POINT('Ctrl Pts',(-54.2558568768288,1.54636009588386,-7.15921369100389));
#30332=CARTESIAN_POINT('Ctrl Pts',(-54.2950429819351,1.55409167594932,-8.48036951587064));
#30333=CARTESIAN_POINT('Ctrl Pts',(-54.3205719897746,1.66848273124656,-9.9244522864012));
#30334=CARTESIAN_POINT('Ctrl Pts',(-54.312568655207,1.87351618397868,-10.9933412080439));
#30335=CARTESIAN_POINT('Ctrl Pts',(-54.2978584316208,2.03643173645517,-11.6154728873208));
#30336=CARTESIAN_POINT('Ctrl Pts',(-54.2867628586866,2.13458357810496,-11.9293880794604));
#30337=CARTESIAN_POINT('Ctrl Pts',(-54.2768008071091,2.2156141577047,-12.1672645885673));
#30338=CARTESIAN_POINT('Ctrl Pts',(-54.267494328204,2.28204721859384,-12.3507732600618));
#30339=CARTESIAN_POINT('Ctrl Pts',(-54.2483789945923,2.42117363210546,-12.6918139021029));
#30340=CARTESIAN_POINT('Ctrl Pts',(-54.2107920579036,2.69225073302814,-13.2700414996205));
#30341=CARTESIAN_POINT('Ctrl Pts',(-54.1030771678834,3.48048502493028,-14.6262372115562));
#30342=CARTESIAN_POINT('Ctrl Pts',(-53.9771754176793,4.47676316804508,-15.9132716989074));
#30343=CARTESIAN_POINT('Ctrl Pts',(-53.8897724903015,5.23569685768015,-17.0368058515114));
#30344=CARTESIAN_POINT('Ctrl Pts',(-53.8579894956111,5.52844808758236,-17.5377958305941));
#30345=CARTESIAN_POINT('Ctrl Pts',(-53.8404307262847,5.6977814388372,-17.8914023062076));
#30346=CARTESIAN_POINT('Ctrl Pts',(-53.8339744984258,5.76028275608763,-18.0485841585714));
#30347=CARTESIAN_POINT('Ctrl Pts',(-53.8297703239331,5.79916255628037,-18.1587919495587));
#30348=CARTESIAN_POINT('Ctrl Pts',(-53.8245910442156,5.83333739156381,-18.2602275211408));
#30349=CARTESIAN_POINT('Ctrl Pts',(-53.8152920655446,5.8914731828385,-18.4478752857952));
#30350=CARTESIAN_POINT('Ctrl Pts',(-53.805059196899,5.94520279417078,-18.6438764863963));
#30351=CARTESIAN_POINT('Ctrl Pts',(-53.794731083789,5.99190214459915,-18.8394772679612));
#30352=CARTESIAN_POINT('Ctrl Pts',(-53.7880865359489,6.01898670176359,-18.963714071526));
#30353=CARTESIAN_POINT('Ctrl Pts',(-53.7827277050717,6.0392157203007,-19.0636531415675));
#30354=CARTESIAN_POINT('Ctrl Pts',(-53.7773234858651,6.05859471368721,-19.1642367417344));
#30355=CARTESIAN_POINT('Ctrl Pts',(-53.7623277089261,6.10835396803088,-19.4430827885807));
#30356=CARTESIAN_POINT('Ctrl Pts',(-53.7372415696916,6.17142503101148,-19.9131603160178));
#30357=CARTESIAN_POINT('Ctrl Pts',(-53.6935132011328,6.24222084540794,-20.7924887338115));
#30358=CARTESIAN_POINT('Ctrl Pts',(-53.6442466092503,6.27298426820498,-21.9784669573157));
#30359=CARTESIAN_POINT('Ctrl Pts',(-53.6155684496993,6.29549036050109,-23.021350889866));
#30360=CARTESIAN_POINT('Ctrl Pts',(-53.6024693749055,6.33239130361649,-23.6991293794627));
#30361=CARTESIAN_POINT('Ctrl Pts',(-53.5985819342631,6.34261691041929,-23.9180512590553));
#30362=CARTESIAN_POINT('Ctrl Pts',(-53.5935358905347,6.35913189985168,-24.3889889387686));
#30363=CARTESIAN_POINT('Ctrl Pts',(-53.5918708358186,6.37391540030867,-25.2107698626316));
#30364=CARTESIAN_POINT('Ctrl Pts',(-53.6040498497994,6.36514225940184,-26.4264201050671));
#30365=CARTESIAN_POINT('Ctrl Pts',(-53.6242207361812,6.33345765269652,-27.9280588553213));
#30366=CARTESIAN_POINT('Ctrl Pts',(-53.6295728505492,6.31943683297756,-28.959629391164));
#30367=CARTESIAN_POINT('Ctrl Pts',(-53.6271869297582,6.31970805391784,-29.5468163864961));
#30368=CARTESIAN_POINT('Ctrl Pts',(-53.6265864783266,6.31978287904433,-29.671384628671));
#30369=CARTESIAN_POINT('Ctrl Pts',(-53.6250667987525,6.31996279399016,-29.923847888049));
#30370=CARTESIAN_POINT('Ctrl Pts',(-53.6216319863939,6.32038187020811,-30.3639241508376));
#30371=CARTESIAN_POINT('Ctrl Pts',(-53.6120885474211,6.32156814777126,-31.2451424338698));
#30372=CARTESIAN_POINT('Ctrl Pts',(-53.5969373333556,6.32371858918401,-32.2504383272288));
#30373=CARTESIAN_POINT('Ctrl Pts',(-53.5813612542214,6.32630002720943,-33.2541958950975));
#30374=CARTESIAN_POINT('Ctrl Pts',(-53.5704027525453,6.32832989098395,-34.0057459397616));
#30375=CARTESIAN_POINT('Ctrl Pts',(-53.5610483743253,6.33039553598111,-34.7556974144078));
#30376=CARTESIAN_POINT('Ctrl Pts',(-53.5565139258382,6.33167213419517,-35.2544308736739));
#30377=CARTESIAN_POINT('Ctrl Pts',(-53.5539829777077,6.33254473266672,-35.6289821016848));
#30378=CARTESIAN_POINT('Ctrl Pts',(-53.5524502113088,6.33310500932045,-35.8802919564392));
#30379=CARTESIAN_POINT('Ctrl Pts',(-53.5499879553691,6.3341905553782,-36.3821337994043));
#30380=CARTESIAN_POINT('Ctrl Pts',(-53.5470469584226,6.33605749177594,-37.2591689062186));
#30381=CARTESIAN_POINT('Ctrl Pts',(-53.545611343113,6.33963029040366,-39.0103239055287));
#30382=CARTESIAN_POINT('Ctrl Pts',(-53.5475157379776,6.34317576888129,-40.5124690600292));
#30383=CARTESIAN_POINT('Ctrl Pts',(-53.5463870493891,6.34658591977076,-41.6452248570771));
#30384=CARTESIAN_POINT('Ctrl Pts',(-53.5460466970974,6.34714783542476,-41.8929952917692));
#30385=CARTESIAN_POINT('Ctrl Pts',(-53.5452852331639,6.3475797869505,-42.2668944327146));
#30386=CARTESIAN_POINT('Ctrl Pts',(-53.5443403736996,6.34769293423752,-42.6412473608991));
#30387=CARTESIAN_POINT('Ctrl Pts',(-53.5429130930101,6.34756107786103,-43.1417584080132));
#30388=CARTESIAN_POINT('Ctrl Pts',(-53.5409700056762,6.34712133883608,-43.7692492442951));
#30389=CARTESIAN_POINT('Ctrl Pts',(-53.5388692960199,6.34698370328379,-44.5249144541569));
#30390=CARTESIAN_POINT('Ctrl Pts',(-53.5377154954766,6.347890329422,-45.1563683365974));
#30391=CARTESIAN_POINT('Ctrl Pts',(-53.5373957112746,6.34965487606607,-45.6623434458641));
#30392=CARTESIAN_POINT('Ctrl Pts',(-53.5375169831425,6.35160171309878,-46.0421706147613));
#30393=CARTESIAN_POINT('Ctrl Pts',(-53.538060660001,6.35427798974301,-46.4222597520264));
#30394=CARTESIAN_POINT('Ctrl Pts',(-53.5394265341858,6.35896795642496,-46.9293851512309));
#30395=CARTESIAN_POINT('Ctrl Pts',(-53.541272296068,6.36388958678053,-47.3098256250045));
#30396=CARTESIAN_POINT('Ctrl Pts',(-53.5437818261607,6.37000480373162,-47.6916677590655));
#30397=CARTESIAN_POINT('Ctrl Pts',(-53.5455924689859,6.37580304256165,-47.960337851122));
#30398=CARTESIAN_POINT('Ctrl Pts',(-53.5498248090328,6.39214339623986,-48.4846410143508));
#30399=CARTESIAN_POINT('Ctrl Pts',(-53.5587313083972,6.43088530243379,-49.3929125059758));
#30400=CARTESIAN_POINT('Ctrl Pts',(-53.5755060111104,6.49968058835098,-50.6493696743647));
#30401=CARTESIAN_POINT('Ctrl Pts',(-53.6004972349383,6.55960541879972,-52.0959799952106));
#30402=CARTESIAN_POINT('Ctrl Pts',(-53.6190623160665,6.558232531547,-53.0168836910162));
#30403=CARTESIAN_POINT('Ctrl Pts',(-53.6306238175058,6.53750837149187,-53.5789969700663));
#30404=CARTESIAN_POINT('Ctrl Pts',(-53.6353606964767,6.52646442318359,-53.7776352503713));
#30405=CARTESIAN_POINT('Ctrl Pts',(-53.645734295578,6.48945316580513,-54.2082374321146));
#30406=CARTESIAN_POINT('Ctrl Pts',(-53.6661324091788,6.39020190256059,-54.9924898053466));
#30407=CARTESIAN_POINT('Ctrl Pts',(-53.713710148044,6.09625529604762,-56.7140879374555));
#30408=CARTESIAN_POINT('Ctrl Pts',(-53.7589051895162,5.84293062820704,-58.4280636037592));
#30409=CARTESIAN_POINT('Ctrl Pts',(-53.7715828337572,5.92250213479751,-59.7656855936463));
#30410=CARTESIAN_POINT('Ctrl Pts',(-53.7731656932649,5.93211149096596,-59.9076936967855));
#30411=CARTESIAN_POINT('Ctrl Pts',(-53.77590163928,5.9559156563119,-60.202093386478));
#30412=CARTESIAN_POINT('Ctrl Pts',(-53.7798532617372,6.00737679110324,-60.708865386902));
#30413=CARTESIAN_POINT('Ctrl Pts',(-53.7845893375299,6.14858231987656,-61.7154729716548));
#30414=CARTESIAN_POINT('Ctrl Pts',(-53.7845303613166,6.38597608025257,-62.8361691722631));
#30415=CARTESIAN_POINT('Ctrl Pts',(-53.7821312316756,6.6794062497289,-63.9285641115212));
#30416=CARTESIAN_POINT('Ctrl Pts',(-53.7804431471772,6.86199977133404,-64.5314447099742));
#30417=CARTESIAN_POINT('Ctrl Pts',(-53.7794000606766,6.98960175420206,-64.9285561501802));
#30418=CARTESIAN_POINT('Ctrl Pts',(-53.778740463873,7.07614276013107,-65.1919565016734));
#30419=CARTESIAN_POINT('Ctrl Pts',(-53.7781525663691,7.16478614425998,-65.453475127933));
#30420=CARTESIAN_POINT('Ctrl Pts',(-53.7777420750812,7.2439118387775,-65.6804847015284));
#30421=CARTESIAN_POINT('Ctrl Pts',(-53.77754221375,7.28954106411927,-65.8096905892259));
#30422=CARTESIAN_POINT('Ctrl Pts',(-53.7772782956537,7.35839330495848,-66.0030101040648));
#30423=CARTESIAN_POINT('Ctrl Pts',(-53.7771430125486,7.41655114813598,-66.1630025048135));
#30424=CARTESIAN_POINT('Ctrl Pts',(-53.7770256834519,7.51395693356719,-66.4271098313235));
#30425=CARTESIAN_POINT('Ctrl Pts',(-53.7752148209481,7.63142091921661,-66.7316129850791));
#30426=CARTESIAN_POINT('Ctrl Pts',(-53.7724247277615,7.87358777963525,-67.3083279285345));
#30427=CARTESIAN_POINT('Ctrl Pts',(-53.7670988596911,8.33298698555509,-68.2966879559896));
#30428=CARTESIAN_POINT('Ctrl Pts',(-53.7586990304113,9.33415198459075,-70.1546042763352));
#30429=CARTESIAN_POINT('Ctrl Pts',(-53.7585430513173,10.2095760158847,-71.6149034133299));
#30430=CARTESIAN_POINT('Ctrl Pts',(-53.7635426717601,10.7635372970318,-72.6672677412076));
#30431=CARTESIAN_POINT('Ctrl Pts',(-53.7630975428578,10.8992077037409,-72.9249499844023));
#30432=CARTESIAN_POINT('Ctrl Pts',(-53.7631233115819,11.164039597928,-73.4265220770171));
#30433=CARTESIAN_POINT('Ctrl Pts',(-53.7628216263235,11.4986106864948,-74.0582634495331));
#30434=CARTESIAN_POINT('Ctrl Pts',(-53.7627152736492,11.8992935984681,-74.8121555077136));
#30435=CARTESIAN_POINT('Ctrl Pts',(-53.7624875317562,12.7024162513666,-76.3197207705758));
#30436=CARTESIAN_POINT('Ctrl Pts',(-53.7625345079358,13.3718089832052,-77.5722790747414));
#30437=CARTESIAN_POINT('Ctrl Pts',(-53.7627793283121,14.3397433529917,-79.3928470096629));
#30438=CARTESIAN_POINT('Ctrl Pts',(-53.7626727299908,14.7770883200868,-80.2155053720511));
#30439=CARTESIAN_POINT('Ctrl Pts',(-53.7626727299913,15.2136099074762,-81.0364830741499));
#30440=CARTESIAN_POINT('Ctrl Pts',(-50.9533304548877,1.12167625420265,24.8307786104982));
#30441=CARTESIAN_POINT('Ctrl Pts',(-50.9534791778414,1.12168955436835,24.7819039865689));
#30442=CARTESIAN_POINT('Ctrl Pts',(-50.9536351645509,1.12170348685097,24.7330304228356));
#30443=CARTESIAN_POINT('Ctrl Pts',(-50.9554771492024,1.12186904382061,24.1824800475833));
#30444=CARTESIAN_POINT('Ctrl Pts',(-50.9567903115075,1.12191614443668,23.1784269860304));
#30445=CARTESIAN_POINT('Ctrl Pts',(-50.9597831991283,1.12195817483025,21.1699338582703));
#30446=CARTESIAN_POINT('Ctrl Pts',(-50.9720463860967,1.12307056520977,19.6658727615868));
#30447=CARTESIAN_POINT('Ctrl Pts',(-50.9985453915116,1.1258322201535,18.4148737681668));
#30448=CARTESIAN_POINT('Ctrl Pts',(-51.0112286601023,1.12711396072438,17.9124017236622));
#30449=CARTESIAN_POINT('Ctrl Pts',(-51.0430398380213,1.13025729638921,16.9086671448333));
#30450=CARTESIAN_POINT('Ctrl Pts',(-51.1113070441228,1.13701225441876,15.1548226495192));
#30451=CARTESIAN_POINT('Ctrl Pts',(-51.1766279251767,1.14401741530908,13.6521351888613));
#30452=CARTESIAN_POINT('Ctrl Pts',(-51.2183692549294,1.14950702495355,12.3963110911906));
#30453=CARTESIAN_POINT('Ctrl Pts',(-51.235533688408,1.15187486393477,11.8947961481062));
#30454=CARTESIAN_POINT('Ctrl Pts',(-51.2708463731445,1.15709885931404,10.8921784782769));
#30455=CARTESIAN_POINT('Ctrl Pts',(-51.3326019245734,1.16696112254147,9.13794308818202));
#30456=CARTESIAN_POINT('Ctrl Pts',(-51.3765146408331,1.17472693684257,7.63358702269936));
#30457=CARTESIAN_POINT('Ctrl Pts',(-51.3959170056814,1.17829663045827,6.50362753793607));
#30458=CARTESIAN_POINT('Ctrl Pts',(-51.3999214168377,1.1790868432743,6.2529883040083));
#30459=CARTESIAN_POINT('Ctrl Pts',(-51.4068538864216,1.18062988460862,5.75153998446659));
#30460=CARTESIAN_POINT('Ctrl Pts',(-51.416308115296,1.18319700036463,4.87278314651673));
#30461=CARTESIAN_POINT('Ctrl Pts',(-51.4257086539026,1.18740562053211,3.11320814186707));
#30462=CARTESIAN_POINT('Ctrl Pts',(-51.4216042553005,1.18821623676665,1.61015579346892));
#30463=CARTESIAN_POINT('Ctrl Pts',(-51.4170601115308,1.18643334864416,0.554416805138194));
#30464=CARTESIAN_POINT('Ctrl Pts',(-51.4164071173122,1.18609291103861,0.431151137820113));
#30465=CARTESIAN_POINT('Ctrl Pts',(-51.4146833613188,1.18495731393319,0.182958129310269));
#30466=CARTESIAN_POINT('Ctrl Pts',(-51.410648398026,1.18187759185579,-0.251235209137858));
#30467=CARTESIAN_POINT('Ctrl Pts',(-51.4024023622892,1.17501101039931,-0.873530111729729));
#30468=CARTESIAN_POINT('Ctrl Pts',(-51.3899724528526,1.16476324658724,-1.62384337035073));
#30469=CARTESIAN_POINT('Ctrl Pts',(-51.3718328018968,1.15121190737502,-2.62909007476115));
#30470=CARTESIAN_POINT('Ctrl Pts',(-51.349775001512,1.13928759628803,-3.89638380984962));
#30471=CARTESIAN_POINT('Ctrl Pts',(-51.3405500283101,1.14653419606001,-4.92478128590191));
#30472=CARTESIAN_POINT('Ctrl Pts',(-51.3398462014328,1.15996094032754,-5.57072457193098));
#30473=CARTESIAN_POINT('Ctrl Pts',(-51.3403303336319,1.16146297983544,-5.77679497093547));
#30474=CARTESIAN_POINT('Ctrl Pts',(-51.3434925138929,1.15595023306681,-6.23609588440421));
#30475=CARTESIAN_POINT('Ctrl Pts',(-51.3541939270753,1.12720006963755,-7.0640227164336));
#30476=CARTESIAN_POINT('Ctrl Pts',(-51.3792213771192,1.06540256207554,-8.36907331474427));
#30477=CARTESIAN_POINT('Ctrl Pts',(-51.4015495864027,1.09674921786008,-9.81997961600263));
#30478=CARTESIAN_POINT('Ctrl Pts',(-51.4021396549063,1.25349998557423,-10.9088976947923));
#30479=CARTESIAN_POINT('Ctrl Pts',(-51.3955703314408,1.39477127206225,-11.5458179296493));
#30480=CARTESIAN_POINT('Ctrl Pts',(-51.389614833581,1.48450113854852,-11.8680356774828));
#30481=CARTESIAN_POINT('Ctrl Pts',(-51.3839415996276,1.56015129354294,-12.1121836484828));
#30482=CARTESIAN_POINT('Ctrl Pts',(-51.3787490189213,1.62065297830379,-12.2947777112652));
#30483=CARTESIAN_POINT('Ctrl Pts',(-51.3682634374915,1.74971620528955,-12.6374645040058));
#30484=CARTESIAN_POINT('Ctrl Pts',(-51.3479996635874,2.00356929358392,-13.2179149355049));
#30485=CARTESIAN_POINT('Ctrl Pts',(-51.2905740263312,2.7533922327797,-14.5828839916141));
#30486=CARTESIAN_POINT('Ctrl Pts',(-51.2256668031853,3.71761730434577,-15.8767255584963));
#30487=CARTESIAN_POINT('Ctrl Pts',(-51.1885763414454,4.47878004447763,-17.0163067639913));
#30488=CARTESIAN_POINT('Ctrl Pts',(-51.1770706210893,4.78354992039058,-17.5313964292859));
#30489=CARTESIAN_POINT('Ctrl Pts',(-51.1704850843513,4.96831779110436,-17.9033237884868));
#30490=CARTESIAN_POINT('Ctrl Pts',(-51.167229188462,5.03974550267696,-18.0726583338754));
#30491=CARTESIAN_POINT('Ctrl Pts',(-51.1643018164506,5.08537209352276,-18.1932669922235));
#30492=CARTESIAN_POINT('Ctrl Pts',(-51.1584545999822,5.12564206537231,-18.3047691678594));
#30493=CARTESIAN_POINT('Ctrl Pts',(-51.1471706920195,5.19551761151212,-18.5102585684698));
#30494=CARTESIAN_POINT('Ctrl Pts',(-51.1328002084724,5.26180800197633,-18.7239464425069));
#30495=CARTESIAN_POINT('Ctrl Pts',(-51.116724658712,5.32133053337001,-18.9355650130454));
#30496=CARTESIAN_POINT('Ctrl Pts',(-51.1057684698181,5.35663234480703,-19.0692789356967));
#30497=CARTESIAN_POINT('Ctrl Pts',(-51.0965781524275,5.38352508729994,-19.1763579639075));
#30498=CARTESIAN_POINT('Ctrl Pts',(-51.0870845657283,5.40964501617818,-19.2838035657413));
#30499=CARTESIAN_POINT('Ctrl Pts',(-51.0598271166654,5.4781846475641,-19.5803077367885));
#30500=CARTESIAN_POINT('Ctrl Pts',(-51.0094406856772,5.57381225777003,-20.0721143614749));
#30501=CARTESIAN_POINT('Ctrl Pts',(-50.910575715869,5.70783467344413,-20.9675428096839));
#30502=CARTESIAN_POINT('Ctrl Pts',(-50.7852287604282,5.82925232102871,-22.1337035918646));
#30503=CARTESIAN_POINT('Ctrl Pts',(-50.7156254993263,5.90750715406542,-23.1221787513864));
#30504=CARTESIAN_POINT('Ctrl Pts',(-50.6898345441324,5.9590716867468,-23.7523466442054));
#30505=CARTESIAN_POINT('Ctrl Pts',(-50.6811721509295,5.97338213884854,-23.9610904354294));
#30506=CARTESIAN_POINT('Ctrl Pts',(-50.6681064463434,5.9951799650087,-24.4095101062452));
#30507=CARTESIAN_POINT('Ctrl Pts',(-50.6558084367241,6.0109657081762,-25.2005643713538));
#30508=CARTESIAN_POINT('Ctrl Pts',(-50.6615509496638,5.98622743157021,-26.3899997669615));
#30509=CARTESIAN_POINT('Ctrl Pts',(-50.6846748525644,5.92620540135337,-27.8927626232332));
#30510=CARTESIAN_POINT('Ctrl Pts',(-50.6950725450099,5.90238162716418,-28.9466459296479));
#30511=CARTESIAN_POINT('Ctrl Pts',(-50.6946680449133,5.90477860278918,-29.5520802304263));
#30512=CARTESIAN_POINT('Ctrl Pts',(-50.6945508254151,5.90534173633429,-29.677033778452));
#30513=CARTESIAN_POINT('Ctrl Pts',(-50.6942580445904,5.9068311947904,-29.9321945236902));
#30514=CARTESIAN_POINT('Ctrl Pts',(-50.6935878682622,5.91026897368014,-30.3756626437439));
#30515=CARTESIAN_POINT('Ctrl Pts',(-50.6917551184676,5.92002859891122,-31.2632127989292));
#30516=CARTESIAN_POINT('Ctrl Pts',(-50.6890613925536,5.9359812317638,-32.2723858506756));
#30517=CARTESIAN_POINT('Ctrl Pts',(-50.6868947412653,5.95289748594645,-33.2770980839551));
#30518=CARTESIAN_POINT('Ctrl Pts',(-50.6858351741547,5.96521819887813,-34.0276841341326));
#30519=CARTESIAN_POINT('Ctrl Pts',(-50.6856401967328,5.97653066469745,-34.7751159223277));
#30520=CARTESIAN_POINT('Ctrl Pts',(-50.6862931357692,5.98283697053856,-35.271052122708));
#30521=CARTESIAN_POINT('Ctrl Pts',(-50.6871553890568,5.98690341449776,-35.6431453859886));
#30522=CARTESIAN_POINT('Ctrl Pts',(-50.6878761975856,5.98962265002083,-35.8946313720791));
#30523=CARTESIAN_POINT('Ctrl Pts',(-50.6898341097545,5.99483435716034,-36.395767705979));
#30524=CARTESIAN_POINT('Ctrl Pts',(-50.6944333194783,6.0036712000655,-37.2720147791089));
#30525=CARTESIAN_POINT('Ctrl Pts',(-50.7069709291633,6.01954031883897,-39.021050925013));
#30526=CARTESIAN_POINT('Ctrl Pts',(-50.7186526447881,6.03145574314737,-40.5212470340552));
#30527=CARTESIAN_POINT('Ctrl Pts',(-50.7231490087732,6.03971614409264,-41.6525612828924));
#30528=CARTESIAN_POINT('Ctrl Pts',(-50.7240138582823,6.04129354764351,-41.9002145372208));
#30529=CARTESIAN_POINT('Ctrl Pts',(-50.7249671509576,6.0432033393967,-42.2737976799135));
#30530=CARTESIAN_POINT('Ctrl Pts',(-50.7256383706633,6.04471914890834,-42.6478327578797));
#30531=CARTESIAN_POINT('Ctrl Pts',(-50.7262316131469,6.04636175646918,-43.1478435611945));
#30532=CARTESIAN_POINT('Ctrl Pts',(-50.7265560428689,6.04793140295822,-43.7746144533213));
#30533=CARTESIAN_POINT('Ctrl Pts',(-50.7267393027773,6.04981561867667,-44.5292312702339));
#30534=CARTESIAN_POINT('Ctrl Pts',(-50.7271050272879,6.0520335529836,-45.1596536767437));
#30535=CARTESIAN_POINT('Ctrl Pts',(-50.7277694704289,6.0545735137265,-45.6647365793174));
#30536=CARTESIAN_POINT('Ctrl Pts',(-50.7285051649595,6.05696506949741,-46.0438451965456));
#30537=CARTESIAN_POINT('Ctrl Pts',(-50.729536775059,6.05993891296549,-46.423168368104));
#30538=CARTESIAN_POINT('Ctrl Pts',(-50.7313883450178,6.06481877022237,-46.9292203912809));
#30539=CARTESIAN_POINT('Ctrl Pts',(-50.7333832907411,6.06963486277635,-47.3087618147421));
#30540=CARTESIAN_POINT('Ctrl Pts',(-50.7359198024195,6.07546295954423,-47.6896758652666));
#30541=CARTESIAN_POINT('Ctrl Pts',(-50.7376702893699,6.0809675711625,-47.9575267341525));
#30542=CARTESIAN_POINT('Ctrl Pts',(-50.7414914696128,6.09641726631753,-48.4804660928323));
#30543=CARTESIAN_POINT('Ctrl Pts',(-50.7489798664707,6.13288565255227,-49.3866459278097));
#30544=CARTESIAN_POINT('Ctrl Pts',(-50.7620693439921,6.19682865621681,-50.6411457416213));
#30545=CARTESIAN_POINT('Ctrl Pts',(-50.7813231122897,6.2499173146937,-52.086868455667));
#30546=CARTESIAN_POINT('Ctrl Pts',(-50.7960716411339,6.2439975724267,-53.0080978203009));
#30547=CARTESIAN_POINT('Ctrl Pts',(-50.8056264058366,6.22071433825672,-53.5706742298222));
#30548=CARTESIAN_POINT('Ctrl Pts',(-50.8094970551415,6.20873941564547,-53.7684937809378));
#30549=CARTESIAN_POINT('Ctrl Pts',(-50.8180425618644,6.16954749151094,-54.1982792283086));
#30550=CARTESIAN_POINT('Ctrl Pts',(-50.834994953766,6.06584658881332,-54.9813661150004));
#30551=CARTESIAN_POINT('Ctrl Pts',(-50.875570231979,5.76112726056181,-56.7026423623578));
#30552=CARTESIAN_POINT('Ctrl Pts',(-50.9151647960118,5.49674034592434,-58.4194361227807));
#30553=CARTESIAN_POINT('Ctrl Pts',(-50.9266859152298,5.57321472253499,-59.761822807359));
#30554=CARTESIAN_POINT('Ctrl Pts',(-50.928128630218,5.58252875863702,-59.9042858995927));
#30555=CARTESIAN_POINT('Ctrl Pts',(-50.9306713131631,5.60583319985075,-60.1996107149606));
#30556=CARTESIAN_POINT('Ctrl Pts',(-50.9344645029265,5.65671550344642,-60.7078459548891));
#30557=CARTESIAN_POINT('Ctrl Pts',(-50.9395525918382,5.79774460568798,-61.7168799795076));
#30558=CARTESIAN_POINT('Ctrl Pts',(-50.940989407537,6.0365126531914,-62.8391349080536));
#30559=CARTESIAN_POINT('Ctrl Pts',(-50.9404102811909,6.33164707325243,-63.9320080217962));
#30560=CARTESIAN_POINT('Ctrl Pts',(-50.9397345638824,6.51512947738313,-64.5347827398139));
#30561=CARTESIAN_POINT('Ctrl Pts',(-50.9393066330775,6.64320899975592,-64.9316825441917));
#30562=CARTESIAN_POINT('Ctrl Pts',(-50.9390387251047,6.73003396949343,-65.1949035881217));
#30563=CARTESIAN_POINT('Ctrl Pts',(-50.9388068656743,6.81889977404073,-65.4561906573326));
#30564=CARTESIAN_POINT('Ctrl Pts',(-50.9386705414863,6.89815450708725,-65.6829499251508));
#30565=CARTESIAN_POINT('Ctrl Pts',(-50.9386150345703,6.94383661586305,-65.811999693998));
#30566=CARTESIAN_POINT('Ctrl Pts',(-50.938555040127,7.01274676059864,-66.0050723994061));
#30567=CARTESIAN_POINT('Ctrl Pts',(-50.938560245344,7.07090482741248,-66.1648314188238));
#30568=CARTESIAN_POINT('Ctrl Pts',(-50.9386359168677,7.16824402500391,-66.428527890208));
#30569=CARTESIAN_POINT('Ctrl Pts',(-50.9371824527114,7.28588624149121,-66.7331492568909));
#30570=CARTESIAN_POINT('Ctrl Pts',(-50.9349525659208,7.52823531103306,-67.3097869512625));
#30571=CARTESIAN_POINT('Ctrl Pts',(-50.9304861349764,7.98794885641103,-68.2981607577382));
#30572=CARTESIAN_POINT('Ctrl Pts',(-50.9230496760407,8.98940213828054,-70.1559710706958));
#30573=CARTESIAN_POINT('Ctrl Pts',(-50.922523410447,9.86476328571874,-71.616315855169));
#30574=CARTESIAN_POINT('Ctrl Pts',(-50.9269629008514,10.4186203997032,-72.668691895132));
#30575=CARTESIAN_POINT('Ctrl Pts',(-50.9265763436931,10.5543070540633,-72.9263651780016));
#30576=CARTESIAN_POINT('Ctrl Pts',(-50.9266081693936,10.8191442348102,-73.4279271585352));
#30577=CARTESIAN_POINT('Ctrl Pts',(-50.9263470769324,11.1537252117817,-74.0596571749007));
#30578=CARTESIAN_POINT('Ctrl Pts',(-50.9262537917075,11.5544067101263,-74.8135397204989));
#30579=CARTESIAN_POINT('Ctrl Pts',(-50.9260447195237,12.3575189311881,-76.3210927366946));
#30580=CARTESIAN_POINT('Ctrl Pts',(-50.9260642885464,13.0268913326518,-77.5736623659616));
#30581=CARTESIAN_POINT('Ctrl Pts',(-50.9262764665433,13.9948297281972,-79.3942546484625));
#30582=CARTESIAN_POINT('Ctrl Pts',(-50.9261813181547,14.4321744477241,-80.2169082365069));
#30583=CARTESIAN_POINT('Ctrl Pts',(-50.9261813181544,14.8686960351134,-81.0378859386059));
#30584=CARTESIAN_POINT('Ctrl Pts',(-48.1081617547539,0.821656359931925,
24.830552683986));
#30585=CARTESIAN_POINT('Ctrl Pts',(-48.1083039636808,0.821672125848511,
24.7816707634521));
#30586=CARTESIAN_POINT('Ctrl Pts',(-48.1084531105878,0.821688653501879,
24.732789784926));
#30587=CARTESIAN_POINT('Ctrl Pts',(-48.1102144775847,0.821884019159318,
24.1821532281473));
#30588=CARTESIAN_POINT('Ctrl Pts',(-48.1115208354339,0.822073222653415,
23.1780001047735));
#30589=CARTESIAN_POINT('Ctrl Pts',(-48.1145318216691,0.822535351985165,
21.1693470838628));
#30590=CARTESIAN_POINT('Ctrl Pts',(-48.126255455966,0.823836447388182,19.6652171497628));
#30591=CARTESIAN_POINT('Ctrl Pts',(-48.1513382795527,0.826399378484051,
18.4141819950539));
#30592=CARTESIAN_POINT('Ctrl Pts',(-48.1633401608167,0.827635914492364,
17.9112439152697));
#30593=CARTESIAN_POINT('Ctrl Pts',(-48.1934269865468,0.830753452240787,
16.9071782974834));
#30594=CARTESIAN_POINT('Ctrl Pts',(-48.2579641279172,0.837425408361244,
15.1533914949236));
#30595=CARTESIAN_POINT('Ctrl Pts',(-48.3196332683591,0.843613068292844,
13.652156435697));
#30596=CARTESIAN_POINT('Ctrl Pts',(-48.3589776117825,0.847210384179055,
12.3982565477228));
#30597=CARTESIAN_POINT('Ctrl Pts',(-48.3751358823534,0.848646943941486,
11.897528758793));
#30598=CARTESIAN_POINT('Ctrl Pts',(-48.4083119188161,0.851471934511271,
10.8960549543969));
#30599=CARTESIAN_POINT('Ctrl Pts',(-48.4662308713391,0.85614738198588,9.14291198624129));
#30600=CARTESIAN_POINT('Ctrl Pts',(-48.5074038448447,0.8592283855912,7.63782893120229));
#30601=CARTESIAN_POINT('Ctrl Pts',(-48.5258475297395,0.860582296955385,
6.5066415629613));
#30602=CARTESIAN_POINT('Ctrl Pts',(-48.5296781633811,0.860845722172545,
6.25655649567007));
#30603=CARTESIAN_POINT('Ctrl Pts',(-48.5363908526945,0.861253424574854,
5.75555852726343));
#30604=CARTESIAN_POINT('Ctrl Pts',(-48.545759656092,0.861687853954917,4.87739075226462));
#30605=CARTESIAN_POINT('Ctrl Pts',(-48.5558977282952,0.861673437671844,
3.11698986917906));
#30606=CARTESIAN_POINT('Ctrl Pts',(-48.5528947975733,0.861079705323928,
1.61023685094202));
#30607=CARTESIAN_POINT('Ctrl Pts',(-48.5480633471258,0.861062762891678,
0.550176309058608));
#30608=CARTESIAN_POINT('Ctrl Pts',(-48.5473893780227,0.861027148752041,
0.424587748163117));
#30609=CARTESIAN_POINT('Ctrl Pts',(-48.5456685819528,0.860841602241671,
0.173139364999722));
#30610=CARTESIAN_POINT('Ctrl Pts',(-48.54174356037,0.860243995795441,-0.266434695632504));
#30611=CARTESIAN_POINT('Ctrl Pts',(-48.5338902708593,0.858800861815022,
-0.893677263874593));
#30612=CARTESIAN_POINT('Ctrl Pts',(-48.5220464083315,0.856663839146366,
-1.64617418074009));
#30613=CARTESIAN_POINT('Ctrl Pts',(-48.5045928368554,0.854088087482596,
-2.64919303917013));
#30614=CARTESIAN_POINT('Ctrl Pts',(-48.4825861334336,0.852765003354847,
-3.90421055258685));
#30615=CARTESIAN_POINT('Ctrl Pts',(-48.4708072113734,0.856709284057601,
-4.91207362175905));
#30616=CARTESIAN_POINT('Ctrl Pts',(-48.467174598008,0.861488882626109,-5.54220041312295));
#30617=CARTESIAN_POINT('Ctrl Pts',(-48.4656412820237,0.860176842610061,
-5.74937675803637));
#30618=CARTESIAN_POINT('Ctrl Pts',(-48.4623409990297,0.847828554841079,
-6.20559665179427));
#30619=CARTESIAN_POINT('Ctrl Pts',(-48.4566143171184,0.805000196574491,
-7.02775369438753));
#30620=CARTESIAN_POINT('Ctrl Pts',(-48.4512568492943,0.714582313920764,
-8.31564021221516));
#30621=CARTESIAN_POINT('Ctrl Pts',(-48.4548272637197,0.695021109452357,
-9.7389343685648));
#30622=CARTESIAN_POINT('Ctrl Pts',(-48.462384639111,0.797115569315175,-10.8079866159256));
#30623=CARTESIAN_POINT('Ctrl Pts',(-48.4674826334621,0.901596608971655,
-11.4354946003987));
#30624=CARTESIAN_POINT('Ctrl Pts',(-48.4701010695859,0.971232007744518,
-11.754049685775));
#30625=CARTESIAN_POINT('Ctrl Pts',(-48.4719964958873,1.03104359761252,-11.9955612518357));
#30626=CARTESIAN_POINT('Ctrl Pts',(-48.473529106806,1.07554150145775,-12.1651151016405));
#30627=CARTESIAN_POINT('Ctrl Pts',(-48.4781623142853,1.17300632768884,-12.4927722796286));
#30628=CARTESIAN_POINT('Ctrl Pts',(-48.489511688992,1.36611982186439,-13.052242725534));
#30629=CARTESIAN_POINT('Ctrl Pts',(-48.5308112607914,1.95530334230472,-14.4053170494689));
#30630=CARTESIAN_POINT('Ctrl Pts',(-48.5888559408709,2.7580852490192,-15.7095673420877));
#30631=CARTESIAN_POINT('Ctrl Pts',(-48.6283106335618,3.45801560557731,-16.8861968690548));
#30632=CARTESIAN_POINT('Ctrl Pts',(-48.6397409855395,3.765486400292,-17.4418615068456));
#30633=CARTESIAN_POINT('Ctrl Pts',(-48.6403024516574,3.97332766253734,-17.8666528805007));
#30634=CARTESIAN_POINT('Ctrl Pts',(-48.636912362217,4.06262286490203,-18.071547516743));
#30635=CARTESIAN_POINT('Ctrl Pts',(-48.632474912663,4.12340082888935,-18.2226153488267));
#30636=CARTESIAN_POINT('Ctrl Pts',(-48.6235145806418,4.17460316445271,-18.3555032689312));
#30637=CARTESIAN_POINT('Ctrl Pts',(-48.605596754408,4.268448050428,-18.6016985693474));
#30638=CARTESIAN_POINT('Ctrl Pts',(-48.5822050597156,4.3620306439826,-18.8545106578251));
#30639=CARTESIAN_POINT('Ctrl Pts',(-48.5555267249322,4.45148589084385,-19.1026422173759));
#30640=CARTESIAN_POINT('Ctrl Pts',(-48.5371827717206,4.50653850905639,-19.2581435796158));
#30641=CARTESIAN_POINT('Ctrl Pts',(-48.5216922566285,4.54977261479859,-19.381926994986));
#30642=CARTESIAN_POINT('Ctrl Pts',(-48.5056253886663,4.59257722741495,-19.5055887283884));
#30643=CARTESIAN_POINT('Ctrl Pts',(-48.4592200249797,4.70838941295987,-19.8446811813429));
#30644=CARTESIAN_POINT('Ctrl Pts',(-48.3717713410061,4.8876721721689,-20.3938681940595));
#30645=CARTESIAN_POINT('Ctrl Pts',(-48.1941620970936,5.1778872714237,-21.3486426272371));
#30646=CARTESIAN_POINT('Ctrl Pts',(-47.9526707384724,5.48953943497499,-22.4918864970005));
#30647=CARTESIAN_POINT('Ctrl Pts',(-47.8049933853911,5.67655780766664,-23.3546093073591));
#30648=CARTESIAN_POINT('Ctrl Pts',(-47.7509567118304,5.76175622151436,-23.8814288993932));
#30649=CARTESIAN_POINT('Ctrl Pts',(-47.73173689534,5.7886209866703,-24.0780477136886));
#30650=CARTESIAN_POINT('Ctrl Pts',(-47.6999262884633,5.8318768540918,-24.4891274562849));
#30651=CARTESIAN_POINT('Ctrl Pts',(-47.6611936995658,5.87571409871005,-25.2313155480994));
#30652=CARTESIAN_POINT('Ctrl Pts',(-47.6459111880626,5.86167981157645,-26.3718474704576));
#30653=CARTESIAN_POINT('Ctrl Pts',(-47.661058373748,5.77950696427442,-27.8554510831928));
#30654=CARTESIAN_POINT('Ctrl Pts',(-47.6739998276547,5.73644434286673,-28.9197758632713));
#30655=CARTESIAN_POINT('Ctrl Pts',(-47.6766918803409,5.73425012421519,-29.5379474946004));
#30656=CARTESIAN_POINT('Ctrl Pts',(-47.6774591617782,5.73378010778106,-29.6585572612093));
#30657=CARTESIAN_POINT('Ctrl Pts',(-47.6795712553516,5.73262182581156,-29.9093968540346));
#30658=CARTESIAN_POINT('Ctrl Pts',(-47.684742928468,5.73015329550106,-30.3440131851773));
#30659=CARTESIAN_POINT('Ctrl Pts',(-47.7003265643364,5.72372749685039,-31.2185001382784));
#30660=CARTESIAN_POINT('Ctrl Pts',(-47.7273744004624,5.71430071429274,-32.2189124389907));
#30661=CARTESIAN_POINT('Ctrl Pts',(-47.757903427418,5.70528168254876,-33.2224570918928));
#30662=CARTESIAN_POINT('Ctrl Pts',(-47.7810759779801,5.69915006762253,-33.9756302585514));
#30663=CARTESIAN_POINT('Ctrl Pts',(-47.8031029240017,5.69388154659206,-34.7292141379704));
#30664=CARTESIAN_POINT('Ctrl Pts',(-47.8160341705809,5.69115517646488,-35.2316463250507));
#30665=CARTESIAN_POINT('Ctrl Pts',(-47.8247247489547,5.68946889060385,-35.6094062744765));
#30666=CARTESIAN_POINT('Ctrl Pts',(-47.8306323129823,5.68830749268304,-35.8606118864872));
#30667=CARTESIAN_POINT('Ctrl Pts',(-47.8426811389759,5.68614016568386,-36.363486472667));
#30668=CARTESIAN_POINT('Ctrl Pts',(-47.8642643869878,5.68250296983621,-37.2416836110121));
#30669=CARTESIAN_POINT('Ctrl Pts',(-47.9075934048008,5.67667099570877,-38.9955257562694));
#30670=CARTESIAN_POINT('Ctrl Pts',(-47.9400147345898,5.67388707997918,-40.5001945577602));
#30671=CARTESIAN_POINT('Ctrl Pts',(-47.9565066550077,5.67372202887156,-41.635163653271));
#30672=CARTESIAN_POINT('Ctrl Pts',(-47.9599386496466,5.67356269835911,-41.8832164151772));
#30673=CARTESIAN_POINT('Ctrl Pts',(-47.9645610192146,5.67294174472812,-42.257684476039));
#30674=CARTESIAN_POINT('Ctrl Pts',(-47.9686903533609,5.67206761727831,-42.6326046825154));
#30675=CARTESIAN_POINT('Ctrl Pts',(-47.9736025573532,5.67069401156819,-43.1339401996902));
#30676=CARTESIAN_POINT('Ctrl Pts',(-47.9787312416865,5.66886933253452,-43.7625304581063));
#30677=CARTESIAN_POINT('Ctrl Pts',(-47.9836100894013,5.66737379968377,-44.519631153679));
#30678=CARTESIAN_POINT('Ctrl Pts',(-47.9868967370082,5.66743536136416,-45.1523662815642));
#30679=CARTESIAN_POINT('Ctrl Pts',(-47.9892190368056,5.66874051397247,-45.6593910470067));
#30680=CARTESIAN_POINT('Ctrl Pts',(-47.9908537750947,5.67044657197521,-46.0400313854599));
#30681=CARTESIAN_POINT('Ctrl Pts',(-47.9924228333032,5.67299423348329,-46.4209581938724));
#30682=CARTESIAN_POINT('Ctrl Pts',(-47.9944851694717,5.67766910053647,-46.929228720508));
#30683=CARTESIAN_POINT('Ctrl Pts',(-47.9960584325483,5.68276825329085,-47.3105867491211));
#30684=CARTESIAN_POINT('Ctrl Pts',(-47.9977427003301,5.68919643937715,-47.6933809474625));
#30685=CARTESIAN_POINT('Ctrl Pts',(-47.9986800935609,5.69530034202098,-47.9631886151501));
#30686=CARTESIAN_POINT('Ctrl Pts',(-48.0000606907457,5.71252845744749,-48.4892800747684));
#30687=CARTESIAN_POINT('Ctrl Pts',(-48.0013833800003,5.7534559225999,-49.4003811610625));
#30688=CARTESIAN_POINT('Ctrl Pts',(-48.0016186359631,5.82668280043133,-50.6595265053002));
#30689=CARTESIAN_POINT('Ctrl Pts',(-48.0031279455766,5.89225151943146,-52.1071552929537));
#30690=CARTESIAN_POINT('Ctrl Pts',(-48.0068413553413,5.89412700469785,-53.0269293633755));
#30691=CARTESIAN_POINT('Ctrl Pts',(-48.0104999550757,5.87504627401801,-53.5877251204438));
#30692=CARTESIAN_POINT('Ctrl Pts',(-48.0119186947241,5.8644984398709,-53.7870157793957));
#30693=CARTESIAN_POINT('Ctrl Pts',(-48.015236046728,5.82868565785535,-54.2180167794228));
#30694=CARTESIAN_POINT('Ctrl Pts',(-48.0223405541487,5.73182312345919,-55.0028496725892));
#30695=CARTESIAN_POINT('Ctrl Pts',(-48.0422819205056,5.44381604950419,-56.7239446729538));
#30696=CARTESIAN_POINT('Ctrl Pts',(-48.0652320306938,5.19648912835514,-58.4362411887274));
#30697=CARTESIAN_POINT('Ctrl Pts',(-48.072145366917,5.27833872248682,-59.7711023692122));
#30698=CARTESIAN_POINT('Ctrl Pts',(-48.0730810994228,5.28813022272174,-59.9127033359094));
#30699=CARTESIAN_POINT('Ctrl Pts',(-48.0748143844032,5.31227047765825,-60.2063755436483));
#30700=CARTESIAN_POINT('Ctrl Pts',(-48.0776908225279,5.36413329883143,-60.7119580011442));
#30701=CARTESIAN_POINT('Ctrl Pts',(-48.0827259548146,5.50557705051933,-61.7166455841316));
#30702=CARTESIAN_POINT('Ctrl Pts',(-48.0870712175635,5.74234063614827,-62.8361337598059));
#30703=CARTESIAN_POINT('Ctrl Pts',(-48.0902785989789,6.03499269362514,-63.9282626842282));
#30704=CARTESIAN_POINT('Ctrl Pts',(-48.09170694666,6.21721384595243,-64.5313341753743));
#30705=CARTESIAN_POINT('Ctrl Pts',(-48.0925230603127,6.34465176117515,-64.9287143411935));
#30706=CARTESIAN_POINT('Ctrl Pts',(-48.0930339900168,6.43110769486847,-65.1923324264293));
#30707=CARTESIAN_POINT('Ctrl Pts',(-48.0934898782398,6.519711978698,-65.4541244578588));
#30708=CARTESIAN_POINT('Ctrl Pts',(-48.0938525513821,6.59884897317687,-65.6814255430501));
#30709=CARTESIAN_POINT('Ctrl Pts',(-48.0940492907279,6.64449948092765,-65.8108129567606));
#30710=CARTESIAN_POINT('Ctrl Pts',(-48.0943334109498,6.71339881074584,-66.0044194815105));
#30711=CARTESIAN_POINT('Ctrl Pts',(-48.0945493743175,6.77163076478862,-66.1646832795354));
#30712=CARTESIAN_POINT('Ctrl Pts',(-48.0948612361393,6.8692076981214,-66.4292745880487));
#30713=CARTESIAN_POINT('Ctrl Pts',(-48.0938879421657,6.98676580433808,-66.7337926781003));
#30714=CARTESIAN_POINT('Ctrl Pts',(-48.0923778740631,7.22916551376678,-67.3107614717401));
#30715=CARTESIAN_POINT('Ctrl Pts',(-48.0889925647051,7.68892715311023,-68.299331484953));
#30716=CARTESIAN_POINT('Ctrl Pts',(-48.0826672547797,8.69063589248501,-70.1574981028561));
#30717=CARTESIAN_POINT('Ctrl Pts',(-48.0816700834379,9.5660147444683,-71.6177387695598));
#30718=CARTESIAN_POINT('Ctrl Pts',(-48.0855496326223,10.1195965515549,-72.669938484722));
#30719=CARTESIAN_POINT('Ctrl Pts',(-48.0852320074524,10.2552979808535,-72.9276394485621));
#30720=CARTESIAN_POINT('Ctrl Pts',(-48.0852797639747,10.5201259530456,-73.4292165411084));
#30721=CARTESIAN_POINT('Ctrl Pts',(-48.0850686567843,10.8547201758687,-74.0609738365155));
#30722=CARTESIAN_POINT('Ctrl Pts',(-48.0849890234844,11.2554147473501,-74.8148760797214));
#30723=CARTESIAN_POINT('Ctrl Pts',(-48.0847893538615,12.0585656117152,-76.3224589816106));
#30724=CARTESIAN_POINT('Ctrl Pts',(-48.0847638687617,12.727967876092,-77.5750096594133));
#30725=CARTESIAN_POINT('Ctrl Pts',(-48.0849471552217,13.6958775601037,-79.395550472923));
#30726=CARTESIAN_POINT('Ctrl Pts',(-48.0848645544605,14.1332336032719,-80.2182152143253));
#30727=CARTESIAN_POINT('Ctrl Pts',(-48.0848645544601,14.5697551906614,-81.0391929164233));
#30728=CARTESIAN_POINT('Ctrl Pts',(-45.2615345930742,0.568923653316842,
24.8305649181971));
#30729=CARTESIAN_POINT('Ctrl Pts',(-45.2616723458727,0.56893639381907,24.7816834208571));
#30730=CARTESIAN_POINT('Ctrl Pts',(-45.2618168168555,0.568949748036691,
24.7328028847575));
#30731=CARTESIAN_POINT('Ctrl Pts',(-45.2635227928271,0.569107674888664,
24.1821708638069));
#30732=CARTESIAN_POINT('Ctrl Pts',(-45.2648687934348,0.569263618641808,
23.1780301850203));
#30733=CARTESIAN_POINT('Ctrl Pts',(-45.2680271544534,0.56964532707125,21.1693806216249));
#30734=CARTESIAN_POINT('Ctrl Pts',(-45.2793788855699,0.57069704852392,19.6652250009272));
#30735=CARTESIAN_POINT('Ctrl Pts',(-45.3032612861431,0.572754317085861,
18.4141650801884));
#30736=CARTESIAN_POINT('Ctrl Pts',(-45.3147245804852,0.573757913519431,
17.9112021425638));
#30737=CARTESIAN_POINT('Ctrl Pts',(-45.343524261982,0.57630797389634,16.90712294505));
#30738=CARTESIAN_POINT('Ctrl Pts',(-45.4052807106741,0.581771843525628,
15.1533712283448));
#30739=CARTESIAN_POINT('Ctrl Pts',(-45.4637749100727,0.586723142739833,
13.652199025009));
#30740=CARTESIAN_POINT('Ctrl Pts',(-45.5001367390707,0.589383332340141,
12.3983651401701));
#30741=CARTESIAN_POINT('Ctrl Pts',(-45.5149616963227,0.590420663495616,
11.8976629685695));
#30742=CARTESIAN_POINT('Ctrl Pts',(-45.5450626839958,0.592375140886463,
10.8962020014157));
#30743=CARTESIAN_POINT('Ctrl Pts',(-45.5969183131899,0.595422785932535,
9.14302426569176));
#30744=CARTESIAN_POINT('Ctrl Pts',(-45.6331060963251,0.597204544866204,
7.63779283188048));
#30745=CARTESIAN_POINT('Ctrl Pts',(-45.6492210307351,0.597934723316499,
6.50656027802753));
#30746=CARTESIAN_POINT('Ctrl Pts',(-45.65252979313,0.598063469500555,6.25653232565011));
#30747=CARTESIAN_POINT('Ctrl Pts',(-45.6581926980207,0.598199683729433,
5.75559249943098));
#30748=CARTESIAN_POINT('Ctrl Pts',(-45.6657464934642,0.598162253780016,
4.87748364246271));
#30749=CARTESIAN_POINT('Ctrl Pts',(-45.6726272003006,0.597307704815268,
3.11705192901595));
#30750=CARTESIAN_POINT('Ctrl Pts',(-45.6685501368452,0.596356338009474,
1.60983415283903));
#30751=CARTESIAN_POINT('Ctrl Pts',(-45.6649011830657,0.596693744906996,
0.549181970152154));
#30752=CARTESIAN_POINT('Ctrl Pts',(-45.6644106870089,0.596736979590196,
0.422841734534823));
#30753=CARTESIAN_POINT('Ctrl Pts',(-45.6632187310025,0.596838489702751,
0.170391518020105));
#30754=CARTESIAN_POINT('Ctrl Pts',(-45.6606080667276,0.597052402569735,
-0.270865388521122));
#30755=CARTESIAN_POINT('Ctrl Pts',(-45.6555447983622,0.597453307539356,
-0.899661574341966));
#30756=CARTESIAN_POINT('Ctrl Pts',(-45.6478740955046,0.598048487429573,
-1.65267183829421));
#30757=CARTESIAN_POINT('Ctrl Pts',(-45.6362241180025,0.598951491118354,
-2.65459475895867));
#30758=CARTESIAN_POINT('Ctrl Pts',(-45.6203342687638,0.600156051117981,
-3.90475578181039));
#30759=CARTESIAN_POINT('Ctrl Pts',(-45.6091709952231,0.601137200513604,
-4.90501268537487));
#30760=CARTESIAN_POINT('Ctrl Pts',(-45.6035954437551,0.601759966525794,
-5.52991529103675));
#30761=CARTESIAN_POINT('Ctrl Pts',(-45.6006108814509,0.599729253591517,
-5.74989315896313));
#30762=CARTESIAN_POINT('Ctrl Pts',(-45.5922177925495,0.588103576083817,
-6.21834474534208));
#30763=CARTESIAN_POINT('Ctrl Pts',(-45.5727398228785,0.551803838808369,
-7.05489906573956));
#30764=CARTESIAN_POINT('Ctrl Pts',(-45.5400034086817,0.478480237096733,
-8.3289803346879));
#30765=CARTESIAN_POINT('Ctrl Pts',(-45.5231977388069,0.451676003483263,
-9.69594050140588));
#30766=CARTESIAN_POINT('Ctrl Pts',(-45.5312196791262,0.505876456142413,
-10.7037545406741));
#30767=CARTESIAN_POINT('Ctrl Pts',(-45.5428674671062,0.56588976699614,-11.2928459671084));
#30768=CARTESIAN_POINT('Ctrl Pts',(-45.5512155153025,0.607023081755394,
-11.5918143476826));
#30769=CARTESIAN_POINT('Ctrl Pts',(-45.5585084115334,0.642699657012322,
-11.8182084602322));
#30770=CARTESIAN_POINT('Ctrl Pts',(-45.564432885722,0.66595079654557,-11.96161215553));
#30771=CARTESIAN_POINT('Ctrl Pts',(-45.579301145316,0.717617991143493,-12.2518240391153));
#30772=CARTESIAN_POINT('Ctrl Pts',(-45.6125589798245,0.818560777400114,
-12.7533508080639));
#30773=CARTESIAN_POINT('Ctrl Pts',(-45.7295753087123,1.13208082807272,-14.026005831991));
#30774=CARTESIAN_POINT('Ctrl Pts',(-45.8977342546569,1.62991439444617,-15.3629814934345));
#30775=CARTESIAN_POINT('Ctrl Pts',(-45.9896689963964,2.1742378659247,-16.6449845617281));
#30776=CARTESIAN_POINT('Ctrl Pts',(-46.0127255866054,2.44684675915175,-17.2789902088887));
#30777=CARTESIAN_POINT('Ctrl Pts',(-46.0139719522059,2.66002778840069,-17.7842019315097));
#30778=CARTESIAN_POINT('Ctrl Pts',(-46.0086322280254,2.76387905082651,-18.0364848019655));
#30779=CARTESIAN_POINT('Ctrl Pts',(-46.0020276494765,2.84044587158191,-18.2258896669335));
#30780=CARTESIAN_POINT('Ctrl Pts',(-45.9916442991187,2.90255746472163,-18.3814126264322));
#30781=CARTESIAN_POINT('Ctrl Pts',(-45.9710572595573,3.02410551438022,-18.670089280978));
#30782=CARTESIAN_POINT('Ctrl Pts',(-45.9455273169221,3.1524972413311,-18.9598642552261));
#30783=CARTESIAN_POINT('Ctrl Pts',(-45.917597839482,3.2829544276836,-19.2407969343877));
#30784=CARTESIAN_POINT('Ctrl Pts',(-45.8989127160357,3.36586638758757,-19.4150986453484));
#30785=CARTESIAN_POINT('Ctrl Pts',(-45.8834412884027,3.43259720471774,-19.5530188450265));
#30786=CARTESIAN_POINT('Ctrl Pts',(-45.8676010038037,3.49963796574981,-19.6902312656681));
#30787=CARTESIAN_POINT('Ctrl Pts',(-45.8226911728824,3.68495541061571,-20.0642598939347));
#30788=CARTESIAN_POINT('Ctrl Pts',(-45.7429920353979,3.99094061991361,-20.6593839193205));
#30789=CARTESIAN_POINT('Ctrl Pts',(-45.5941611777489,4.5158905048341,-21.6696940569923));
#30790=CARTESIAN_POINT('Ctrl Pts',(-45.4103185036997,5.08397172095285,-22.8408731099591));
#30791=CARTESIAN_POINT('Ctrl Pts',(-45.2952033585105,5.35220520103119,-23.6349105739773));
#30792=CARTESIAN_POINT('Ctrl Pts',(-45.2470258602545,5.45367407042719,-24.0675321019981));
#30793=CARTESIAN_POINT('Ctrl Pts',(-45.2275642403591,5.49554360971262,-24.2646881816929));
#30794=CARTESIAN_POINT('Ctrl Pts',(-45.1897213634604,5.56191922129806,-24.6530653715348));
#30795=CARTESIAN_POINT('Ctrl Pts',(-45.126169787784,5.64579968547833,-25.3632536240763));
#30796=CARTESIAN_POINT('Ctrl Pts',(-45.0485809628158,5.68330120258022,-26.4538851411555));
#30797=CARTESIAN_POINT('Ctrl Pts',(-44.9827225203447,5.65136303060178,-27.9001949288379));
#30798=CARTESIAN_POINT('Ctrl Pts',(-44.9521248674338,5.6293916709228,-28.949492421806));
#30799=CARTESIAN_POINT('Ctrl Pts',(-44.9367599336799,5.63616027776272,-29.5612290563094));
#30800=CARTESIAN_POINT('Ctrl Pts',(-44.9335170536817,5.63713457503584,-29.6743255452956));
#30801=CARTESIAN_POINT('Ctrl Pts',(-44.9278388436267,5.63805208961385,-29.9142811768491));
#30802=CARTESIAN_POINT('Ctrl Pts',(-44.9198488782374,5.63668801870017,-30.3297606990247));
#30803=CARTESIAN_POINT('Ctrl Pts',(-44.9109910089194,5.62340525515849,-31.1739498277202));
#30804=CARTESIAN_POINT('Ctrl Pts',(-44.9136021605173,5.58905379630781,-32.1537761072688));
#30805=CARTESIAN_POINT('Ctrl Pts',(-44.9221536485736,5.54708312381198,-33.151610222345));
#30806=CARTESIAN_POINT('Ctrl Pts',(-44.9298865257232,5.51492405417621,-33.9076686728183));
#30807=CARTESIAN_POINT('Ctrl Pts',(-44.9372328903042,5.48530913853536,-34.6714518503932));
#30808=CARTESIAN_POINT('Ctrl Pts',(-44.9407885305601,5.46943186190011,-35.1856910262279));
#30809=CARTESIAN_POINT('Ctrl Pts',(-44.9425441216053,5.45980858080541,-35.5739854943983));
#30810=CARTESIAN_POINT('Ctrl Pts',(-44.9438779864364,5.45366779071273,-35.8236942203539));
#30811=CARTESIAN_POINT('Ctrl Pts',(-44.9471787513647,5.44144439102455,-36.3285083384014));
#30812=CARTESIAN_POINT('Ctrl Pts',(-44.9543182354928,5.42068637952117,-37.2078627950992));
#30813=CARTESIAN_POINT('Ctrl Pts',(-44.9725136640791,5.38222432218129,-38.9666810450322));
#30814=CARTESIAN_POINT('Ctrl Pts',(-44.988587990644,5.35608797243692,-40.4758943628781));
#30815=CARTESIAN_POINT('Ctrl Pts',(-44.9949719986201,5.34203825053049,-41.6149771521622));
#30816=CARTESIAN_POINT('Ctrl Pts',(-44.9962209741261,5.33888938097108,-41.8633286625312));
#30817=CARTESIAN_POINT('Ctrl Pts',(-44.9976487140526,5.33392929542106,-42.2386401419984));
#30818=CARTESIAN_POINT('Ctrl Pts',(-44.9987078765806,5.32890196674228,-42.6143871354106));
#30819=CARTESIAN_POINT('Ctrl Pts',(-44.9997164946637,5.32225541986517,-43.1170091303405));
#30820=CARTESIAN_POINT('Ctrl Pts',(-45.0004034480282,5.31439673661683,-43.7474301700452));
#30821=CARTESIAN_POINT('Ctrl Pts',(-45.000868285242,5.30671511110962,-44.5071548518077));
#30822=CARTESIAN_POINT('Ctrl Pts',(-45.0014224520297,5.30264469307216,-45.1424238784898));
#30823=CARTESIAN_POINT('Ctrl Pts',(-45.0022711041608,5.30134971650009,-45.6517276051057));
#30824=CARTESIAN_POINT('Ctrl Pts',(-45.0031683624121,5.30147692668183,-46.0341874242821));
#30825=CARTESIAN_POINT('Ctrl Pts',(-45.0043982702481,5.302839018119,-46.4170469581394));
#30826=CARTESIAN_POINT('Ctrl Pts',(-45.0065803989924,5.30648560360591,-46.9280543328961));
#30827=CARTESIAN_POINT('Ctrl Pts',(-45.0089112966019,5.31146635095098,-47.3116150666946));
#30828=CARTESIAN_POINT('Ctrl Pts',(-45.0118707869184,5.3182531796772,-47.6967600511927));
#30829=CARTESIAN_POINT('Ctrl Pts',(-45.013909593286,5.32485825500584,-47.9686672018424));
#30830=CARTESIAN_POINT('Ctrl Pts',(-45.0183049428734,5.34390019871555,-48.4982682740304));
#30831=CARTESIAN_POINT('Ctrl Pts',(-45.0267916828321,5.38990717621575,-49.4147594958146));
#30832=CARTESIAN_POINT('Ctrl Pts',(-45.0413469150811,5.47438659865881,-50.6789313209984));
#30833=CARTESIAN_POINT('Ctrl Pts',(-45.0626179306112,5.55591976262862,-52.1287880158482));
#30834=CARTESIAN_POINT('Ctrl Pts',(-45.0792744990489,5.56824779334821,-53.047472923302));
#30835=CARTESIAN_POINT('Ctrl Pts',(-45.0903088412658,5.55518331394269,-53.6068866561389));
#30836=CARTESIAN_POINT('Ctrl Pts',(-45.0949604559406,5.54685392911716,-53.8080038405276));
#30837=CARTESIAN_POINT('Ctrl Pts',(-45.1051935354558,5.51631442715935,-54.2407427058968));
#30838=CARTESIAN_POINT('Ctrl Pts',(-45.1253875800908,5.43020787584997,-55.0280992059488));
#30839=CARTESIAN_POINT('Ctrl Pts',(-45.1724343081567,5.16829959423166,-56.7498442628009));
#30840=CARTESIAN_POINT('Ctrl Pts',(-45.2150323715158,4.94541364590222,-58.4563942878425));
#30841=CARTESIAN_POINT('Ctrl Pts',(-45.229079940856,5.03428012136371,-59.7812103826349));
#30842=CARTESIAN_POINT('Ctrl Pts',(-45.2308059711601,5.0447516841388,-59.9217813236452));
#30843=CARTESIAN_POINT('Ctrl Pts',(-45.2339258062422,5.07004070521539,-60.2134142346763));
#30844=CARTESIAN_POINT('Ctrl Pts',(-45.2387137009182,5.12323156118997,-60.7157770799439));
#30845=CARTESIAN_POINT('Ctrl Pts',(-45.2457313086932,5.26509173462011,-61.7152178901686));
#30846=CARTESIAN_POINT('Ctrl Pts',(-45.2491207511983,5.49878674246531,-62.8315177848284));
#30847=CARTESIAN_POINT('Ctrl Pts',(-45.2501521594165,5.78765739615891,-63.9229299880029));
#30848=CARTESIAN_POINT('Ctrl Pts',(-45.2502525085497,5.96793885408008,-64.5264537867342));
#30849=CARTESIAN_POINT('Ctrl Pts',(-45.2502885274417,6.09435349669486,-64.9244694933693));
#30850=CARTESIAN_POINT('Ctrl Pts',(-45.2503156383113,6.18020953797663,-65.1885989491818));
#30851=CARTESIAN_POINT('Ctrl Pts',(-45.2503590074845,6.26835846071443,-65.4510299828515));
#30852=CARTESIAN_POINT('Ctrl Pts',(-45.2504452439476,6.34725184610613,-65.6790016185538));
#30853=CARTESIAN_POINT('Ctrl Pts',(-45.2505118720077,6.39281215966707,-65.8088036964063));
#30854=CARTESIAN_POINT('Ctrl Pts',(-45.2506305029969,6.46162677822535,-66.0030624735293));
#30855=CARTESIAN_POINT('Ctrl Pts',(-45.2507736039379,6.51990099608607,-66.1639364315662));
#30856=CARTESIAN_POINT('Ctrl Pts',(-45.2510741641748,6.6177086878099,-66.4295992762849));
#30857=CARTESIAN_POINT('Ctrl Pts',(-45.250321477465,6.73509315111427,-66.7340020498313));
#30858=CARTESIAN_POINT('Ctrl Pts',(-45.249119758346,6.97744203040324,-67.3113803339706));
#30859=CARTESIAN_POINT('Ctrl Pts',(-45.2463020674733,7.43710776352219,-68.3002085477061));
#30860=CARTESIAN_POINT('Ctrl Pts',(-45.240708715144,8.43898108975228,-70.1588293463694));
#30861=CARTESIAN_POINT('Ctrl Pts',(-45.2394128134625,9.31441095850817,-71.6189345572044));
#30862=CARTESIAN_POINT('Ctrl Pts',(-45.2425963587864,9.86768814163015,-72.6709320003031));
#30863=CARTESIAN_POINT('Ctrl Pts',(-45.242318918496,10.0033992160793,-72.928669941724));
#30864=CARTESIAN_POINT('Ctrl Pts',(-45.2423411399073,10.2682109987263,-73.4302705769965));
#30865=CARTESIAN_POINT('Ctrl Pts',(-45.2421524693102,10.6028146584613,-74.0620653647392));
#30866=CARTESIAN_POINT('Ctrl Pts',(-45.2420837499708,11.0035248370368,-74.8159945743116));
#30867=CARTESIAN_POINT('Ctrl Pts',(-45.2419300164671,11.8067277607913,-76.3236157009755));
#30868=CARTESIAN_POINT('Ctrl Pts',(-45.2419413548527,12.476175379063,-77.5761363944957));
#30869=CARTESIAN_POINT('Ctrl Pts',(-45.2420965906919,13.444046814902,-79.3966073326402));
#30870=CARTESIAN_POINT('Ctrl Pts',(-45.2420269735312,13.881415378809,-80.219287048203));
#30871=CARTESIAN_POINT('Ctrl Pts',(-45.2420269735315,14.3179369661985,-81.0402647503008));
#30872=CARTESIAN_POINT('Ctrl Pts',(-42.8889107614918,0.396069854539573,
24.8306499092207));
#30873=CARTESIAN_POINT('Ctrl Pts',(-42.8890409472221,0.396078250577575,
24.7817710962967));
#30874=CARTESIAN_POINT('Ctrl Pts',(-42.889177481851,0.396087052970513,24.7328933096333));
#30875=CARTESIAN_POINT('Ctrl Pts',(-42.8907898049868,0.396191175579392,
24.1822922709228));
#30876=CARTESIAN_POINT('Ctrl Pts',(-42.8920476582943,0.396261310671983,
23.1781820957105));
#30877=CARTESIAN_POINT('Ctrl Pts',(-42.8949896800306,0.396415381007176,
21.1695908064305));
#30878=CARTESIAN_POINT('Ctrl Pts',(-42.905718534153,0.397110116062497,19.6654456243867));
#30879=CARTESIAN_POINT('Ctrl Pts',(-42.9283626135728,0.398632648763516,
18.4143922632001));
#30880=CARTESIAN_POINT('Ctrl Pts',(-42.9392337126744,0.399361970835517,
17.9115967319916));
#30881=CARTESIAN_POINT('Ctrl Pts',(-42.9665506853066,0.401193597804371,
16.9076321680773));
#30882=CARTESIAN_POINT('Ctrl Pts',(-43.0251392083456,0.405128861753337,
15.1538536921797));
#30883=CARTESIAN_POINT('Ctrl Pts',(-43.0806351134471,0.40889600092376,13.652114312685));
#30884=CARTESIAN_POINT('Ctrl Pts',(-43.1151374652814,0.411298449155565,
12.39756559081));
#30885=CARTESIAN_POINT('Ctrl Pts',(-43.1292109879026,0.412286158686825,
11.8965753436264));
#30886=CARTESIAN_POINT('Ctrl Pts',(-43.157799097833,0.414317517348359,10.8946870573607));
#30887=CARTESIAN_POINT('Ctrl Pts',(-43.20706598892,0.417869362120652,9.14109869268271));
#30888=CARTESIAN_POINT('Ctrl Pts',(-43.2413947466429,0.420389756470078,
7.63604088896889));
#30889=CARTESIAN_POINT('Ctrl Pts',(-43.256602039586,0.421503566320526,6.50522218228596));
#30890=CARTESIAN_POINT('Ctrl Pts',(-43.2597224872715,0.421733781313164,
6.25498871804423));
#30891=CARTESIAN_POINT('Ctrl Pts',(-43.2650504875047,0.422134349062575,
5.75387948222069));
#30892=CARTESIAN_POINT('Ctrl Pts',(-43.2721220238125,0.422687100151175,
4.87552731214186));
#30893=CARTESIAN_POINT('Ctrl Pts',(-43.2784194879523,0.423255845091349,
3.11535973815131));
#30894=CARTESIAN_POINT('Ctrl Pts',(-43.274315924288,0.423057704554917,1.60922363435097));
#30895=CARTESIAN_POINT('Ctrl Pts',(-43.2706427662616,0.422748404666616,
0.550030671665346));
#30896=CARTESIAN_POINT('Ctrl Pts',(-43.2701595719556,0.422707204277705,
0.423860675108253));
#30897=CARTESIAN_POINT('Ctrl Pts',(-43.269016774996,0.422610273212511,0.171737684639995));
#30898=CARTESIAN_POINT('Ctrl Pts',(-43.2665760293404,0.42240324124909,-0.268981603410207));
#30899=CARTESIAN_POINT('Ctrl Pts',(-43.2619490022914,0.422015480510026,
-0.897168941895786));
#30900=CARTESIAN_POINT('Ctrl Pts',(-43.2549691537298,0.42142408674007,-1.64956521349317));
#30901=CARTESIAN_POINT('Ctrl Pts',(-43.2442733407787,0.420531584961871,
-2.65104169285572));
#30902=CARTESIAN_POINT('Ctrl Pts',(-43.2292854654237,0.419295148862323,
-3.90125771123846));
#30903=CARTESIAN_POINT('Ctrl Pts',(-43.2175701879556,0.418343911838244,
-4.90193027537972));
#30904=CARTESIAN_POINT('Ctrl Pts',(-43.2109790319918,0.417761881888926,
-5.52777685401367));
#30905=CARTESIAN_POINT('Ctrl Pts',(-43.2075375110887,0.416182369454823,
-5.76115929569839));
#30906=CARTESIAN_POINT('Ctrl Pts',(-43.1980371664098,0.408543968449964,
-6.24417082539291));
#30907=CARTESIAN_POINT('Ctrl Pts',(-43.1761218601326,0.385936981481704,
-7.09905037037054));
#30908=CARTESIAN_POINT('Ctrl Pts',(-43.1386135133381,0.34225609408002,-8.36515361030123));
#30909=CARTESIAN_POINT('Ctrl Pts',(-43.116395210378,0.325805827361278,-9.68282802245736));
#30910=CARTESIAN_POINT('Ctrl Pts',(-43.1211039919704,0.353517782545892,
-10.6331211566615));
#30911=CARTESIAN_POINT('Ctrl Pts',(-43.1312872417939,0.384608831349905,
-11.1834209787052));
#30912=CARTESIAN_POINT('Ctrl Pts',(-43.1391431884441,0.405967964406648,
-11.4612161011621));
#30913=CARTESIAN_POINT('Ctrl Pts',(-43.1462045688855,0.424475570505401,
-11.6708316967806));
#30914=CARTESIAN_POINT('Ctrl Pts',(-43.1516654022893,0.43559362531917,-11.7951174044754));
#30915=CARTESIAN_POINT('Ctrl Pts',(-43.1648351192485,0.459330218746731,
-12.0539176614948));
#30916=CARTESIAN_POINT('Ctrl Pts',(-43.1935325849912,0.502791872139162,
-12.5042798495235));
#30917=CARTESIAN_POINT('Ctrl Pts',(-43.2918349048567,0.629156086175763,
-13.6778160448311));
#30918=CARTESIAN_POINT('Ctrl Pts',(-43.4467642620028,0.841231802133456,
-15.019464871798));
#30919=CARTESIAN_POINT('Ctrl Pts',(-43.5583459167546,1.17536390238127,-16.3968425054621));
#30920=CARTESIAN_POINT('Ctrl Pts',(-43.5968156257216,1.37364721670612,-17.0927150275281));
#30921=CARTESIAN_POINT('Ctrl Pts',(-43.6139523508331,1.55240857647083,-17.6538909094906));
#30922=CARTESIAN_POINT('Ctrl Pts',(-43.6175451144521,1.6485074056122,-17.9356670485181));
#30923=CARTESIAN_POINT('Ctrl Pts',(-43.6181302561629,1.72310984528553,-18.1473356018224));
#30924=CARTESIAN_POINT('Ctrl Pts',(-43.615423729367,1.78144840511499,-18.3099380413222));
#30925=CARTESIAN_POINT('Ctrl Pts',(-43.6102834716429,1.90052337855645,-18.6147533670115));
#30926=CARTESIAN_POINT('Ctrl Pts',(-43.6028756356143,2.02979449666717,-18.916104536019));
#30927=CARTESIAN_POINT('Ctrl Pts',(-43.5946265935477,2.16472139261033,-19.2068666513642));
#30928=CARTESIAN_POINT('Ctrl Pts',(-43.5890067356035,2.25154884571202,-19.3861828601404));
#30929=CARTESIAN_POINT('Ctrl Pts',(-43.5843537026808,2.32209811486412,-19.5276752804076));
#30930=CARTESIAN_POINT('Ctrl Pts',(-43.5795884739498,2.39336597516418,-19.6681250028613));
#30931=CARTESIAN_POINT('Ctrl Pts',(-43.566082556781,2.59196363352519,-20.0498673569958));
#30932=CARTESIAN_POINT('Ctrl Pts',(-43.5426641158337,2.92794406976125,-20.6519833438532));
#30933=CARTESIAN_POINT('Ctrl Pts',(-43.502946975925,3.52412707502357,-21.6678184692176));
#30934=CARTESIAN_POINT('Ctrl Pts',(-43.4668549917711,4.21026357501831,-22.8465894487001));
#30935=CARTESIAN_POINT('Ctrl Pts',(-43.4611694703721,4.57462701073374,-23.6690582823401));
#30936=CARTESIAN_POINT('Ctrl Pts',(-43.4553982014206,4.71697932248017,-24.1238951932113));
#30937=CARTESIAN_POINT('Ctrl Pts',(-43.4462062290868,4.77898111591247,-24.343408087553));
#30938=CARTESIAN_POINT('Ctrl Pts',(-43.4250726566578,4.88081822070273,-24.7665431378758));
#30939=CARTESIAN_POINT('Ctrl Pts',(-43.37239277437,5.02244505804989,-25.5330343096657));
#30940=CARTESIAN_POINT('Ctrl Pts',(-43.2645514756731,5.13286377920033,-26.6650074898123));
#30941=CARTESIAN_POINT('Ctrl Pts',(-43.1112830283311,5.19738964776005,-28.1015600780752));
#30942=CARTESIAN_POINT('Ctrl Pts',(-43.0184092334532,5.23942265301599,-29.1106062811467));
#30943=CARTESIAN_POINT('Ctrl Pts',(-42.9752707928305,5.27425180200197,-29.6911654008103));
#30944=CARTESIAN_POINT('Ctrl Pts',(-42.966080271284,5.28009112339822,-29.8027089865303));
#30945=CARTESIAN_POINT('Ctrl Pts',(-42.9476684412197,5.29118639926699,-30.0366412065176));
#30946=CARTESIAN_POINT('Ctrl Pts',(-42.9160330273132,5.30655790883432,-30.443405350357));
#30947=CARTESIAN_POINT('Ctrl Pts',(-42.8548567708032,5.32453906176737,-31.2704688469183));
#30948=CARTESIAN_POINT('Ctrl Pts',(-42.7908746025857,5.32108460865568,-32.2357156564981));
#30949=CARTESIAN_POINT('Ctrl Pts',(-42.7334017987881,5.30747776413526,-33.2239132019661));
#30950=CARTESIAN_POINT('Ctrl Pts',(-42.6934997484444,5.29594667190586,-33.9755180951015));
#30951=CARTESIAN_POINT('Ctrl Pts',(-42.656735262742,5.28708252845668,-34.7375742637586));
#30952=CARTESIAN_POINT('Ctrl Pts',(-42.6342288122971,5.285790467693,-35.2525723965959));
#30953=CARTESIAN_POINT('Ctrl Pts',(-42.6180198871815,5.28767511879397,-35.6420443252481));
#30954=CARTESIAN_POINT('Ctrl Pts',(-42.6075403525927,5.28879993451498,-35.889267876483));
#30955=CARTESIAN_POINT('Ctrl Pts',(-42.5880311795273,5.29088059660548,-36.3910999468938));
#30956=CARTESIAN_POINT('Ctrl Pts',(-42.5574740714464,5.29404486631059,-37.2645796050843));
#30957=CARTESIAN_POINT('Ctrl Pts',(-42.5084906513819,5.29882509433162,-39.0133321957582));
#30958=CARTESIAN_POINT('Ctrl Pts',(-42.4805858811114,5.30240885701596,-40.5146262302045));
#30959=CARTESIAN_POINT('Ctrl Pts',(-42.4597594875166,5.30695522943146,-41.6480970175863));
#30960=CARTESIAN_POINT('Ctrl Pts',(-42.4550925408997,5.30776155485162,-41.895606773929));
#30961=CARTESIAN_POINT('Ctrl Pts',(-42.4480332237712,5.30857619507488,-42.2692941279595));
#30962=CARTESIAN_POINT('Ctrl Pts',(-42.4410083438519,5.30906868577314,-42.6433511919673));
#30963=CARTESIAN_POINT('Ctrl Pts',(-42.4318302536459,5.30942931340334,-43.143491020825));
#30964=CARTESIAN_POINT('Ctrl Pts',(-42.4209580775566,5.30954744650048,-43.7704874992468));
#30965=CARTESIAN_POINT('Ctrl Pts',(-42.4096873604175,5.30990040654643,-44.5255677386172));
#30966=CARTESIAN_POINT('Ctrl Pts',(-42.4024519124516,5.31099253303746,-45.156538694259));
#30967=CARTESIAN_POINT('Ctrl Pts',(-42.3983446705665,5.31272170388111,-45.6621639986098));
#30968=CARTESIAN_POINT('Ctrl Pts',(-42.3962160420237,5.31454333820731,-46.0417335671184));
#30969=CARTESIAN_POINT('Ctrl Pts',(-42.3951398730034,5.31698481800948,-46.4215727361831));
#30970=CARTESIAN_POINT('Ctrl Pts',(-42.3952426337664,5.32120622622578,-46.9283776251192));
#30971=CARTESIAN_POINT('Ctrl Pts',(-42.3972151547764,5.32558029912895,-47.3085737880552));
#30972=CARTESIAN_POINT('Ctrl Pts',(-42.4006589313626,5.33101012342549,-47.6901709112403));
#30973=CARTESIAN_POINT('Ctrl Pts',(-42.4034686953696,5.33625743612167,-47.9582779372634));
#30974=CARTESIAN_POINT('Ctrl Pts',(-42.4109197846148,5.35122933246416,-48.4817957617174));
#30975=CARTESIAN_POINT('Ctrl Pts',(-42.4284500089677,5.38698475992364,-49.3888319680093));
#30976=CARTESIAN_POINT('Ctrl Pts',(-42.4643923523527,5.45039872226269,-50.6443179207177));
#30977=CARTESIAN_POINT('Ctrl Pts',(-42.5189548253264,5.5040358902261,-52.0909303402843));
#30978=CARTESIAN_POINT('Ctrl Pts',(-42.5586526259613,5.49929556965035,-53.0127495907653));
#30979=CARTESIAN_POINT('Ctrl Pts',(-42.583009031644,5.47695283862441,-53.5757195163897));
#30980=CARTESIAN_POINT('Ctrl Pts',(-42.5934150689954,5.46535897339064,-53.7741421322066));
#30981=CARTESIAN_POINT('Ctrl Pts',(-42.6162874901187,5.42723297073372,-54.2046560451703));
#30982=CARTESIAN_POINT('Ctrl Pts',(-42.6608944871551,5.32608219999238,-54.988660204803));
#30983=CARTESIAN_POINT('Ctrl Pts',(-42.7601501828626,5.02862385309719,-56.7101234471156));
#30984=CARTESIAN_POINT('Ctrl Pts',(-42.8417295651558,4.77257551658811,-58.4251999633534));
#30985=CARTESIAN_POINT('Ctrl Pts',(-42.8686094143971,4.85145432001225,-59.7649620853934));
#30986=CARTESIAN_POINT('Ctrl Pts',(-42.8717657002582,4.86099496633503,-59.9072004863649));
#30987=CARTESIAN_POINT('Ctrl Pts',(-42.8773262490722,4.88469292687789,-60.2020612790792));
#30988=CARTESIAN_POINT('Ctrl Pts',(-42.8853093445454,4.93604879276198,-60.7095931176271));
#30989=CARTESIAN_POINT('Ctrl Pts',(-42.8949090270911,5.07731157743547,-61.7175466105396));
#30990=CARTESIAN_POINT('Ctrl Pts',(-42.8947467815965,5.31517540413371,-62.8393181260782));
#30991=CARTESIAN_POINT('Ctrl Pts',(-42.8900097131894,5.60915460119308,-63.932328552125));
#30992=CARTESIAN_POINT('Ctrl Pts',(-42.8867894283273,5.7920401895333,-64.5353932787128));
#30993=CARTESIAN_POINT('Ctrl Pts',(-42.8848858010747,5.91980672807307,-64.9325635567599));
#30994=CARTESIAN_POINT('Ctrl Pts',(-42.8837125739361,6.00644847706447,-65.1959859459554));
#30995=CARTESIAN_POINT('Ctrl Pts',(-42.882724377332,6.09517694280922,-65.4575020380078));
#30996=CARTESIAN_POINT('Ctrl Pts',(-42.8821069494855,6.17435955732801,-65.6844870530957));
#30997=CARTESIAN_POINT('Ctrl Pts',(-42.8818355425142,6.22001574696898,-65.8136725464171));
#30998=CARTESIAN_POINT('Ctrl Pts',(-42.8815148822881,6.28890287374054,-66.0069553415058));
#30999=CARTESIAN_POINT('Ctrl Pts',(-42.8814404622754,6.34707681703438,-66.1669031179569));
#31000=CARTESIAN_POINT('Ctrl Pts',(-42.8816188770637,6.44449486278725,-66.4309243422751));
#31001=CARTESIAN_POINT('Ctrl Pts',(-42.880851859429,6.56223130155641,-66.7356201814902));
#31002=CARTESIAN_POINT('Ctrl Pts',(-42.8796354188091,6.80477221912943,-67.3125008499134));
#31003=CARTESIAN_POINT('Ctrl Pts',(-42.8769453178782,7.26482353503976,-68.3011228654526));
#31004=CARTESIAN_POINT('Ctrl Pts',(-42.8717733301943,8.26679949765506,-70.1591795787803));
#31005=CARTESIAN_POINT('Ctrl Pts',(-42.870413129688,9.14210741751194,-71.6194843562164));
#31006=CARTESIAN_POINT('Ctrl Pts',(-42.8729356151749,9.69552819953706,-72.671723686886));
#31007=CARTESIAN_POINT('Ctrl Pts',(-42.8726762410367,9.83124532059666,-72.9294181564817));
#31008=CARTESIAN_POINT('Ctrl Pts',(-42.8726546748704,10.0960730243121,-73.4309906589323));
#31009=CARTESIAN_POINT('Ctrl Pts',(-42.8724705779236,10.4306758301375,-74.0627413153577));
#31010=CARTESIAN_POINT('Ctrl Pts',(-42.8724112796876,10.8313703210138,-74.8166367741079));
#31011=CARTESIAN_POINT('Ctrl Pts',(-42.8723200277616,11.6345193230121,-76.3242084294796));
#31012=CARTESIAN_POINT('Ctrl Pts',(-42.8724075953763,12.3039112027909,-77.576767132054));
#31013=CARTESIAN_POINT('Ctrl Pts',(-42.8725343781945,13.2718195563419,-79.3973298027057));
#31014=CARTESIAN_POINT('Ctrl Pts',(-42.8724765736113,13.7091763374169,-80.2199919219157));
#31015=CARTESIAN_POINT('Ctrl Pts',(-42.8724765736115,14.1456979248064,-81.0409696240142));
#31016=CARTESIAN_POINT('Ctrl Pts',(-40.9893941583173,0.280290173804462,
24.8306665397013));
#31017=CARTESIAN_POINT('Ctrl Pts',(-40.9895177486156,0.280296428295455,
24.7817882354976));
#31018=CARTESIAN_POINT('Ctrl Pts',(-40.989647367799,0.280302986842126,24.7329109790473));
#31019=CARTESIAN_POINT('Ctrl Pts',(-40.9911780305211,0.280380545189393,
24.1823155147162));
#31020=CARTESIAN_POINT('Ctrl Pts',(-40.9923510756847,0.280421693213243,
23.1782062681366));
#31021=CARTESIAN_POINT('Ctrl Pts',(-40.995081018544,0.280503669861664,21.1696270086331));
#31022=CARTESIAN_POINT('Ctrl Pts',(-41.0052679693907,0.281021736168168,
19.6654822805891));
#31023=CARTESIAN_POINT('Ctrl Pts',(-41.0268730592858,0.282211835134878,
18.4144323008035));
#31024=CARTESIAN_POINT('Ctrl Pts',(-41.0372378337411,0.28277635701125,17.9116777228209));
#31025=CARTESIAN_POINT('Ctrl Pts',(-41.0632709191315,0.284184273608307,
16.9077383763575));
#31026=CARTESIAN_POINT('Ctrl Pts',(-41.1191113931709,0.287209632289243,
15.1539432392821));
#31027=CARTESIAN_POINT('Ctrl Pts',(-41.1721280107876,0.290186683943603,
13.6520484506017));
#31028=CARTESIAN_POINT('Ctrl Pts',(-41.2052986276455,0.292230205805187,
12.397322192359));
#31029=CARTESIAN_POINT('Ctrl Pts',(-41.2188536880839,0.29308595464525,11.8962622431662));
#31030=CARTESIAN_POINT('Ctrl Pts',(-41.2464704555292,0.294896996873047,
10.8942718424413));
#31031=CARTESIAN_POINT('Ctrl Pts',(-41.2942284734365,0.298167507818841,
9.14059348098497));
#31032=CARTESIAN_POINT('Ctrl Pts',(-41.3276788341157,0.300601301858155,
7.63555392933036));
#31033=CARTESIAN_POINT('Ctrl Pts',(-41.3424956731047,0.301692855427609,
6.50481572178853));
#31034=CARTESIAN_POINT('Ctrl Pts',(-41.3455479496262,0.301926824087675,
6.25451208273883));
#31035=CARTESIAN_POINT('Ctrl Pts',(-41.3508061529118,0.302363239284339,
5.75333715203142));
#31036=CARTESIAN_POINT('Ctrl Pts',(-41.3579058294151,0.303039188454316,
4.87488423146479));
#31037=CARTESIAN_POINT('Ctrl Pts',(-41.3646446561493,0.303994073880602,
3.11477538310501));
#31038=CARTESIAN_POINT('Ctrl Pts',(-41.3609067466047,0.30398518686012,1.60893149366535));
#31039=CARTESIAN_POINT('Ctrl Pts',(-41.3568515310369,0.303452938888166,
0.550184452068615));
#31040=CARTESIAN_POINT('Ctrl Pts',(-41.3563184779633,0.303382434888984,
0.424092420441241));
#31041=CARTESIAN_POINT('Ctrl Pts',(-41.3550634218872,0.303215802556436,
0.172099832926385));
#31042=CARTESIAN_POINT('Ctrl Pts',(-41.3523931530852,0.302859818499856,
-0.268408450246914));
#31043=CARTESIAN_POINT('Ctrl Pts',(-41.3473577456846,0.30218733918811,-0.896407546601593));
#31044=CARTESIAN_POINT('Ctrl Pts',(-41.3397754482278,0.301179512381092,
-1.64862299843257));
#31045=CARTESIAN_POINT('Ctrl Pts',(-41.3281793044161,0.299652753592981,
-2.65005274693771));
#31046=CARTESIAN_POINT('Ctrl Pts',(-41.3119317130866,0.297544977724727,
-3.90045626766242));
#31047=CARTESIAN_POINT('Ctrl Pts',(-41.2993328034355,0.296007850935482,
-4.90158738099382));
#31048=CARTESIAN_POINT('Ctrl Pts',(-41.2922774157016,0.295203263328682,
-5.52814145730737));
#31049=CARTESIAN_POINT('Ctrl Pts',(-41.2888114147919,0.294151273016196,
-5.76976978184256));
#31050=CARTESIAN_POINT('Ctrl Pts',(-41.2797870177376,0.289634238603212,
-6.26180555436338));
#31051=CARTESIAN_POINT('Ctrl Pts',(-41.2597421505567,0.27681258848934,-7.12814873920402));
#31052=CARTESIAN_POINT('Ctrl Pts',(-41.2260511487051,0.252733800345328,
-8.38969650658993));
#31053=CARTESIAN_POINT('Ctrl Pts',(-41.2044973404892,0.24345916428999,-9.67758707980947));
#31054=CARTESIAN_POINT('Ctrl Pts',(-41.2056903628757,0.257265492438425,
-10.5928358962625));
#31055=CARTESIAN_POINT('Ctrl Pts',(-41.2124295969221,0.272938590382539,
-11.1192946726198));
#31056=CARTESIAN_POINT('Ctrl Pts',(-41.2180486738718,0.283730411189719,
-11.3838864658141));
#31057=CARTESIAN_POINT('Ctrl Pts',(-41.2232136440982,0.2930859116899,-11.5831004907457));
#31058=CARTESIAN_POINT('Ctrl Pts',(-41.2270561501629,0.298405308527004,
-11.7004395131457));
#31059=CARTESIAN_POINT('Ctrl Pts',(-41.2359452524065,0.308839615257286,
-11.946106685933));
#31060=CARTESIAN_POINT('Ctrl Pts',(-41.2546055704108,0.325559075605228,
-12.3752463137554));
#31061=CARTESIAN_POINT('Ctrl Pts',(-41.3164265455899,0.366930410177482,
-13.5036868298348));
#31062=CARTESIAN_POINT('Ctrl Pts',(-41.4165120412304,0.432307031414684,
-14.8218483401688));
#31063=CARTESIAN_POINT('Ctrl Pts',(-41.5127262532785,0.611950064184939,
-16.2117418031106));
#31064=CARTESIAN_POINT('Ctrl Pts',(-41.5561223426356,0.739176733282308,
-16.9227777590329));
#31065=CARTESIAN_POINT('Ctrl Pts',(-41.5858614479214,0.867942626871003,
-17.5004660887901));
#31066=CARTESIAN_POINT('Ctrl Pts',(-41.5986983768322,0.94206072424014,-17.7917806119061));
#31067=CARTESIAN_POINT('Ctrl Pts',(-41.6073703760708,1.00139682202911,-18.0106350515628));
#31068=CARTESIAN_POINT('Ctrl Pts',(-41.6123650780398,1.04574782279505,-18.1684664922214));
#31069=CARTESIAN_POINT('Ctrl Pts',(-41.6233648741053,1.13917584297077,-18.4708250805361));
#31070=CARTESIAN_POINT('Ctrl Pts',(-41.634803967744,1.24230920609741,-18.7691933000577));
#31071=CARTESIAN_POINT('Ctrl Pts',(-41.6467674858292,1.35219820309014,-19.0591948969288));
#31072=CARTESIAN_POINT('Ctrl Pts',(-41.6543663333302,1.42359984545195,-19.2381423937385));
#31073=CARTESIAN_POINT('Ctrl Pts',(-41.6605197218763,1.4820643382338,-19.3796077886087));
#31074=CARTESIAN_POINT('Ctrl Pts',(-41.6667092573891,1.54138879073417,-19.5200999449311));
#31075=CARTESIAN_POINT('Ctrl Pts',(-41.6838703240796,1.70782961601363,-19.9023775192806));
#31076=CARTESIAN_POINT('Ctrl Pts',(-41.7124555728774,1.99507960498138,-20.5066336265271));
#31077=CARTESIAN_POINT('Ctrl Pts',(-41.762410749083,2.51980468748958,-21.5288699023996));
#31078=CARTESIAN_POINT('Ctrl Pts',(-41.819893857012,3.15292972952515,-22.7211160695818));
#31079=CARTESIAN_POINT('Ctrl Pts',(-41.848746085566,3.53754515746703,-23.5902702058667));
#31080=CARTESIAN_POINT('Ctrl Pts',(-41.8531760227506,3.70920242886249,-24.1019496614625));
#31081=CARTESIAN_POINT('Ctrl Pts',(-41.8475597634427,3.78250620861328,-24.3425402779051));
#31082=CARTESIAN_POINT('Ctrl Pts',(-41.8332475454277,3.91348902157027,-24.805984915587));
#31083=CARTESIAN_POINT('Ctrl Pts',(-41.7917422112982,4.11801901399799,-25.6355828824697));
#31084=CARTESIAN_POINT('Ctrl Pts',(-41.6981795389215,4.34113924375327,-26.8317148586573));
#31085=CARTESIAN_POINT('Ctrl Pts',(-41.5528775003771,4.53997149540172,-28.2866430086673));
#31086=CARTESIAN_POINT('Ctrl Pts',(-41.458479131446,4.65222796034505,-29.2631070048381));
#31087=CARTESIAN_POINT('Ctrl Pts',(-41.4151931262802,4.71539802949842,-29.8137442335345));
#31088=CARTESIAN_POINT('Ctrl Pts',(-41.4060298351662,4.72790458771569,-29.9284510055469));
#31089=CARTESIAN_POINT('Ctrl Pts',(-41.3871249451852,4.75189565799189,-30.1629293166748));
#31090=CARTESIAN_POINT('Ctrl Pts',(-41.3535090630033,4.78947966529287,-30.572866073278));
#31091=CARTESIAN_POINT('Ctrl Pts',(-41.2839763646377,4.85023216494433,-31.401771891854));
#31092=CARTESIAN_POINT('Ctrl Pts',(-41.2021060952701,4.89366453810222,-32.3653918006517));
#31093=CARTESIAN_POINT('Ctrl Pts',(-41.1226823950886,4.92648406614013,-33.3475001279598));
#31094=CARTESIAN_POINT('Ctrl Pts',(-41.0655540894473,4.9494840992214,-34.0930378769679));
#31095=CARTESIAN_POINT('Ctrl Pts',(-41.011989975364,4.97464424292071,-34.8476229623568));
#31096=CARTESIAN_POINT('Ctrl Pts',(-40.9793866125484,4.99541429903991,-35.3568061789837));
#31097=CARTESIAN_POINT('Ctrl Pts',(-40.9562950743291,5.013520002653,-35.7416216108422));
#31098=CARTESIAN_POINT('Ctrl Pts',(-40.9413580508551,5.02474703743586,-35.9871460126007));
#31099=CARTESIAN_POINT('Ctrl Pts',(-40.9129411234468,5.04703973134136,-36.4848114727042));
#31100=CARTESIAN_POINT('Ctrl Pts',(-40.8670672335441,5.0841199248743,-37.3515626087591));
#31101=CARTESIAN_POINT('Ctrl Pts',(-40.7887382032561,5.15284178929198,-39.0869347384886));
#31102=CARTESIAN_POINT('Ctrl Pts',(-40.7383890275233,5.20209094587151,-40.5776698659022));
#31103=CARTESIAN_POINT('Ctrl Pts',(-40.7026003827779,5.23629387418686,-41.7033590423549));
#31104=CARTESIAN_POINT('Ctrl Pts',(-40.6947447559412,5.24353641556213,-41.9494496889739));
#31105=CARTESIAN_POINT('Ctrl Pts',(-40.6831450578572,5.25366097348401,-42.3207558307205));
#31106=CARTESIAN_POINT('Ctrl Pts',(-40.6718150888099,5.26309548536225,-42.692400344777));
#31107=CARTESIAN_POINT('Ctrl Pts',(-40.6571661791622,5.27485319002791,-43.1891777061944));
#31108=CARTESIAN_POINT('Ctrl Pts',(-40.6399177519583,5.2881969783719,-43.8117785949811));
#31109=CARTESIAN_POINT('Ctrl Pts',(-40.6215360973513,5.30262611370692,-44.5612594341765));
#31110=CARTESIAN_POINT('Ctrl Pts',(-40.6086618487947,5.31381997478719,-45.1873091829714));
#31111=CARTESIAN_POINT('Ctrl Pts',(-40.6001715928118,5.32264137343099,-45.6888585175579));
#31112=CARTESIAN_POINT('Ctrl Pts',(-40.594768069357,5.32923855463232,-46.0652951836812));
#31113=CARTESIAN_POINT('Ctrl Pts',(-40.5904073885478,5.33589999628747,-46.4419280754876));
#31114=CARTESIAN_POINT('Ctrl Pts',(-40.5860983180208,5.34497333867694,-46.9443661359885));
#31115=CARTESIAN_POINT('Ctrl Pts',(-40.5846293700653,5.35210128769182,-47.3211687659398));
#31116=CARTESIAN_POINT('Ctrl Pts',(-40.5845324546587,5.35963258663933,-47.6992852599114));
#31117=CARTESIAN_POINT('Ctrl Pts',(-40.5849097349468,5.36600268597118,-47.9641074827081));
#31118=CARTESIAN_POINT('Ctrl Pts',(-40.5873494265197,5.38199177152275,-48.4821214154056));
#31119=CARTESIAN_POINT('Ctrl Pts',(-40.5957227204869,5.41657899625576,-49.3804111342591));
#31120=CARTESIAN_POINT('Ctrl Pts',(-40.6178354563581,5.47168116794954,-50.6268280187354));
#31121=CARTESIAN_POINT('Ctrl Pts',(-40.6556343690552,5.50866564955266,-52.0671976655524));
#31122=CARTESIAN_POINT('Ctrl Pts',(-40.6853664855489,5.4917947350123,-52.9879942074645));
#31123=CARTESIAN_POINT('Ctrl Pts',(-40.7044696227113,5.46214712496547,-53.5512304200892));
#31124=CARTESIAN_POINT('Ctrl Pts',(-40.7128455580891,5.44787630494579,-53.7456026395922));
#31125=CARTESIAN_POINT('Ctrl Pts',(-40.7318083464858,5.40309378786118,-54.171519977409));
#31126=CARTESIAN_POINT('Ctrl Pts',(-40.7701270093372,5.28776865106253,-54.948811372113));
#31127=CARTESIAN_POINT('Ctrl Pts',(-40.8593317204784,4.95330030990605,-56.6664624097345));
#31128=CARTESIAN_POINT('Ctrl Pts',(-40.9364947249792,4.65832218134193,-58.3911740051108));
#31129=CARTESIAN_POINT('Ctrl Pts',(-40.9617903823933,4.72638396747244,-59.7488048668769));
#31130=CARTESIAN_POINT('Ctrl Pts',(-40.9647461461571,4.73485155802129,-59.8925661466653));
#31131=CARTESIAN_POINT('Ctrl Pts',(-40.9700258512831,4.75671650338397,-60.1906469541753));
#31132=CARTESIAN_POINT('Ctrl Pts',(-40.9777600062064,4.80587520115248,-60.7031893893145));
#31133=CARTESIAN_POINT('Ctrl Pts',(-40.987752912195,4.94604258228551,-61.7194421890793));
#31134=CARTESIAN_POINT('Ctrl Pts',(-40.9895154351334,5.18793826020981,-62.8463958974618));
#31135=CARTESIAN_POINT('Ctrl Pts',(-40.9871730813637,5.48701942402319,-63.940890731633));
#31136=CARTESIAN_POINT('Ctrl Pts',(-40.9852848038056,5.67251371052068,-64.5434949804964));
#31137=CARTESIAN_POINT('Ctrl Pts',(-40.9841884694266,5.80164006935051,-64.9398526733912));
#31138=CARTESIAN_POINT('Ctrl Pts',(-40.9835271184745,5.8890677405049,-65.2025993618358));
#31139=CARTESIAN_POINT('Ctrl Pts',(-40.9830027941993,5.97838745269654,-65.4632441843856));
#31140=CARTESIAN_POINT('Ctrl Pts',(-40.9827382954141,6.05786032431043,-65.6892951122439));
#31141=CARTESIAN_POINT('Ctrl Pts',(-40.9826514989447,6.10361269246761,-65.8178979997058));
#31142=CARTESIAN_POINT('Ctrl Pts',(-40.9825900249628,6.17257138556137,-66.0102599184474));
#31143=CARTESIAN_POINT('Ctrl Pts',(-40.9826914604614,6.23064889175667,-66.1693354930749));
#31144=CARTESIAN_POINT('Ctrl Pts',(-40.9831030283092,6.32767483575051,-66.4318170111501));
#31145=CARTESIAN_POINT('Ctrl Pts',(-40.9826595018947,6.44574019605698,-66.7368488770948));
#31146=CARTESIAN_POINT('Ctrl Pts',(-40.9819573406223,6.68846187245255,-67.3133359663928));
#31147=CARTESIAN_POINT('Ctrl Pts',(-40.9799958154659,7.14893613993861,-68.3018775822024));
#31148=CARTESIAN_POINT('Ctrl Pts',(-40.9755278485363,8.15121009323467,-70.1595076830405));
#31149=CARTESIAN_POINT('Ctrl Pts',(-40.973771100275,9.02663496104393,-71.619963856248));
#31150=CARTESIAN_POINT('Ctrl Pts',(-40.9759105947828,9.58019735042475,-72.6723092429353));
#31151=CARTESIAN_POINT('Ctrl Pts',(-40.975697760016,9.71592560132571,-72.9299653026806));
#31152=CARTESIAN_POINT('Ctrl Pts',(-40.9756869923594,9.9807728149155,-73.4315008472055));
#31153=CARTESIAN_POINT('Ctrl Pts',(-40.9755363779319,10.3153830864914,-74.0632051376608));
#31154=CARTESIAN_POINT('Ctrl Pts',(-40.9754873852925,10.7160627683641,-74.8170628142835));
#31155=CARTESIAN_POINT('Ctrl Pts',(-40.975405045408,11.5191559679699,-76.3245831081049));
#31156=CARTESIAN_POINT('Ctrl Pts',(-40.9754603446411,12.1885044744805,-77.577180313731));
#31157=CARTESIAN_POINT('Ctrl Pts',(-40.9755617664425,13.1564671972782,-79.3978378813868));
#31158=CARTESIAN_POINT('Ctrl Pts',(-40.9755123070535,13.5938177436188,-80.2204798316628));
#31159=CARTESIAN_POINT('Ctrl Pts',(-40.9755123070534,14.0303393310083,-81.0414575337613));
#31160=CARTESIAN_POINT('Ctrl Pts',(-39.0888001402497,0.180014935889884,
24.830657879308));
#31161=CARTESIAN_POINT('Ctrl Pts',(-39.088917316815,0.180019720217799,24.7817793004034));
#31162=CARTESIAN_POINT('Ctrl Pts',(-39.0890402101583,0.180024736696177,
24.7329017756012));
#31163=CARTESIAN_POINT('Ctrl Pts',(-39.0904914691558,0.1800840769936,24.1823027164344));
#31164=CARTESIAN_POINT('Ctrl Pts',(-39.0915869337663,0.180115913204324,
23.1781842967628));
#31165=CARTESIAN_POINT('Ctrl Pts',(-39.0941254999962,0.180179361754887,
21.1695999880857));
#31166=CARTESIAN_POINT('Ctrl Pts',(-39.1037841631934,0.180575900260667,
19.6654506338937));
#31167=CARTESIAN_POINT('Ctrl Pts',(-39.1243530113637,0.181485107226502,
18.4144014643961));
#31168=CARTESIAN_POINT('Ctrl Pts',(-39.1342130895912,0.181914718605493,
17.9116384563228));
#31169=CARTESIAN_POINT('Ctrl Pts',(-39.1589647024343,0.182983006233729,
16.9076901036643));
#31170=CARTESIAN_POINT('Ctrl Pts',(-39.2120609298036,0.185277316979706,
15.1538859030914));
#31171=CARTESIAN_POINT('Ctrl Pts',(-39.2625778615799,0.187551451732393,
13.6519981771989));
#31172=CARTESIAN_POINT('Ctrl Pts',(-39.2943891236822,0.189143259235937,
12.3973026245927));
#31173=CARTESIAN_POINT('Ctrl Pts',(-39.3074124097061,0.189812747891297,
11.8962578221136));
#31174=CARTESIAN_POINT('Ctrl Pts',(-39.3340182664446,0.191239244045362,
10.8942890475992));
#31175=CARTESIAN_POINT('Ctrl Pts',(-39.3801811561126,0.193834769361145,
9.14063943512921));
#31176=CARTESIAN_POINT('Ctrl Pts',(-39.4126589643153,0.195790079789512,
7.63554879952261));
#31177=CARTESIAN_POINT('Ctrl Pts',(-39.4270732637367,0.196673507474238,
6.50476253261587));
#31178=CARTESIAN_POINT('Ctrl Pts',(-39.4300591616367,0.196865202842096,
6.25445276686468));
#31179=CARTESIAN_POINT('Ctrl Pts',(-39.435258941596,0.197232346757206,5.75326596535956));
#31180=CARTESIAN_POINT('Ctrl Pts',(-39.4424218889848,0.197824694995779,
4.87478350553763));
#31181=CARTESIAN_POINT('Ctrl Pts',(-39.4497283637274,0.198728008388997,
3.11464478187555));
#31182=CARTESIAN_POINT('Ctrl Pts',(-39.4464205151028,0.198795280639079,
1.60867012703468));
#31183=CARTESIAN_POINT('Ctrl Pts',(-39.4418897974239,0.198252367947847,
0.549909941536338));
#31184=CARTESIAN_POINT('Ctrl Pts',(-39.4412945938795,0.19817944770704,0.423835971767908));
#31185=CARTESIAN_POINT('Ctrl Pts',(-39.4398911800345,0.198005968854597,
0.171865376680441));
#31186=CARTESIAN_POINT('Ctrl Pts',(-39.4369038750975,0.197632386715154,
-0.268604612588512));
#31187=CARTESIAN_POINT('Ctrl Pts',(-39.4312715773556,0.196928009174792,
-0.896605488280534));
#31188=CARTESIAN_POINT('Ctrl Pts',(-39.4228297437873,0.195872319618578,
-1.64880469502484));
#31189=CARTESIAN_POINT('Ctrl Pts',(-39.4099859739263,0.194306211522286,
-2.65032787018934));
#31190=CARTESIAN_POINT('Ctrl Pts',(-39.3922032627337,0.19221850645099,-3.90095990403691));
#31191=CARTESIAN_POINT('Ctrl Pts',(-39.378747393108,0.190844849193783,-4.90238820218311));
#31192=CARTESIAN_POINT('Ctrl Pts',(-39.3714091220386,0.190178367126032,
-5.52939258666469));
#31193=CARTESIAN_POINT('Ctrl Pts',(-39.3680546353478,0.18966453923232,-5.77732002007598));
#31194=CARTESIAN_POINT('Ctrl Pts',(-39.3599802837624,0.187845064398476,
-6.27624133314443));
#31195=CARTESIAN_POINT('Ctrl Pts',(-39.3430898444979,0.183072961379129,
-7.15137827865571));
#31196=CARTESIAN_POINT('Ctrl Pts',(-39.3157200332037,0.174613443335135,
-8.40956553707685));
#31197=CARTESIAN_POINT('Ctrl Pts',(-39.2965427974573,0.171291036054527,
-9.67486480366862));
#31198=CARTESIAN_POINT('Ctrl Pts',(-39.2939925399169,0.175456322303922,
-10.5634021553277));
#31199=CARTESIAN_POINT('Ctrl Pts',(-39.2965820046209,0.180257888939277,
-11.0715965941404));
#31200=CARTESIAN_POINT('Ctrl Pts',(-39.2993797017071,0.183568770539792,
-11.3259916623919));
#31201=CARTESIAN_POINT('Ctrl Pts',(-39.3021139832257,0.18643660005113,-11.5172312282543));
#31202=CARTESIAN_POINT('Ctrl Pts',(-39.3040028599904,0.18784577223247,-11.6321372911683));
#31203=CARTESIAN_POINT('Ctrl Pts',(-39.3079866743959,0.189457764488112,
-11.8713533836034));
#31204=CARTESIAN_POINT('Ctrl Pts',(-39.315572292305,0.189102148698272,-12.290150002075));
#31205=CARTESIAN_POINT('Ctrl Pts',(-39.3387249841932,0.176966665062875,
-13.3922597388429));
#31206=CARTESIAN_POINT('Ctrl Pts',(-39.3793104509326,0.152177319720917,
-14.684616780296));
#31207=CARTESIAN_POINT('Ctrl Pts',(-39.4444008963079,0.21143366494283,-16.0553046278289));
#31208=CARTESIAN_POINT('Ctrl Pts',(-39.4833859783724,0.272345394836458,
-16.7594975111963));
#31209=CARTESIAN_POINT('Ctrl Pts',(-39.5185388384933,0.345561837178436,
-17.3338623275751));
#31210=CARTESIAN_POINT('Ctrl Pts',(-39.5373323495522,0.391465068195811,
-17.6244284353275));
#31211=CARTESIAN_POINT('Ctrl Pts',(-39.5518079010771,0.429580386052769,
-17.8427249662891));
#31212=CARTESIAN_POINT('Ctrl Pts',(-39.5620866349126,0.456154357016654,
-17.9895464754391));
#31213=CARTESIAN_POINT('Ctrl Pts',(-39.5848759972109,0.514268268353239,
-18.2788335636466));
#31214=CARTESIAN_POINT('Ctrl Pts',(-39.6107202132686,0.579518601695886,
-18.5650135488669));
#31215=CARTESIAN_POINT('Ctrl Pts',(-39.6389605015963,0.651049904192671,
-18.8469815608269));
#31216=CARTESIAN_POINT('Ctrl Pts',(-39.6574562047748,0.698220492300876,
-19.0217040811562));
#31217=CARTESIAN_POINT('Ctrl Pts',(-39.6726828915373,0.737326663489326,
-19.1604954431962));
#31218=CARTESIAN_POINT('Ctrl Pts',(-39.6881655249372,0.77731466885754,-19.2986584821118));
#31219=CARTESIAN_POINT('Ctrl Pts',(-39.7316739135483,0.890776531212825,
-19.6760510166773));
#31220=CARTESIAN_POINT('Ctrl Pts',(-39.8066717585052,1.09398254141055,-20.279461655595));
#31221=CARTESIAN_POINT('Ctrl Pts',(-39.938277838171,1.48656520365138,-21.3150620832206));
#31222=CARTESIAN_POINT('Ctrl Pts',(-40.077341632778,2.00010489798032,-22.5472072770752));
#31223=CARTESIAN_POINT('Ctrl Pts',(-40.1321456942686,2.35388577460762,-23.4873219699195));
#31224=CARTESIAN_POINT('Ctrl Pts',(-40.1423069080736,2.53192731380775,-24.0633993869248));
#31225=CARTESIAN_POINT('Ctrl Pts',(-40.1399193224519,2.60832765495067,-24.3236021119375));
#31226=CARTESIAN_POINT('Ctrl Pts',(-40.1306249350369,2.75420279393139,-24.8247767992029));
#31227=CARTESIAN_POINT('Ctrl Pts',(-40.0971915732182,3.00295949420497,-25.7086237547162));
#31228=CARTESIAN_POINT('Ctrl Pts',(-40.0175805133852,3.3317714798528,-26.9556647229161));
#31229=CARTESIAN_POINT('Ctrl Pts',(-39.9025787170737,3.67809396319729,-28.4272529350418));
#31230=CARTESIAN_POINT('Ctrl Pts',(-39.8342238291159,3.86827373793614,-29.3797360671715));
#31231=CARTESIAN_POINT('Ctrl Pts',(-39.8047440456974,3.96216351133329,-29.9060423092907));
#31232=CARTESIAN_POINT('Ctrl Pts',(-39.7980205429724,3.98281121426406,-30.0247942372537));
#31233=CARTESIAN_POINT('Ctrl Pts',(-39.7842215053032,4.02234921237497,-30.2618607419045));
#31234=CARTESIAN_POINT('Ctrl Pts',(-39.759065878212,4.08747327702048,-30.6785565729723));
#31235=CARTESIAN_POINT('Ctrl Pts',(-39.7053748797711,4.20257737944751,-31.5169004102997));
#31236=CARTESIAN_POINT('Ctrl Pts',(-39.6384024007534,4.30612538685423,-32.4870338490126));
#31237=CARTESIAN_POINT('Ctrl Pts',(-39.5709404467581,4.39498269524525,-33.4687208426889));
#31238=CARTESIAN_POINT('Ctrl Pts',(-39.5215021532756,4.45768407502833,-34.2108591571771));
#31239=CARTESIAN_POINT('Ctrl Pts',(-39.4745696175246,4.51979157863402,-34.9587372020336));
#31240=CARTESIAN_POINT('Ctrl Pts',(-39.445985531223,4.56308844149943,-35.4612789463547));
#31241=CARTESIAN_POINT('Ctrl Pts',(-39.4259196026876,4.59716788322673,-35.8403775332147));
#31242=CARTESIAN_POINT('Ctrl Pts',(-39.4131817355006,4.61873093705687,-36.0854247647449));
#31243=CARTESIAN_POINT('Ctrl Pts',(-39.3886213104214,4.66107995131486,-36.5801668389091));
#31244=CARTESIAN_POINT('Ctrl Pts',(-39.3484506852508,4.73169399829863,-37.4426539206428));
#31245=CARTESIAN_POINT('Ctrl Pts',(-39.2770325138226,4.86037280466502,-39.1682155632337));
#31246=CARTESIAN_POINT('Ctrl Pts',(-39.2250551732578,4.9518917528671,-40.6505718461251));
#31247=CARTESIAN_POINT('Ctrl Pts',(-39.1846961695626,5.01278499443786,-41.7696323310482));
#31248=CARTESIAN_POINT('Ctrl Pts',(-39.1759032210977,5.02560217778097,-42.0139439899814));
#31249=CARTESIAN_POINT('Ctrl Pts',(-39.1629861359318,5.04379504566374,-42.3827593007497));
#31250=CARTESIAN_POINT('Ctrl Pts',(-39.1503600309008,5.06089925268883,-42.751882115462));
#31251=CARTESIAN_POINT('Ctrl Pts',(-39.1339231628734,5.08244887061201,-43.2453711960376));
#31252=CARTESIAN_POINT('Ctrl Pts',(-39.1141180502777,5.10720146264421,-43.8639216187556));
#31253=CARTESIAN_POINT('Ctrl Pts',(-39.0915763560939,5.13419137727256,-44.6086927863444));
#31254=CARTESIAN_POINT('Ctrl Pts',(-39.0738339354335,5.15507688085906,-45.2309580981883));
#31255=CARTESIAN_POINT('Ctrl Pts',(-39.0601599988728,5.1711967266364,-45.7295050929459));
#31256=CARTESIAN_POINT('Ctrl Pts',(-39.0502199963603,5.18311514449177,-46.1037425988828));
#31257=CARTESIAN_POINT('Ctrl Pts',(-39.040590911943,5.19496343795989,-46.4782291876173));
#31258=CARTESIAN_POINT('Ctrl Pts',(-39.0281251283629,5.21082106856711,-46.9778584393184));
#31259=CARTESIAN_POINT('Ctrl Pts',(-39.0193494459446,5.22292443950463,-47.3527036794028));
#31260=CARTESIAN_POINT('Ctrl Pts',(-39.010785432795,5.23546148056151,-47.7288783242806));
#31261=CARTESIAN_POINT('Ctrl Pts',(-39.0049867958231,5.24532767241946,-47.99209865349));
#31262=CARTESIAN_POINT('Ctrl Pts',(-38.9935183667642,5.26803527005199,-48.5071264413013));
#31263=CARTESIAN_POINT('Ctrl Pts',(-38.9740978249696,5.31410466326364,-49.4002542868204));
#31264=CARTESIAN_POINT('Ctrl Pts',(-38.950268636064,5.38418388501746,-50.6397406224838));
#31265=CARTESIAN_POINT('Ctrl Pts',(-38.932566017396,5.43631146552384,-52.0727982524135));
#31266=CARTESIAN_POINT('Ctrl Pts',(-38.9304335441673,5.42536496789242,-52.989488255695));
#31267=CARTESIAN_POINT('Ctrl Pts',(-38.9325212625522,5.39799805998086,-53.5500667727227));
#31268=CARTESIAN_POINT('Ctrl Pts',(-38.9336400312047,5.38485977924212,-53.7411047660093));
#31269=CARTESIAN_POINT('Ctrl Pts',(-38.9381602028544,5.34123153060828,-54.162852555021));
#31270=CARTESIAN_POINT('Ctrl Pts',(-38.9511573760908,5.22510906383587,-54.9346379848697));
#31271=CARTESIAN_POINT('Ctrl Pts',(-38.99249631887,4.87818796877245,-56.6484569514821));
#31272=CARTESIAN_POINT('Ctrl Pts',(-39.0347434104756,4.56039247618866,-58.3763175489968));
#31273=CARTESIAN_POINT('Ctrl Pts',(-39.047584331385,4.62341883253982,-59.7441081601773));
#31274=CARTESIAN_POINT('Ctrl Pts',(-39.0491546243172,4.63134886187758,-59.888231420937));
#31275=CARTESIAN_POINT('Ctrl Pts',(-39.0521002138274,4.65230957090921,-60.1874606307571));
#31276=CARTESIAN_POINT('Ctrl Pts',(-39.0568531914575,4.70032857345361,-60.7016038103045));
#31277=CARTESIAN_POINT('Ctrl Pts',(-39.0648358030033,4.83977848561367,-61.7205854703363));
#31278=CARTESIAN_POINT('Ctrl Pts',(-39.0710371837721,5.08321114489323,-62.8490547844155));
#31279=CARTESIAN_POINT('Ctrl Pts',(-39.0752893734243,5.38430626057982,-63.9439118204513));
#31280=CARTESIAN_POINT('Ctrl Pts',(-39.0771678446726,5.57084391741088,-64.5463225625434));
#31281=CARTESIAN_POINT('Ctrl Pts',(-39.0782980372909,5.7005156786258,-64.9424025034742));
#31282=CARTESIAN_POINT('Ctrl Pts',(-39.0790260694853,5.78826738637908,-65.2049249557145));
#31283=CARTESIAN_POINT('Ctrl Pts',(-39.0797243904785,5.87782236693452,-65.4652869654959));
#31284=CARTESIAN_POINT('Ctrl Pts',(-39.0803275770349,5.9574276594848,-65.6910396260822));
#31285=CARTESIAN_POINT('Ctrl Pts',(-39.0806724498338,6.00323009922179,-65.8194573134073));
#31286=CARTESIAN_POINT('Ctrl Pts',(-39.0811905813148,6.07223862779016,-66.0115272311747));
#31287=CARTESIAN_POINT('Ctrl Pts',(-39.0816290864477,6.1302936813055,-66.1703283551057));
#31288=CARTESIAN_POINT('Ctrl Pts',(-39.0823627216747,6.22720787006558,-66.4323252988748));
#31289=CARTESIAN_POINT('Ctrl Pts',(-39.0823776143426,6.34540720480139,-66.7374778327143));
#31290=CARTESIAN_POINT('Ctrl Pts',(-39.0823957104839,6.58823809941028,-67.313857165032));
#31291=CARTESIAN_POINT('Ctrl Pts',(-39.0814717921701,7.04891545187278,-68.3024021835632));
#31292=CARTESIAN_POINT('Ctrl Pts',(-39.0780496028852,8.05141164755579,-70.1599254084202));
#31293=CARTESIAN_POINT('Ctrl Pts',(-39.0759953206185,8.92684028983922,-71.6204368595171));
#31294=CARTESIAN_POINT('Ctrl Pts',(-39.0778599491261,9.48038853571346,-72.6727773216162));
#31295=CARTESIAN_POINT('Ctrl Pts',(-39.0777132912002,9.61612625611812,-72.9304182491998));
#31296=CARTESIAN_POINT('Ctrl Pts',(-39.0777424553879,9.88098000736009,-73.4319337176093));
#31297=CARTESIAN_POINT('Ctrl Pts',(-39.0776485013891,10.2155871994595,-74.0636178095387));
#31298=CARTESIAN_POINT('Ctrl Pts',(-39.0776133302215,10.6162558456429,-74.8174574888145));
#31299=CARTESIAN_POINT('Ctrl Pts',(-39.0775181921913,11.4193149429609,-76.324955350321));
#31300=CARTESIAN_POINT('Ctrl Pts',(-39.0775016266082,12.0886088877304,-77.5775761907898));
#31301=CARTESIAN_POINT('Ctrl Pts',(-39.0775880817214,13.0565775367831,-79.3982814865315));
#31302=CARTESIAN_POINT('Ctrl Pts',(-39.0775513690795,13.4939157183239,-80.220915054068));
#31303=CARTESIAN_POINT('Ctrl Pts',(-39.0775513690794,13.9304373057134,-81.0418927561665));
#31304=CARTESIAN_POINT('Ctrl Pts',(-36.711201720155,0.0846755602148468,
24.8306211994035));
#31305=CARTESIAN_POINT('Ctrl Pts',(-36.7113120028643,0.0846793100877247,
24.781741457617));
#31306=CARTESIAN_POINT('Ctrl Pts',(-36.7114276655895,0.0846832415760904,
24.7328627565529));
#31307=CARTESIAN_POINT('Ctrl Pts',(-36.7127935402306,0.0847297050999628,
24.1822497869885));
#31308=CARTESIAN_POINT('Ctrl Pts',(-36.7138292815451,0.0847707447900342,
23.1781129164513));
#31309=CARTESIAN_POINT('Ctrl Pts',(-36.7162322116714,0.0848690308091877,
21.1695035269936));
#31310=CARTESIAN_POINT('Ctrl Pts',(-36.7253229946257,0.0851785210529226,
19.6653423171276));
#31311=CARTESIAN_POINT('Ctrl Pts',(-36.7446583985594,0.08580782489809,18.4142882582294));
#31312=CARTESIAN_POINT('Ctrl Pts',(-36.7539257158908,0.0861108837197817,
17.9114529545179));
#31313=CARTESIAN_POINT('Ctrl Pts',(-36.7771865730825,0.0868740440157173,
16.907452295697));
#31314=CARTESIAN_POINT('Ctrl Pts',(-36.8270801555423,0.0885088814981871,
15.1536537250934));
#31315=CARTESIAN_POINT('Ctrl Pts',(-36.8745592957761,0.0900397746859907,
13.6519842643687));
#31316=CARTESIAN_POINT('Ctrl Pts',(-36.9044697043829,0.0909569223699599,
12.3975856133512));
#31317=CARTESIAN_POINT('Ctrl Pts',(-36.9167133201501,0.0913268259956495,
11.8966636497452));
#31318=CARTESIAN_POINT('Ctrl Pts',(-36.9417262912308,0.0920656429738596,
10.8948714710037));
#31319=CARTESIAN_POINT('Ctrl Pts',(-36.9851279506764,0.0933122188435441,
9.1413912793788));
#31320=CARTESIAN_POINT('Ctrl Pts',(-37.0156998270508,0.094154200871692,
7.63616215370004));
#31321=CARTESIAN_POINT('Ctrl Pts',(-37.0293041574709,0.0945217035687127,
6.50517410116762));
#31322=CARTESIAN_POINT('Ctrl Pts',(-37.0321344090801,0.0945957446429915,
6.25497355792918));
#31323=CARTESIAN_POINT('Ctrl Pts',(-37.0371099539078,0.0947172428471553,
5.75388043569213));
#31324=CARTESIAN_POINT('Ctrl Pts',(-37.0440813507022,0.0948653916598738,
4.87550989883566));
#31325=CARTESIAN_POINT('Ctrl Pts',(-37.0515656864022,0.0949446315277831,
3.11521636198001));
#31326=CARTESIAN_POINT('Ctrl Pts',(-37.0486042606475,0.0947837520977546,
1.60843751337755));
#31327=CARTESIAN_POINT('Ctrl Pts',(-37.0436575257864,0.0946981767982494,
0.548825679997348));
#31328=CARTESIAN_POINT('Ctrl Pts',(-37.043006429047,0.0946869608203108,
0.42262179116806));
#31329=CARTESIAN_POINT('Ctrl Pts',(-37.0414718052386,0.0946612696963625,
0.170422155403115));
#31330=CARTESIAN_POINT('Ctrl Pts',(-37.0382061177981,0.0946079689969842,
-0.270422265079373));
#31331=CARTESIAN_POINT('Ctrl Pts',(-37.0320655020198,0.0945099200478035,
-0.898877882758254));
#31332=CARTESIAN_POINT('Ctrl Pts',(-37.0228968170096,0.0943654510376819,
-1.65141723036078));
#31333=CARTESIAN_POINT('Ctrl Pts',(-37.0090454046044,0.0941451688310354,
-2.65321592415316));
#31334=CARTESIAN_POINT('Ctrl Pts',(-36.9900886001485,0.0938334943865793,
-3.90374987560333));
#31335=CARTESIAN_POINT('Ctrl Pts',(-36.9762392465201,0.0935908348151571,
-4.90470775986227));
#31336=CARTESIAN_POINT('Ctrl Pts',(-36.9689346734598,0.0934561646239056,
-5.53141437390056));
#31337=CARTESIAN_POINT('Ctrl Pts',(-36.965885586203,0.0934560411160533,
-5.78303893549836));
#31338=CARTESIAN_POINT('Ctrl Pts',(-36.9593883633974,0.0936321220515418,
-6.28587838196509));
#31339=CARTESIAN_POINT('Ctrl Pts',(-36.9472326785285,0.0942940185030665,
-7.16602952983162));
#31340=CARTESIAN_POINT('Ctrl Pts',(-36.9291349809246,0.0956253346127282,
-8.42199169718575));
#31341=CARTESIAN_POINT('Ctrl Pts',(-36.9140717168774,0.0958606590365747,
-9.67372572928418));
#31342=CARTESIAN_POINT('Ctrl Pts',(-36.9072337971097,0.0946254783342841,
-10.5462632941664));
#31343=CARTESIAN_POINT('Ctrl Pts',(-36.9046865248374,0.0934036409850022,
-11.0435648660092));
#31344=CARTESIAN_POINT('Ctrl Pts',(-36.9039172100298,0.0926004122272295,
-11.2918236171607));
#31345=CARTESIAN_POINT('Ctrl Pts',(-36.9035454721218,0.091917758319367,
-11.4784129535007));
#31346=CARTESIAN_POINT('Ctrl Pts',(-36.903145201881,0.0912228891846152,
-11.5969669025978));
#31347=CARTESIAN_POINT('Ctrl Pts',(-36.90181679827,0.0887691377984597,-11.8388638582651));
#31348=CARTESIAN_POINT('Ctrl Pts',(-36.8982881049238,0.0819826877349684,
-12.2623898158901));
#31349=CARTESIAN_POINT('Ctrl Pts',(-36.8849363606277,0.0544659407479422,
-13.3650568718358));
#31350=CARTESIAN_POINT('Ctrl Pts',(-36.8684847756465,0.00874815982371367,
-14.627968204471));
#31351=CARTESIAN_POINT('Ctrl Pts',(-36.8839622816576,-0.00132236754599921,
-15.9394295488705));
#31352=CARTESIAN_POINT('Ctrl Pts',(-36.9025953000082,0.00750601117003104,
-16.6076385810686));
#31353=CARTESIAN_POINT('Ctrl Pts',(-36.925786968904,0.0259046380924417,
-17.1501533085901));
#31354=CARTESIAN_POINT('Ctrl Pts',(-36.9404471432345,0.0394895220043137,
-17.4241536500862));
#31355=CARTESIAN_POINT('Ctrl Pts',(-36.9526487163045,0.0514713443528451,
-17.6296084885903));
#31356=CARTESIAN_POINT('Ctrl Pts',(-36.9613582831,0.0590767589393235,-17.7579478738763));
#31357=CARTESIAN_POINT('Ctrl Pts',(-36.9811360664443,0.0758277090006206,
-18.0191008493755));
#31358=CARTESIAN_POINT('Ctrl Pts',(-37.0042522483177,0.0943242665168838,
-18.2787705289901));
#31359=CARTESIAN_POINT('Ctrl Pts',(-37.0302501055141,0.114900987587735,
-18.5394145596037));
#31360=CARTESIAN_POINT('Ctrl Pts',(-37.0476045005527,0.128621094582331,
-18.7021796534871));
#31361=CARTESIAN_POINT('Ctrl Pts',(-37.0620917261753,0.140142097953813,
-18.8324923503967));
#31362=CARTESIAN_POINT('Ctrl Pts',(-37.0769615753961,0.152028238022326,
-18.962802336705));
#31363=CARTESIAN_POINT('Ctrl Pts',(-37.1193491862782,0.186251732259979,
-19.3212842178248));
#31364=CARTESIAN_POINT('Ctrl Pts',(-37.1959492565623,0.250921168216482,
-19.9083037268163));
#31365=CARTESIAN_POINT('Ctrl Pts',(-37.3417692430452,0.391973810946715,
-20.953189482416));
#31366=CARTESIAN_POINT('Ctrl Pts',(-37.5201245015063,0.618043471751103,
-22.2608038425323));
#31367=CARTESIAN_POINT('Ctrl Pts',(-37.6147314284528,0.841427703283629,
-23.309409082731));
#31368=CARTESIAN_POINT('Ctrl Pts',(-37.6482532597087,0.988116899634828,
-23.9659064207315));
#31369=CARTESIAN_POINT('Ctrl Pts',(-37.6592078803129,1.05206229864543,-24.2450313789672));
#31370=CARTESIAN_POINT('Ctrl Pts',(-37.6763853789569,1.18703243134129,-24.7843844548707));
#31371=CARTESIAN_POINT('Ctrl Pts',(-37.6941213656748,1.44305036514919,-25.7168694041114));
#31372=CARTESIAN_POINT('Ctrl Pts',(-37.6942808345933,1.83715730036241,-26.9990587814339));
#31373=CARTESIAN_POINT('Ctrl Pts',(-37.6819068176747,2.28970554590047,-28.4722406036395));
#31374=CARTESIAN_POINT('Ctrl Pts',(-37.6788534272093,2.54049055463771,-29.4066814895956));
#31375=CARTESIAN_POINT('Ctrl Pts',(-37.6805320778864,2.65829402513679,-29.9180192372393));
#31376=CARTESIAN_POINT('Ctrl Pts',(-37.6798971142878,2.68560134538136,-30.040367654817));
#31377=CARTESIAN_POINT('Ctrl Pts',(-37.6787749519767,2.73822820054902,-30.2806011843286));
#31378=CARTESIAN_POINT('Ctrl Pts',(-37.6756535886323,2.82773000309687,-30.704499948019));
#31379=CARTESIAN_POINT('Ctrl Pts',(-37.6665461775974,2.99523119806346,-31.554291765181));
#31380=CARTESIAN_POINT('Ctrl Pts',(-37.6512941902261,3.1648836902586,-32.5343411196971));
#31381=CARTESIAN_POINT('Ctrl Pts',(-37.6352765540523,3.3201650196893,-33.5196880727089));
#31382=CARTESIAN_POINT('Ctrl Pts',(-37.6236857795041,3.43146974877078,-34.261318219947));
#31383=CARTESIAN_POINT('Ctrl Pts',(-37.6133520513342,3.53951935406892,-35.0050084877505));
#31384=CARTESIAN_POINT('Ctrl Pts',(-37.6078242854473,3.61074952100345,-35.5020159286179));
#31385=CARTESIAN_POINT('Ctrl Pts',(-37.6043859413745,3.66452465859539,-35.8759848351879));
#31386=CARTESIAN_POINT('Ctrl Pts',(-37.6026077149196,3.69976408043587,-36.1223505688103));
#31387=CARTESIAN_POINT('Ctrl Pts',(-37.599521736483,3.76888157611279,-36.61706583695));
#31388=CARTESIAN_POINT('Ctrl Pts',(-37.5956363167035,3.88540317672125,-37.4809407775669));
#31389=CARTESIAN_POINT('Ctrl Pts',(-37.5910272717758,4.10181112895166,-39.2087099360799));
#31390=CARTESIAN_POINT('Ctrl Pts',(-37.5842203316147,4.2577499695969,-40.6943345599309));
#31391=CARTESIAN_POINT('Ctrl Pts',(-37.5695004329624,4.36034742096726,-41.8160021984482));
#31392=CARTESIAN_POINT('Ctrl Pts',(-37.5665328375025,4.38195344965808,-42.0583510628435));
#31393=CARTESIAN_POINT('Ctrl Pts',(-37.5619914612557,4.41277915320487,-42.426101932401));
#31394=CARTESIAN_POINT('Ctrl Pts',(-37.5574198149966,4.44190858472651,-42.7942788920664));
#31395=CARTESIAN_POINT('Ctrl Pts',(-37.5510699275548,4.47881121386559,-43.2875510134486));
#31396=CARTESIAN_POINT('Ctrl Pts',(-37.5424456046618,4.5216064260077,-43.9072300669672));
#31397=CARTESIAN_POINT('Ctrl Pts',(-37.5300912088607,4.56887774110081,-44.6558662586516));
#31398=CARTESIAN_POINT('Ctrl Pts',(-37.51734300484,4.60589289567608,-45.2834091457517));
#31399=CARTESIAN_POINT('Ctrl Pts',(-37.5051522081724,4.63477136604078,-45.7875099169756));
#31400=CARTESIAN_POINT('Ctrl Pts',(-37.4948762495891,4.65621548144282,-46.1665760379686));
#31401=CARTESIAN_POINT('Ctrl Pts',(-37.4833238302732,4.6776217492016,-46.5465778715606));
#31402=CARTESIAN_POINT('Ctrl Pts',(-37.4660098448967,4.70636683890851,-47.0545196654333));
#31403=CARTESIAN_POINT('Ctrl Pts',(-37.450643270566,4.72841232401127,-47.4366878571963));
#31404=CARTESIAN_POINT('Ctrl Pts',(-37.4332726036606,4.75130339337673,-47.8210731631867));
#31405=CARTESIAN_POINT('Ctrl Pts',(-37.4202177511839,4.7687530603907,-48.0908393827046));
#31406=CARTESIAN_POINT('Ctrl Pts',(-37.3907011252467,4.80681531263838,-48.6174288437083));
#31407=CARTESIAN_POINT('Ctrl Pts',(-37.330364145368,4.88087940265647,-49.5287521262629));
#31408=CARTESIAN_POINT('Ctrl Pts',(-37.2253304066405,4.99306825383668,-50.7857376411557));
#31409=CARTESIAN_POINT('Ctrl Pts',(-37.0880949687414,5.09629346708032,-52.2184190483748));
#31410=CARTESIAN_POINT('Ctrl Pts',(-37.0044748217046,5.11858167612536,-53.1159739539212));
#31411=CARTESIAN_POINT('Ctrl Pts',(-36.9601697039679,5.11062258468734,-53.6591378281997));
#31412=CARTESIAN_POINT('Ctrl Pts',(-36.9420090151494,5.10243329745112,-53.8510380841647));
#31413=CARTESIAN_POINT('Ctrl Pts',(-36.9054489373111,5.07227248968504,-54.268045146635));
#31414=CARTESIAN_POINT('Ctrl Pts',(-36.8424140357631,4.98413489528138,-55.0311205144958));
#31415=CARTESIAN_POINT('Ctrl Pts',(-36.7331692162939,4.7101346920984,-56.7253922598548));
#31416=CARTESIAN_POINT('Ctrl Pts',(-36.6715454224966,4.46365934886385,-58.4421024895548));
#31417=CARTESIAN_POINT('Ctrl Pts',(-36.6475119464927,4.55546795666475,-59.7851949896994));
#31418=CARTESIAN_POINT('Ctrl Pts',(-36.6449059782589,4.56606514697575,-59.9247754976334));
#31419=CARTESIAN_POINT('Ctrl Pts',(-36.6407132493246,4.59161748760519,-60.2162198707081));
#31420=CARTESIAN_POINT('Ctrl Pts',(-36.6359637670275,4.64494516710093,-60.7173390880193));
#31421=CARTESIAN_POINT('Ctrl Pts',(-36.6356179299687,4.78614159531689,-61.7151817385737));
#31422=CARTESIAN_POINT('Ctrl Pts',(-36.6505932905658,5.01770949926151,-62.8302806803964));
#31423=CARTESIAN_POINT('Ctrl Pts',(-36.6702551267837,5.30484735480991,-63.9217143924267));
#31424=CARTESIAN_POINT('Ctrl Pts',(-36.6811882701522,5.48443590993431,-64.5254920127128));
#31425=CARTESIAN_POINT('Ctrl Pts',(-36.6876545273568,5.61053871830678,-64.9237987567574));
#31426=CARTESIAN_POINT('Ctrl Pts',(-36.6917013086277,5.69622530650803,-65.1881525877755));
#31427=CARTESIAN_POINT('Ctrl Pts',(-36.6952656678883,5.78426189393477,-65.4508510728054));
#31428=CARTESIAN_POINT('Ctrl Pts',(-36.6978474820544,5.86310702128428,-65.6791061932655));
#31429=CARTESIAN_POINT('Ctrl Pts',(-36.6991500771139,5.90865362346796,-65.8090850134188));
#31430=CARTESIAN_POINT('Ctrl Pts',(-36.7009227045981,5.97746142112317,-66.0036242828082));
#31431=CARTESIAN_POINT('Ctrl Pts',(-36.7019998161728,6.03575793707553,-66.1647643785117));
#31432=CARTESIAN_POINT('Ctrl Pts',(-36.7031586109764,6.13363851366078,-66.430917607253));
#31433=CARTESIAN_POINT('Ctrl Pts',(-36.7038836856841,6.2510371660943,-66.7354556850828));
#31434=CARTESIAN_POINT('Ctrl Pts',(-36.7050109434939,6.49353163277098,-67.3132344553444));
#31435=CARTESIAN_POINT('Ctrl Pts',(-36.7057406882881,6.953561818789,-68.3024919286853));
#31436=CARTESIAN_POINT('Ctrl Pts',(-36.704221792431,7.95641216887806,-70.1615298613546));
#31437=CARTESIAN_POINT('Ctrl Pts',(-36.7020473445366,8.83230535659937,-71.6214506940054));
#31438=CARTESIAN_POINT('Ctrl Pts',(-36.7036840316439,9.38520851996215,-72.6730413981383));
#31439=CARTESIAN_POINT('Ctrl Pts',(-36.7036514060824,9.52095780102533,-72.9307926088001));
#31440=CARTESIAN_POINT('Ctrl Pts',(-36.7037729430077,9.78577010106223,-73.4323636649782));
#31441=CARTESIAN_POINT('Ctrl Pts',(-36.7037702968015,10.1203926230654,-74.0641471677288));
#31442=CARTESIAN_POINT('Ctrl Pts',(-36.7037495101504,10.5210994519818,-74.8180587766035));
#31443=CARTESIAN_POINT('Ctrl Pts',(-36.7035868948437,11.3242891788236,-76.3256640873389));
#31444=CARTESIAN_POINT('Ctrl Pts',(-36.7033606006525,11.9937021323769,-77.5781837508716));
#31445=CARTESIAN_POINT('Ctrl Pts',(-36.7034150745067,12.9615748789859,-79.3986762846247));
#31446=CARTESIAN_POINT('Ctrl Pts',(-36.7033839066019,13.3989424741646,-80.2213448491822));
#31447=CARTESIAN_POINT('Ctrl Pts',(-36.703383906602,13.835464061554,-81.0423225512805));
#31448=CARTESIAN_POINT('Ctrl Pts',(-34.1764447559102,0.0259685887429924,
24.8306203013275));
#31449=CARTESIAN_POINT('Ctrl Pts',(-34.1765480191343,0.0259706743427907,
24.781740533954));
#31450=CARTESIAN_POINT('Ctrl Pts',(-34.1766563187642,0.0259728602730872,
24.7328618093536));
#31451=CARTESIAN_POINT('Ctrl Pts',(-34.177935244816,0.0259987139595002,
24.1822484567547));
#31452=CARTESIAN_POINT('Ctrl Pts',(-34.1789192015653,0.0260245301400927,
23.1781109563667));
#31453=CARTESIAN_POINT('Ctrl Pts',(-34.1812111794164,0.0260877526726797,
21.1695007383349));
#31454=CARTESIAN_POINT('Ctrl Pts',(-34.1897227180841,0.0262600038941574,
19.6653375775111));
#31455=CARTESIAN_POINT('Ctrl Pts',(-34.2077555773017,0.0265955167688952,
18.4142816557505));
#31456=CARTESIAN_POINT('Ctrl Pts',(-34.2164043864526,0.026759174673617,
17.9114377995702));
#31457=CARTESIAN_POINT('Ctrl Pts',(-34.2381226623577,0.0271751853534956,
16.9074310683423));
#31458=CARTESIAN_POINT('Ctrl Pts',(-34.2847040215993,0.0280665516383967,
15.1536348084952));
#31459=CARTESIAN_POINT('Ctrl Pts',(-34.3289440787915,0.0288744170692373,
13.6519879457826));
#31460=CARTESIAN_POINT('Ctrl Pts',(-34.3566565846591,0.0293063872750294,
12.3976215172641));
#31461=CARTESIAN_POINT('Ctrl Pts',(-34.367982385136,0.0294745804022541,
11.8967125448909));
#31462=CARTESIAN_POINT('Ctrl Pts',(-34.3910627681017,0.0297910247937516,
10.8949354521761));
#31463=CARTESIAN_POINT('Ctrl Pts',(-34.4309925890151,0.0302831881620811,
9.14146337731071));
#31464=CARTESIAN_POINT('Ctrl Pts',(-34.4590006955027,0.0305702214085873,
7.63620452746495));
#31465=CARTESIAN_POINT('Ctrl Pts',(-34.4714526930686,0.0306863666185977,
6.50520016575504));
#31466=CARTESIAN_POINT('Ctrl Pts',(-34.4740409189562,0.0307019421184336,
6.25507309871996));
#31467=CARTESIAN_POINT('Ctrl Pts',(-34.4785821354951,0.030699029376128,
5.75405743334002));
#31468=CARTESIAN_POINT('Ctrl Pts',(-34.484920601066,0.03062048531772,4.87578204819422));
#31469=CARTESIAN_POINT('Ctrl Pts',(-34.4916138238924,0.0302903478700228,
3.11542709937152));
#31470=CARTESIAN_POINT('Ctrl Pts',(-34.4886869377477,0.0301425423443907,
1.60816029882331));
#31471=CARTESIAN_POINT('Ctrl Pts',(-34.4839896140949,0.0304955552585745,
0.548003023478769));
#31472=CARTESIAN_POINT('Ctrl Pts',(-34.4833725318882,0.0305416251743624,
0.421705744044932));
#31473=CARTESIAN_POINT('Ctrl Pts',(-34.4819234181444,0.0306499058822111,
0.169346943515288));
#31474=CARTESIAN_POINT('Ctrl Pts',(-34.4788505524739,0.0308785738956989,
-0.271757550688972));
#31475=CARTESIAN_POINT('Ctrl Pts',(-34.4730977900133,0.0313026784127056,
-0.900513330898582));
#31476=CARTESIAN_POINT('Ctrl Pts',(-34.4645288667361,0.0319138001759487,
-1.6532738974642));
#31477=CARTESIAN_POINT('Ctrl Pts',(-34.4516077232543,0.0328022853878508,
-2.65522365151925));
#31478=CARTESIAN_POINT('Ctrl Pts',(-34.4339496901778,0.0339207349723135,
-3.90560610978848));
#31479=CARTESIAN_POINT('Ctrl Pts',(-34.4210607531741,0.0345605068751547,
-4.9061316839446));
#31480=CARTESIAN_POINT('Ctrl Pts',(-34.4142586034067,0.0347905599414902,
-5.53243263620395));
#31481=CARTESIAN_POINT('Ctrl Pts',(-34.411552250874,0.0349353447619312,
-5.78405959293063));
#31482=CARTESIAN_POINT('Ctrl Pts',(-34.4062021269632,0.0353907288013687,
-6.28681327556158));
#31483=CARTESIAN_POINT('Ctrl Pts',(-34.3969869916172,0.0365103197768133,
-7.16686416697398));
#31484=CARTESIAN_POINT('Ctrl Pts',(-34.3841583516796,0.0383883562234742,
-8.42268589789923));
#31485=CARTESIAN_POINT('Ctrl Pts',(-34.3715179979297,0.0388972389018156,
-9.67421926002958));
#31486=CARTESIAN_POINT('Ctrl Pts',(-34.3626323059108,0.0376172677793105,
-10.5464996684573));
#31487=CARTESIAN_POINT('Ctrl Pts',(-34.3575249176696,0.0362881792757959,
-11.0436539495391));
#31488=CARTESIAN_POINT('Ctrl Pts',(-34.3549594447717,0.0354026940840104,
-11.2917817789517));
#31489=CARTESIAN_POINT('Ctrl Pts',(-34.353020902462,0.0346440961100884,
-11.4784125652706));
#31490=CARTESIAN_POINT('Ctrl Pts',(-34.3515853254475,0.0340253440693036,
-11.6018310614995));
#31491=CARTESIAN_POINT('Ctrl Pts',(-34.3482348486648,0.0323903181822838,
-11.8498926617208));
#31492=CARTESIAN_POINT('Ctrl Pts',(-34.3412463574436,0.0285811707377088,
-12.2836696573919));
#31493=CARTESIAN_POINT('Ctrl Pts',(-34.3188269874935,0.0148037986272326,
-13.4013716450607));
#31494=CARTESIAN_POINT('Ctrl Pts',(-34.2887178607569,-0.00644829959073418,
-14.6519870417332));
#31495=CARTESIAN_POINT('Ctrl Pts',(-34.2770936766063,-0.0173469197916623,
-15.9208591392115));
#31496=CARTESIAN_POINT('Ctrl Pts',(-34.2778715282682,-0.0189151721828352,
-16.5603275873268));
#31497=CARTESIAN_POINT('Ctrl Pts',(-34.2835910948713,-0.0170361134882322,
-17.0753241807094));
#31498=CARTESIAN_POINT('Ctrl Pts',(-34.2883451506099,-0.0149121363734472,
-17.3340551145771));
#31499=CARTESIAN_POINT('Ctrl Pts',(-34.2926726541808,-0.0128327334582615,
-17.527607743022));
#31500=CARTESIAN_POINT('Ctrl Pts',(-34.2957083466975,-0.0114556391860327,
-17.6501483562369));
#31501=CARTESIAN_POINT('Ctrl Pts',(-34.3024626660491,-0.00884695070967751,
-17.8989735893196));
#31502=CARTESIAN_POINT('Ctrl Pts',(-34.3102090859748,-0.00635436130592169,
-18.1473631261843));
#31503=CARTESIAN_POINT('Ctrl Pts',(-34.3188794786108,-0.00390516257062937,
-18.397159467746));
#31504=CARTESIAN_POINT('Ctrl Pts',(-34.3246725770309,-0.00236337394245413,
-18.553466654483));
#31505=CARTESIAN_POINT('Ctrl Pts',(-34.3295238385326,-0.00111268941660546,
-18.67876279445));
#31506=CARTESIAN_POINT('Ctrl Pts',(-34.3345179440761,0.000154153990505383,
-18.8041757961903));
#31507=CARTESIAN_POINT('Ctrl Pts',(-34.3488294337639,0.00374222852032763,
-19.1496292775457));
#31508=CARTESIAN_POINT('Ctrl Pts',(-34.3753237352747,0.010295460514461,
-19.7179520756166));
#31509=CARTESIAN_POINT('Ctrl Pts',(-34.4302004564404,0.0269303197528827,
-20.737473605222));
#31510=CARTESIAN_POINT('Ctrl Pts',(-34.5123332226738,0.0632200852246043,
-22.03016336335));
#31511=CARTESIAN_POINT('Ctrl Pts',(-34.588378884647,0.12643758942332,-23.0852752905503));
#31512=CARTESIAN_POINT('Ctrl Pts',(-34.6367374718653,0.18257139651334,-23.7495053415597));
#31513=CARTESIAN_POINT('Ctrl Pts',(-34.6568882840014,0.206942034622488,
-24.0174275813682));
#31514=CARTESIAN_POINT('Ctrl Pts',(-34.7002228691302,0.263440964308869,
-24.5469866326856));
#31515=CARTESIAN_POINT('Ctrl Pts',(-34.7824956712819,0.380990003104775,
-25.4672846369282));
#31516=CARTESIAN_POINT('Ctrl Pts',(-34.9084923498233,0.591534619965779,
-26.7554490787649));
#31517=CARTESIAN_POINT('Ctrl Pts',(-35.045972665964,0.87096394672074,-28.2560450148336));
#31518=CARTESIAN_POINT('Ctrl Pts',(-35.1159825518541,1.04214946371602,-29.2248771910313));
#31519=CARTESIAN_POINT('Ctrl Pts',(-35.147426229867,1.12467880819707,-29.7614661868142));
#31520=CARTESIAN_POINT('Ctrl Pts',(-35.1541715034908,1.14325309257035,-29.885785553879));
#31521=CARTESIAN_POINT('Ctrl Pts',(-35.1671738936228,1.1797785822778,-30.1318470076868));
#31522=CARTESIAN_POINT('Ctrl Pts',(-35.1885183811244,1.24269729319185,-30.5645356763689));
#31523=CARTESIAN_POINT('Ctrl Pts',(-35.2261496790866,1.36441854460525,-31.4312425399043));
#31524=CARTESIAN_POINT('Ctrl Pts',(-35.259457736917,1.49582490437396,-32.427062269871));
#31525=CARTESIAN_POINT('Ctrl Pts',(-35.2865720248284,1.623146359731,-33.4256684888729));
#31526=CARTESIAN_POINT('Ctrl Pts',(-35.3045754711524,1.71760899132426,-34.1758807071139));
#31527=CARTESIAN_POINT('Ctrl Pts',(-35.3209683482824,1.81196474024708,-34.9268708239082));
#31528=CARTESIAN_POINT('Ctrl Pts',(-35.3312868839817,1.87550180720795,-35.4278812620332));
#31529=CARTESIAN_POINT('Ctrl Pts',(-35.3389836740974,1.9237881832193,-35.8046197278162));
#31530=CARTESIAN_POINT('Ctrl Pts',(-35.3442435332927,1.95598856799882,-36.0547424865498));
#31531=CARTESIAN_POINT('Ctrl Pts',(-35.3547061858924,2.02038327537595,-36.5556382205856));
#31532=CARTESIAN_POINT('Ctrl Pts',(-35.3728056791848,2.13248774397748,-37.4302883273256));
#31533=CARTESIAN_POINT('Ctrl Pts',(-35.4062812466005,2.35380345787832,-39.1773607273832));
#31534=CARTESIAN_POINT('Ctrl Pts',(-35.4239022459999,2.53348259946413,-40.6774928642993));
#31535=CARTESIAN_POINT('Ctrl Pts',(-35.4241465093225,2.65916632645815,-41.8091242366946));
#31536=CARTESIAN_POINT('Ctrl Pts',(-35.4247462543187,2.68537536054886,-42.0492494691377));
#31537=CARTESIAN_POINT('Ctrl Pts',(-35.4251349689881,2.72277666504169,-42.4172280256115));
#31538=CARTESIAN_POINT('Ctrl Pts',(-35.4252853138477,2.75824759465529,-42.7860354981063));
#31539=CARTESIAN_POINT('Ctrl Pts',(-35.4248317572573,2.8037332042836,-43.2822379294712));
#31540=CARTESIAN_POINT('Ctrl Pts',(-35.4228770896236,2.85811465763686,-43.9084301033932));
#31541=CARTESIAN_POINT('Ctrl Pts',(-35.417311058886,2.92290442773719,-44.6698102121672));
#31542=CARTESIAN_POINT('Ctrl Pts',(-35.4091513232251,2.97943063806857,-45.311954153181));
#31543=CARTESIAN_POINT('Ctrl Pts',(-35.3999100222585,3.02803855823651,-45.830164972453));
#31544=CARTESIAN_POINT('Ctrl Pts',(-35.3914714749811,3.0666435275713,-46.2210682704118));
#31545=CARTESIAN_POINT('Ctrl Pts',(-35.3813564535755,3.10787646492832,-46.6141898897007));
#31546=CARTESIAN_POINT('Ctrl Pts',(-35.3653687619548,3.1670258645019,-47.1413517987742));
#31547=CARTESIAN_POINT('Ctrl Pts',(-35.3503107206238,3.21680331408655,-47.5400216957549));
#31548=CARTESIAN_POINT('Ctrl Pts',(-35.3326246137773,3.27145538187517,-47.9423865315486));
#31549=CARTESIAN_POINT('Ctrl Pts',(-35.3183119345572,3.31249728321088,-48.2260516348631));
#31550=CARTESIAN_POINT('Ctrl Pts',(-35.2865988651605,3.40282719589082,-48.7769682789169));
#31551=CARTESIAN_POINT('Ctrl Pts',(-35.2221127750781,3.58077321947741,-49.7262778060027));
#31552=CARTESIAN_POINT('Ctrl Pts',(-35.1137593741292,3.86342779255355,-51.0239732801702));
#31553=CARTESIAN_POINT('Ctrl Pts',(-34.9762521475711,4.16691945495112,-52.4854944337859));
#31554=CARTESIAN_POINT('Ctrl Pts',(-34.8885472983672,4.29756020423801,-53.3819511812763));
#31555=CARTESIAN_POINT('Ctrl Pts',(-34.8370493297166,4.34621727555356,-53.9147329162006));
#31556=CARTESIAN_POINT('Ctrl Pts',(-34.8157958118834,4.36068859569375,-54.1265981568054));
#31557=CARTESIAN_POINT('Ctrl Pts',(-34.768631396821,4.37775308482033,-54.5626870837952));
#31558=CARTESIAN_POINT('Ctrl Pts',(-34.6769728514841,4.3790834998756,-55.3502991729764));
#31559=CARTESIAN_POINT('Ctrl Pts',(-34.4703881875133,4.31550812532453,-57.0345848267836));
#31560=CARTESIAN_POINT('Ctrl Pts',(-34.3052078475783,4.29868794505819,-58.6813927067186));
#31561=CARTESIAN_POINT('Ctrl Pts',(-34.2389432707123,4.47416039380388,-59.926986696457));
#31562=CARTESIAN_POINT('Ctrl Pts',(-34.231463357557,4.49260480950002,-60.0560807286205));
#31563=CARTESIAN_POINT('Ctrl Pts',(-34.2178691418411,4.53282011579336,-60.3270192009488));
#31564=CARTESIAN_POINT('Ctrl Pts',(-34.1978085732581,4.60623812460767,-60.7953802851783));
#31565=CARTESIAN_POINT('Ctrl Pts',(-34.1709155858825,4.76983222090131,-61.7386111802352));
#31566=CARTESIAN_POINT('Ctrl Pts',(-34.1637778925812,4.99512102374594,-62.8160929526715));
#31567=CARTESIAN_POINT('Ctrl Pts',(-34.167090502353,5.2654214482681,-63.8931464258179));
#31568=CARTESIAN_POINT('Ctrl Pts',(-34.170474004141,5.43561574664774,-64.497241832218));
#31569=CARTESIAN_POINT('Ctrl Pts',(-34.1723711287775,5.55721115726879,-64.8991000042908));
#31570=CARTESIAN_POINT('Ctrl Pts',(-34.1734792843691,5.64047104498202,-65.1667042461347));
#31571=CARTESIAN_POINT('Ctrl Pts',(-34.1742466344374,5.72712066020137,-65.4339225707906));
#31572=CARTESIAN_POINT('Ctrl Pts',(-34.1744645507659,5.80596045959028,-65.6672469462392));
#31573=CARTESIAN_POINT('Ctrl Pts',(-34.174435438371,5.85189259297455,-65.8004333090785));
#31574=CARTESIAN_POINT('Ctrl Pts',(-34.1742272593377,5.92168347597517,-66.0000802553368));
#31575=CARTESIAN_POINT('Ctrl Pts',(-34.173683287128,5.98170708043398,-66.1661304146234));
#31576=CARTESIAN_POINT('Ctrl Pts',(-34.1721771518986,6.08376886778207,-66.440957951523));
#31577=CARTESIAN_POINT('Ctrl Pts',(-34.1707247734496,6.20051035645416,-66.7410825653339));
#31578=CARTESIAN_POINT('Ctrl Pts',(-34.168627217271,6.4438181995821,-67.3180377329392));
#31579=CARTESIAN_POINT('Ctrl Pts',(-34.1666336424948,6.90263474958834,-68.3028697099307));
#31580=CARTESIAN_POINT('Ctrl Pts',(-34.1674540085646,7.90114792029037,-70.1595842761014));
#31581=CARTESIAN_POINT('Ctrl Pts',(-34.1714825205131,8.77266649621883,-71.6191472444224));
#31582=CARTESIAN_POINT('Ctrl Pts',(-34.1722134259569,9.3266065933815,-72.6734520257454));
#31583=CARTESIAN_POINT('Ctrl Pts',(-34.1721742703938,9.46222766969651,-72.9311238226013));
#31584=CARTESIAN_POINT('Ctrl Pts',(-34.1722036357289,9.72703498910348,-73.4329215553792));
#31585=CARTESIAN_POINT('Ctrl Pts',(-34.1721788912052,10.0616140288131,-74.0647536923517));
#31586=CARTESIAN_POINT('Ctrl Pts',(-34.1721637242811,10.4623925547618,-74.8188030680971));
#31587=CARTESIAN_POINT('Ctrl Pts',(-34.1721036934396,11.2657757252011,-76.3265339173854));
#31588=CARTESIAN_POINT('Ctrl Pts',(-34.172046148687,11.9353594497907,-77.5788066455772));
#31589=CARTESIAN_POINT('Ctrl Pts',(-34.1720774576037,12.9030459298434,-79.3988899707441));
#31590=CARTESIAN_POINT('Ctrl Pts',(-34.1720596536215,13.340445430675,-80.2215858878274));
#31591=CARTESIAN_POINT('Ctrl Pts',(-34.1720596536215,13.7769670180645,-81.0425635899257));
#31592=CARTESIAN_POINT('Ctrl Pts',(-31.9633899561928,0.00119778082931517,
24.83063334628));
#31593=CARTESIAN_POINT('Ctrl Pts',(-31.963486415328,0.00119848231513045,
24.7817539900166));
#31594=CARTESIAN_POINT('Ctrl Pts',(-31.963587579573,0.00119921736695464,
24.7328756853541));
#31595=CARTESIAN_POINT('Ctrl Pts',(-31.9647822144503,0.00120792687973987,
24.1822671216868));
#31596=CARTESIAN_POINT('Ctrl Pts',(-31.9657019119787,0.00121427805477512,
23.1781340896351));
#31597=CARTESIAN_POINT('Ctrl Pts',(-31.9678452034461,0.00122829672387729,
21.1695331470275));
#31598=CARTESIAN_POINT('Ctrl Pts',(-31.9757952029295,0.00128662321772465,
19.6653742893852));
#31599=CARTESIAN_POINT('Ctrl Pts',(-31.9926356403998,0.00141196690703649,
18.4143207108312));
#31600=CARTESIAN_POINT('Ctrl Pts',(-32.0007139956558,0.00147248024287243,
17.9115005631452));
#31601=CARTESIAN_POINT('Ctrl Pts',(-32.0210021408705,0.00162548582569014,
16.9075098249226));
#31602=CARTESIAN_POINT('Ctrl Pts',(-32.064517452415,0.00195429177169138,
15.1537076950091));
#31603=CARTESIAN_POINT('Ctrl Pts',(-32.1058279763341,0.00226423029483334,
13.6519809000191));
#31604=CARTESIAN_POINT('Ctrl Pts',(-32.1316771815726,0.00245046653420001,
12.3975155713652));
#31605=CARTESIAN_POINT('Ctrl Pts',(-32.1422393341866,0.00252575916266231,
11.8965655658827));
#31606=CARTESIAN_POINT('Ctrl Pts',(-32.1637543912761,0.00267706382077597,
10.8947278493917));
#31607=CARTESIAN_POINT('Ctrl Pts',(-32.200957346963,0.002933521609905,9.14119507582939));
#31608=CARTESIAN_POINT('Ctrl Pts',(-32.2270184972505,0.0031079433499766,
7.63596847755042));
#31609=CARTESIAN_POINT('Ctrl Pts',(-32.2385906509075,0.00318140759757139,
6.50502566211766));
#31610=CARTESIAN_POINT('Ctrl Pts',(-32.240993356192,0.00319344205154197,
6.25484166364325));
#31611=CARTESIAN_POINT('Ctrl Pts',(-32.2451971504006,0.00320342667236139,
5.75377227711905));
#31612=CARTESIAN_POINT('Ctrl Pts',(-32.251033308732,0.00319090078006513,
4.87542789539196));
#31613=CARTESIAN_POINT('Ctrl Pts',(-32.2570919217592,0.00309167642484667,
3.11514117234228));
#31614=CARTESIAN_POINT('Ctrl Pts',(-32.2542667706258,0.00305980010968048,
1.608240603948));
#31615=CARTESIAN_POINT('Ctrl Pts',(-32.2499919488482,0.00321703737406999,
0.548503699734546));
#31616=CARTESIAN_POINT('Ctrl Pts',(-32.2494317489446,0.00323715527579488,
0.422276103173599));
#31617=CARTESIAN_POINT('Ctrl Pts',(-32.2481177291307,0.00328435765801334,
0.170036446586959));
#31618=CARTESIAN_POINT('Ctrl Pts',(-32.2453355398337,0.00338329837949874,
-0.270874468574266));
#31619=CARTESIAN_POINT('Ctrl Pts',(-32.2401289344388,0.00356642375268749,
-0.899419623093153));
#31620=CARTESIAN_POINT('Ctrl Pts',(-32.2323778555354,0.00382560313618471,
-1.65202044069393));
#31621=CARTESIAN_POINT('Ctrl Pts',(-32.2206654026539,0.00420060825483769,
-2.65388902201657));
#31622=CARTESIAN_POINT('Ctrl Pts',(-32.2046156275384,0.00466044519571738,
-3.90438805638575));
#31623=CARTESIAN_POINT('Ctrl Pts',(-32.1927725437737,0.00491225358191858,
-4.9052688291125));
#31624=CARTESIAN_POINT('Ctrl Pts',(-32.1864653645559,0.00499290243202669,
-5.53181917851233));
#31625=CARTESIAN_POINT('Ctrl Pts',(-32.1839612151424,0.00502739650865295,
-5.78278124881988));
#31626=CARTESIAN_POINT('Ctrl Pts',(-32.1790195663831,0.00510449628433056,
-6.28488274216901));
#31627=CARTESIAN_POINT('Ctrl Pts',(-32.1705210287039,0.00524909157024554,
-7.16411633179275));
#31628=CARTESIAN_POINT('Ctrl Pts',(-32.1586291276295,0.00542161434796207,
-8.4205372245363));
#31629=CARTESIAN_POINT('Ctrl Pts',(-32.146652015432,0.00537912234140981,
-9.6747258081599));
#31630=CARTESIAN_POINT('Ctrl Pts',(-32.1379970004511,0.00514992564405705,
-10.5500118621068));
#31631=CARTESIAN_POINT('Ctrl Pts',(-32.1329426296684,0.00495142736476526,
-11.0492147722401));
#31632=CARTESIAN_POINT('Ctrl Pts',(-32.1303718438646,0.00482809344718019,
-11.2984600882129));
#31633=CARTESIAN_POINT('Ctrl Pts',(-32.1284184632243,0.00472552966013362,
-11.4860294914805));
#31634=CARTESIAN_POINT('Ctrl Pts',(-32.1270425359593,0.00465137659907829,
-11.6119657079845));
#31635=CARTESIAN_POINT('Ctrl Pts',(-32.1240617896758,0.00447600785169626,
-11.8636240728352));
#31636=CARTESIAN_POINT('Ctrl Pts',(-32.1182999721354,0.00410789350910049,
-12.3033615968514));
#31637=CARTESIAN_POINT('Ctrl Pts',(-32.1012865417164,0.00290356550380467,
-13.4313439833862));
#31638=CARTESIAN_POINT('Ctrl Pts',(-32.0794453681356,0.00111694721556185,
-14.6793098499892));
#31639=CARTESIAN_POINT('Ctrl Pts',(-32.0657768239458,-0.000412029585329937,
-15.9311210824324));
#31640=CARTESIAN_POINT('Ctrl Pts',(-32.0618775272173,-0.00105043126173075,
-16.5587290362317));
#31641=CARTESIAN_POINT('Ctrl Pts',(-32.0611309886276,-0.00145536140317013,
-17.0623192438171));
#31642=CARTESIAN_POINT('Ctrl Pts',(-32.0616249769825,-0.00161050528413247,
-17.3146953342562));
#31643=CARTESIAN_POINT('Ctrl Pts',(-32.0623618610294,-0.00170653275002977,
-17.5034091618793));
#31644=CARTESIAN_POINT('Ctrl Pts',(-32.0628530949887,-0.00183129271206578,
-17.62715680891));
#31645=CARTESIAN_POINT('Ctrl Pts',(-32.0638781191395,-0.00217493216688328,
-17.8755151481028));
#31646=CARTESIAN_POINT('Ctrl Pts',(-32.0649763454848,-0.00266617360748607,
-18.1239882231087));
#31647=CARTESIAN_POINT('Ctrl Pts',(-32.0662428621126,-0.00324346823411917,
-18.3729472805465));
#31648=CARTESIAN_POINT('Ctrl Pts',(-32.0671071195084,-0.00363231595324318,
-18.5286660178601));
#31649=CARTESIAN_POINT('Ctrl Pts',(-32.0678541578989,-0.00395311658654445,
-18.6533413353119));
#31650=CARTESIAN_POINT('Ctrl Pts',(-32.0686393791069,-0.00427792217060808,
-18.7780730762426));
#31651=CARTESIAN_POINT('Ctrl Pts',(-32.0709513003664,-0.00519258990406764,
-19.1213246305473));
#31652=CARTESIAN_POINT('Ctrl Pts',(-32.0757287337685,-0.00665094281689207,
-19.6843236758518));
#31653=CARTESIAN_POINT('Ctrl Pts',(-32.0881606714366,-0.00840130287364682,
-20.6888453830507));
#31654=CARTESIAN_POINT('Ctrl Pts',(-32.1129225851262,-0.00756561865649902,
-21.9510487186381));
#31655=CARTESIAN_POINT('Ctrl Pts',(-32.1474366561549,-0.00189334990781983,
-22.9680105823071));
#31656=CARTESIAN_POINT('Ctrl Pts',(-32.1757176507403,0.00431896066786876,
-23.6045341315906));
#31657=CARTESIAN_POINT('Ctrl Pts',(-32.1879292627242,0.0068719456290228,
-23.8544532539764));
#31658=CARTESIAN_POINT('Ctrl Pts',(-32.2162312123548,0.0126773366715741,
-24.3563730776259));
#31659=CARTESIAN_POINT('Ctrl Pts',(-32.2748706455199,0.024969194001814,
-25.2364165939835));
#31660=CARTESIAN_POINT('Ctrl Pts',(-32.3786778435036,0.0513919839388159,
-26.4994086242991));
#31661=CARTESIAN_POINT('Ctrl Pts',(-32.5122749838379,0.101647104051024,
-28.0190052683457));
#31662=CARTESIAN_POINT('Ctrl Pts',(-32.5898304514288,0.144960956006053,
-29.0308522953232));
#31663=CARTESIAN_POINT('Ctrl Pts',(-32.6257479842602,0.169979253770006,
-29.5987031989526));
#31664=CARTESIAN_POINT('Ctrl Pts',(-32.6336861496392,0.175447346686321,
-29.7240888929289));
#31665=CARTESIAN_POINT('Ctrl Pts',(-32.6492514964225,0.186521785199724,
-29.9755083146498));
#31666=CARTESIAN_POINT('Ctrl Pts',(-32.6757338386092,0.206108161838533,
-30.4156921895497));
#31667=CARTESIAN_POINT('Ctrl Pts',(-32.7258571497013,0.246439084399044,
-31.2978925893485));
#31668=CARTESIAN_POINT('Ctrl Pts',(-32.7774103551025,0.296091287968215,
-32.3090426401619));
#31669=CARTESIAN_POINT('Ctrl Pts',(-32.8249726523566,0.351419932056421,
-33.3220680979162));
#31670=CARTESIAN_POINT('Ctrl Pts',(-32.8590641990171,0.396329061978688,
-34.0824306694152));
#31671=CARTESIAN_POINT('Ctrl Pts',(-32.8918831270656,0.445269987187108,
-34.8429797692874));
#31672=CARTESIAN_POINT('Ctrl Pts',(-32.9132036462384,0.480991058541578,
-35.34996569469));
#31673=CARTESIAN_POINT('Ctrl Pts',(-32.9291295102912,0.509166421897822,
-35.7311084598365));
#31674=CARTESIAN_POINT('Ctrl Pts',(-32.9398787407322,0.528403120565872,
-35.9852790675309));
#31675=CARTESIAN_POINT('Ctrl Pts',(-32.9614622283884,0.568373208158851,
-36.4933031905527));
#31676=CARTESIAN_POINT('Ctrl Pts',(-32.9991180244276,0.641977900674228,
-37.3798806011782));
#31677=CARTESIAN_POINT('Ctrl Pts',(-33.0712435325354,0.801360507046883,
-39.1472531161535));
#31678=CARTESIAN_POINT('Ctrl Pts',(-33.1186067375816,0.952013620523383,
-40.6594854156347));
#31679=CARTESIAN_POINT('Ctrl Pts',(-33.1377759168148,1.06467111808059,-41.797880604425));
#31680=CARTESIAN_POINT('Ctrl Pts',(-33.1424761583679,1.08750542024222,-42.0352953990767));
#31681=CARTESIAN_POINT('Ctrl Pts',(-33.1487725066544,1.12002822361257,-42.4026020567513));
#31682=CARTESIAN_POINT('Ctrl Pts',(-33.1546134098907,1.15073236623629,-42.7711097762434));
#31683=CARTESIAN_POINT('Ctrl Pts',(-33.1614844769426,1.19044675002746,-43.2688659578312));
#31684=CARTESIAN_POINT('Ctrl Pts',(-33.168217111019,1.23915922377811,-43.8996126182923));
#31685=CARTESIAN_POINT('Ctrl Pts',(-33.1724047691856,1.30155995660813,-44.6708248666733));
#31686=CARTESIAN_POINT('Ctrl Pts',(-33.171848709337,1.36144920188157,-45.3244573998258));
#31687=CARTESIAN_POINT('Ctrl Pts',(-33.1683254913266,1.41695997132591,-45.8536664211606));
#31688=CARTESIAN_POINT('Ctrl Pts',(-33.1640407718665,1.46315617965921,-46.2536671617113));
#31689=CARTESIAN_POINT('Ctrl Pts',(-33.157956831207,1.51466683832569,-46.6566748244397));
#31690=CARTESIAN_POINT('Ctrl Pts',(-33.1471917328883,1.59147860129533,-47.1979163208453));
#31691=CARTESIAN_POINT('Ctrl Pts',(-33.1360240660687,1.65939874991629,-47.6081090714609));
#31692=CARTESIAN_POINT('Ctrl Pts',(-33.1222528318697,1.73608488175619,-48.0222509129967));
#31693=CARTESIAN_POINT('Ctrl Pts',(-33.1110161789402,1.79348070878201,-48.3112911687026));
#31694=CARTESIAN_POINT('Ctrl Pts',(-33.0869896268488,1.92005463882968,-48.8720316258399));
#31695=CARTESIAN_POINT('Ctrl Pts',(-33.0400148518847,2.17032107029229,-49.8333463233307));
#31696=CARTESIAN_POINT('Ctrl Pts',(-32.9672074568071,2.5745685495611,-51.1406511782623));
#31697=CARTESIAN_POINT('Ctrl Pts',(-32.8831126446119,3.04088716857611,-52.6173629512002));
#31698=CARTESIAN_POINT('Ctrl Pts',(-32.8313136420262,3.28144591160892,-53.5347432801643));
#31699=CARTESIAN_POINT('Ctrl Pts',(-32.7982104275538,3.39474521054215,-54.0845057230478));
#31700=CARTESIAN_POINT('Ctrl Pts',(-32.7828042277012,3.43945308197284,-54.3169641369898));
#31701=CARTESIAN_POINT('Ctrl Pts',(-32.7480508776641,3.5183173872759,-54.7827999168957));
#31702=CARTESIAN_POINT('Ctrl Pts',(-32.6763054399274,3.63577804335648,-55.6164158521495));
#31703=CARTESIAN_POINT('Ctrl Pts',(-32.4972734098398,3.8175982572053,-57.3413344054663));
#31704=CARTESIAN_POINT('Ctrl Pts',(-32.3197492131095,4.0060677251506,-58.9245285098112));
#31705=CARTESIAN_POINT('Ctrl Pts',(-32.2367784110144,4.25684399776631,-60.0831956985914));
#31706=CARTESIAN_POINT('Ctrl Pts',(-32.2274934881362,4.28368004661584,-60.2080193295285));
#31707=CARTESIAN_POINT('Ctrl Pts',(-32.2091622758131,4.34003457150938,-60.4673425661025));
#31708=CARTESIAN_POINT('Ctrl Pts',(-32.1788227946222,4.43923363502762,-60.9181944078175));
#31709=CARTESIAN_POINT('Ctrl Pts',(-32.1240781685771,4.64620879476816,-61.8293188184246));
#31710=CARTESIAN_POINT('Ctrl Pts',(-32.0745304065476,4.90556161313208,-62.8804545977846));
#31711=CARTESIAN_POINT('Ctrl Pts',(-32.035229490394,5.20094248181456,-63.9402395323815));
#31712=CARTESIAN_POINT('Ctrl Pts',(-32.0164215840077,5.38318470466738,-64.5381662417493));
#31713=CARTESIAN_POINT('Ctrl Pts',(-32.0050248580873,5.51257267172476,-64.9372802738423));
#31714=CARTESIAN_POINT('Ctrl Pts',(-31.9977169116196,5.60101109084162,-65.2034253818815));
#31715=CARTESIAN_POINT('Ctrl Pts',(-31.990820420896,5.69286410115348,-65.4696998065714));
#31716=CARTESIAN_POINT('Ctrl Pts',(-31.9851064655405,5.7764135570505,-65.7026587699087));
#31717=CARTESIAN_POINT('Ctrl Pts',(-31.9819272561518,5.82509734658462,-65.8357626083149));
#31718=CARTESIAN_POINT('Ctrl Pts',(-31.9772414758308,5.89908237020845,-66.0354027013822));
#31719=CARTESIAN_POINT('Ctrl Pts',(-31.9735043246712,5.96276395488274,-66.2017138853978));
#31720=CARTESIAN_POINT('Ctrl Pts',(-31.967505526974,6.07113175039066,-66.4771126058172));
#31721=CARTESIAN_POINT('Ctrl Pts',(-31.9620408805721,6.1904845906763,-66.7691393250134));
#31722=CARTESIAN_POINT('Ctrl Pts',(-31.9538882168921,6.43821266169139,-67.3366326463683));
#31723=CARTESIAN_POINT('Ctrl Pts',(-31.9459533165198,6.89814538538485,-68.306149005519));
#31724=CARTESIAN_POINT('Ctrl Pts',(-31.9481839501384,7.88472205125732,-70.1482783297304));
#31725=CARTESIAN_POINT('Ctrl Pts',(-31.961892702002,8.74259077718073,-71.6099794297969));
#31726=CARTESIAN_POINT('Ctrl Pts',(-31.9613594031242,9.30272515454331,-72.6751607545568));
#31727=CARTESIAN_POINT('Ctrl Pts',(-31.9611909682197,9.4379959891971,-72.9319898102899));
#31728=CARTESIAN_POINT('Ctrl Pts',(-31.9609722373197,9.70305345665459,-73.4340042881566));
#31729=CARTESIAN_POINT('Ctrl Pts',(-31.9608149848749,10.037473067343,-74.0653454773225));
#31730=CARTESIAN_POINT('Ctrl Pts',(-31.9607946888063,10.4382175724794,-74.8193049140468));
#31731=CARTESIAN_POINT('Ctrl Pts',(-31.960975349681,11.2413208987991,-76.326711544533));
#31732=CARTESIAN_POINT('Ctrl Pts',(-31.9614077113351,11.9106302089475,-77.578887791324));
#31733=CARTESIAN_POINT('Ctrl Pts',(-31.961425949037,12.8784241477409,-79.3991342446787));
#31734=CARTESIAN_POINT('Ctrl Pts',(-31.9614229449857,13.3157470610903,-80.2216653571697));
#31735=CARTESIAN_POINT('Ctrl Pts',(-31.9614229449857,13.7522686484798,-81.0426430592681));
#31736=CARTESIAN_POINT('Ctrl Pts',(-30.071633215331,-0.00597951180148264,
24.830640601082));
#31737=CARTESIAN_POINT('Ctrl Pts',(-30.0717235578503,-0.00597957100751475,
24.7817614745945));
#31738=CARTESIAN_POINT('Ctrl Pts',(-30.071818306792,-0.00597963374140348,
24.7328834062058));
#31739=CARTESIAN_POINT('Ctrl Pts',(-30.0729372132796,-0.00598033382817053,
24.1822774716252));
#31740=CARTESIAN_POINT('Ctrl Pts',(-30.0737952229211,-0.00598426985520875,
23.1781457908663));
#31741=CARTESIAN_POINT('Ctrl Pts',(-30.075791952375,-0.00599635555943293,
21.1695503823648));
#31742=CARTESIAN_POINT('Ctrl Pts',(-30.0832387269141,-0.00600043596979835,
19.6653947528371));
#31743=CARTESIAN_POINT('Ctrl Pts',(-30.0990299640353,-0.00599207384416433,
18.414343595586));
#31744=CARTESIAN_POINT('Ctrl Pts',(-30.1066040175471,-0.00598923956017259,
17.91153802072));
#31745=CARTESIAN_POINT('Ctrl Pts',(-30.1256246862676,-0.00598378310477602,
16.9075565358832));
#31746=CARTESIAN_POINT('Ctrl Pts',(-30.1664223909486,-0.00597099758907751,
15.1537482643775));
#31747=CARTESIAN_POINT('Ctrl Pts',(-30.2051735404777,-0.00593914521947482,
13.6519695231452));
#31748=CARTESIAN_POINT('Ctrl Pts',(-30.2294490691694,-0.00588682107155954,
12.3974438775068));
#31749=CARTESIAN_POINT('Ctrl Pts',(-30.2393714334099,-0.00586177248898783,
11.8964689449408));
#31750=CARTESIAN_POINT('Ctrl Pts',(-30.2595955046103,-0.00579832815387727,
10.8945948339458));
#31751=CARTESIAN_POINT('Ctrl Pts',(-30.2945883665757,-0.00566357321014015,
9.14102577198835));
#31752=CARTESIAN_POINT('Ctrl Pts',(-30.3191303455414,-0.00554193805532452,
7.63581837867654));
#31753=CARTESIAN_POINT('Ctrl Pts',(-30.3300222173341,-0.00548627568986584,
6.50490508050203));
#31754=CARTESIAN_POINT('Ctrl Pts',(-30.3322859039162,-0.00546883603165987,
6.25461090169528));
#31755=CARTESIAN_POINT('Ctrl Pts',(-30.3362571088473,-0.00541696448505553,
5.75342693978769));
#31756=CARTESIAN_POINT('Ctrl Pts',(-30.3417982210222,-0.00529187093641845,
4.87493705883473));
#31757=CARTESIAN_POINT('Ctrl Pts',(-30.3476306312681,-0.00499582274034348,
3.11475253958408));
#31758=CARTESIAN_POINT('Ctrl Pts',(-30.3450141067293,-0.00495422222763471,
1.60853806549901));
#31759=CARTESIAN_POINT('Ctrl Pts',(-30.3408229503568,-0.00531572945932111,
0.54960980273059));
#31760=CARTESIAN_POINT('Ctrl Pts',(-30.3402731096133,-0.00536321355987347,
0.423522389547206));
#31761=CARTESIAN_POINT('Ctrl Pts',(-30.3389860512078,-0.00547324323998226,
0.171520488298055));
#31762=CARTESIAN_POINT('Ctrl Pts',(-30.3362646548094,-0.00570340570257375,
-0.269002060186466));
#31763=CARTESIAN_POINT('Ctrl Pts',(-30.3311870586109,-0.00612312604494034,
-0.897120357819737));
#31764=CARTESIAN_POINT('Ctrl Pts',(-30.323628029892,-0.00673069550680428,
-1.64939756698134));
#31765=CARTESIAN_POINT('Ctrl Pts',(-30.3122283222796,-0.00761099476841721,
-2.6510987622667));
#31766=CARTESIAN_POINT('Ctrl Pts',(-30.2966115981415,-0.00873495975655074,
-3.901868850698));
#31767=CARTESIAN_POINT('Ctrl Pts',(-30.2851276194664,-0.00940831283083989,
-4.90349257029006));
#31768=CARTESIAN_POINT('Ctrl Pts',(-30.2790097090084,-0.00968935407965794,
-5.53063466061613));
#31769=CARTESIAN_POINT('Ctrl Pts',(-30.2765467626583,-0.00981889465309108,
-5.78128773220245));
#31770=CARTESIAN_POINT('Ctrl Pts',(-30.2715829076617,-0.0101295382798206,
-6.28319987592385));
#31771=CARTESIAN_POINT('Ctrl Pts',(-30.2628332180127,-0.0107668890000689,
-7.16221259468513));
#31772=CARTESIAN_POINT('Ctrl Pts',(-30.250371375551,-0.0117035847530645,
-8.4192279934331));
#31773=CARTESIAN_POINT('Ctrl Pts',(-30.238509689104,-0.0120489224396454,
-9.67503048875515));
#31774=CARTESIAN_POINT('Ctrl Pts',(-30.2308111114464,-0.0116521148942716,
-10.5520356855271));
#31775=CARTESIAN_POINT('Ctrl Pts',(-30.2266269145913,-0.0111957267883302,
-11.0523825887198));
#31776=CARTESIAN_POINT('Ctrl Pts',(-30.2246146128345,-0.0108829124011361,
-11.302251951277));
#31777=CARTESIAN_POINT('Ctrl Pts',(-30.2231309221615,-0.0106128757297351,
-11.4903272187712));
#31778=CARTESIAN_POINT('Ctrl Pts',(-30.2221305481449,-0.0104027620643398,
-11.6171410305863));
#31779=CARTESIAN_POINT('Ctrl Pts',(-30.2201215864471,-0.00987262369023837,
-11.8701276993885));
#31780=CARTESIAN_POINT('Ctrl Pts',(-30.2165957861575,-0.00868010383560238,
-12.3120640957198));
#31781=CARTESIAN_POINT('Ctrl Pts',(-30.2075713677146,-0.00448774131343062,
-13.4440946831459));
#31782=CARTESIAN_POINT('Ctrl Pts',(-30.198231970908,0.00214994989502799,
-14.6923215132386));
#31783=CARTESIAN_POINT('Ctrl Pts',(-30.1911141964365,0.00666814874968618,
-15.9396992247391));
#31784=CARTESIAN_POINT('Ctrl Pts',(-30.1882525322469,0.00806802357273801,
-16.5639410441624));
#31785=CARTESIAN_POINT('Ctrl Pts',(-30.1864389162173,0.00844614510224558,
-17.0641007737644));
#31786=CARTESIAN_POINT('Ctrl Pts',(-30.1857067562827,0.00835852581970067,
-17.314498665145));
#31787=CARTESIAN_POINT('Ctrl Pts',(-30.1852277504504,0.00817254577115206,
-17.5017086410094));
#31788=CARTESIAN_POINT('Ctrl Pts',(-30.1848863847523,0.00808121126398812,
-17.6268680840601));
#31789=CARTESIAN_POINT('Ctrl Pts',(-30.1841191343115,0.00792206787407538,
-17.8763295177763));
#31790=CARTESIAN_POINT('Ctrl Pts',(-30.1832483101601,0.00781028158237286,
-18.1260366256064));
#31791=CARTESIAN_POINT('Ctrl Pts',(-30.1823129235598,0.0076824914715805,
-18.3755346530741));
#31792=CARTESIAN_POINT('Ctrl Pts',(-30.1817116725309,0.0075943715824794,
-18.5314870098462));
#31793=CARTESIAN_POINT('Ctrl Pts',(-30.1812257724091,0.00751113785243645,
-18.6562250235203));
#31794=CARTESIAN_POINT('Ctrl Pts',(-30.1807390870507,0.00741801411575103,
-18.7809607744239));
#31795=CARTESIAN_POINT('Ctrl Pts',(-30.1794008187061,0.00713188016881434,
-19.1239465463915));
#31796=CARTESIAN_POINT('Ctrl Pts',(-30.1773269821708,0.00634650351198699,
-19.6850783141798));
#31797=CARTESIAN_POINT('Ctrl Pts',(-30.1749159485127,0.00345073637503823,
-20.6824072644305));
#31798=CARTESIAN_POINT('Ctrl Pts',(-30.1765408003496,-0.00429941117768114,
-21.9292244997599));
#31799=CARTESIAN_POINT('Ctrl Pts',(-30.1863638355369,-0.0164890122786689,
-22.9271492452985));
#31800=CARTESIAN_POINT('Ctrl Pts',(-30.1960969485234,-0.0266514272288744,
-23.5490862532691));
#31801=CARTESIAN_POINT('Ctrl Pts',(-30.2003709868961,-0.0311728989940625,
-23.7916452788537));
#31802=CARTESIAN_POINT('Ctrl Pts',(-30.2102787176068,-0.0421759399504831,
-24.2814720313785));
#31803=CARTESIAN_POINT('Ctrl Pts',(-30.2308081746281,-0.0658145899230264,
-25.1435534007399));
#31804=CARTESIAN_POINT('Ctrl Pts',(-30.2665379126669,-0.10845369408875,
-26.3915697905687));
#31805=CARTESIAN_POINT('Ctrl Pts',(-30.3138158155059,-0.160647057996072,
-27.910620294727));
#31806=CARTESIAN_POINT('Ctrl Pts',(-30.3444695979264,-0.185350408131475,
-28.9361950965051));
#31807=CARTESIAN_POINT('Ctrl Pts',(-30.3603670215602,-0.19305099486998,
-29.5158505234813));
#31808=CARTESIAN_POINT('Ctrl Pts',(-30.3638764419697,-0.19467795492099,
-29.6412874995611));
#31809=CARTESIAN_POINT('Ctrl Pts',(-30.370841372724,-0.197795903543105,
-29.8942199006252));
#31810=CARTESIAN_POINT('Ctrl Pts',(-30.3828772641937,-0.202787979986712,
-30.3362471315004));
#31811=CARTESIAN_POINT('Ctrl Pts',(-30.4065867576155,-0.210771558043477,
-31.2223969914582));
#31812=CARTESIAN_POINT('Ctrl Pts',(-30.4336147741352,-0.214394541709777,
-32.2371582827311));
#31813=CARTESIAN_POINT('Ctrl Pts',(-30.4623143224833,-0.210608117314953,
-33.2535256868337));
#31814=CARTESIAN_POINT('Ctrl Pts',(-30.4850901250171,-0.203586469340701,
-34.0161657514148));
#31815=CARTESIAN_POINT('Ctrl Pts',(-30.509434012464,-0.191909535416984,
-34.7788584001386));
#31816=CARTESIAN_POINT('Ctrl Pts',(-30.527000089848,-0.180699245887847,
-35.2871635656252));
#31817=CARTESIAN_POINT('Ctrl Pts',(-30.5408206753329,-0.170838943841918,
-35.6692991188219));
#31818=CARTESIAN_POINT('Ctrl Pts',(-30.5504135271421,-0.163762007732125,
-35.9248598303208));
#31819=CARTESIAN_POINT('Ctrl Pts',(-30.5707746738688,-0.147753019969481,
-36.4352385447715));
#31820=CARTESIAN_POINT('Ctrl Pts',(-30.6089400303616,-0.115224998830483,
-37.3259440140739));
#31821=CARTESIAN_POINT('Ctrl Pts',(-30.6919117001604,-0.0327245065930569,
-39.1007929179948));
#31822=CARTESIAN_POINT('Ctrl Pts',(-30.7614648092647,0.0618686371559721,
-40.6170327393275));
#31823=CARTESIAN_POINT('Ctrl Pts',(-30.8002466391313,0.139773646463282,
-41.7574484740374));
#31824=CARTESIAN_POINT('Ctrl Pts',(-30.8088584930596,0.155056003248883,
-41.9933086116199));
#31825=CARTESIAN_POINT('Ctrl Pts',(-30.8212074427548,0.176328014535857,
-42.3598877698462));
#31826=CARTESIAN_POINT('Ctrl Pts',(-30.8331286126518,0.195988082731291,
-42.7278573057299));
#31827=CARTESIAN_POINT('Ctrl Pts',(-30.8483932090505,0.221309159407272,
-43.2258448569499));
#31828=CARTESIAN_POINT('Ctrl Pts',(-30.8663204058983,0.252903186846109,
-43.858221607421));
#31829=CARTESIAN_POINT('Ctrl Pts',(-30.8858735298339,0.296914557133909,
-44.6336920117819));
#31830=CARTESIAN_POINT('Ctrl Pts',(-30.900358069208,0.344014155448641,-45.2926442163476));
#31831=CARTESIAN_POINT('Ctrl Pts',(-30.9106122658943,0.391419190964656,
-45.8272055125904));
#31832=CARTESIAN_POINT('Ctrl Pts',(-30.9176059406292,0.432669988209861,
-46.2316555240505));
#31833=CARTESIAN_POINT('Ctrl Pts',(-30.9238322302709,0.480506653593239,
-46.6395184948446));
#31834=CARTESIAN_POINT('Ctrl Pts',(-30.930979550014,0.554279800503014,-47.1876716982823));
#31835=CARTESIAN_POINT('Ctrl Pts',(-30.9350040618108,0.622153380577239,
-47.603401841639));
#31836=CARTESIAN_POINT('Ctrl Pts',(-30.937853668355,0.700470061956545,-48.0229458365958));
#31837=CARTESIAN_POINT('Ctrl Pts',(-30.9398837417028,0.757623241431886,
-48.3078419742728));
#31838=CARTESIAN_POINT('Ctrl Pts',(-30.9447094693403,0.884257780076132,
-48.8663016682787));
#31839=CARTESIAN_POINT('Ctrl Pts',(-30.9540884552519,1.13479418413515,-49.8247060904745));
#31840=CARTESIAN_POINT('Ctrl Pts',(-30.9658562738545,1.54639350434677,-51.1377722660007));
#31841=CARTESIAN_POINT('Ctrl Pts',(-30.9672655462429,2.04700692304314,-52.6362661460573));
#31842=CARTESIAN_POINT('Ctrl Pts',(-30.9542947585683,2.33739849305094,-53.586533226448));
#31843=CARTESIAN_POINT('Ctrl Pts',(-30.9382889729449,2.49141968435564,-54.1662912690709));
#31844=CARTESIAN_POINT('Ctrl Pts',(-30.9291225129865,2.55517267883511,-54.4141505897421));
#31845=CARTESIAN_POINT('Ctrl Pts',(-30.9068388800674,2.67658080355494,-54.9058577640804));
#31846=CARTESIAN_POINT('Ctrl Pts',(-30.8560495734567,2.88053387167694,-55.7782833871445));
#31847=CARTESIAN_POINT('Ctrl Pts',(-30.718141123549,3.26645565618861,-57.5487625857468));
#31848=CARTESIAN_POINT('Ctrl Pts',(-30.5680043924138,3.6255385292795,-59.1042781383112));
#31849=CARTESIAN_POINT('Ctrl Pts',(-30.4891640217922,3.94202721780659,-60.2106447919612));
#31850=CARTESIAN_POINT('Ctrl Pts',(-30.4801173902694,3.97803208143601,-60.3371690260636));
#31851=CARTESIAN_POINT('Ctrl Pts',(-30.461387852414,4.05171834984927,-60.5951852873439));
#31852=CARTESIAN_POINT('Ctrl Pts',(-30.4280986510233,4.18090295995364,-61.0456191802627));
#31853=CARTESIAN_POINT('Ctrl Pts',(-30.3593934569128,4.44492181141008,-61.952351166067));
#31854=CARTESIAN_POINT('Ctrl Pts',(-30.2799851930437,4.76470369438984,-62.9948419468024));
#31855=CARTESIAN_POINT('Ctrl Pts',(-30.2076940068515,5.11416131601914,-64.0402606257236));
#31856=CARTESIAN_POINT('Ctrl Pts',(-30.1712404393034,5.32354239948677,-64.6282546742671));
#31857=CARTESIAN_POINT('Ctrl Pts',(-30.1492726927023,5.46923721772613,-65.0199525053915));
#31858=CARTESIAN_POINT('Ctrl Pts',(-30.1352898838634,5.56802668462955,-65.2809631375061));
#31859=CARTESIAN_POINT('Ctrl Pts',(-30.1223429458612,5.66942002501773,-65.5418067682793));
#31860=CARTESIAN_POINT('Ctrl Pts',(-30.1120234596837,5.76050010640036,-65.7697948671604));
#31861=CARTESIAN_POINT('Ctrl Pts',(-30.1064253922327,5.81324289372803,-65.8999984503125));
#31862=CARTESIAN_POINT('Ctrl Pts',(-30.0983336314726,5.89306380492265,-66.0952289388947));
#31863=CARTESIAN_POINT('Ctrl Pts',(-30.0922333964975,5.9610784662157,-66.2577492366815));
#31864=CARTESIAN_POINT('Ctrl Pts',(-30.0830549482081,6.07581543646423,-66.5266981578281));
#31865=CARTESIAN_POINT('Ctrl Pts',(-30.0746943339823,6.19979525758211,-66.8097215279348));
#31866=CARTESIAN_POINT('Ctrl Pts',(-30.0620885458429,6.45378746289753,-67.3629354741228));
#31867=CARTESIAN_POINT('Ctrl Pts',(-30.0494866581976,6.91657589646975,-68.3117542359668));
#31868=CARTESIAN_POINT('Ctrl Pts',(-30.0519299035184,7.88784277604413,-70.1317633075454));
#31869=CARTESIAN_POINT('Ctrl Pts',(-30.0724797044386,8.7274639830299,-71.5972679336727));
#31870=CARTESIAN_POINT('Ctrl Pts',(-30.0710020759233,9.29689859995957,-72.6777777073672));
#31871=CARTESIAN_POINT('Ctrl Pts',(-30.0707113821031,9.43171519037961,-72.9332896071135));
#31872=CARTESIAN_POINT('Ctrl Pts',(-30.070282603693,9.69719653373554,-73.4354404713998));
#31873=CARTESIAN_POINT('Ctrl Pts',(-30.0699952412353,10.0314082669893,-74.0659143981115));
#31874=CARTESIAN_POINT('Ctrl Pts',(-30.0699631027953,10.4320333495277,-74.8195879198025));
#31875=CARTESIAN_POINT('Ctrl Pts',(-30.0703311662541,11.2344964301764,-76.32633032144));
#31876=CARTESIAN_POINT('Ctrl Pts',(-30.0711438759096,11.9032275320862,-77.5785599567108));
#31877=CARTESIAN_POINT('Ctrl Pts',(-30.0711381425972,12.8714052347748,-79.3994559074687));
#31878=CARTESIAN_POINT('Ctrl Pts',(-30.0711343370146,13.3085843007755,-80.2216793738818));
#31879=CARTESIAN_POINT('Ctrl Pts',(-30.0711343370145,13.745105888165,-81.0426570759801));
#31880=CARTESIAN_POINT('Ctrl Pts',(-28.1863005461827,-0.00460604167494977,
24.8306401042851));
#31881=CARTESIAN_POINT('Ctrl Pts',(-28.1863847775742,-0.00460633545135409,
24.7817609620066));
#31882=CARTESIAN_POINT('Ctrl Pts',(-28.1864731178034,-0.00460664429642971,
24.7328828792526));
#31883=CARTESIAN_POINT('Ctrl Pts',(-28.1875163330769,-0.0046102481476268,
24.1822767102568));
#31884=CARTESIAN_POINT('Ctrl Pts',(-28.1883126217779,-0.00461560258461171,
23.1781432543363));
#31885=CARTESIAN_POINT('Ctrl Pts',(-28.1901636158954,-0.0046304985039466,
21.1695480668301));
#31886=CARTESIAN_POINT('Ctrl Pts',(-28.1971064762245,-0.00465391042639694,
19.6653941983213));
#31887=CARTESIAN_POINT('Ctrl Pts',(-28.2118477398425,-0.00469056804568364,
18.4143448435113));
#31888=CARTESIAN_POINT('Ctrl Pts',(-28.2189167353326,-0.00470939894775233,
17.9115392779163));
#31889=CARTESIAN_POINT('Ctrl Pts',(-28.2366663011845,-0.0047586054950456,
16.9075569728651));
#31890=CARTESIAN_POINT('Ctrl Pts',(-28.2747390509576,-0.00486360912988234,
15.1537447443413));
#31891=CARTESIAN_POINT('Ctrl Pts',(-28.3109227936906,-0.00494472184720988,
13.6519622575988));
#31892=CARTESIAN_POINT('Ctrl Pts',(-28.3336317464906,-0.0049640640775537,
12.3974379027123));
#31893=CARTESIAN_POINT('Ctrl Pts',(-28.3429188492018,-0.00496852004088664,
11.896463348646));
#31894=CARTESIAN_POINT('Ctrl Pts',(-28.3618627525136,-0.00496581361296356,
10.8945900324065));
#31895=CARTESIAN_POINT('Ctrl Pts',(-28.3946724405316,-0.00493736126333316,
9.14102108292138));
#31896=CARTESIAN_POINT('Ctrl Pts',(-28.4177082765907,-0.00489031242012178,
7.63581293756268));
#31897=CARTESIAN_POINT('Ctrl Pts',(-28.427936275759,-0.00486645967896916,
6.50489137702784));
#31898=CARTESIAN_POINT('Ctrl Pts',(-28.430076222178,-0.00484956678344242,
6.25451917695903));
#31899=CARTESIAN_POINT('Ctrl Pts',(-28.4338784345938,-0.00477752765288108,
5.75325079164063));
#31900=CARTESIAN_POINT('Ctrl Pts',(-28.4392992625228,-0.00457292789812331,
4.87465469053201));
#31901=CARTESIAN_POINT('Ctrl Pts',(-28.4453694619222,-0.00403931884329462,
3.11453429456818));
#31902=CARTESIAN_POINT('Ctrl Pts',(-28.4429563699568,-0.00398414553418337,
1.60880108702352));
#31903=CARTESIAN_POINT('Ctrl Pts',(-28.4381704350487,-0.00474055572035643,
0.550446199667754));
#31904=CARTESIAN_POINT('Ctrl Pts',(-28.4375445621273,-0.00483960300428552,
0.424461121558914));
#31905=CARTESIAN_POINT('Ctrl Pts',(-28.4360822446314,-0.0050688520581819,
0.17263186514994));
#31906=CARTESIAN_POINT('Ctrl Pts',(-28.432999126287,-0.00554756712592698,
-0.267607748437768));
#31907=CARTESIAN_POINT('Ctrl Pts',(-28.4272652661807,-0.00641984888925787,
-0.89541244968379));
#31908=CARTESIAN_POINT('Ctrl Pts',(-28.4187863090284,-0.0076797759635048,
-1.64744927029274));
#31909=CARTESIAN_POINT('Ctrl Pts',(-28.406065940695,-0.00950538541273805,
-2.64901595059585));
#31910=CARTESIAN_POINT('Ctrl Pts',(-28.3888401377251,-0.011829617360604,
-3.89997598939455));
#31911=CARTESIAN_POINT('Ctrl Pts',(-28.376493002255,-0.0131975675662079,
-4.90214870528169));
#31912=CARTESIAN_POINT('Ctrl Pts',(-28.3701063743469,-0.0137396685467702,
-5.52975857296791));
#31913=CARTESIAN_POINT('Ctrl Pts',(-28.3675242803865,-0.0139619450347725,
-5.78051104302905));
#31914=CARTESIAN_POINT('Ctrl Pts',(-28.3622872451714,-0.0144149998525911,
-6.2826421124058));
#31915=CARTESIAN_POINT('Ctrl Pts',(-28.3530121884009,-0.0152005766043735,
-7.16194751912559));
#31916=CARTESIAN_POINT('Ctrl Pts',(-28.3398977716336,-0.0161385482469937,
-8.41920740101793));
#31917=CARTESIAN_POINT('Ctrl Pts',(-28.3281935808401,-0.0163896778099333,
-9.67501169157448));
#31918=CARTESIAN_POINT('Ctrl Pts',(-28.3213834537875,-0.0159739830935321,
-10.5519002670555));
#31919=CARTESIAN_POINT('Ctrl Pts',(-28.3179797696801,-0.01553293702959,
-11.0521448672915));
#31920=CARTESIAN_POINT('Ctrl Pts',(-28.3164549382297,-0.0152391975934058,
-11.3019518748116));
#31921=CARTESIAN_POINT('Ctrl Pts',(-28.3153795119772,-0.0149880839074049,
-11.489973567269));
#31922=CARTESIAN_POINT('Ctrl Pts',(-28.314685095118,-0.014792879670191,
-11.6166790902712));
#31923=CARTESIAN_POINT('Ctrl Pts',(-28.3134047585379,-0.0143102633951334,
-11.8695121594015));
#31924=CARTESIAN_POINT('Ctrl Pts',(-28.3114336217475,-0.0132401939293641,
-12.311206357399));
#31925=CARTESIAN_POINT('Ctrl Pts',(-28.3076038610431,-0.00951646921472725,
-13.4428824026115));
#31926=CARTESIAN_POINT('Ctrl Pts',(-28.3061586258559,-0.00364668722937351,
-14.691316859968));
#31927=CARTESIAN_POINT('Ctrl Pts',(-28.3050443425316,0.000568090034001496,
-15.939616939592));
#31928=CARTESIAN_POINT('Ctrl Pts',(-28.3043418144241,0.00198931723314658,
-16.5645176054236));
#31929=CARTESIAN_POINT('Ctrl Pts',(-28.3035947968661,0.00254663777454252,
-17.0653489248785));
#31930=CARTESIAN_POINT('Ctrl Pts',(-28.3031304898045,0.00260742789917509,
-17.3161305034899));
#31931=CARTESIAN_POINT('Ctrl Pts',(-28.3027467966274,0.00256088562709459,
-17.5036502999823));
#31932=CARTESIAN_POINT('Ctrl Pts',(-28.3025155137543,0.00254198055265861,
-17.6290856683236));
#31933=CARTESIAN_POINT('Ctrl Pts',(-28.3021374514763,0.00259174819776393,
-17.8790380467737));
#31934=CARTESIAN_POINT('Ctrl Pts',(-28.3018630375286,0.00274320347158438,
-18.1292232356557));
#31935=CARTESIAN_POINT('Ctrl Pts',(-28.3016839981496,0.00296417225329587,
-18.3791633923168));
#31936=CARTESIAN_POINT('Ctrl Pts',(-28.3016017365269,0.00312302677002713,
-18.5353803170869));
#31937=CARTESIAN_POINT('Ctrl Pts',(-28.3015528172302,0.00325835718774737,
-18.6603210609758));
#31938=CARTESIAN_POINT('Ctrl Pts',(-28.301513346424,0.00339789381416274,
-18.785253407746));
#31939=CARTESIAN_POINT('Ctrl Pts',(-28.3014335207091,0.00378777524423548,
-19.1287568608658));
#31940=CARTESIAN_POINT('Ctrl Pts',(-28.3014303865288,0.00441569054555669,
-19.6905720048103));
#31941=CARTESIAN_POINT('Ctrl Pts',(-28.3012214735957,0.00463831851483729,
-20.6885682611972));
#31942=CARTESIAN_POINT('Ctrl Pts',(-28.2993755605549,0.00165391259089476,
-21.9346838395311));
#31943=CARTESIAN_POINT('Ctrl Pts',(-28.2941297489489,-0.00805261113508078,
-22.9304888622303));
#31944=CARTESIAN_POINT('Ctrl Pts',(-28.2891626298632,-0.0175098653397202,
-23.5509560293143));
#31945=CARTESIAN_POINT('Ctrl Pts',(-28.2868822650861,-0.0217358296645737,
-23.7941797621322));
#31946=CARTESIAN_POINT('Ctrl Pts',(-28.2813074727843,-0.032077390509107,
-24.2844080322069));
#31947=CARTESIAN_POINT('Ctrl Pts',(-28.2693454732741,-0.0544057891600798,
-25.147158667633));
#31948=CARTESIAN_POINT('Ctrl Pts',(-28.2486784083908,-0.0942889514449492,
-26.3948278722657));
#31949=CARTESIAN_POINT('Ctrl Pts',(-28.2257077673537,-0.14255782676672,
-27.9110090292924));
#31950=CARTESIAN_POINT('Ctrl Pts',(-28.216385187724,-0.167029701575379,
-28.9316551969023));
#31951=CARTESIAN_POINT('Ctrl Pts',(-28.2142667044121,-0.176558653404427,
-29.5076376535198));
#31952=CARTESIAN_POINT('Ctrl Pts',(-28.2138126885783,-0.178615435337877,
-29.633065948268));
#31953=CARTESIAN_POINT('Ctrl Pts',(-28.2129475846591,-0.182637689761345,
-29.8854739383231));
#31954=CARTESIAN_POINT('Ctrl Pts',(-28.2115838536727,-0.189353462795671,
-30.3266897748748));
#31955=CARTESIAN_POINT('Ctrl Pts',(-28.2096267231321,-0.201505456968724,
-31.2105582168276));
#31956=CARTESIAN_POINT('Ctrl Pts',(-28.2100031363158,-0.212082202476106,
-32.2217394016259));
#31957=CARTESIAN_POINT('Ctrl Pts',(-28.214681940452,-0.218758095344881,
-33.2334878724097));
#31958=CARTESIAN_POINT('Ctrl Pts',(-28.2207706234283,-0.221641983732676,
-33.9921974180832));
#31959=CARTESIAN_POINT('Ctrl Pts',(-28.2298770732745,-0.222163231633312,
-34.7504699343643));
#31960=CARTESIAN_POINT('Ctrl Pts',(-28.238249225568,-0.220820903106427,
-35.2555188277877));
#31961=CARTESIAN_POINT('Ctrl Pts',(-28.245520562333,-0.219135849961407,
-35.6351015437609));
#31962=CARTESIAN_POINT('Ctrl Pts',(-28.2508731165334,-0.217786895183696,
-35.889230843851));
#31963=CARTESIAN_POINT('Ctrl Pts',(-28.2633058084189,-0.214239235970583,
-36.3967042830002));
#31964=CARTESIAN_POINT('Ctrl Pts',(-28.2891464643115,-0.205729147312358,
-37.2826146212146));
#31965=CARTESIAN_POINT('Ctrl Pts',(-28.3534019588011,-0.180241286852696,
-39.0487948012157));
#31966=CARTESIAN_POINT('Ctrl Pts',(-28.4172498273522,-0.144300921438199,
-40.5588253834969));
#31967=CARTESIAN_POINT('Ctrl Pts',(-28.4564486934885,-0.111653453402085,
-41.6953858046599));
#31968=CARTESIAN_POINT('Ctrl Pts',(-28.4649228404561,-0.105861983781313,
-41.9313674162035));
#31969=CARTESIAN_POINT('Ctrl Pts',(-28.4772841445845,-0.0991681183657871,
-42.2973103574194));
#31970=CARTESIAN_POINT('Ctrl Pts',(-28.4893593522273,-0.0941570899006693,
-42.6645390481917));
#31971=CARTESIAN_POINT('Ctrl Pts',(-28.505203288971,-0.0887045924743431,
-43.1610624503874));
#31972=CARTESIAN_POINT('Ctrl Pts',(-28.5247366850926,-0.0826468713669569,
-43.7910003417678));
#31973=CARTESIAN_POINT('Ctrl Pts',(-28.5484404118947,-0.0709530661363236,
-44.5626348394999));
#31974=CARTESIAN_POINT('Ctrl Pts',(-28.5689764856386,-0.0525654338336199,
-45.2178320678155));
#31975=CARTESIAN_POINT('Ctrl Pts',(-28.5861701425892,-0.0294661635961474,
-45.7492950011563));
#31976=CARTESIAN_POINT('Ctrl Pts',(-28.5995201029825,-0.00712421863073947,
-46.1513607436204));
#31977=CARTESIAN_POINT('Ctrl Pts',(-28.613385212919,0.0210865954295373,
-46.5568519528627));
#31978=CARTESIAN_POINT('Ctrl Pts',(-28.6326148639367,0.0677117422033199,
-47.1019015008582));
#31979=CARTESIAN_POINT('Ctrl Pts',(-28.6479582923095,0.114099562474359,
-47.5154787240077));
#31980=CARTESIAN_POINT('Ctrl Pts',(-28.6639629462404,0.170110982033969,
-47.9327508282799));
#31981=CARTESIAN_POINT('Ctrl Pts',(-28.6760104425626,0.208815074499745,
-48.2040495811931));
#31982=CARTESIAN_POINT('Ctrl Pts',(-28.7034894331993,0.296045118550941,
-48.7479340590624));
#31983=CARTESIAN_POINT('Ctrl Pts',(-28.7587570263741,0.470865910892395,
-49.6895209659119));
#31984=CARTESIAN_POINT('Ctrl Pts',(-28.8456712155738,0.776483402567067,
-51.0114022234942));
#31985=CARTESIAN_POINT('Ctrl Pts',(-28.927339437998,1.19547757616793,-52.5558913273152));
#31986=CARTESIAN_POINT('Ctrl Pts',(-28.9490218947129,1.47956209353257,-53.5617487549242));
#31987=CARTESIAN_POINT('Ctrl Pts',(-28.9473547952781,1.65012798643743,-54.186254485831));
#31988=CARTESIAN_POINT('Ctrl Pts',(-28.9444871311617,1.72175364071754,-54.4480453615726));
#31989=CARTESIAN_POINT('Ctrl Pts',(-28.9341668134448,1.86520562706103,-54.9665377909226));
#31990=CARTESIAN_POINT('Ctrl Pts',(-28.9039504324693,2.12133746067361,-55.877091855804));
#31991=CARTESIAN_POINT('Ctrl Pts',(-28.8061314957623,2.6529879289795,-57.6947502180311));
#31992=CARTESIAN_POINT('Ctrl Pts',(-28.6903443350229,3.15423154962865,-59.2397974222075));
#31993=CARTESIAN_POINT('Ctrl Pts',(-28.6263471470519,3.53403403606696,-60.3184713489117));
#31994=CARTESIAN_POINT('Ctrl Pts',(-28.6183525944514,3.5803669285416,-60.4500322101376));
#31995=CARTESIAN_POINT('Ctrl Pts',(-28.6016837617537,3.67372926736117,-60.7128442372547));
#31996=CARTESIAN_POINT('Ctrl Pts',(-28.5708003187594,3.83905363322346,-61.1727900519157));
#31997=CARTESIAN_POINT('Ctrl Pts',(-28.503394716372,4.1776943041034,-62.0913978688054));
#31998=CARTESIAN_POINT('Ctrl Pts',(-28.4188521456682,4.5846543218748,-63.1356496646742));
#31999=CARTESIAN_POINT('Ctrl Pts',(-28.3388845614405,5.01183715274042,-64.1687182709692));
#32000=CARTESIAN_POINT('Ctrl Pts',(-28.2979803171294,5.25917876202764,-64.7449014612071));
#32001=CARTESIAN_POINT('Ctrl Pts',(-28.2733358642123,5.42676450286561,-65.1266980782478));
#32002=CARTESIAN_POINT('Ctrl Pts',(-28.2576679953265,5.53917211512882,-65.3805903841216));
#32003=CARTESIAN_POINT('Ctrl Pts',(-28.2432271711642,5.65260419490981,-65.6335437356018));
#32004=CARTESIAN_POINT('Ctrl Pts',(-28.2318222335131,5.75266344337316,-65.8539777388884));
#32005=CARTESIAN_POINT('Ctrl Pts',(-28.2256772991046,5.81006471456788,-65.9796823611048));
#32006=CARTESIAN_POINT('Ctrl Pts',(-28.2168428029436,5.89638926812434,-66.167985912538));
#32007=CARTESIAN_POINT('Ctrl Pts',(-28.2102987830632,5.96877716465577,-66.324358053145));
#32008=CARTESIAN_POINT('Ctrl Pts',(-28.2006623951268,6.08925573052596,-66.5826915117347));
#32009=CARTESIAN_POINT('Ctrl Pts',(-28.1918397593507,6.21898802956303,-66.8567837258073));
#32010=CARTESIAN_POINT('Ctrl Pts',(-28.1784070116348,6.48002646242587,-67.3934340007737));
#32011=CARTESIAN_POINT('Ctrl Pts',(-28.1646562164352,6.94658361661508,-68.3190168217354));
#32012=CARTESIAN_POINT('Ctrl Pts',(-28.1663770295904,7.90084850797895,-70.1119324976335));
#32013=CARTESIAN_POINT('Ctrl Pts',(-28.1881081132948,8.71948558422654,-71.582446078205));
#32014=CARTESIAN_POINT('Ctrl Pts',(-28.1863206363366,9.30013791883288,-72.680964220891));
#32015=CARTESIAN_POINT('Ctrl Pts',(-28.1859809829049,9.43444168834478,-72.9348507263182));
#32016=CARTESIAN_POINT('Ctrl Pts',(-28.1854737933729,9.70045760038316,-73.4370577568619));
#32017=CARTESIAN_POINT('Ctrl Pts',(-28.1851399583262,10.034413389861,-74.0664101829464));
#32018=CARTESIAN_POINT('Ctrl Pts',(-28.185104743579,10.4348437144677,-74.8196494289759));
#32019=CARTESIAN_POINT('Ctrl Pts',(-28.1855469585286,11.2363852336376,-76.3254833102637));
#32020=CARTESIAN_POINT('Ctrl Pts',(-28.1865222320035,11.9042541659904,-77.5779156822583));
#32021=CARTESIAN_POINT('Ctrl Pts',(-28.1865189209674,12.8729892730661,-79.399855078337));
#32022=CARTESIAN_POINT('Ctrl Pts',(-28.1865194110349,13.3099555663221,-80.221676071923));
#32023=CARTESIAN_POINT('Ctrl Pts',(-28.1865194110349,13.7464771537116,-81.0426537740213));
#32024=CARTESIAN_POINT('Ctrl Pts',(-26.3067668117876,-0.000538699954624175,
24.8306355267635));
#32025=CARTESIAN_POINT('Ctrl Pts',(-26.3068451876501,-0.000538876189496768,
24.781756239974));
#32026=CARTESIAN_POINT('Ctrl Pts',(-26.306927385946,-0.000539061754406431,
24.7328780109039));
#32027=CARTESIAN_POINT('Ctrl Pts',(-26.3078981083115,-0.000541218695861637,
24.1822701223404));
#32028=CARTESIAN_POINT('Ctrl Pts',(-26.308638797907,-0.000542921187126547,
23.1781339115758));
#32029=CARTESIAN_POINT('Ctrl Pts',(-26.3103596540731,-0.000547510562500565,
21.1695358988917));
#32030=CARTESIAN_POINT('Ctrl Pts',(-26.3168206355383,-0.000561494614877348,
19.6653821365272));
#32031=CARTESIAN_POINT('Ctrl Pts',(-26.3305400639719,-0.000590835905523418,
18.4143333475625));
#32032=CARTESIAN_POINT('Ctrl Pts',(-26.3371183800673,-0.000605254926751675,
17.9115190955673));
#32033=CARTESIAN_POINT('Ctrl Pts',(-26.3536351484472,-0.000641926725106596,
16.9075303164735));
#32034=CARTESIAN_POINT('Ctrl Pts',(-26.3890629920332,-0.000720784918182074,
15.1537172634109));
#32035=CARTESIAN_POINT('Ctrl Pts',(-26.4227431417796,-0.000791449315555003,
13.6519609598852));
#32036=CARTESIAN_POINT('Ctrl Pts',(-26.4438929028652,-0.000829734955752551,
12.3974737776712));
#32037=CARTESIAN_POINT('Ctrl Pts',(-26.4525430650074,-0.00084487329312605,
11.8965144636692));
#32038=CARTESIAN_POINT('Ctrl Pts',(-26.4701923515509,-0.000873398605924195,
10.8946630473504));
#32039=CARTESIAN_POINT('Ctrl Pts',(-26.5007676037454,-0.000918523372976478,
9.14111543813712));
#32040=CARTESIAN_POINT('Ctrl Pts',(-26.5222561422087,-0.000942796547773691,
7.63589175690357));
#32041=CARTESIAN_POINT('Ctrl Pts',(-26.5318021172031,-0.000952582193824432,
6.50494958170678));
#32042=CARTESIAN_POINT('Ctrl Pts',(-26.5338202972566,-0.000947585409883766,
6.25463586694622));
#32043=CARTESIAN_POINT('Ctrl Pts',(-26.5374815994599,-0.000913662062184531,
5.75342822449203));
#32044=CARTESIAN_POINT('Ctrl Pts',(-26.542884293761,-0.000804479291789807,
4.87490869188615));
#32045=CARTESIAN_POINT('Ctrl Pts',(-26.5494687884833,-0.000504712387683716,
3.11473294922618));
#32046=CARTESIAN_POINT('Ctrl Pts',(-26.5472854591206,-0.000478066320458629,
1.60861764398263));
#32047=CARTESIAN_POINT('Ctrl Pts',(-26.5414101923829,-0.000937735640324079,
0.549835984673704));
#32048=CARTESIAN_POINT('Ctrl Pts',(-26.5406416200034,-0.000998055376415954,
0.423780445023005));
#32049=CARTESIAN_POINT('Ctrl Pts',(-26.5388520301281,-0.0011376182369757,
0.171831141482077));
#32050=CARTESIAN_POINT('Ctrl Pts',(-26.5350910798596,-0.00142888191146685,
-0.268602127637444));
#32051=CARTESIAN_POINT('Ctrl Pts',(-26.5281424169917,-0.00195699496613554,
-0.896615216968427));
#32052=CARTESIAN_POINT('Ctrl Pts',(-26.5179253790002,-0.00271609093358323,
-1.64879887106375));
#32053=CARTESIAN_POINT('Ctrl Pts',(-26.5027296125362,-0.00380454918085976,
-2.65042863623411));
#32054=CARTESIAN_POINT('Ctrl Pts',(-26.4824144417945,-0.00516579915528091,
-3.90123622681562));
#32055=CARTESIAN_POINT('Ctrl Pts',(-26.4683792072888,-0.00593730752158881,
-4.90305082619869));
#32056=CARTESIAN_POINT('Ctrl Pts',(-26.4613995433984,-0.00622942189138888,
-5.53038586337433));
#32057=CARTESIAN_POINT('Ctrl Pts',(-26.4586055525338,-0.0063380563385362,
-5.78133473549539));
#32058=CARTESIAN_POINT('Ctrl Pts',(-26.4530433222871,-0.00652495285022699,
-6.28361018998542));
#32059=CARTESIAN_POINT('Ctrl Pts',(-26.4434403582543,-0.00677386241630181,
-7.16308898027664));
#32060=CARTESIAN_POINT('Ctrl Pts',(-26.4304432957718,-0.0069274983770433,
-8.42004337635663));
#32061=CARTESIAN_POINT('Ctrl Pts',(-26.419323612753,-0.00686441290470747,
-9.67491166013457));
#32062=CARTESIAN_POINT('Ctrl Pts',(-26.4130042716163,-0.0067357043217891,
-10.5507828150709));
#32063=CARTESIAN_POINT('Ctrl Pts',(-26.4098829159842,-0.00664094240293327,
-11.0503441710192));
#32064=CARTESIAN_POINT('Ctrl Pts',(-26.4084973739244,-0.0065873715842191,
-11.2997774800692));
#32065=CARTESIAN_POINT('Ctrl Pts',(-26.4075238006317,-0.00654481180717828,
-11.4874960340828));
#32066=CARTESIAN_POINT('Ctrl Pts',(-26.4068990555078,-0.0065126789462424,
-11.6137055904411));
#32067=CARTESIAN_POINT('Ctrl Pts',(-26.4057636148961,-0.00643259146762249,
-11.8657795877875));
#32068=CARTESIAN_POINT('Ctrl Pts',(-26.4040634719408,-0.00625453645064599,
-12.3062201720521));
#32069=CARTESIAN_POINT('Ctrl Pts',(-26.4010267927984,-0.00563307175450961,
-13.4355782116524));
#32070=CARTESIAN_POINT('Ctrl Pts',(-26.4007771402918,-0.00460249839055765,
-14.6839857455774));
#32071=CARTESIAN_POINT('Ctrl Pts',(-26.4011342734351,-0.00376334242939199,
-15.9348201084843));
#32072=CARTESIAN_POINT('Ctrl Pts',(-26.4012564354109,-0.00344118371370728,
-16.5615920969361));
#32073=CARTESIAN_POINT('Ctrl Pts',(-26.4011953559784,-0.00327847224339482,
-17.0642625997816));
#32074=CARTESIAN_POINT('Ctrl Pts',(-26.4010889745752,-0.00323185749929953,
-17.3160885549663));
#32075=CARTESIAN_POINT('Ctrl Pts',(-26.4009744528728,-0.00321370813660455,
-17.5043944183102));
#32076=CARTESIAN_POINT('Ctrl Pts',(-26.4009502260798,-0.00319047410131549,
-17.6291798260985));
#32077=CARTESIAN_POINT('Ctrl Pts',(-26.401090732026,-0.00313045400635487,
-17.8786393400492));
#32078=CARTESIAN_POINT('Ctrl Pts',(-26.4014814965549,-0.00304331594204274,
-18.1282409226063));
#32079=CARTESIAN_POINT('Ctrl Pts',(-26.4020734283397,-0.00294946836358305,
-18.3778951727794));
#32080=CARTESIAN_POINT('Ctrl Pts',(-26.4025133950277,-0.00288718042293722,
-18.5339729656228));
#32081=CARTESIAN_POINT('Ctrl Pts',(-26.4029014443056,-0.00283774620801123,
-18.6588550278531));
#32082=CARTESIAN_POINT('Ctrl Pts',(-26.4033113524095,-0.00278891479687412,
-18.7837532047067));
#32083=CARTESIAN_POINT('Ctrl Pts',(-26.4045102812651,-0.00265070793138668,
-19.1272863938833));
#32084=CARTESIAN_POINT('Ctrl Pts',(-26.4068039814181,-0.00246061209984525,
-19.6897931196873));
#32085=CARTESIAN_POINT('Ctrl Pts',(-26.4105766396482,-0.00235074624862679,
-20.6909483135089));
#32086=CARTESIAN_POINT('Ctrl Pts',(-26.4127186181016,-0.0030500036225254,
-21.944804180922));
#32087=CARTESIAN_POINT('Ctrl Pts',(-26.4066977217584,-0.00478894319038026,
-22.9508245281247));
#32088=CARTESIAN_POINT('Ctrl Pts',(-26.3990835556788,-0.0064034352788766,
-23.5787686036408));
#32089=CARTESIAN_POINT('Ctrl Pts',(-26.3955759960211,-0.00713908522416187,
-23.8270180069377));
#32090=CARTESIAN_POINT('Ctrl Pts',(-26.3867350909327,-0.0088416464694765,
-24.3247318868074));
#32091=CARTESIAN_POINT('Ctrl Pts',(-26.3671611553572,-0.0123384937718505,
-25.1980292444309));
#32092=CARTESIAN_POINT('Ctrl Pts',(-26.3309962257493,-0.0179683153941739,
-26.451199300417));
#32093=CARTESIAN_POINT('Ctrl Pts',(-26.286983275886,-0.0241164221772839,
-27.9603145633623));
#32094=CARTESIAN_POINT('Ctrl Pts',(-26.2648364528597,-0.0269527012872554,
-28.9674675109934));
#32095=CARTESIAN_POINT('Ctrl Pts',(-26.2565759171718,-0.0281304007585666,
-29.5336179009703));
#32096=CARTESIAN_POINT('Ctrl Pts',(-26.2547552462034,-0.0284027765599454,
-29.6589431501243));
#32097=CARTESIAN_POINT('Ctrl Pts',(-26.2511601601551,-0.0289274610454118,
-29.9099370325545));
#32098=CARTESIAN_POINT('Ctrl Pts',(-26.2450037793416,-0.0298100005573521,
-30.3491931563502));
#32099=CARTESIAN_POINT('Ctrl Pts',(-26.23347324007,-0.031427036391679,-31.2283707605503));
#32100=CARTESIAN_POINT('Ctrl Pts',(-26.2229714198081,-0.0329540249543629,
-32.2337271230666));
#32101=CARTESIAN_POINT('Ctrl Pts',(-26.2170313145426,-0.0341652924499194,
-33.2388001712352));
#32102=CARTESIAN_POINT('Ctrl Pts',(-26.2153206044666,-0.0349193705859608,
-33.9921653671943));
#32103=CARTESIAN_POINT('Ctrl Pts',(-26.2167440409269,-0.0354991514690913,
-34.744715353211));
#32104=CARTESIAN_POINT('Ctrl Pts',(-26.2201074284133,-0.0357706548368423,
-35.245701175117));
#32105=CARTESIAN_POINT('Ctrl Pts',(-26.2236621317938,-0.0359215423046611,
-35.6221289590457));
#32106=CARTESIAN_POINT('Ctrl Pts',(-26.226523386943,-0.036036968596862,
-35.874004709527));
#32107=CARTESIAN_POINT('Ctrl Pts',(-26.2339799499197,-0.0362914675196322,
-36.3772691388551));
#32108=CARTESIAN_POINT('Ctrl Pts',(-26.2510933692841,-0.0368106569182081,
-37.2561994063118));
#32109=CARTESIAN_POINT('Ctrl Pts',(-26.2977812793891,-0.0373645488137689,
-39.0104730415285));
#32110=CARTESIAN_POINT('Ctrl Pts',(-26.346463654717,-0.035831460880283,
-40.5130518138167));
#32111=CARTESIAN_POINT('Ctrl Pts',(-26.3743845800949,-0.0318724213306068,
-41.6455984565211));
#32112=CARTESIAN_POINT('Ctrl Pts',(-26.3803646184719,-0.0319919850056345,
-41.8821563107312));
#32113=CARTESIAN_POINT('Ctrl Pts',(-26.3888990724742,-0.0344735418328895,
-42.2477051044875));
#32114=CARTESIAN_POINT('Ctrl Pts',(-26.3970924896663,-0.0387561876770233,
-42.6143309685538));
#32115=CARTESIAN_POINT('Ctrl Pts',(-26.4077089334092,-0.0461283281546971,
-43.1092311587212));
#32116=CARTESIAN_POINT('Ctrl Pts',(-26.4206471327102,-0.0570574791966879,
-43.7359587822667));
#32117=CARTESIAN_POINT('Ctrl Pts',(-26.4365127811393,-0.0682199099401007,
-44.5016798704673));
#32118=CARTESIAN_POINT('Ctrl Pts',(-26.4507600954306,-0.0717721409268919,
-45.1502723734384));
#32119=CARTESIAN_POINT('Ctrl Pts',(-26.4631485089363,-0.0684515872827657,
-45.6756036567527));
#32120=CARTESIAN_POINT('Ctrl Pts',(-26.4730834273353,-0.0622375662230723,
-46.0726037171871));
#32121=CARTESIAN_POINT('Ctrl Pts',(-26.4837699828375,-0.0515935685134581,
-46.4726163317117));
#32122=CARTESIAN_POINT('Ctrl Pts',(-26.4991359060241,-0.0305036443217214,
-47.009862706898));
#32123=CARTESIAN_POINT('Ctrl Pts',(-26.5121828351866,-0.00591486366776645,
-47.4170859639793));
#32124=CARTESIAN_POINT('Ctrl Pts',(-26.526370740002,0.026204196782403,-47.8275722662938));
#32125=CARTESIAN_POINT('Ctrl Pts',(-26.5368999472404,0.0469741353359872,
-48.0837653863055));
#32126=CARTESIAN_POINT('Ctrl Pts',(-26.561505249712,0.0933214806286183,
-48.6082125153391));
#32127=CARTESIAN_POINT('Ctrl Pts',(-26.6122988327719,0.185167815068433,
-49.5236130485645));
#32128=CARTESIAN_POINT('Ctrl Pts',(-26.6981479760903,0.354523776728155,
-50.8430742403432));
#32129=CARTESIAN_POINT('Ctrl Pts',(-26.7897670019238,0.632358244960462,
-52.4342725278277));
#32130=CARTESIAN_POINT('Ctrl Pts',(-26.8215844026514,0.870582339384173,
-53.4999944261828));
#32131=CARTESIAN_POINT('Ctrl Pts',(-26.8260719038306,1.03697665514042,-54.1689646396975));
#32132=CARTESIAN_POINT('Ctrl Pts',(-26.8267141003341,1.10670827271461,-54.4412685219691));
#32133=CARTESIAN_POINT('Ctrl Pts',(-26.8239229838561,1.2530150747219,-54.9820638531088));
#32134=CARTESIAN_POINT('Ctrl Pts',(-26.8094090076117,1.52687003205735,-55.9232842367911));
#32135=CARTESIAN_POINT('Ctrl Pts',(-26.7502718252429,2.13524051873476,-57.7806701159655));
#32136=CARTESIAN_POINT('Ctrl Pts',(-26.6752243845139,2.7305383529955,-59.3268082550157));
#32137=CARTESIAN_POINT('Ctrl Pts',(-26.6326526327287,3.15991915978893,-60.3965741559011));
#32138=CARTESIAN_POINT('Ctrl Pts',(-26.626796545975,3.21513955923081,-60.5332834491796));
#32139=CARTESIAN_POINT('Ctrl Pts',(-26.6147773682979,3.32555826188788,-60.802125674637));
#32140=CARTESIAN_POINT('Ctrl Pts',(-26.5921560075181,3.52329843623239,-61.2727430817421));
#32141=CARTESIAN_POINT('Ctrl Pts',(-26.5424166539232,3.93163734514937,-62.2048352783439));
#32142=CARTESIAN_POINT('Ctrl Pts',(-26.4798588133065,4.42290831484138,-63.2519488087729));
#32143=CARTESIAN_POINT('Ctrl Pts',(-26.4209725251522,4.92351798754586,-64.275801140273));
#32144=CARTESIAN_POINT('Ctrl Pts',(-26.3908305504492,5.20574309869606,-64.842548605701));
#32145=CARTESIAN_POINT('Ctrl Pts',(-26.3726624707943,5.39290454963424,-65.2162099904711));
#32146=CARTESIAN_POINT('Ctrl Pts',(-26.3611127413162,5.51731893373302,-65.4641867626717));
#32147=CARTESIAN_POINT('Ctrl Pts',(-26.350457060261,5.64112088719479,-65.7104773833032));
#32148=CARTESIAN_POINT('Ctrl Pts',(-26.3420548604655,5.74863241414718,-65.924405367996));
#32149=CARTESIAN_POINT('Ctrl Pts',(-26.337532095308,5.8098084630586,-66.0461948795629));
#32150=CARTESIAN_POINT('Ctrl Pts',(-26.3310362843529,5.90130035682774,-66.2284296655541));
#32151=CARTESIAN_POINT('Ctrl Pts',(-26.3262335770603,5.97694150202082,-66.3793158252329));
#32152=CARTESIAN_POINT('Ctrl Pts',(-26.319205668863,6.10130572534613,-66.6280505446839));
#32153=CARTESIAN_POINT('Ctrl Pts',(-26.3127232182357,6.23599075482196,-66.8956533728625));
#32154=CARTESIAN_POINT('Ctrl Pts',(-26.3027625454309,6.50273866782855,-67.4190586948082));
#32155=CARTESIAN_POINT('Ctrl Pts',(-26.292289466235,6.97273749902019,-68.3260826013178));
#32156=CARTESIAN_POINT('Ctrl Pts',(-26.2927638675289,7.91373509191888,-70.0956972417704));
#32157=CARTESIAN_POINT('Ctrl Pts',(-26.3084135850719,8.71555338749269,-71.5704800074898));
#32158=CARTESIAN_POINT('Ctrl Pts',(-26.3069267097133,9.30581961794523,-72.6838758449878));
#32159=CARTESIAN_POINT('Ctrl Pts',(-26.3066448287013,9.43971394243508,-72.9363526706905));
#32160=CARTESIAN_POINT('Ctrl Pts',(-26.3062240590782,9.70620739982533,-73.4385206011396));
#32161=CARTESIAN_POINT('Ctrl Pts',(-26.305940355283,10.0399597181007,-74.0668450111416));
#32162=CARTESIAN_POINT('Ctrl Pts',(-26.3059074450485,10.4401946275587,-74.8196393294015));
#32163=CARTESIAN_POINT('Ctrl Pts',(-26.3062657564787,11.2408551638692,-76.3246049709325));
#32164=CARTESIAN_POINT('Ctrl Pts',(-26.3070482825158,11.9079288942245,-77.5772542386599));
#32165=CARTESIAN_POINT('Ctrl Pts',(-26.3070325410241,12.8772469790119,-79.4002400070955));
#32166=CARTESIAN_POINT('Ctrl Pts',(-26.3070253104064,13.3140222206688,-80.2216760094386));
#32167=CARTESIAN_POINT('Ctrl Pts',(-26.3070253104064,13.7505438080583,-81.0426537115369));
#32168=CARTESIAN_POINT('Ctrl Pts',(-24.4302598458315,0.00207241768738013,
24.8306321780374));
#32169=CARTESIAN_POINT('Ctrl Pts',(-24.4303326385072,0.00207243626309089,
24.7817527847082));
#32170=CARTESIAN_POINT('Ctrl Pts',(-24.4304089822103,0.00207245410495211,
24.7328744451339));
#32171=CARTESIAN_POINT('Ctrl Pts',(-24.431310518414,0.00207273452647534,
24.1822653742894));
#32172=CARTESIAN_POINT('Ctrl Pts',(-24.4319997949999,0.002074798633469,
23.1781282789352));
#32173=CARTESIAN_POINT('Ctrl Pts',(-24.4336029354561,0.00207958583484067,
21.169528032579));
#32174=CARTESIAN_POINT('Ctrl Pts',(-24.4396028097008,0.00208213590548975,
19.665375037048));
#32175=CARTESIAN_POINT('Ctrl Pts',(-24.4523362120325,0.00207846071060644,
18.4143265564543));
#32176=CARTESIAN_POINT('Ctrl Pts',(-24.4584422452079,0.00207700396147341,
17.9115055015473));
#32177=CARTESIAN_POINT('Ctrl Pts',(-24.4737736243947,0.00207419848106817,
16.9075122978479));
#32178=CARTESIAN_POINT('Ctrl Pts',(-24.5066586150648,0.00206743293100846,
15.1537005858998));
#32179=CARTESIAN_POINT('Ctrl Pts',(-24.5379117822613,0.00205552255842673,
13.6519696262246));
#32180=CARTESIAN_POINT('Ctrl Pts',(-24.5575252982735,0.00203417914685445,
12.3975128714527));
#32181=CARTESIAN_POINT('Ctrl Pts',(-24.5655458139266,0.0020235622723546,
11.896565806553));
#32182=CARTESIAN_POINT('Ctrl Pts',(-24.581904661484,0.00199730192436314,
10.8947319643132));
#32183=CARTESIAN_POINT('Ctrl Pts',(-24.6102349989673,0.00194086962837188,
9.14120368806769));
#32184=CARTESIAN_POINT('Ctrl Pts',(-24.6301298063699,0.00189647960059792,
7.63597166157432));
#32185=CARTESIAN_POINT('Ctrl Pts',(-24.6389709679162,0.00187539772952453,
6.50503228212297));
#32186=CARTESIAN_POINT('Ctrl Pts',(-24.6408586920625,0.00185852210705859,
6.25496417883429));
#32187=CARTESIAN_POINT('Ctrl Pts',(-24.6443450540568,0.00178646142423656,
5.75402051427475));
#32188=CARTESIAN_POINT('Ctrl Pts',(-24.6496310763466,0.00158564485051102,
4.87583468008954));
#32189=CARTESIAN_POINT('Ctrl Pts',(-24.6564832101539,0.001060595851991,
3.11545176947256));
#32190=CARTESIAN_POINT('Ctrl Pts',(-24.6544271176886,0.0010725556503662,
1.60780682331442));
#32191=CARTESIAN_POINT('Ctrl Pts',(-24.6477393559816,0.00187911894342457,
0.547228808229092));
#32192=CARTESIAN_POINT('Ctrl Pts',(-24.6468670454309,0.00198228716043408,
0.420859272548393));
#32193=CARTESIAN_POINT('Ctrl Pts',(-24.6448379805963,0.00222154099192133,
0.168378929386594));
#32194=CARTESIAN_POINT('Ctrl Pts',(-24.6405822662372,0.00271852968384454,
-0.27292074557853));
#32195=CARTESIAN_POINT('Ctrl Pts',(-24.6327330953819,0.00362879071700781,
-0.901883303165047));
#32196=CARTESIAN_POINT('Ctrl Pts',(-24.6212550923228,0.00492381701602845,
-1.65477326639694));
#32197=CARTESIAN_POINT('Ctrl Pts',(-24.6042511572935,0.00681216662778669,
-2.65675225674018));
#32198=CARTESIAN_POINT('Ctrl Pts',(-24.5817526291741,0.00920233268893764,
-3.90689693828391));
#32199=CARTESIAN_POINT('Ctrl Pts',(-24.5665854070869,0.0106595112999088,
-4.90704239014045));
#32200=CARTESIAN_POINT('Ctrl Pts',(-24.5592701464447,0.011252652744233,
-5.53300978139183));
#32201=CARTESIAN_POINT('Ctrl Pts',(-24.5563805916875,0.0114808742337481,
-5.78390798487287));
#32202=CARTESIAN_POINT('Ctrl Pts',(-24.5507648758424,0.0119110310305683,
-6.28579785044557));
#32203=CARTESIAN_POINT('Ctrl Pts',(-24.5413723315553,0.0125867636336026,
-7.16473631064441));
#32204=CARTESIAN_POINT('Ctrl Pts',(-24.5292461080297,0.013296537346102,
-8.42079248918329));
#32205=CARTESIAN_POINT('Ctrl Pts',(-24.5189813407149,0.0135655554008891,
-9.6747509929314));
#32206=CARTESIAN_POINT('Ctrl Pts',(-24.5128446667743,0.0134673077102899,
-10.5499339117164));
#32207=CARTESIAN_POINT('Ctrl Pts',(-24.5096481069911,0.0133233761694472,
-11.0490941768464));
#32208=CARTESIAN_POINT('Ctrl Pts',(-24.5081546115769,0.0132207732092439,
-11.298325141733));
#32209=CARTESIAN_POINT('Ctrl Pts',(-24.5070700376299,0.0131315030567913,
-11.4858819021457));
#32210=CARTESIAN_POINT('Ctrl Pts',(-24.5063550638443,0.0130605512375759,
-11.6116968164213));
#32211=CARTESIAN_POINT('Ctrl Pts',(-24.5049805016318,0.0128761532028387,
-11.8631927519117));
#32212=CARTESIAN_POINT('Ctrl Pts',(-24.5027188133538,0.0124505890990866,
-12.3026550313652));
#32213=CARTESIAN_POINT('Ctrl Pts',(-24.4976258539558,0.0109093890863102,
-13.4301717344791));
#32214=CARTESIAN_POINT('Ctrl Pts',(-24.4940183631344,0.00834978154633404,
-14.6783035848225));
#32215=CARTESIAN_POINT('Ctrl Pts',(-24.4922145413803,0.00639335755892261,
-15.9307710268368));
#32216=CARTESIAN_POINT('Ctrl Pts',(-24.4917335592822,0.00569212405988055,
-16.5588156965784));
#32217=CARTESIAN_POINT('Ctrl Pts',(-24.4915994843194,0.00536769089701191,
-17.0627887753014));
#32218=CARTESIAN_POINT('Ctrl Pts',(-24.4916099867796,0.00529831606360045,
-17.3153668936557));
#32219=CARTESIAN_POINT('Ctrl Pts',(-24.4916481807073,0.00528513131603834,
-17.5042432457089));
#32220=CARTESIAN_POINT('Ctrl Pts',(-24.4917240828623,0.0052615853092459,
-17.6284683291437));
#32221=CARTESIAN_POINT('Ctrl Pts',(-24.4920652428219,0.00517239651012107,
-17.8774695208318));
#32222=CARTESIAN_POINT('Ctrl Pts',(-24.4926623408773,0.0050290820999663,
-18.126553375236));
#32223=CARTESIAN_POINT('Ctrl Pts',(-24.493478719597,0.00485067977437561,
-18.375950292712));
#32224=CARTESIAN_POINT('Ctrl Pts',(-24.4940684557923,0.00472919091578594,
-18.531904423794));
#32225=CARTESIAN_POINT('Ctrl Pts',(-24.4945834813114,0.00462833140614637,
-18.6567339566448));
#32226=CARTESIAN_POINT('Ctrl Pts',(-24.4951251970626,0.00452598289165581,
-18.7816014343059));
#32227=CARTESIAN_POINT('Ctrl Pts',(-24.4967125631211,0.00424156214605843,
-19.1251545575784));
#32228=CARTESIAN_POINT('Ctrl Pts',(-24.4997778141386,0.00379928994353248,
-19.6882390161473));
#32229=CARTESIAN_POINT('Ctrl Pts',(-24.5055739239131,0.00349296678830271,
-20.691948680636));
#32230=CARTESIAN_POINT('Ctrl Pts',(-24.5116689861703,0.00477590510021411,
-21.9517128859598));
#32231=CARTESIAN_POINT('Ctrl Pts',(-24.5114599746138,0.00915274888702006,
-22.9653116795392));
#32232=CARTESIAN_POINT('Ctrl Pts',(-24.5085973031169,0.0134042955649363,
-23.5989907703078));
#32233=CARTESIAN_POINT('Ctrl Pts',(-24.5071839600544,0.0153250677326657,
-23.8507766410973));
#32234=CARTESIAN_POINT('Ctrl Pts',(-24.5033609516529,0.0199682168708636,
-24.3539080326969));
#32235=CARTESIAN_POINT('Ctrl Pts',(-24.494397425932,0.0299078898256353,
-25.2349883068055));
#32236=CARTESIAN_POINT('Ctrl Pts',(-24.4769679435678,0.0476718924133547,
-26.493080401859));
#32237=CARTESIAN_POINT('Ctrl Pts',(-24.4546824689337,0.0693532016334583,
-27.9987128880141));
#32238=CARTESIAN_POINT('Ctrl Pts',(-24.4428315205947,0.0806786400363348,
-28.9969020103129));
#32239=CARTESIAN_POINT('Ctrl Pts',(-24.4381971026002,0.0851810986839638,
-29.5562517451831));
#32240=CARTESIAN_POINT('Ctrl Pts',(-24.437158111982,0.0861796630639383,
-29.6816608219294));
#32241=CARTESIAN_POINT('Ctrl Pts',(-24.4350376262919,0.0881342235921294,
-29.9318858140557));
#32242=CARTESIAN_POINT('Ctrl Pts',(-24.431243098981,0.0914552866878719,
-30.3701639510382));
#32243=CARTESIAN_POINT('Ctrl Pts',(-24.4235320523414,0.0976282111301398,
-31.2466767067308));
#32244=CARTESIAN_POINT('Ctrl Pts',(-24.4153961523886,0.103398142960177,
-32.2483511659307));
#32245=CARTESIAN_POINT('Ctrl Pts',(-24.4098556239652,0.107400651713681,
-33.2487697414918));
#32246=CARTESIAN_POINT('Ctrl Pts',(-24.407476970373,0.109398407187711,-33.9982272445929));
#32247=CARTESIAN_POINT('Ctrl Pts',(-24.407340084132,0.110290937033988,-34.7464252744325));
#32248=CARTESIAN_POINT('Ctrl Pts',(-24.4090646693321,0.110065084728235,
-35.2442253444765));
#32249=CARTESIAN_POINT('Ctrl Pts',(-24.4111627264825,0.109555550582656,
-35.6181363661944));
#32250=CARTESIAN_POINT('Ctrl Pts',(-24.4129585191794,0.109054162214716,
-35.8680609341064));
#32251=CARTESIAN_POINT('Ctrl Pts',(-24.417942569389,0.107468332881441,-36.3678457663949));
#32252=CARTESIAN_POINT('Ctrl Pts',(-24.4298882542792,0.103316258927521,
-37.2412402280608));
#32253=CARTESIAN_POINT('Ctrl Pts',(-24.4630849505217,0.0905723985382749,
-38.9871180300605));
#32254=CARTESIAN_POINT('Ctrl Pts',(-24.4953445175915,0.0759084845649608,
-40.4869183501336));
#32255=CARTESIAN_POINT('Ctrl Pts',(-24.5091123507204,0.0669078016820844,
-41.6192789458791));
#32256=CARTESIAN_POINT('Ctrl Pts',(-24.5119517950053,0.0641038462103697,
-41.8564784811102));
#32257=CARTESIAN_POINT('Ctrl Pts',(-24.5156935975892,0.0575419311246697,
-42.222261181654));
#32258=CARTESIAN_POINT('Ctrl Pts',(-24.5189923423272,0.0491744390235501,
-42.5889094138677));
#32259=CARTESIAN_POINT('Ctrl Pts',(-24.5229053335981,0.0362327533694244,
-43.0832933189361));
#32260=CARTESIAN_POINT('Ctrl Pts',(-24.5270743109208,0.0179897766914957,
-43.7085230130832));
#32261=CARTESIAN_POINT('Ctrl Pts',(-24.5315455407593,-0.00303568299465702,
-44.4709890642209));
#32262=CARTESIAN_POINT('Ctrl Pts',(-24.5353508868689,-0.0161922105588385,
-45.1156507267256));
#32263=CARTESIAN_POINT('Ctrl Pts',(-24.5387295038189,-0.0217811995201414,
-45.6371377033781));
#32264=CARTESIAN_POINT('Ctrl Pts',(-24.5415198954755,-0.0229289638506116,
-46.0308811465701));
#32265=CARTESIAN_POINT('Ctrl Pts',(-24.5446424675927,-0.0204296702137602,
-46.4272764748594));
#32266=CARTESIAN_POINT('Ctrl Pts',(-24.5493386649675,-0.0113998295332617,
-46.9592228942674));
#32267=CARTESIAN_POINT('Ctrl Pts',(-24.5536095026516,0.00267333340698166,
-47.3619485254795));
#32268=CARTESIAN_POINT('Ctrl Pts',(-24.5584966620003,0.0229773607762555,
-47.7674954424624));
#32269=CARTESIAN_POINT('Ctrl Pts',(-24.5621553335303,0.0354725859022536,
-48.0152906571207));
#32270=CARTESIAN_POINT('Ctrl Pts',(-24.5707909193746,0.0622711721228399,
-48.5281809417318));
#32271=CARTESIAN_POINT('Ctrl Pts',(-24.5887105266626,0.113497280171948,
-49.4272609544128));
#32272=CARTESIAN_POINT('Ctrl Pts',(-24.6187359609351,0.210192496210709,
-50.740361535343));
#32273=CARTESIAN_POINT('Ctrl Pts',(-24.6503243045101,0.398680573907358,
-52.3517752767282));
#32274=CARTESIAN_POINT('Ctrl Pts',(-24.6607334085916,0.59837907497145,-53.449706273352));
#32275=CARTESIAN_POINT('Ctrl Pts',(-24.6613898700266,0.75495658257339,-54.1427419081582));
#32276=CARTESIAN_POINT('Ctrl Pts',(-24.6612844713376,0.820215401011333,
-54.4191314775285));
#32277=CARTESIAN_POINT('Ctrl Pts',(-24.6594955603515,0.960978655381601,
-54.9704129351631));
#32278=CARTESIAN_POINT('Ctrl Pts',(-24.6526704548069,1.23130756620562,-55.9263760818197));
#32279=CARTESIAN_POINT('Ctrl Pts',(-24.6268775428713,1.85499360305803,-57.8066070350233));
#32280=CARTESIAN_POINT('Ctrl Pts',(-24.5937661179274,2.48615112714016,-59.3601307886181));
#32281=CARTESIAN_POINT('Ctrl Pts',(-24.5743043395494,2.94126764369053,-60.4331272568145));
#32282=CARTESIAN_POINT('Ctrl Pts',(-24.5716009404588,3.00134291718464,-60.5731555051268));
#32283=CARTESIAN_POINT('Ctrl Pts',(-24.5661071223651,3.12119743169122,-60.8463917069801));
#32284=CARTESIAN_POINT('Ctrl Pts',(-24.5558500913542,3.33727209231942,-61.3242676932214));
#32285=CARTESIAN_POINT('Ctrl Pts',(-24.5336696574173,3.78612502179004,-62.2654638944784));
#32286=CARTESIAN_POINT('Ctrl Pts',(-24.5065252373297,4.32737664175834,-63.314694069021));
#32287=CARTESIAN_POINT('Ctrl Pts',(-24.4812937594002,4.87146583166284,-64.3341137358084));
#32288=CARTESIAN_POINT('Ctrl Pts',(-24.4684022046568,5.17422033520213,-64.8960125401331));
#32289=CARTESIAN_POINT('Ctrl Pts',(-24.4606128848326,5.3727638471553,-65.265377211583));
#32290=CARTESIAN_POINT('Ctrl Pts',(-24.455653438339,5.50412132243228,-65.5101940366358));
#32291=CARTESIAN_POINT('Ctrl Pts',(-24.4510643974821,5.63382037500812,-65.7528735627069));
#32292=CARTESIAN_POINT('Ctrl Pts',(-24.4474287044718,5.74548701822204,-65.9632044442411));
#32293=CARTESIAN_POINT('Ctrl Pts',(-24.4454660639254,5.80873343716068,-66.0828078307119));
#32294=CARTESIAN_POINT('Ctrl Pts',(-24.4426410572854,5.90302204618168,-66.2616316609985));
#32295=CARTESIAN_POINT('Ctrl Pts',(-24.4405393173356,5.98032222827673,-66.4093865925176));
#32296=CARTESIAN_POINT('Ctrl Pts',(-24.4374419315558,6.10651196484111,-66.6525651721026));
#32297=CARTESIAN_POINT('Ctrl Pts',(-24.4345549187866,6.2440967110459,-66.9170042846155));
#32298=CARTESIAN_POINT('Ctrl Pts',(-24.4300637962104,6.51409741201617,-67.4333801335246));
#32299=CARTESIAN_POINT('Ctrl Pts',(-24.425168552151,6.98636377680275,-68.3305700423672));
#32300=CARTESIAN_POINT('Ctrl Pts',(-24.4246416609853,7.92087819494418,-70.0871472467393));
#32301=CARTESIAN_POINT('Ctrl Pts',(-24.4309659146112,8.71389867548645,-71.5642871099131));
#32302=CARTESIAN_POINT('Ctrl Pts',(-24.4301357399251,9.30957432990654,-72.6856843844485));
#32303=CARTESIAN_POINT('Ctrl Pts',(-24.4299759003447,9.44326321325677,-72.9373360128412));
#32304=CARTESIAN_POINT('Ctrl Pts',(-24.4297382797287,9.71004184609948,-73.4393965823722));
#32305=CARTESIAN_POINT('Ctrl Pts',(-24.4295787141261,10.0436707306615,-74.0670696937808));
#32306=CARTESIAN_POINT('Ctrl Pts',(-24.4295603802771,10.4437552277089,-74.8195394237861));
#32307=CARTESIAN_POINT('Ctrl Pts',(-24.429763590671,11.2438033081569,-76.323923224447));
#32308=CARTESIAN_POINT('Ctrl Pts',(-24.4302109127262,11.9102911176329,-77.5767536096995));
#32309=CARTESIAN_POINT('Ctrl Pts',(-24.4302054054525,12.8800006302382,-79.4004972959445));
#32310=CARTESIAN_POINT('Ctrl Pts',(-24.4302025491906,13.3166339961519,-80.2216776786048));
#32311=CARTESIAN_POINT('Ctrl Pts',(-24.4302025491907,13.7531555835413,-81.0426553807033));
#32312=CARTESIAN_POINT('Ctrl Pts',(-21.9279465977811,0.00175951622296883,
24.8306324554501));
#32313=CARTESIAN_POINT('Ctrl Pts',(-21.9280121170153,0.00175964344790449,
24.781753071759));
#32314=CARTESIAN_POINT('Ctrl Pts',(-21.9280808293462,0.00175977781990619,
24.7328747382815));
#32315=CARTESIAN_POINT('Ctrl Pts',(-21.92889238123,0.00176131782851828,
24.1822659030951));
#32316=CARTESIAN_POINT('Ctrl Pts',(-21.9295158979077,0.00176336457478976,
23.1781303380483));
#32317=CARTESIAN_POINT('Ctrl Pts',(-21.9309656870421,0.00176950496491764,
21.1695302130375));
#32318=CARTESIAN_POINT('Ctrl Pts',(-21.9363681073529,0.00177920907406832,
19.6653789377107));
#32319=CARTESIAN_POINT('Ctrl Pts',(-21.9478185541189,0.00179538797735874,
18.4143308425655));
#32320=CARTESIAN_POINT('Ctrl Pts',(-21.9533099655257,0.00180374455169626,
17.9115099719552));
#32321=CARTESIAN_POINT('Ctrl Pts',(-21.9670999905151,0.00182548904108017,
16.9075176911551));
#32322=CARTESIAN_POINT('Ctrl Pts',(-21.9966773686041,0.00187213302403837,
15.1537079278605));
#32323=CARTESIAN_POINT('Ctrl Pts',(-22.0247784148631,0.00190770551231591,
13.651983107781));
#32324=CARTESIAN_POINT('Ctrl Pts',(-22.0423878964479,0.00191697506843397,
12.3975281756335));
#32325=CARTESIAN_POINT('Ctrl Pts',(-22.0495852477736,0.00191946799397687,
11.8965814801248));
#32326=CARTESIAN_POINT('Ctrl Pts',(-22.0642572378507,0.00191940508346344,
10.8947480143028));
#32327=CARTESIAN_POINT('Ctrl Pts',(-22.0896457188007,0.00190964450556511,
9.14122391316817));
#32328=CARTESIAN_POINT('Ctrl Pts',(-22.1074723723614,0.0018880970889791,
7.63599689309631));
#32329=CARTESIAN_POINT('Ctrl Pts',(-22.1153910834707,0.00187742024493833,
6.50508897037416));
#32330=CARTESIAN_POINT('Ctrl Pts',(-22.1170806542096,0.00183745708476382,
6.25535887539741));
#32331=CARTESIAN_POINT('Ctrl Pts',(-22.1202010397395,0.00163413418158526,
5.7547810784773));
#32332=CARTESIAN_POINT('Ctrl Pts',(-22.1249365315808,0.00102700920702048,
4.87705708893644));
#32333=CARTESIAN_POINT('Ctrl Pts',(-22.1310631764226,-0.000586504213302211,
3.11639638920408));
#32334=CARTESIAN_POINT('Ctrl Pts',(-22.1292472805707,-0.000624428257233562,
1.60666654112928));
#32335=CARTESIAN_POINT('Ctrl Pts',(-22.1232338886141,0.00196592706724001,
0.543614270522805));
#32336=CARTESIAN_POINT('Ctrl Pts',(-22.1224468642436,0.00230434065417858,
0.41680611961292));
#32337=CARTESIAN_POINT('Ctrl Pts',(-22.1206195413777,0.00308485495392856,
0.163585690488821));
#32338=CARTESIAN_POINT('Ctrl Pts',(-22.1167890626131,0.00470887143392074,
-0.278924031202465));
#32339=CARTESIAN_POINT('Ctrl Pts',(-22.1097491817296,0.00765941886444899,
-0.909217618427138));
#32340=CARTESIAN_POINT('Ctrl Pts',(-22.099434434,0.0119006843220359,-1.66311655997141));
#32341=CARTESIAN_POINT('Ctrl Pts',(-22.0841832508903,0.0180424043540248,
-2.66563404729465));
#32342=CARTESIAN_POINT('Ctrl Pts',(-22.0639466303909,0.0258459431950208,
-3.91493137792277));
#32343=CARTESIAN_POINT('Ctrl Pts',(-22.0502884904995,0.0304341271802674,
-4.91271788975723));
#32344=CARTESIAN_POINT('Ctrl Pts',(-22.0436783572246,0.0322449760248729,
-5.53670268338412));
#32345=CARTESIAN_POINT('Ctrl Pts',(-22.0410867838493,0.0329253083784759,
-5.78724516906531));
#32346=CARTESIAN_POINT('Ctrl Pts',(-22.0361114300666,0.0340915037912527,
-6.28827188597159));
#32347=CARTESIAN_POINT('Ctrl Pts',(-22.027930623879,0.0356660657653625,
-7.16603921623362));
#32348=CARTESIAN_POINT('Ctrl Pts',(-22.017585062098,0.0367750778497687,
-8.42096472119512));
#32349=CARTESIAN_POINT('Ctrl Pts',(-22.0085785512836,0.0369101653247734,
-9.67464069070803));
#32350=CARTESIAN_POINT('Ctrl Pts',(-22.0027354354742,0.0367827534589613,
-10.5500380438823));
#32351=CARTESIAN_POINT('Ctrl Pts',(-21.9994999796009,0.036687215795415,
-11.0494463898198));
#32352=CARTESIAN_POINT('Ctrl Pts',(-21.9979116395995,0.0366384598287954,
-11.2988436135343));
#32353=CARTESIAN_POINT('Ctrl Pts',(-21.9967239254123,0.0366042714378169,
-11.4865372190639));
#32354=CARTESIAN_POINT('Ctrl Pts',(-21.995920574385,0.0365690242444882,
-11.6122999921727));
#32355=CARTESIAN_POINT('Ctrl Pts',(-21.9942994172464,0.036453560970677,
-11.8637724354554));
#32356=CARTESIAN_POINT('Ctrl Pts',(-21.9914369892605,0.0361403869370173,
-12.3031537286525));
#32357=CARTESIAN_POINT('Ctrl Pts',(-21.9840608742727,0.0348460947202343,
-13.430502857113));
#32358=CARTESIAN_POINT('Ctrl Pts',(-21.9764939645097,0.0324567970781609,
-14.6784689813424));
#32359=CARTESIAN_POINT('Ctrl Pts',(-21.9715831482783,0.0305970299247923,
-15.9308156393427));
#32360=CARTESIAN_POINT('Ctrl Pts',(-21.9699662011677,0.0299202348326696,
-16.5588078732846));
#32361=CARTESIAN_POINT('Ctrl Pts',(-21.9692791158919,0.0296011100378451,
-17.0627381988692));
#32362=CARTESIAN_POINT('Ctrl Pts',(-21.969153381612,0.0295292129838952,
-17.3152951382543));
#32363=CARTESIAN_POINT('Ctrl Pts',(-21.9691483617438,0.0295116738601406,
-17.5041552476115));
#32364=CARTESIAN_POINT('Ctrl Pts',(-21.96916733847,0.0294900157658974,-17.6283858382307));
#32365=CARTESIAN_POINT('Ctrl Pts',(-21.9692943053054,0.0294045671680399,
-17.8773833116316));
#32366=CARTESIAN_POINT('Ctrl Pts',(-21.9695468595739,0.0292701391130193,
-18.1264625823667));
#32367=CARTESIAN_POINT('Ctrl Pts',(-21.9699270373279,0.0290973238702737,
-18.3758457729672));
#32368=CARTESIAN_POINT('Ctrl Pts',(-21.97021437127,0.0289788704117424,-18.5317897716106));
#32369=CARTESIAN_POINT('Ctrl Pts',(-21.9704745061476,0.0288790791668411,
-18.6566094709869));
#32370=CARTESIAN_POINT('Ctrl Pts',(-21.9707547161318,0.0287766287899759,
-18.7814662301224));
#32371=CARTESIAN_POINT('Ctrl Pts',(-21.9715975974669,0.0284937059708799,
-19.124987759595));
#32372=CARTESIAN_POINT('Ctrl Pts',(-21.9734082967844,0.0280234505304098,
-19.6880028128856));
#32373=CARTESIAN_POINT('Ctrl Pts',(-21.9776629528484,0.0275971656286527,
-20.6915562006487));
#32374=CARTESIAN_POINT('Ctrl Pts',(-21.9848932360202,0.0284341672262077,
-21.9510748950649));
#32375=CARTESIAN_POINT('Ctrl Pts',(-21.9920427959345,0.0322868659644219,
-22.9644653051218));
#32376=CARTESIAN_POINT('Ctrl Pts',(-21.9968786544342,0.0361029476538094,
-23.5980019232506));
#32377=CARTESIAN_POINT('Ctrl Pts',(-21.9989557767391,0.0378167863464522,
-23.849607605715));
#32378=CARTESIAN_POINT('Ctrl Pts',(-22.0036228945842,0.041998979988164,
-24.3525147490087));
#32379=CARTESIAN_POINT('Ctrl Pts',(-22.0129828236567,0.0510204938530624,
-25.2333101457441));
#32380=CARTESIAN_POINT('Ctrl Pts',(-22.0284157293752,0.0674214893682064,
-26.4913997422044));
#32381=CARTESIAN_POINT('Ctrl Pts',(-22.0470780687344,0.0877279468049168,
-27.9975063885432));
#32382=CARTESIAN_POINT('Ctrl Pts',(-22.0569039621362,0.098625472528748,
-28.9962578683356));
#32383=CARTESIAN_POINT('Ctrl Pts',(-22.061123162479,0.103028053224532,-29.5559979397897));
#32384=CARTESIAN_POINT('Ctrl Pts',(-22.0620360130022,0.104005175649616,
-29.6816094949658));
#32385=CARTESIAN_POINT('Ctrl Pts',(-22.063733901438,0.105945232381167,-29.9321457064587));
#32386=CARTESIAN_POINT('Ctrl Pts',(-22.0663793393813,0.109304486647811,
-30.3709342542632));
#32387=CARTESIAN_POINT('Ctrl Pts',(-22.0705750456291,0.115762611980201,
-31.2481658337376));
#32388=CARTESIAN_POINT('Ctrl Pts',(-22.0735587465917,0.122130800122623,
-32.2500012284327));
#32389=CARTESIAN_POINT('Ctrl Pts',(-22.0763008034624,0.126640527630062,
-33.2498713812575));
#32390=CARTESIAN_POINT('Ctrl Pts',(-22.0786225028573,0.128886482354336,
-33.9985658158203));
#32391=CARTESIAN_POINT('Ctrl Pts',(-22.0815007275582,0.129824944286313,
-34.7456311160509));
#32392=CARTESIAN_POINT('Ctrl Pts',(-22.0840662047962,0.129436579270529,
-35.2424402794722));
#32393=CARTESIAN_POINT('Ctrl Pts',(-22.0863382225049,0.128717640802482,
-35.6155133325656));
#32394=CARTESIAN_POINT('Ctrl Pts',(-22.0880810035669,0.128037969530672,
-35.8646198141343));
#32395=CARTESIAN_POINT('Ctrl Pts',(-22.0922926297467,0.125949254046027,
-36.3631591269725));
#32396=CARTESIAN_POINT('Ctrl Pts',(-22.1011590699198,0.120534929666342,
-37.2348392323456));
#32397=CARTESIAN_POINT('Ctrl Pts',(-22.1219758473207,0.10447665392804,-38.9797400897251));
#32398=CARTESIAN_POINT('Ctrl Pts',(-22.1351457038762,0.086800106356149,
-40.4823985574855));
#32399=CARTESIAN_POINT('Ctrl Pts',(-22.1325839123372,0.0773464135856958,
-41.6183954976229));
#32400=CARTESIAN_POINT('Ctrl Pts',(-22.1318279488977,0.074521697206918,
-41.856276485494));
#32401=CARTESIAN_POINT('Ctrl Pts',(-22.1301651456598,0.0680399957608525,
-42.222979159865));
#32402=CARTESIAN_POINT('Ctrl Pts',(-22.127982690836,0.0598733749880051,
-42.5903995515794));
#32403=CARTESIAN_POINT('Ctrl Pts',(-22.1244120000825,0.0473241374375181,
-43.0856421099198));
#32404=CARTESIAN_POINT('Ctrl Pts',(-22.1187339509867,0.0297859917647642,
-43.7116175102801));
#32405=CARTESIAN_POINT('Ctrl Pts',(-22.1101180735002,0.00980274759246461,
-44.4744759591554));
#32406=CARTESIAN_POINT('Ctrl Pts',(-22.1015488286281,-0.00245109850784833,
-45.1190547033691));
#32407=CARTESIAN_POINT('Ctrl Pts',(-22.0938461907087,-0.00732163858416031,
-45.6402470682028));
#32408=CARTESIAN_POINT('Ctrl Pts',(-22.0876997960238,-0.00798116879003842,
-46.0336530958471));
#32409=CARTESIAN_POINT('Ctrl Pts',(-22.0811966447842,-0.00506200183720292,
-46.42959582729));
#32410=CARTESIAN_POINT('Ctrl Pts',(-22.0720393034145,0.00442485698173024,
-46.9607970498843));
#32411=CARTESIAN_POINT('Ctrl Pts',(-22.0647624157281,0.0186330222264071,
-47.3627877957541));
#32412=CARTESIAN_POINT('Ctrl Pts',(-22.0571129555406,0.0389521252813495,
-47.7675399696603));
#32413=CARTESIAN_POINT('Ctrl Pts',(-22.0515225047895,0.0515088587977791,
-48.0159301973195));
#32414=CARTESIAN_POINT('Ctrl Pts',(-22.0387634523023,0.0785805657956414,
-48.5291621989758));
#32415=CARTESIAN_POINT('Ctrl Pts',(-22.0129658748973,0.130648390847141,
-49.4286561122732));
#32416=CARTESIAN_POINT('Ctrl Pts',(-21.9702800819051,0.229437488371507,
-50.7405595922032));
#32417=CARTESIAN_POINT('Ctrl Pts',(-21.9214343424393,0.419726202256797,
-52.3470454894489));
#32418=CARTESIAN_POINT('Ctrl Pts',(-21.898911774298,0.616568864009376,-53.4393474162767));
#32419=CARTESIAN_POINT('Ctrl Pts',(-21.8902388128371,0.768961070459955,
-54.128571033495));
#32420=CARTESIAN_POINT('Ctrl Pts',(-21.8869634548092,0.831824753648006,
-54.401827475866));
#32421=CARTESIAN_POINT('Ctrl Pts',(-21.8815941860788,0.966965310402138,
-54.9488620484349));
#32422=CARTESIAN_POINT('Ctrl Pts',(-21.8749151942011,1.22522399032231,-55.8993882470461));
#32423=CARTESIAN_POINT('Ctrl Pts',(-21.8703887781199,1.82095337687199,-57.7787441431066));
#32424=CARTESIAN_POINT('Ctrl Pts',(-21.8751637879929,2.43617689572333,-59.3440137893041));
#32425=CARTESIAN_POINT('Ctrl Pts',(-21.8779292841487,2.89418131546219,-60.4294964038471));
#32426=CARTESIAN_POINT('Ctrl Pts',(-21.8784919227777,2.95453939264026,-60.570781472954));
#32427=CARTESIAN_POINT('Ctrl Pts',(-21.8797312083696,3.07529745046665,-60.8464556959951));
#32428=CARTESIAN_POINT('Ctrl Pts',(-21.8824452933382,3.29355533259279,-61.3280540237837));
#32429=CARTESIAN_POINT('Ctrl Pts',(-21.8895449231649,3.74887633727324,-62.274937263336));
#32430=CARTESIAN_POINT('Ctrl Pts',(-21.9001371399266,4.3004097935474,-63.3272029625683));
#32431=CARTESIAN_POINT('Ctrl Pts',(-21.9107842226101,4.85424205636823,-64.3470411142037));
#32432=CARTESIAN_POINT('Ctrl Pts',(-21.916354209389,5.16169784818111,-64.9082123410851));
#32433=CARTESIAN_POINT('Ctrl Pts',(-21.9196919975189,5.36282079275618,-65.2766897005441));
#32434=CARTESIAN_POINT('Ctrl Pts',(-21.921808591829,5.49572942117165,-65.5208032178986));
#32435=CARTESIAN_POINT('Ctrl Pts',(-21.9237231005401,5.62672574373137,-65.7626107899648));
#32436=CARTESIAN_POINT('Ctrl Pts',(-21.9252038876219,5.73924436353136,-65.9720206725958));
#32437=CARTESIAN_POINT('Ctrl Pts',(-21.9259867036262,5.80289378805119,-66.0910507820888));
#32438=CARTESIAN_POINT('Ctrl Pts',(-21.9270959306165,5.89769989954532,-66.268968124062));
#32439=CARTESIAN_POINT('Ctrl Pts',(-21.92787046439,5.97524992867064,-66.4158616225611));
#32440=CARTESIAN_POINT('Ctrl Pts',(-21.928940083139,6.1015843192719,-66.657495581125));
#32441=CARTESIAN_POINT('Ctrl Pts',(-21.9298881234652,6.24001972444046,-66.9217149445331));
#32442=CARTESIAN_POINT('Ctrl Pts',(-21.9312815177686,6.51102410622419,-67.4369602737428));
#32443=CARTESIAN_POINT('Ctrl Pts',(-21.9324876222294,6.98469072279545,-68.3327696709343));
#32444=CARTESIAN_POINT('Ctrl Pts',(-21.9312406243433,7.92002328406678,-70.0871946567983));
#32445=CARTESIAN_POINT('Ctrl Pts',(-21.9276469013653,8.71290538373861,-71.5643646538029));
#32446=CARTESIAN_POINT('Ctrl Pts',(-21.9275638685428,9.30971569874061,-72.6865383203896));
#32447=CARTESIAN_POINT('Ctrl Pts',(-21.9275520227615,9.44341875895882,-72.9379611812549));
#32448=CARTESIAN_POINT('Ctrl Pts',(-21.9275331342995,9.71029529116342,-73.439824462405));
#32449=CARTESIAN_POINT('Ctrl Pts',(-21.9275143845236,10.0439103544011,-74.0672059355723));
#32450=CARTESIAN_POINT('Ctrl Pts',(-21.9275097575012,10.4438969252603,-74.8194571285693));
#32451=CARTESIAN_POINT('Ctrl Pts',(-21.9275180953303,11.2436125671748,-76.3235296670018));
#32452=CARTESIAN_POINT('Ctrl Pts',(-21.9275251403254,11.909792269642,-77.5764539148375));
#32453=CARTESIAN_POINT('Ctrl Pts',(-21.9275097517017,12.8797558916182,-79.4006430631371));
#32454=CARTESIAN_POINT('Ctrl Pts',(-21.9275018204326,13.3163203389153,-80.2216771291613));
#32455=CARTESIAN_POINT('Ctrl Pts',(-21.9275018204325,13.7528419263048,-81.0426548312598));
#32456=CARTESIAN_POINT('Ctrl Pts',(-19.4210619460671,-0.000916505951998524,
24.8306358879637));
#32457=CARTESIAN_POINT('Ctrl Pts',(-19.4211200360562,-0.000916505829417001,
24.7817566113921));
#32458=CARTESIAN_POINT('Ctrl Pts',(-19.4211809608811,-0.000916508832693608,
24.7328783890003));
#32459=CARTESIAN_POINT('Ctrl Pts',(-19.4219003643249,-0.000916399674711829,
24.1822707423388));
#32460=CARTESIAN_POINT('Ctrl Pts',(-19.4224514915254,-0.000916151011694828,
23.1781361925135));
#32461=CARTESIAN_POINT('Ctrl Pts',(-19.4237349522675,-0.000917980264369305,
21.1695382470795));
#32462=CARTESIAN_POINT('Ctrl Pts',(-19.4285220752422,-0.000915706084191834,
19.6653858677669));
#32463=CARTESIAN_POINT('Ctrl Pts',(-19.4386760515693,-0.000911420001045353,
18.4143371794428));
#32464=CARTESIAN_POINT('Ctrl Pts',(-19.4435460762392,-0.000909876636940407,
17.9115228552616));
#32465=CARTESIAN_POINT('Ctrl Pts',(-19.4557752214484,-0.000906076814717268,
16.9075348604225));
#32466=CARTESIAN_POINT('Ctrl Pts',(-19.482006160143,-0.000898354421432531,
15.1537241714337));
#32467=CARTESIAN_POINT('Ctrl Pts',(-19.5069222841565,-0.000883362688828362,
13.6519746322136));
#32468=CARTESIAN_POINT('Ctrl Pts',(-19.5225393837494,-0.000868771700885713,
12.397489885296));
#32469=CARTESIAN_POINT('Ctrl Pts',(-19.5289239036206,-0.000862754752594793,
11.8965312672799));
#32470=CARTESIAN_POINT('Ctrl Pts',(-19.5419385856058,-0.000847400333427081,
10.894680435061));
#32471=CARTESIAN_POINT('Ctrl Pts',(-19.5644638714673,-0.000817476897641216,
9.14113732412567));
#32472=CARTESIAN_POINT('Ctrl Pts',(-19.580257867826,-0.000779847760490609,
7.63591652937965));
#32473=CARTESIAN_POINT('Ctrl Pts',(-19.5872721615326,-0.00076358859827383,
6.50500747984503));
#32474=CARTESIAN_POINT('Ctrl Pts',(-19.5886972281251,-0.000782736056155837,
6.25506299062874));
#32475=CARTESIAN_POINT('Ctrl Pts',(-19.5910800027927,-0.000892230357137512,
5.7542530427598));
#32476=CARTESIAN_POINT('Ctrl Pts',(-19.5941198555159,-0.00122168871274602,
4.87623338232857));
#32477=CARTESIAN_POINT('Ctrl Pts',(-19.5964733422871,-0.0021199224373692,
3.1157476232137));
#32478=CARTESIAN_POINT('Ctrl Pts',(-19.5947716363984,-0.00205443966891327,
1.60737716484397));
#32479=CARTESIAN_POINT('Ctrl Pts',(-19.5943674949496,-0.000605263955023937,
0.545854015138203));
#32480=CARTESIAN_POINT('Ctrl Pts',(-19.5943137164219,-0.000421092946140771,
0.419298119551482));
#32481=CARTESIAN_POINT('Ctrl Pts',(-19.5941782922409,9.22222472031788E-6,
0.166505185772947));
#32482=CARTESIAN_POINT('Ctrl Pts',(-19.5938698855079,0.000905763389535935,
-0.275321494516036));
#32483=CARTESIAN_POINT('Ctrl Pts',(-19.5932146204517,0.00255021532002368,
-0.904904183802462));
#32484=CARTESIAN_POINT('Ctrl Pts',(-19.5921048641433,0.00486262550340788,
-1.65833181536422));
#32485=CARTESIAN_POINT('Ctrl Pts',(-19.590178420896,0.00818343368721628,
-2.66069903279666));
#32486=CARTESIAN_POINT('Ctrl Pts',(-19.587000103224,0.0122365579874156,
-3.91061817196258));
#32487=CARTESIAN_POINT('Ctrl Pts',(-19.5836302092038,0.0145300342991261,
-4.90966274692559));
#32488=CARTESIAN_POINT('Ctrl Pts',(-19.5812386079632,0.015367054816335,
-5.53462804813499));
#32489=CARTESIAN_POINT('Ctrl Pts',(-19.5802022899887,0.0156483145176531,
-5.78514459578171));
#32490=CARTESIAN_POINT('Ctrl Pts',(-19.5778668906237,0.0160679382836999,
-6.28637862974742));
#32491=CARTESIAN_POINT('Ctrl Pts',(-19.5731682577045,0.0164580977986604,
-7.16443891094301));
#32492=CARTESIAN_POINT('Ctrl Pts',(-19.5652302476183,0.0162972237888366,
-8.42002258121338));
#32493=CARTESIAN_POINT('Ctrl Pts',(-19.557064496691,0.0158192131697322,
-9.67455998065912));
#32494=CARTESIAN_POINT('Ctrl Pts',(-19.5519697806829,0.0156446112291823,
-10.5507139521068));
#32495=CARTESIAN_POINT('Ctrl Pts',(-19.549338791014,0.0156404148149878,
-11.050593627762));
#32496=CARTESIAN_POINT('Ctrl Pts',(-19.5481338881641,0.0156781632889342,
-11.3002387949875));
#32497=CARTESIAN_POINT('Ctrl Pts',(-19.5472749165968,0.0157242021426955,
-11.488131352607));
#32498=CARTESIAN_POINT('Ctrl Pts',(-19.546695715977,0.0157584682458296,
-11.6142688933052));
#32499=CARTESIAN_POINT('Ctrl Pts',(-19.5455310250035,0.0158376730394181,
-11.8663068121108));
#32500=CARTESIAN_POINT('Ctrl Pts',(-19.5434825830314,0.0160038830033236,
-12.3066351073796));
#32501=CARTESIAN_POINT('Ctrl Pts',(-19.5382292295015,0.0165498799783075,
-13.4357721193144));
#32502=CARTESIAN_POINT('Ctrl Pts',(-19.5328369824923,0.01736958990664,-14.6839651499632));
#32503=CARTESIAN_POINT('Ctrl Pts',(-19.5291128862856,0.0179736079118189,
-15.9347209983996));
#32504=CARTESIAN_POINT('Ctrl Pts',(-19.527763502,0.0181925712051342,-16.561478567343));
#32505=CARTESIAN_POINT('Ctrl Pts',(-19.5270563863637,0.0182932341679571,
-17.0641679158956));
#32506=CARTESIAN_POINT('Ctrl Pts',(-19.526835967203,0.0183163694167679,
-17.3160098089783));
#32507=CARTESIAN_POINT('Ctrl Pts',(-19.5267251826946,0.0183219158333973,
-17.504332176674));
#32508=CARTESIAN_POINT('Ctrl Pts',(-19.5266621148149,0.0183306924441913,
-17.6291328941662));
#32509=CARTESIAN_POINT('Ctrl Pts',(-19.5265769037342,0.0183696641094957,
-17.878620482306));
#32510=CARTESIAN_POINT('Ctrl Pts',(-19.5265537745837,0.0184355791817818,
-18.1282475743827));
#32511=CARTESIAN_POINT('Ctrl Pts',(-19.5265933327143,0.0185212039296075,
-18.3779283557147));
#32512=CARTESIAN_POINT('Ctrl Pts',(-19.5266445208543,0.0185809757856958,
-18.5340216452474));
#32513=CARTESIAN_POINT('Ctrl Pts',(-19.5267013915317,0.0186316683340416,
-18.6589159726346));
#32514=CARTESIAN_POINT('Ctrl Pts',(-19.5267686767785,0.018684079673204,
-18.7838261805894));
#32515=CARTESIAN_POINT('Ctrl Pts',(-19.5270008023804,0.018830814209969,
-19.1273876797336));
#32516=CARTESIAN_POINT('Ctrl Pts',(-19.5276179635945,0.0190852158251253,
-19.6899274884205));
#32517=CARTESIAN_POINT('Ctrl Pts',(-19.5294557494281,0.019370063550402,
-20.691048800915));
#32518=CARTESIAN_POINT('Ctrl Pts',(-19.5330639946868,0.0191287867613026,
-21.9446352642524));
#32519=CARTESIAN_POINT('Ctrl Pts',(-19.5375547434322,0.0174801796606266,
-22.9501448874616));
#32520=CARTESIAN_POINT('Ctrl Pts',(-19.5408112124324,0.0158055036722608,
-23.5777955722769));
#32521=CARTESIAN_POINT('Ctrl Pts',(-19.5422114714015,0.0150511106350368,
-23.8258589230651));
#32522=CARTESIAN_POINT('Ctrl Pts',(-19.5454469135472,0.013207219676755,
-24.3232982958536));
#32523=CARTESIAN_POINT('Ctrl Pts',(-19.5520791800536,0.00922621734496209,
-25.1962301250459));
#32524=CARTESIAN_POINT('Ctrl Pts',(-19.5636214428665,0.00206128376255883,
-26.4493421322969));
#32525=CARTESIAN_POINT('Ctrl Pts',(-19.5778196153715,-0.00664813705533941,
-27.9588536438995));
#32526=CARTESIAN_POINT('Ctrl Pts',(-19.5858724946287,-0.0111975382757344,
-28.9664156053144));
#32527=CARTESIAN_POINT('Ctrl Pts',(-19.5894199088021,-0.0130148584392199,
-29.5328122940666));
#32528=CARTESIAN_POINT('Ctrl Pts',(-19.5901963882779,-0.0134115298228288,
-29.6583647772461));
#32529=CARTESIAN_POINT('Ctrl Pts',(-19.5917246464236,-0.0141634489634931,
-29.9096808259213));
#32530=CARTESIAN_POINT('Ctrl Pts',(-19.5943400924366,-0.0153825265994865,
-30.3494739152574));
#32531=CARTESIAN_POINT('Ctrl Pts',(-19.59930001926,-0.017452777268995,-31.2293526898474));
#32532=CARTESIAN_POINT('Ctrl Pts',(-19.6043489049884,-0.0191261396280685,
-32.2347494206712));
#32533=CARTESIAN_POINT('Ctrl Pts',(-19.6086516849793,-0.0204363624778105,
-33.2389780365613));
#32534=CARTESIAN_POINT('Ctrl Pts',(-19.6114742352471,-0.0213296337544048,
-33.9912721629546));
#32535=CARTESIAN_POINT('Ctrl Pts',(-19.6139183172787,-0.0222359159331191,
-34.7423334052815));
#32536=CARTESIAN_POINT('Ctrl Pts',(-19.6152624456389,-0.0229101368754363,
-35.2420615653454));
#32537=CARTESIAN_POINT('Ctrl Pts',(-19.6161576020686,-0.0234681565954076,
-35.6174351663918));
#32538=CARTESIAN_POINT('Ctrl Pts',(-19.6167566587891,-0.0239017902451974,
-35.8683357370975));
#32539=CARTESIAN_POINT('Ctrl Pts',(-19.6179540719398,-0.0249342552168865,
-36.370103134513));
#32540=CARTESIAN_POINT('Ctrl Pts',(-19.6199848251125,-0.0270541396195468,
-37.2470687416748));
#32541=CARTESIAN_POINT('Ctrl Pts',(-19.623233273403,-0.0317230467432112,
-39.00028772146));
#32542=CARTESIAN_POINT('Ctrl Pts',(-19.6222297610433,-0.0331281923398602,
-40.5063468964214));
#32543=CARTESIAN_POINT('Ctrl Pts',(-19.617501610984,-0.029738409662969,
-41.6423833562812));
#32544=CARTESIAN_POINT('Ctrl Pts',(-19.6164284597141,-0.0299257028766041,
-41.8800353799142));
#32545=CARTESIAN_POINT('Ctrl Pts',(-19.6146902487838,-0.0323119462871963,
-42.246776723759));
#32546=CARTESIAN_POINT('Ctrl Pts',(-19.6128111946042,-0.0363403388279717,
-42.6144158763));
#32547=CARTESIAN_POINT('Ctrl Pts',(-19.6100854265847,-0.0431877514880426,
-43.1103019468172));
#32548=CARTESIAN_POINT('Ctrl Pts',(-19.6062259946451,-0.0532162990883177,
-43.7376670054504));
#32549=CARTESIAN_POINT('Ctrl Pts',(-19.6006968468197,-0.063196357447491,
-44.5031764047218));
#32550=CARTESIAN_POINT('Ctrl Pts',(-19.5951934401697,-0.0659653604278103,
-45.1507878703742));
#32551=CARTESIAN_POINT('Ctrl Pts',(-19.5902116566121,-0.0624520398921263,
-45.6748227179991));
#32552=CARTESIAN_POINT('Ctrl Pts',(-19.5861424054888,-0.0563207359842689,
-46.0706039170931));
#32553=CARTESIAN_POINT('Ctrl Pts',(-19.581721807771,-0.0460566055141686,
-46.469146416803));
#32554=CARTESIAN_POINT('Ctrl Pts',(-19.575351012063,-0.0260000737641728,
-47.0041046909466));
#32555=CARTESIAN_POINT('Ctrl Pts',(-19.5699477020232,-0.00276787019770777,
-47.4092388334075));
#32556=CARTESIAN_POINT('Ctrl Pts',(-19.5641458342478,0.0273068266469621,
-47.8174344977143));
#32557=CARTESIAN_POINT('Ctrl Pts',(-19.5599406370288,0.0468609417018277,
-48.0730561138821));
#32558=CARTESIAN_POINT('Ctrl Pts',(-19.5503695770238,0.0900955080363308,
-48.5957398962124));
#32559=CARTESIAN_POINT('Ctrl Pts',(-19.531042785612,0.174928325946335,-49.5082382959596));
#32560=CARTESIAN_POINT('Ctrl Pts',(-19.4985615237133,0.327996612663541,
-50.8231236678266));
#32561=CARTESIAN_POINT('Ctrl Pts',(-19.4604047596137,0.575748356626434,
-52.4111165545092));
#32562=CARTESIAN_POINT('Ctrl Pts',(-19.4406878844852,0.792935696991215,
-53.4767992959842));
#32563=CARTESIAN_POINT('Ctrl Pts',(-19.4317522726001,0.948041883886683,
-54.1457388948874));
#32564=CARTESIAN_POINT('Ctrl Pts',(-19.4282772934766,1.01183076778066,-54.4134605162196));
#32565=CARTESIAN_POINT('Ctrl Pts',(-19.4218630286443,1.14625404644578,-54.949384838544));
#32566=CARTESIAN_POINT('Ctrl Pts',(-19.4119486847664,1.39806011300074,-55.8843438780089));
#32567=CARTESIAN_POINT('Ctrl Pts',(-19.3970680007187,1.96484144832662,-57.7440060585629));
#32568=CARTESIAN_POINT('Ctrl Pts',(-19.3915395103084,2.54557848517724,-59.311537388298));
#32569=CARTESIAN_POINT('Ctrl Pts',(-19.3902776363852,2.99144062937233,-60.4060886231981));
#32570=CARTESIAN_POINT('Ctrl Pts',(-19.3902371034511,3.04914363192602,-60.5460390725025));
#32571=CARTESIAN_POINT('Ctrl Pts',(-19.3903364333557,3.165067562148,-60.820610591561));
#32572=CARTESIAN_POINT('Ctrl Pts',(-19.391050624363,3.37413960864631,-61.2999999169842));
#32573=CARTESIAN_POINT('Ctrl Pts',(-19.3942701404576,3.81025112716761,-62.244556982017));
#32574=CARTESIAN_POINT('Ctrl Pts',(-19.4008744605687,4.33894413365338,-63.2968001570556));
#32575=CARTESIAN_POINT('Ctrl Pts',(-19.408032994212,4.87295933801209,-64.3191518232226));
#32576=CARTESIAN_POINT('Ctrl Pts',(-19.4118534041911,5.17099277029054,-64.8826381760206));
#32577=CARTESIAN_POINT('Ctrl Pts',(-19.414138409824,5.36680743778216,-65.2530842010791));
#32578=CARTESIAN_POINT('Ctrl Pts',(-19.4155782054507,5.49646259973421,-65.4986251742135));
#32579=CARTESIAN_POINT('Ctrl Pts',(-19.4168834240223,5.62461885273898,-65.7420455204344));
#32580=CARTESIAN_POINT('Ctrl Pts',(-19.4178675237502,5.73509674141069,-65.9530362578082));
#32581=CARTESIAN_POINT('Ctrl Pts',(-19.4183812835749,5.7977079991849,-66.0730215724873));
#32582=CARTESIAN_POINT('Ctrl Pts',(-19.419100544842,5.89108965768411,-66.2524240198914));
#32583=CARTESIAN_POINT('Ctrl Pts',(-19.4195923407601,5.96772063530916,-66.4006740118791));
#32584=CARTESIAN_POINT('Ctrl Pts',(-19.4202302030272,6.09294374601363,-66.6447083575439));
#32585=CARTESIAN_POINT('Ctrl Pts',(-19.420811048886,6.23015025712785,-66.9109507681786));
#32586=CARTESIAN_POINT('Ctrl Pts',(-19.4216849945587,6.49984220861854,-67.4300688672473));
#32587=CARTESIAN_POINT('Ctrl Pts',(-19.4225561721023,6.9732157016267,-68.331546792137));
#32588=CARTESIAN_POINT('Ctrl Pts',(-19.4222665935473,7.91403700035587,-70.0931374115175));
#32589=CARTESIAN_POINT('Ctrl Pts',(-19.4206541084763,8.71289353145056,-71.5687521510131));
#32590=CARTESIAN_POINT('Ctrl Pts',(-19.4207401430524,9.30691320802472,-72.6860330122269));
#32591=CARTESIAN_POINT('Ctrl Pts',(-19.4207537005546,9.44077794422047,-72.9378075977793));
#32592=CARTESIAN_POINT('Ctrl Pts',(-19.4207750104813,9.70754452589275,-73.4395419598208));
#32593=CARTESIAN_POINT('Ctrl Pts',(-19.4207918757636,10.0412095495097,-74.0670948518826));
#32594=CARTESIAN_POINT('Ctrl Pts',(-19.4207949784166,10.4411892601614,-74.8193526804547));
#32595=CARTESIAN_POINT('Ctrl Pts',(-19.4207803986868,11.2409741801607,-76.3235224409878));
#32596=CARTESIAN_POINT('Ctrl Pts',(-19.4207534481394,11.9071720009682,-77.5764574158514));
#32597=CARTESIAN_POINT('Ctrl Pts',(-19.4207606707605,12.8770765807768,-79.4006016434487));
#32598=CARTESIAN_POINT('Ctrl Pts',(-19.4207643941571,13.3136450649744,-80.221677332283));
#32599=CARTESIAN_POINT('Ctrl Pts',(-19.4207643941571,13.7501666523639,-81.0426550343813));
#32600=CARTESIAN_POINT('Ctrl Pts',(-16.913660379476,-0.000827524452366188,
24.8306357980468));
#32601=CARTESIAN_POINT('Ctrl Pts',(-16.9137108968607,-0.000827562593606038,
24.7817565175913));
#32602=CARTESIAN_POINT('Ctrl Pts',(-16.9137638734474,-0.000827595928633068,
24.7328783162098));
#32603=CARTESIAN_POINT('Ctrl Pts',(-16.9143897036163,-0.000828290732081643,
24.1822697845243));
#32604=CARTESIAN_POINT('Ctrl Pts',(-16.9148697187099,-0.000831039143720871,
23.1781280489857));
#32605=CARTESIAN_POINT('Ctrl Pts',(-16.915983118499,-0.000833657719236496,
21.1695293293891));
#32606=CARTESIAN_POINT('Ctrl Pts',(-16.9201504841003,-0.000841378666284282,
19.6653597636092));
#32607=CARTESIAN_POINT('Ctrl Pts',(-16.9289876731134,-0.00084736231422761,
18.414303705657));
#32608=CARTESIAN_POINT('Ctrl Pts',(-16.9332251626503,-0.000849785270073788,
17.9114881806577));
#32609=CARTESIAN_POINT('Ctrl Pts',(-16.9438656945415,-0.000856758256674359,
16.907495137435));
#32610=CARTESIAN_POINT('Ctrl Pts',(-16.9666882842702,-0.000870140538567631,
15.1536788536165));
#32611=CARTESIAN_POINT('Ctrl Pts',(-16.9883804934798,-0.000888969966369119,
13.6518892300676));
#32612=CARTESIAN_POINT('Ctrl Pts',(-17.0019864152639,-0.000893597145185849,
12.3973860955814));
#32613=CARTESIAN_POINT('Ctrl Pts',(-17.0075488559807,-0.000893453937685075,
11.896422233197));
#32614=CARTESIAN_POINT('Ctrl Pts',(-17.0188932522792,-0.000893246999643471,
10.8945664248175));
#32615=CARTESIAN_POINT('Ctrl Pts',(-17.0385337832344,-0.000885605163967994,
9.14097928832284));
#32616=CARTESIAN_POINT('Ctrl Pts',(-17.0523343964969,-0.000904878685921128,
7.63574110810873));
#32617=CARTESIAN_POINT('Ctrl Pts',(-17.058462893848,-0.000910611061803188,
6.50455257652354));
#32618=CARTESIAN_POINT('Ctrl Pts',(-17.0594955260761,-0.000682540425813807,
6.25140352785833));
#32619=CARTESIAN_POINT('Ctrl Pts',(-17.060467662109,0.000515190728335706,
5.74711946451873));
#32620=CARTESIAN_POINT('Ctrl Pts',(-17.0598052676819,0.00408390829977201,
4.86471861541086));
#32621=CARTESIAN_POINT('Ctrl Pts',(-17.0530133395588,0.0136791305464913,
3.10686987562814));
#32622=CARTESIAN_POINT('Ctrl Pts',(-17.0516180191862,0.0134886283242293,
1.61853830947895));
#32623=CARTESIAN_POINT('Ctrl Pts',(-17.065678391724,-0.00182901029311958,
0.580426886332494));
#32624=CARTESIAN_POINT('Ctrl Pts',(-17.0675004108405,-0.00380065202265222,
0.457974728958677));
#32625=CARTESIAN_POINT('Ctrl Pts',(-17.071705724231,-0.00835573562866867,
0.212109502037044));
#32626=CARTESIAN_POINT('Ctrl Pts',(-17.0804338756127,-0.0177940242792748,
-0.218431181088192));
#32627=CARTESIAN_POINT('Ctrl Pts',(-17.0962659546607,-0.0348756595322693,
-0.835714085139599));
#32628=CARTESIAN_POINT('Ctrl Pts',(-17.1187683270229,-0.0589813267680445,
-1.58010214196588));
#32629=CARTESIAN_POINT('Ctrl Pts',(-17.1510521082473,-0.0934349918654345,
-2.57819276246352));
#32630=CARTESIAN_POINT('Ctrl Pts',(-17.1909713554602,-0.135908212143206,
-3.83709577057073));
#32631=CARTESIAN_POINT('Ctrl Pts',(-17.2128352459153,-0.16041053381123,
-4.85804507598944));
#32632=CARTESIAN_POINT('Ctrl Pts',(-17.2204011685386,-0.170144998815634,
-5.50097319703451));
#32633=CARTESIAN_POINT('Ctrl Pts',(-17.2230212629696,-0.173691798969035,
-5.75463993676661));
#32634=CARTESIAN_POINT('Ctrl Pts',(-17.226773868513,-0.179673592855956,
-6.26361243491258));
#32635=CARTESIAN_POINT('Ctrl Pts',(-17.2298530876921,-0.187463581975278,
-7.15218489059402));
#32636=CARTESIAN_POINT('Ctrl Pts',(-17.2265650894144,-0.192574991909092,
-8.41811165575204));
#32637=CARTESIAN_POINT('Ctrl Pts',(-17.2190399777856,-0.193630202867038,
-9.67560107069014));
#32638=CARTESIAN_POINT('Ctrl Pts',(-17.2146902681715,-0.194244578555661,
-10.5502480830811));
#32639=CARTESIAN_POINT('Ctrl Pts',(-17.2129238439725,-0.194853172807012,
-11.0481815051936));
#32640=CARTESIAN_POINT('Ctrl Pts',(-17.2123555665687,-0.195290853822891,
-11.2964895401434));
#32641=CARTESIAN_POINT('Ctrl Pts',(-17.2120742904713,-0.195688068967561,
-11.4832796278456));
#32642=CARTESIAN_POINT('Ctrl Pts',(-17.2118759660511,-0.195936161386144,
-11.6101075392821));
#32643=CARTESIAN_POINT('Ctrl Pts',(-17.2114470879894,-0.196355384094459,
-11.8626834939792));
#32644=CARTESIAN_POINT('Ctrl Pts',(-17.21061966665,-0.19690157283447,-12.3042683349485));
#32645=CARTESIAN_POINT('Ctrl Pts',(-17.2081713370828,-0.197446873889082,
-13.4358154650848));
#32646=CARTESIAN_POINT('Ctrl Pts',(-17.2049351929916,-0.196136768310324,
-14.6854741481397));
#32647=CARTESIAN_POINT('Ctrl Pts',(-17.2024782246753,-0.194764755203927,
-15.9361627357538));
#32648=CARTESIAN_POINT('Ctrl Pts',(-17.2015627415889,-0.194229737741456,
-16.5625565005464));
#32649=CARTESIAN_POINT('Ctrl Pts',(-17.2010751272355,-0.193977141073183,
-17.0647351725833));
#32650=CARTESIAN_POINT('Ctrl Pts',(-17.2009273546625,-0.193928109111946,
-17.3162519971077));
#32651=CARTESIAN_POINT('Ctrl Pts',(-17.2008550310802,-0.19392460053942,
-17.5043116056623));
#32652=CARTESIAN_POINT('Ctrl Pts',(-17.2008258624349,-0.193913976446662,
-17.6291696252631));
#32653=CARTESIAN_POINT('Ctrl Pts',(-17.2008354253315,-0.193863398359589,
-17.8786368721972));
#32654=CARTESIAN_POINT('Ctrl Pts',(-17.2009458402694,-0.193777953248453,
-18.1282934782865));
#32655=CARTESIAN_POINT('Ctrl Pts',(-17.2011338662123,-0.193661867242172,
-18.3779773053783));
#32656=CARTESIAN_POINT('Ctrl Pts',(-17.2012835071638,-0.193580598815288,
-18.5340783504585));
#32657=CARTESIAN_POINT('Ctrl Pts',(-17.2014194303729,-0.193510762286717,
-18.6589766827682));
#32658=CARTESIAN_POINT('Ctrl Pts',(-17.2015653324318,-0.193438044296604,
-18.7838916531124));
#32659=CARTESIAN_POINT('Ctrl Pts',(-17.2020178074861,-0.193235661709927,
-19.1274644447809));
#32660=CARTESIAN_POINT('Ctrl Pts',(-17.2029485625811,-0.192872842355594,
-19.6900253638797));
#32661=CARTESIAN_POINT('Ctrl Pts',(-17.2049585767724,-0.192422272388314,
-20.6911781623881));
#32662=CARTESIAN_POINT('Ctrl Pts',(-17.2073250106957,-0.192486080415645,
-21.9448455152447));
#32663=CARTESIAN_POINT('Ctrl Pts',(-17.2081516600097,-0.194217925765995,
-22.9504307734254));
#32664=CARTESIAN_POINT('Ctrl Pts',(-17.2077723489864,-0.195987817235101,
-23.5781458830157));
#32665=CARTESIAN_POINT('Ctrl Pts',(-17.207531945452,-0.196779858340764,
-23.8262844322728));
#32666=CARTESIAN_POINT('Ctrl Pts',(-17.2068115037894,-0.198739021591868,
-24.3238297132593));
#32667=CARTESIAN_POINT('Ctrl Pts',(-17.2049496914524,-0.203003236988368,
-25.1969032515018));
#32668=CARTESIAN_POINT('Ctrl Pts',(-17.2013628141071,-0.21087970254429,
-26.4501042965554));
#32669=CARTESIAN_POINT('Ctrl Pts',(-17.1966376310898,-0.220641929842346,
-27.9594600939016));
#32670=CARTESIAN_POINT('Ctrl Pts',(-17.1947174123027,-0.225915093926835,
-28.9669128292201));
#32671=CARTESIAN_POINT('Ctrl Pts',(-17.1941033398868,-0.228011167691387,
-29.5330458281712));
#32672=CARTESIAN_POINT('Ctrl Pts',(-17.1940103235576,-0.228509201821878,
-29.6568748700719));
#32673=CARTESIAN_POINT('Ctrl Pts',(-17.1940415331691,-0.22968414567057,
-29.9059782896191));
#32674=CARTESIAN_POINT('Ctrl Pts',(-17.1946196742512,-0.232137119393154,
-30.3421046429563));
#32675=CARTESIAN_POINT('Ctrl Pts',(-17.1973975961259,-0.238217812899528,
-31.2177721129568));
#32676=CARTESIAN_POINT('Ctrl Pts',(-17.2023621216832,-0.245855180371747,
-32.2244667020336));
#32677=CARTESIAN_POINT('Ctrl Pts',(-17.2051791592324,-0.250277943790212,
-33.2363333375358));
#32678=CARTESIAN_POINT('Ctrl Pts',(-17.2052435872608,-0.250996682862532,
-33.99745418694));
#32679=CARTESIAN_POINT('Ctrl Pts',(-17.2023928576229,-0.248121563635076,
-34.7605998167641));
#32680=CARTESIAN_POINT('Ctrl Pts',(-17.1978710785691,-0.243111695047323,
-35.2705175595103));
#32681=CARTESIAN_POINT('Ctrl Pts',(-17.1932447017443,-0.237922214682433,
-35.6544712301579));
#32682=CARTESIAN_POINT('Ctrl Pts',(-17.189572689603,-0.233756496190182,
-35.9138599889488));
#32683=CARTESIAN_POINT('Ctrl Pts',(-17.1801995897282,-0.223079963618858,
-36.4288669924271));
#32684=CARTESIAN_POINT('Ctrl Pts',(-17.1591257574078,-0.198762387458058,
-37.3248896233205));
#32685=CARTESIAN_POINT('Ctrl Pts',(-17.1043112841144,-0.134136510171068,
-39.0948524820125));
#32686=CARTESIAN_POINT('Ctrl Pts',(-17.055677831133,-0.0715788885984206,
-40.5774563651269));
#32687=CARTESIAN_POINT('Ctrl Pts',(-17.039939163976,-0.0473933387138723,
-41.676723963463));
#32688=CARTESIAN_POINT('Ctrl Pts',(-17.0368530908193,-0.0436179589478702,
-41.9105485570633));
#32689=CARTESIAN_POINT('Ctrl Pts',(-17.0331788357747,-0.0410479343042623,
-42.2702794698711));
#32690=CARTESIAN_POINT('Ctrl Pts',(-17.0303848046245,-0.041194751765132,
-42.6322830520466));
#32691=CARTESIAN_POINT('Ctrl Pts',(-17.0276749280209,-0.0441037814641113,
-43.1211740281135));
#32692=CARTESIAN_POINT('Ctrl Pts',(-17.0259722716986,-0.051378215425189,
-43.7416256933687));
#32693=CARTESIAN_POINT('Ctrl Pts',(-17.0257955214629,-0.0606767901658299,
-44.5013944238914));
#32694=CARTESIAN_POINT('Ctrl Pts',(-17.0265207254421,-0.0642878465005962,
-45.1464567264756));
#32695=CARTESIAN_POINT('Ctrl Pts',(-17.0273584080279,-0.061868937121287,
-45.6697526773922));
#32696=CARTESIAN_POINT('Ctrl Pts',(-17.0279500941828,-0.0565894168579634,
-46.0656376499745));
#32697=CARTESIAN_POINT('Ctrl Pts',(-17.0284130754296,-0.0470726749227195,
-46.4649407204044));
#32698=CARTESIAN_POINT('Ctrl Pts',(-17.0287785102378,-0.027711324519983,
-47.0017778071796));
#32699=CARTESIAN_POINT('Ctrl Pts',(-17.0284489638891,-0.00433057001500467,
-47.409310418673));
#32700=CARTESIAN_POINT('Ctrl Pts',(-17.0277061342787,0.026533196437943,
-47.820450921256));
#32701=CARTESIAN_POINT('Ctrl Pts',(-17.0272980415244,0.04630747610463,-48.0746939995828));
#32702=CARTESIAN_POINT('Ctrl Pts',(-17.0267681470394,0.0898860246021606,
-48.5966914106082));
#32703=CARTESIAN_POINT('Ctrl Pts',(-17.0264136197667,0.174680315576811,
-49.507451228005));
#32704=CARTESIAN_POINT('Ctrl Pts',(-17.0263194698604,0.326520770084301,
-50.8215873882974));
#32705=CARTESIAN_POINT('Ctrl Pts',(-17.0244732262949,0.571748883938012,
-52.4101266340064));
#32706=CARTESIAN_POINT('Ctrl Pts',(-17.019680884052,0.787993337413998,-53.4770518292365));
#32707=CARTESIAN_POINT('Ctrl Pts',(-17.0152049765085,0.943054767162755,
-54.1469480985672));
#32708=CARTESIAN_POINT('Ctrl Pts',(-17.0132158520225,1.00675878632521,-54.4147385821911));
#32709=CARTESIAN_POINT('Ctrl Pts',(-17.0084771905012,1.14111853808085,-54.9509279640968));
#32710=CARTESIAN_POINT('Ctrl Pts',(-16.9984395285394,1.39294874261741,-55.8861129023711));
#32711=CARTESIAN_POINT('Ctrl Pts',(-16.973683877416,1.96030674557442,-57.745888315172));
#32712=CARTESIAN_POINT('Ctrl Pts',(-16.9517208177551,2.54171784587128,-59.3129141111068));
#32713=CARTESIAN_POINT('Ctrl Pts',(-16.9425566585775,2.98804610390464,-60.4072064077515));
#32714=CARTESIAN_POINT('Ctrl Pts',(-16.9414412312354,3.04585547552463,-60.5471782172652));
#32715=CARTESIAN_POINT('Ctrl Pts',(-16.9393064923459,3.16197853912094,-60.8217554937349));
#32716=CARTESIAN_POINT('Ctrl Pts',(-16.9357919546893,3.37142078514763,-61.3011519121273));
#32717=CARTESIAN_POINT('Ctrl Pts',(-16.9295918848644,3.80832828880345,-62.2456574911334));
#32718=CARTESIAN_POINT('Ctrl Pts',(-16.9242940338859,4.33788660464919,-63.2977932858732));
#32719=CARTESIAN_POINT('Ctrl Pts',(-16.9201929569173,4.8726619443111,-64.3200099674657));
#32720=CARTESIAN_POINT('Ctrl Pts',(-16.9182376614387,5.17106378403726,-64.8834056112915));
#32721=CARTESIAN_POINT('Ctrl Pts',(-16.9170492480065,5.36707898374819,-65.2537774280137));
#32722=CARTESIAN_POINT('Ctrl Pts',(-16.9162791853453,5.4968614910262,-65.4992648282184));
#32723=CARTESIAN_POINT('Ctrl Pts',(-16.9155642280653,5.62511071424056,-65.7426262959858));
#32724=CARTESIAN_POINT('Ctrl Pts',(-16.9149560935067,5.73566048116463,-65.9535571297107));
#32725=CARTESIAN_POINT('Ctrl Pts',(-16.9146160876875,5.79830681867362,-66.0735058527206));
#32726=CARTESIAN_POINT('Ctrl Pts',(-16.9141117770561,5.89173625215646,-66.2528507981329));
#32727=CARTESIAN_POINT('Ctrl Pts',(-16.9137145858612,5.96838687667906,-66.4010494961629));
#32728=CARTESIAN_POINT('Ctrl Pts',(-16.9130609416537,6.09363292623985,-66.6449889221048));
#32729=CARTESIAN_POINT('Ctrl Pts',(-16.9124754105693,6.23087155580065,-66.9111670250714));
#32730=CARTESIAN_POINT('Ctrl Pts',(-16.9116001717781,6.50058807743624,-67.4301500253597));
#32731=CARTESIAN_POINT('Ctrl Pts',(-16.9108116823416,6.97391496129387,-68.3314415541294));
#32732=CARTESIAN_POINT('Ctrl Pts',(-16.9113899890333,7.91445730841173,-70.0927851753583));
#32733=CARTESIAN_POINT('Ctrl Pts',(-16.9134592054242,8.71297949991766,-71.5685144368547));
#32734=CARTESIAN_POINT('Ctrl Pts',(-16.9134782723112,9.30706797837199,-72.6860024639261));
#32735=CARTESIAN_POINT('Ctrl Pts',(-16.9134755702942,9.44092506181541,-72.9377664497756));
#32736=CARTESIAN_POINT('Ctrl Pts',(-16.913473633529,9.70769196988074,-73.4395108223667));
#32737=CARTESIAN_POINT('Ctrl Pts',(-16.9134806352122,10.0413473332645,-74.0670656031285));
#32738=CARTESIAN_POINT('Ctrl Pts',(-16.9134848785104,10.441325488255,-74.8193285939959));
#32739=CARTESIAN_POINT('Ctrl Pts',(-16.9134974165686,11.2411072259944,-76.3235025515291));
#32740=CARTESIAN_POINT('Ctrl Pts',(-16.9135408055664,11.9072850484377,-77.5764491734321));
#32741=CARTESIAN_POINT('Ctrl Pts',(-16.9135615147347,12.8771726655419,-79.4005966696148));
#32742=CARTESIAN_POINT('Ctrl Pts',(-16.9135721726838,13.3137342085495,-80.2216774052325));
#32743=CARTESIAN_POINT('Ctrl Pts',(-16.9135721726839,13.7502557959389,-81.0426551073307));
#32744=CARTESIAN_POINT('Ctrl Pts',(-15.0340696487865,-0.000210821217461291,
24.8306350086551));
#32745=CARTESIAN_POINT('Ctrl Pts',(-15.0341145257418,-0.000210843949456753,
24.7817557045308));
#32746=CARTESIAN_POINT('Ctrl Pts',(-15.0341615944517,-0.000210872430609927,
24.7328775245175));
#32747=CARTESIAN_POINT('Ctrl Pts',(-15.034717309544,-0.000210997311721509,
24.1822671849837));
#32748=CARTESIAN_POINT('Ctrl Pts',(-15.0351415677414,-0.000210036235135822,
23.1781123136946));
#32749=CARTESIAN_POINT('Ctrl Pts',(-15.0361299132171,-0.000210786122590035,
21.1695117270465));
#32750=CARTESIAN_POINT('Ctrl Pts',(-15.0398270933617,-0.000209397903320249,
19.6653103377228));
#32751=CARTESIAN_POINT('Ctrl Pts',(-15.0476763535126,-0.000211290125626849,
18.4142404576199));
#32752=CARTESIAN_POINT('Ctrl Pts',(-15.0514406999345,-0.000212723869813204,
17.9114214084088));
#32753=CARTESIAN_POINT('Ctrl Pts',(-15.0608925135565,-0.000216077529731644,
16.9074183611299));
#32754=CARTESIAN_POINT('Ctrl Pts',(-15.0811667598752,-0.000224215406749858,
15.1535926470682));
#32755=CARTESIAN_POINT('Ctrl Pts',(-15.1004296936536,-0.000224600233301203,
13.6517348544103));
#32756=CARTESIAN_POINT('Ctrl Pts',(-15.112515932568,-0.000224155863509205,
12.3972032802743));
#32757=CARTESIAN_POINT('Ctrl Pts',(-15.1174586204932,-0.000224715802731574,
11.8962330298534));
#32758=CARTESIAN_POINT('Ctrl Pts',(-15.1275381508422,-0.000223899547587101,
10.894368074858));
#32759=CARTESIAN_POINT('Ctrl Pts',(-15.1449930229432,-0.000222875154932196,
9.14071542262987));
#32760=CARTESIAN_POINT('Ctrl Pts',(-15.1572362388009,-0.000202554275669931,
7.63540656559452));
#32761=CARTESIAN_POINT('Ctrl Pts',(-15.1626756856597,-0.000193665754207598,
6.50379563471612));
#32762=CARTESIAN_POINT('Ctrl Pts',(-15.1633713553078,0.000401434165705328,
6.24603324501292));
#32763=CARTESIAN_POINT('Ctrl Pts',(-15.1630692903181,0.00352516011666141,
5.73674929179688));
#32764=CARTESIAN_POINT('Ctrl Pts',(-15.1589762101693,0.0128138667348422,
4.84803318861574));
#32765=CARTESIAN_POINT('Ctrl Pts',(-15.1436218457689,0.0375658550561563,
3.09396402820915));
#32766=CARTESIAN_POINT('Ctrl Pts',(-15.1422991151934,0.0370420676052799,
1.63422915566954));
#32767=CARTESIAN_POINT('Ctrl Pts',(-15.1698636910876,-0.000984415113118122,
0.629751746190038));
#32768=CARTESIAN_POINT('Ctrl Pts',(-15.1734444074368,-0.00581318203249671,
0.51323032427116));
#32769=CARTESIAN_POINT('Ctrl Pts',(-15.1817096352969,-0.0170453275908212,
0.277362288633637));
#32770=CARTESIAN_POINT('Ctrl Pts',(-15.1988795725625,-0.0403918395228711,
-0.136893473663548));
#32771=CARTESIAN_POINT('Ctrl Pts',(-15.2300183738483,-0.0828742763000551,
-0.736456418724525));
#32772=CARTESIAN_POINT('Ctrl Pts',(-15.274431671662,-0.14357994765381,-1.46782575099239));
#32773=CARTESIAN_POINT('Ctrl Pts',(-15.338283327315,-0.23092306394781,-2.45974486050588));
#32774=CARTESIAN_POINT('Ctrl Pts',(-15.4179285166044,-0.340180783742031,
-3.7316228060576));
#32775=CARTESIAN_POINT('Ctrl Pts',(-15.463058609532,-0.403833363193915,
-4.78418508811165));
#32776=CARTESIAN_POINT('Ctrl Pts',(-15.479901874256,-0.429108529628997,
-5.45306890189568));
#32777=CARTESIAN_POINT('Ctrl Pts',(-15.4858622096508,-0.438063691875341,
-5.71135488848376));
#32778=CARTESIAN_POINT('Ctrl Pts',(-15.4952017506763,-0.453072758781202,
-6.23156910938738));
#32779=CARTESIAN_POINT('Ctrl Pts',(-15.5053595039547,-0.472016689866684,
-7.13537326829117));
#32780=CARTESIAN_POINT('Ctrl Pts',(-15.506211843786,-0.483114774661327,
-8.41610862916057));
#32781=CARTESIAN_POINT('Ctrl Pts',(-15.4990448698447,-0.484040471410166,
-9.6776078698402));
#32782=CARTESIAN_POINT('Ctrl Pts',(-15.4950833952651,-0.484882331836825,
-10.5498451372121));
#32783=CARTESIAN_POINT('Ctrl Pts',(-15.4938652554776,-0.486172211228457,
-11.0448123107463));
#32784=CARTESIAN_POINT('Ctrl Pts',(-15.4937284111205,-0.487212411291013,
-11.2911040176186));
#32785=CARTESIAN_POINT('Ctrl Pts',(-15.4938501089971,-0.488192194439701,
-11.4762353961436));
#32786=CARTESIAN_POINT('Ctrl Pts',(-15.4939127005871,-0.488825135949953,
-11.6039934931571));
#32787=CARTESIAN_POINT('Ctrl Pts',(-15.4939510398894,-0.489929912388259,
-11.8572340996596));
#32788=CARTESIAN_POINT('Ctrl Pts',(-15.4938086869916,-0.49148328892933,
-12.3004477072361));
#32789=CARTESIAN_POINT('Ctrl Pts',(-15.4925012109195,-0.493701376635383,
-13.4350955010258));
#32790=CARTESIAN_POINT('Ctrl Pts',(-15.4891073643623,-0.49213447753875,
-14.6867391068569));
#32791=CARTESIAN_POINT('Ctrl Pts',(-15.486293576516,-0.490119048938007,
-15.9375432059456));
#32792=CARTESIAN_POINT('Ctrl Pts',(-15.4852325972702,-0.489277658623344,
-16.5635934600252));
#32793=CARTESIAN_POINT('Ctrl Pts',(-15.4847213819187,-0.488889211225351,
-17.065228188401));
#32794=CARTESIAN_POINT('Ctrl Pts',(-15.4845974520452,-0.488816016851646,
-17.316390296355));
#32795=CARTESIAN_POINT('Ctrl Pts',(-15.4845624417368,-0.488818430391284,
-17.5041561557632));
#32796=CARTESIAN_POINT('Ctrl Pts',(-15.4845605084085,-0.488813854935621,
-17.6289594914254));
#32797=CARTESIAN_POINT('Ctrl Pts',(-15.4846357561806,-0.488781645831683,
-17.8782617656739));
#32798=CARTESIAN_POINT('Ctrl Pts',(-15.4848197730921,-0.488717003757751,
-18.1278185570752));
#32799=CARTESIAN_POINT('Ctrl Pts',(-15.4850956191003,-0.488627896471198,
-18.3774196991142));
#32800=CARTESIAN_POINT('Ctrl Pts',(-15.4853021884926,-0.48856290194664,
-18.5334870841398));
#32801=CARTESIAN_POINT('Ctrl Pts',(-15.4854858266379,-0.48850631211949,
-18.6583654216715));
#32802=CARTESIAN_POINT('Ctrl Pts',(-15.4856808325107,-0.488446790050174,
-18.783266238916));
#32803=CARTESIAN_POINT('Ctrl Pts',(-15.4862618105197,-0.488272898475504,
-19.1268260250996));
#32804=CARTESIAN_POINT('Ctrl Pts',(-15.487416933585,-0.487940562173684,
-19.6894910265984));
#32805=CARTESIAN_POINT('Ctrl Pts',(-15.4896816665822,-0.487363835529118,
-20.6912070174202));
#32806=CARTESIAN_POINT('Ctrl Pts',(-15.4921467801256,-0.486910225703765,
-21.946226880138));
#32807=CARTESIAN_POINT('Ctrl Pts',(-15.4922291859508,-0.487421197561042,
-22.9536208320778));
#32808=CARTESIAN_POINT('Ctrl Pts',(-15.4911855039851,-0.488171590611569,
-23.582669839668));
#32809=CARTESIAN_POINT('Ctrl Pts',(-15.4906590900156,-0.488520922739212,
-23.8315946634435));
#32810=CARTESIAN_POINT('Ctrl Pts',(-15.4892167417865,-0.489406629375772,
-24.3303557486252));
#32811=CARTESIAN_POINT('Ctrl Pts',(-15.485795202301,-0.491377665390427,
-25.2051694330726));
#32812=CARTESIAN_POINT('Ctrl Pts',(-15.479157002439,-0.495019484766462,
-26.4594627009045));
#32813=CARTESIAN_POINT('Ctrl Pts',(-15.4707510145125,-0.499469758305157,
-27.9680031668306));
#32814=CARTESIAN_POINT('Ctrl Pts',(-15.4665564296506,-0.501764663321334,
-28.9735615475648));
#32815=CARTESIAN_POINT('Ctrl Pts',(-15.4650261259966,-0.502651525309478,
-29.5380529341808));
#32816=CARTESIAN_POINT('Ctrl Pts',(-15.4647905618725,-0.502970120966628,
-29.6594213057265));
#32817=CARTESIAN_POINT('Ctrl Pts',(-15.46471593299,-0.504074559115558,-29.9052068360382));
#32818=CARTESIAN_POINT('Ctrl Pts',(-15.4655271857808,-0.507104822699974,
-30.3358816568284));
#32819=CARTESIAN_POINT('Ctrl Pts',(-15.4701084649425,-0.516544753536145,
-31.2050201931821));
#32820=CARTESIAN_POINT('Ctrl Pts',(-15.4784576095206,-0.530407269101178,
-32.2128483187638));
#32821=CARTESIAN_POINT('Ctrl Pts',(-15.4825296956784,-0.537652201710911,
-33.2347909521993));
#32822=CARTESIAN_POINT('Ctrl Pts',(-15.4815887421991,-0.537269746738212,
-34.0078583156326));
#32823=CARTESIAN_POINT('Ctrl Pts',(-15.4747982556546,-0.528507549680347,
-34.7874935349868));
#32824=CARTESIAN_POINT('Ctrl Pts',(-15.4650828361564,-0.515241059459426,
-35.3114265018969));
#32825=CARTESIAN_POINT('Ctrl Pts',(-15.4553238411324,-0.501698729642147,
-35.7072440104675));
#32826=CARTESIAN_POINT('Ctrl Pts',(-15.4475606882035,-0.490722023148797,
-35.9784948813668));
#32827=CARTESIAN_POINT('Ctrl Pts',(-15.4279351556162,-0.462963031630886,
-36.5119195277882));
#32828=CARTESIAN_POINT('Ctrl Pts',(-15.3843101231493,-0.40092723253623,
-37.4342446096674));
#32829=CARTESIAN_POINT('Ctrl Pts',(-15.2718006860811,-0.239170262616976,
-39.2262614686388));
#32830=CARTESIAN_POINT('Ctrl Pts',(-15.1742119209602,-0.0943688510220052,
-40.6745248011419));
#32831=CARTESIAN_POINT('Ctrl Pts',(-15.1433506285053,-0.0457555244295182,
-41.7210473027235));
#32832=CARTESIAN_POINT('Ctrl Pts',(-15.1372456044953,-0.0370431808461871,
-41.9494258875079));
#32833=CARTESIAN_POINT('Ctrl Pts',(-15.1300553792688,-0.0285684953548626,
-42.2990803123208));
#32834=CARTESIAN_POINT('Ctrl Pts',(-15.1246437573577,-0.0242103880382995,
-42.6529450614386));
#32835=CARTESIAN_POINT('Ctrl Pts',(-15.1195490929288,-0.0228952361957256,
-43.1316637113185));
#32836=CARTESIAN_POINT('Ctrl Pts',(-15.1166812517057,-0.0279587687423588,
-43.7419250921212));
#32837=CARTESIAN_POINT('Ctrl Pts',(-15.117316613805,-0.0385683079696591,
-44.4929517663402));
#32838=CARTESIAN_POINT('Ctrl Pts',(-15.1199844499608,-0.0456198942806182,
-45.1337752418407));
#32839=CARTESIAN_POINT('Ctrl Pts',(-15.1226575630422,-0.0465603840325312,
-45.6554805491814));
#32840=CARTESIAN_POINT('Ctrl Pts',(-15.1247395447071,-0.0439822094079027,
-46.0510733259666));
#32841=CARTESIAN_POINT('Ctrl Pts',(-15.1267099246971,-0.0371484216702725,
-46.4509914011933));
#32842=CARTESIAN_POINT('Ctrl Pts',(-15.1289391518283,-0.0210245151836314,
-46.9898517547243));
#32843=CARTESIAN_POINT('Ctrl Pts',(-15.1298649672635,0.000485826508328478,
-47.4002758033805));
#32844=CARTESIAN_POINT('Ctrl Pts',(-15.1299281441084,0.030449471970366,
-47.8150612254708));
#32845=CARTESIAN_POINT('Ctrl Pts',(-15.1301783436448,0.0490313999239923,
-48.0659849956426));
#32846=CARTESIAN_POINT('Ctrl Pts',(-15.1314065155196,0.0897518029660117,
-48.5852232398212));
#32847=CARTESIAN_POINT('Ctrl Pts',(-15.1351320722241,0.167897705960403,
-49.4908701828698));
#32848=CARTESIAN_POINT('Ctrl Pts',(-15.1430849163375,0.307470878327013,
-50.8028655589996));
#32849=CARTESIAN_POINT('Ctrl Pts',(-15.1508412363502,0.539435350524335,
-52.3947240716309));
#32850=CARTESIAN_POINT('Ctrl Pts',(-15.1506480567004,0.751131888791374,
-53.4682817329514));
#32851=CARTESIAN_POINT('Ctrl Pts',(-15.1476109567481,0.905912498453314,
-54.1433711240342));
#32852=CARTESIAN_POINT('Ctrl Pts',(-15.1461202952764,0.969433044413928,
-54.4122310142868));
#32853=CARTESIAN_POINT('Ctrl Pts',(-15.142109011906,1.10399607711384,-54.9508340108951));
#32854=CARTESIAN_POINT('Ctrl Pts',(-15.1327556378678,1.35716166152049,-55.8892951044509));
#32855=CARTESIAN_POINT('Ctrl Pts',(-15.1073672179884,1.93029757933884,-57.753246710139));
#32856=CARTESIAN_POINT('Ctrl Pts',(-15.083216275239,2.51865994279119,-59.3197411843726));
#32857=CARTESIAN_POINT('Ctrl Pts',(-15.0731431840729,2.96744566208701,-60.4121663185723));
#32858=CARTESIAN_POINT('Ctrl Pts',(-15.0718837363928,3.02578692306643,-60.5524387601586));
#32859=CARTESIAN_POINT('Ctrl Pts',(-15.0694481839692,3.14288176895106,-60.8272805211502));
#32860=CARTESIAN_POINT('Ctrl Pts',(-15.065320652537,3.35419364121946,-61.3072037551322));
#32861=CARTESIAN_POINT('Ctrl Pts',(-15.0576778829909,3.79504838543236,-62.2523204944424));
#32862=CARTESIAN_POINT('Ctrl Pts',(-15.050338429514,4.32946696887476,-63.3045514635493));
#32863=CARTESIAN_POINT('Ctrl Pts',(-15.0443029598303,4.86848074759074,-64.3262573936111));
#32864=CARTESIAN_POINT('Ctrl Pts',(-15.0413660979999,5.16889192858953,-64.8891493786111));
#32865=CARTESIAN_POINT('Ctrl Pts',(-15.039590403758,5.36604126182675,-65.2590864213906));
#32866=CARTESIAN_POINT('Ctrl Pts',(-15.0384540513163,5.4965130215108,-65.5042581947861));
#32867=CARTESIAN_POINT('Ctrl Pts',(-15.0373902749899,5.62537760635623,-65.7472584806305));
#32868=CARTESIAN_POINT('Ctrl Pts',(-15.0365197826222,5.73636055026298,-65.9578371846317));
#32869=CARTESIAN_POINT('Ctrl Pts',(-15.0360397843803,5.79922704441969,-66.0775731162684));
#32870=CARTESIAN_POINT('Ctrl Pts',(-15.0353370564175,5.89295702670228,-66.2565875810318));
#32871=CARTESIAN_POINT('Ctrl Pts',(-15.0347884103062,5.96980765329387,-66.404481691943));
#32872=CARTESIAN_POINT('Ctrl Pts',(-15.0339269335575,6.09528802680313,-66.6478866046348));
#32873=CARTESIAN_POINT('Ctrl Pts',(-15.033147894299,6.23279681431226,-66.9136268045961));
#32874=CARTESIAN_POINT('Ctrl Pts',(-15.0319847166712,6.50279848479195,-67.431768557194));
#32875=CARTESIAN_POINT('Ctrl Pts',(-15.030883245086,6.97621744887788,-68.3318284641148));
#32876=CARTESIAN_POINT('Ctrl Pts',(-15.0315271538091,7.91561157226374,-70.091628231057));
#32877=CARTESIAN_POINT('Ctrl Pts',(-15.0340468472341,8.71293629115863,-71.5676334552757));
#32878=CARTESIAN_POINT('Ctrl Pts',(-15.034013342273,9.30764415560229,-72.6861482880389));
#32879=CARTESIAN_POINT('Ctrl Pts',(-15.0340065308162,9.44146712074772,-72.9378378628493));
#32880=CARTESIAN_POINT('Ctrl Pts',(-15.0339964645219,9.70825955523391,-73.4396095072806));
#32881=CARTESIAN_POINT('Ctrl Pts',(-15.0339906484446,10.0419117529944,-74.0671244842568));
#32882=CARTESIAN_POINT('Ctrl Pts',(-15.0339903349211,10.4418952801368,-74.8193852863724));
#32883=CARTESIAN_POINT('Ctrl Pts',(-15.034000079842,11.2416696930003,-76.3235367360246));
#32884=CARTESIAN_POINT('Ctrl Pts',(-15.0340231534456,11.9078687631932,-77.5764650361812));
#32885=CARTESIAN_POINT('Ctrl Pts',(-15.0340251082683,12.8777820837011,-79.4006095900798));
#32886=CARTESIAN_POINT('Ctrl Pts',(-15.0340261179702,13.3143507467422,-80.2216773228945));
#32887=CARTESIAN_POINT('Ctrl Pts',(-15.0340261179702,13.7508723341316,-81.0426550249928));
#32888=CARTESIAN_POINT('Ctrl Pts',(-13.1551501085346,0.000334283317693157,
24.8306343036982));
#32889=CARTESIAN_POINT('Ctrl Pts',(-13.1551893734422,0.000334288576141201,
24.7817549764308));
#32890=CARTESIAN_POINT('Ctrl Pts',(-13.1552305486304,0.000334309069330346,
24.732876823539));
#32891=CARTESIAN_POINT('Ctrl Pts',(-13.1557170169322,0.000333869307825757,
24.1822645064593));
#32892=CARTESIAN_POINT('Ctrl Pts',(-13.1560904963607,0.000329952799201668,
23.1780950644636));
#32893=CARTESIAN_POINT('Ctrl Pts',(-13.1569561071082,0.000330340267912158,
21.1694924498549));
#32894=CARTESIAN_POINT('Ctrl Pts',(-13.1601960309673,0.000320300549670185,
19.6652554863826));
#32895=CARTESIAN_POINT('Ctrl Pts',(-13.1670648392222,0.000315420358113045,
18.4141701152996));
#32896=CARTESIAN_POINT('Ctrl Pts',(-13.1703583133568,0.000314645245098799,
17.911347262654));
#32897=CARTESIAN_POINT('Ctrl Pts',(-13.1786284036948,0.000311635286896385,
16.9073331364927));
#32898=CARTESIAN_POINT('Ctrl Pts',(-13.1963663451238,0.000308308368792227,
15.1534970060382));
#32899=CARTESIAN_POINT('Ctrl Pts',(-13.2132280020023,0.000282947619664433,
13.6515624916615));
#32900=CARTESIAN_POINT('Ctrl Pts',(-13.2238045208785,0.000267953770380593,
12.3969987794564));
#32901=CARTESIAN_POINT('Ctrl Pts',(-13.2281281999324,0.000264653615848435,
11.8960199930155));
#32902=CARTESIAN_POINT('Ctrl Pts',(-13.2369467167224,0.000252238528283899,
10.8941480683364));
#32903=CARTESIAN_POINT('Ctrl Pts',(-13.2522139598646,0.000235521042924121,
9.1404079120666));
#32904=CARTESIAN_POINT('Ctrl Pts',(-13.2629486208776,0.000157953311529688,
7.63506274647202));
#32905=CARTESIAN_POINT('Ctrl Pts',(-13.2677164336163,0.000130044779467958,
6.5028757710561));
#32906=CARTESIAN_POINT('Ctrl Pts',(-13.2681176025061,0.00126267364318012,
6.23854702865849));
#32907=CARTESIAN_POINT('Ctrl Pts',(-13.2667638439163,0.00719521979917226,
5.72215032975373));
#32908=CARTESIAN_POINT('Ctrl Pts',(-13.2599284214127,0.0246871106678599,
4.82449852059114));
#32909=CARTESIAN_POINT('Ctrl Pts',(-13.2378016283123,0.0708993897733014,
3.07581123919757));
#32910=CARTESIAN_POINT('Ctrl Pts',(-13.2367589129128,0.0686478918711237,
1.6571204667629));
#32911=CARTESIAN_POINT('Ctrl Pts',(-13.2749785132875,0.000629895584349044,
0.70032287348691));
#32912=CARTESIAN_POINT('Ctrl Pts',(-13.2799367989849,-0.00777849232495627,
0.592200628888257));
#32913=CARTESIAN_POINT('Ctrl Pts',(-13.2913797621347,-0.0275861271661714,
0.370450620181562));
#32914=CARTESIAN_POINT('Ctrl Pts',(-13.3151282376604,-0.068962804676975,
-0.0208960537362408));
#32915=CARTESIAN_POINT('Ctrl Pts',(-13.3581349865091,-0.14539257342901,
-0.595770614284169));
#32916=CARTESIAN_POINT('Ctrl Pts',(-13.4192403351803,-0.256485334484831,
-1.30926981255708));
#32917=CARTESIAN_POINT('Ctrl Pts',(-13.5070022246835,-0.419351414251861,
-2.2930728602858));
#32918=CARTESIAN_POINT('Ctrl Pts',(-13.6164651099767,-0.628546828230703,
-3.58331904027932));
#32919=CARTESIAN_POINT('Ctrl Pts',(-13.6794191786112,-0.75494668425885,
-4.67998105132848));
#32920=CARTESIAN_POINT('Ctrl Pts',(-13.7034053121075,-0.805364352070461,
-5.38531907968524));
#32921=CARTESIAN_POINT('Ctrl Pts',(-13.711812253373,-0.82264389406825,-5.65011752865608));
#32922=CARTESIAN_POINT('Ctrl Pts',(-13.7253016587713,-0.851689010827571,
-6.18616764618947));
#32923=CARTESIAN_POINT('Ctrl Pts',(-13.7407257068587,-0.88773407989656,
-7.11147181124667));
#32924=CARTESIAN_POINT('Ctrl Pts',(-13.7449258328838,-0.907719595052291,
-8.41317522414356));
#32925=CARTESIAN_POINT('Ctrl Pts',(-13.7384418678751,-0.908107987950047,
-9.68045569583018));
#32926=CARTESIAN_POINT('Ctrl Pts',(-13.7348891547529,-0.90901605019472,
-10.5493544319712));
#32927=CARTESIAN_POINT('Ctrl Pts',(-13.7340705601867,-0.911173060866272,
-11.0401724781861));
#32928=CARTESIAN_POINT('Ctrl Pts',(-13.7342181547962,-0.913040175168312,
-11.2836385676462));
#32929=CARTESIAN_POINT('Ctrl Pts',(-13.734595811174,-0.914830641973323,
-11.4664445586127));
#32930=CARTESIAN_POINT('Ctrl Pts',(-13.7348265495321,-0.916019414652225,
-11.5955414439621));
#32931=CARTESIAN_POINT('Ctrl Pts',(-13.7351468223391,-0.918096161386488,
-11.8497587471897));
#32932=CARTESIAN_POINT('Ctrl Pts',(-13.7353808308897,-0.921076812804577,
-12.2953368249091));
#32933=CARTESIAN_POINT('Ctrl Pts',(-13.7344944584954,-0.925632694184054,
-13.4344907253095));
#32934=CARTESIAN_POINT('Ctrl Pts',(-13.7303643879806,-0.923608185100719,
-14.6889600179318));
#32935=CARTESIAN_POINT('Ctrl Pts',(-13.7267867092688,-0.920518695146856,
-15.9397629453685));
#32936=CARTESIAN_POINT('Ctrl Pts',(-13.7254524072941,-0.919219914483102,
-16.5652138437354));
#32937=CARTESIAN_POINT('Ctrl Pts',(-13.7248363073386,-0.918615753584493,
-17.0659631831709));
#32938=CARTESIAN_POINT('Ctrl Pts',(-13.7247119123663,-0.918511435023379,
-17.3165574963283));
#32939=CARTESIAN_POINT('Ctrl Pts',(-13.7246978826119,-0.918524245907937,
-17.5038581677432));
#32940=CARTESIAN_POINT('Ctrl Pts',(-13.7247086069979,-0.918530104126422,
-17.6286329123153));
#32941=CARTESIAN_POINT('Ctrl Pts',(-13.7248036965319,-0.918530711256441,
-17.8777412014854));
#32942=CARTESIAN_POINT('Ctrl Pts',(-13.7250049145367,-0.918518178892288,
-18.1271988002274));
#32943=CARTESIAN_POINT('Ctrl Pts',(-13.7252915898653,-0.918488106487544,
-18.3767028364522));
#32944=CARTESIAN_POINT('Ctrl Pts',(-13.7255046554761,-0.918463530061787,
-18.5327310273419));
#32945=CARTESIAN_POINT('Ctrl Pts',(-13.7256927785562,-0.918439784078445,
-18.6575838103995));
#32946=CARTESIAN_POINT('Ctrl Pts',(-13.7258919014263,-0.918413320075625,
-18.7824655906309));
#32947=CARTESIAN_POINT('Ctrl Pts',(-13.7264890957503,-0.918334197338507,
-19.1259957677016));
#32948=CARTESIAN_POINT('Ctrl Pts',(-13.7276729411882,-0.918147331683812,
-19.6887422443658));
#32949=CARTESIAN_POINT('Ctrl Pts',(-13.7300976648197,-0.917698555102597,
-20.6909608145285));
#32950=CARTESIAN_POINT('Ctrl Pts',(-13.7329660445855,-0.916847221647031,
-21.9472991675568));
#32951=CARTESIAN_POINT('Ctrl Pts',(-13.7339260928259,-0.915974400434199,
-22.9564516405322));
#32952=CARTESIAN_POINT('Ctrl Pts',(-13.7335909065193,-0.91532061521922,
-23.586839406153));
#32953=CARTESIAN_POINT('Ctrl Pts',(-13.7333720459406,-0.915033425050764,
-23.8365407161973));
#32954=CARTESIAN_POINT('Ctrl Pts',(-13.7326725951122,-0.914383629983113,
-24.336514511158));
#32955=CARTESIAN_POINT('Ctrl Pts',(-13.7308173358681,-0.913067424616607,
-25.2130517805888));
#32956=CARTESIAN_POINT('Ctrl Pts',(-13.727027503321,-0.910893971946881,
-26.4684878476616));
#32957=CARTESIAN_POINT('Ctrl Pts',(-13.7219681203734,-0.908224716400938,
-27.9762313767341));
#32958=CARTESIAN_POINT('Ctrl Pts',(-13.7195680699122,-0.906809058233843,
-28.9800397373653));
#32959=CARTESIAN_POINT('Ctrl Pts',(-13.7186976728711,-0.906178401053505,
-29.5428491015415));
#32960=CARTESIAN_POINT('Ctrl Pts',(-13.7186357852207,-0.906282813123428,
-29.660789949837));
#32961=CARTESIAN_POINT('Ctrl Pts',(-13.7190115634281,-0.907362158204569,
-29.9020317928129));
#32962=CARTESIAN_POINT('Ctrl Pts',(-13.7208604212975,-0.911336577467707,
-30.325235025951));
#32963=CARTESIAN_POINT('Ctrl Pts',(-13.7282606251036,-0.925829752687878,
-31.1855963678829));
#32964=CARTESIAN_POINT('Ctrl Pts',(-13.7403872876803,-0.948982661328658,
-32.1954921925686));
#32965=CARTESIAN_POINT('Ctrl Pts',(-13.7464168159969,-0.960613228500291,
-33.23190086473));
#32966=CARTESIAN_POINT('Ctrl Pts',(-13.7453894841776,-0.958641743033242,
-34.0218962636807));
#32967=CARTESIAN_POINT('Ctrl Pts',(-13.7362878221931,-0.940841001845677,
-34.8248369835493));
#32968=CARTESIAN_POINT('Ctrl Pts',(-13.7230148534269,-0.914724221017991,
-35.3684905729439));
#32969=CARTESIAN_POINT('Ctrl Pts',(-13.7096037677254,-0.888181576735158,
-35.7809178353369));
#32970=CARTESIAN_POINT('Ctrl Pts',(-13.6987970364002,-0.866293009330416,
-36.0686926579714));
#32971=CARTESIAN_POINT('Ctrl Pts',(-13.671569771722,-0.811851434411236,
-36.6277044534425));
#32972=CARTESIAN_POINT('Ctrl Pts',(-13.6108442528254,-0.691666448454139,
-37.5865862183716));
#32973=CARTESIAN_POINT('Ctrl Pts',(-13.4543351700341,-0.38735629443809,
-39.410125440965));
#32974=CARTESIAN_POINT('Ctrl Pts',(-13.3154256245931,-0.133535009111489,
-40.8132820690543));
#32975=CARTESIAN_POINT('Ctrl Pts',(-13.2698135895045,-0.0536258159889684,
-41.7861584105223));
#32976=CARTESIAN_POINT('Ctrl Pts',(-13.2607691869315,-0.0382086490022178,
-42.0069186031658));
#32977=CARTESIAN_POINT('Ctrl Pts',(-13.249920904955,-0.0216881580641046,
-42.3424365601118));
#32978=CARTESIAN_POINT('Ctrl Pts',(-13.2415653675482,-0.0109728837688096,
-42.6848694711389));
#32979=CARTESIAN_POINT('Ctrl Pts',(-13.2333766019918,-0.0034432187711669,
-43.1493156575476));
#32980=CARTESIAN_POINT('Ctrl Pts',(-13.2280268298175,-0.00466010038720499,
-43.7453358598114));
#32981=CARTESIAN_POINT('Ctrl Pts',(-13.2272319558763,-0.0158111723549196,
-44.4842770335761));
#32982=CARTESIAN_POINT('Ctrl Pts',(-13.2294437231869,-0.0263474888916997,
-45.1193836607821));
#32983=CARTESIAN_POINT('Ctrl Pts',(-13.2319498926359,-0.0310811416053446,
-45.6390704954399));
#32984=CARTESIAN_POINT('Ctrl Pts',(-13.2338868711412,-0.0315492607015707,
-46.0344362473196));
#32985=CARTESIAN_POINT('Ctrl Pts',(-13.2356169499968,-0.0276988033612878,
-46.4354227169262));
#32986=CARTESIAN_POINT('Ctrl Pts',(-13.2373207078135,-0.0151057061868057,
-46.9774255790535));
#32987=CARTESIAN_POINT('Ctrl Pts',(-13.23740813852,0.00481574300534024,
-47.3921808544604));
#32988=CARTESIAN_POINT('Ctrl Pts',(-13.2362799960084,0.0344572958470751,
-47.8123785321966));
#32989=CARTESIAN_POINT('Ctrl Pts',(-13.2357060059805,0.0521042990666052,
-48.0591893755926));
#32990=CARTESIAN_POINT('Ctrl Pts',(-13.2351927606908,0.0904170132760224,
-48.5752630537383));
#32991=CARTESIAN_POINT('Ctrl Pts',(-13.2356915822,0.162356093353207,-49.4747201946233));
#32992=CARTESIAN_POINT('Ctrl Pts',(-13.2387758395764,0.289567892495778,
-50.7837952574958));
#32993=CARTESIAN_POINT('Ctrl Pts',(-13.2419496016628,0.506524792408763,
-52.3789559389661));
#32994=CARTESIAN_POINT('Ctrl Pts',(-13.2402837800499,0.712955021961898,
-53.4596155677194));
#32995=CARTESIAN_POINT('Ctrl Pts',(-13.2372260073496,0.867360271403418,
-54.1403451215742));
#32996=CARTESIAN_POINT('Ctrl Pts',(-13.2358187991522,0.930601816612459,
-54.4102300948697));
#32997=CARTESIAN_POINT('Ctrl Pts',(-13.2322860209069,1.06528164613938,-54.9512789187452));
#32998=CARTESIAN_POINT('Ctrl Pts',(-13.2244696261721,1.31979280601954,-55.8929368737511));
#32999=CARTESIAN_POINT('Ctrl Pts',(-13.2043422333084,1.89931808336194,-57.760958976205));
#33000=CARTESIAN_POINT('Ctrl Pts',(-13.1860395153099,2.49496689438429,-59.3266437846506));
#33001=CARTESIAN_POINT('Ctrl Pts',(-13.1786973988809,2.94640801214391,-60.4171710430611));
#33002=CARTESIAN_POINT('Ctrl Pts',(-13.1778006140846,3.00533999312714,-60.5577447895152));
#33003=CARTESIAN_POINT('Ctrl Pts',(-13.1760857276374,3.12351075972109,-60.8328452449694));
#33004=CARTESIAN_POINT('Ctrl Pts',(-13.1732576712662,3.33685108478691,-61.3132715282016));
#33005=CARTESIAN_POINT('Ctrl Pts',(-13.1682631404326,3.78194623518818,-62.2589108855292));
#33006=CARTESIAN_POINT('Ctrl Pts',(-13.1639566703889,4.32129412642347,-63.311132796502));
#33007=CARTESIAN_POINT('Ctrl Pts',(-13.1606134591638,4.86461088337284,-64.3322721484445));
#33008=CARTESIAN_POINT('Ctrl Pts',(-13.1590189299969,5.16708564585913,-64.8946512637013));
#33009=CARTESIAN_POINT('Ctrl Pts',(-13.1580495871756,5.36539495771196,-65.2641506500079));
#33010=CARTESIAN_POINT('Ctrl Pts',(-13.1574229026006,5.49658427915357,-65.5090051569745));
#33011=CARTESIAN_POINT('Ctrl Pts',(-13.1568375735826,5.62605738444092,-65.7516476611018));
#33012=CARTESIAN_POINT('Ctrl Pts',(-13.156342424908,5.73748582541207,-65.9618743170868));
#33013=CARTESIAN_POINT('Ctrl Pts',(-13.156065649456,5.80057812624236,-66.0813973232228));
#33014=CARTESIAN_POINT('Ctrl Pts',(-13.1556555185828,5.8946184745073,-66.2600804080991));
#33015=CARTESIAN_POINT('Ctrl Pts',(-13.1553306040581,5.97165884095127,-66.4076735552761));
#33016=CARTESIAN_POINT('Ctrl Pts',(-13.1547985747114,6.09737128380689,-66.6505431582039));
#33017=CARTESIAN_POINT('Ctrl Pts',(-13.1543196231653,6.23514411689466,-66.9158510378909));
#33018=CARTESIAN_POINT('Ctrl Pts',(-13.153602518776,6.50542741523817,-67.4331524864784));
#33019=CARTESIAN_POINT('Ctrl Pts',(-13.1529416894374,6.97888521210212,-68.3319968438596));
#33020=CARTESIAN_POINT('Ctrl Pts',(-13.1533756026942,7.91707121646751,-70.0902548994053));
#33021=CARTESIAN_POINT('Ctrl Pts',(-13.1550149191262,8.71301264450386,-71.5666401701622));
#33022=CARTESIAN_POINT('Ctrl Pts',(-13.1550167477829,9.30829962930597,-72.6862300805453));
#33023=CARTESIAN_POINT('Ctrl Pts',(-13.1550132987847,9.44208731458616,-72.9378417548579));
#33024=CARTESIAN_POINT('Ctrl Pts',(-13.1550094243293,9.70890149614314,-73.439640119029));
#33025=CARTESIAN_POINT('Ctrl Pts',(-13.1550116726656,10.0425338980053,-74.0671190188514));
#33026=CARTESIAN_POINT('Ctrl Pts',(-13.1550139473927,10.4425138027341,-74.8193776474128));
#33027=CARTESIAN_POINT('Ctrl Pts',(-13.1550236387193,11.2422628255351,-76.3235076738163));
#33028=CARTESIAN_POINT('Ctrl Pts',(-13.1550542350392,11.9084264257806,-77.5764481272447));
#33029=CARTESIAN_POINT('Ctrl Pts',(-13.1550663076038,12.8783378734336,-79.4006160379139));
#33030=CARTESIAN_POINT('Ctrl Pts',(-13.1550725189431,13.3148957927065,-80.2216773986545));
#33031=CARTESIAN_POINT('Ctrl Pts',(-13.1550725189431,13.751417380096,-81.0426551007529));
#33032=CARTESIAN_POINT('Ctrl Pts',(-10.650042270715,0.000365604416696912,
24.8306342582036));
#33033=CARTESIAN_POINT('Ctrl Pts',(-10.6500740847871,0.000365622567542727,
24.7817549302156));
#33034=CARTESIAN_POINT('Ctrl Pts',(-10.6501074661384,0.00036562337306155,
24.7328768714934));
#33035=CARTESIAN_POINT('Ctrl Pts',(-10.6505009657446,0.000366460923403975,
24.1822613516484));
#33036=CARTESIAN_POINT('Ctrl Pts',(-10.6507985217012,0.000371994166762139,
23.1780652609194));
#33037=CARTESIAN_POINT('Ctrl Pts',(-10.6515005557346,0.000373666904444558,
21.1694597397613));
#33038=CARTESIAN_POINT('Ctrl Pts',(-10.6541120400923,0.00038789274538446,
19.665156351013));
#33039=CARTESIAN_POINT('Ctrl Pts',(-10.6596693248198,0.000395383454766491,
18.4140420097379));
#33040=CARTESIAN_POINT('Ctrl Pts',(-10.6623360336828,0.000397268296322463,
17.9112146130549));
#33041=CARTESIAN_POINT('Ctrl Pts',(-10.6690310413239,0.000403612342891138,
16.9071816012036));
#33042=CARTESIAN_POINT('Ctrl Pts',(-10.6833946406787,0.000413304763147904,
15.1533257466147));
#33043=CARTESIAN_POINT('Ctrl Pts',(-10.6970194022592,0.000446367192448972,
13.65123967164));
#33044=CARTESIAN_POINT('Ctrl Pts',(-10.7055652765539,0.000460391626742008,
12.396604516728));
#33045=CARTESIAN_POINT('Ctrl Pts',(-10.7090622322879,0.000462138910872274,
11.8956069838844));
#33046=CARTESIAN_POINT('Ctrl Pts',(-10.71618705933,0.000470076121078105,
10.8937100869054));
#33047=CARTESIAN_POINT('Ctrl Pts',(-10.7285262732713,0.00047519876483419,
9.13982057473998));
#33048=CARTESIAN_POINT('Ctrl Pts',(-10.7371199899901,0.000549749028605339,
7.63434823533288));
#33049=CARTESIAN_POINT('Ctrl Pts',(-10.7409414889771,0.000581970750385906,
6.50124583376022));
#33050=CARTESIAN_POINT('Ctrl Pts',(-10.741125057236,0.00259570504651152,
6.2267602931048));
#33051=CARTESIAN_POINT('Ctrl Pts',(-10.7392878601745,0.0130556637491886,
5.69935608672766));
#33052=CARTESIAN_POINT('Ctrl Pts',(-10.7315460602503,0.0436541037719018,
4.78794501792968));
#33053=CARTESIAN_POINT('Ctrl Pts',(-10.7076995794509,0.122780759576109,
3.04730104516099));
#33054=CARTESIAN_POINT('Ctrl Pts',(-10.7066809728001,0.117468289823324,
1.69232053262551));
#33055=CARTESIAN_POINT('Ctrl Pts',(-10.7467593103304,0.00918488066074162,
0.807560256124786));
#33056=CARTESIAN_POINT('Ctrl Pts',(-10.7519626603441,-0.00366202002174799,
0.712117710399012));
#33057=CARTESIAN_POINT('Ctrl Pts',(-10.7639074270763,-0.0346127647497942,
0.511455864381113));
#33058=CARTESIAN_POINT('Ctrl Pts',(-10.7885508414982,-0.100020448640092,
0.153839003233626));
#33059=CARTESIAN_POINT('Ctrl Pts',(-10.8325098601214,-0.224187245889308,
-0.385975306818793));
#33060=CARTESIAN_POINT('Ctrl Pts',(-10.8945063363775,-0.411994785650364,
-1.07465867196766));
#33061=CARTESIAN_POINT('Ctrl Pts',(-10.9836120542585,-0.696313194115999,
-2.04671364700164));
#33062=CARTESIAN_POINT('Ctrl Pts',(-11.0985387251657,-1.0796369475826,-3.35899297291827));
#33063=CARTESIAN_POINT('Ctrl Pts',(-11.171886523949,-1.32333560794751,-4.51856097352981));
#33064=CARTESIAN_POINT('Ctrl Pts',(-11.2013328963089,-1.42155056846409,
-5.2797800642824));
#33065=CARTESIAN_POINT('Ctrl Pts',(-11.2111143269299,-1.45404461826559,
-5.55455206726266));
#33066=CARTESIAN_POINT('Ctrl Pts',(-11.2273042145085,-1.50896260405546,
-6.1151264956646));
#33067=CARTESIAN_POINT('Ctrl Pts',(-11.2461025439228,-1.5759155046305,-7.07410960662139));
#33068=CARTESIAN_POINT('Ctrl Pts',(-11.2526452650533,-1.61081946830704,
-8.40897150999976));
#33069=CARTESIAN_POINT('Ctrl Pts',(-11.2470489340527,-1.60877605321405,
-9.68549243928046));
#33070=CARTESIAN_POINT('Ctrl Pts',(-11.2440734077914,-1.60906768347938,
-10.5492612995141));
#33071=CARTESIAN_POINT('Ctrl Pts',(-11.2435490792222,-1.61234277070398,
-11.0336093167728));
#33072=CARTESIAN_POINT('Ctrl Pts',(-11.2438342641925,-1.61546267429326,
-11.2726534396781));
#33073=CARTESIAN_POINT('Ctrl Pts',(-11.2443128285622,-1.61853239351233,
-11.4518215569661));
#33074=CARTESIAN_POINT('Ctrl Pts',(-11.244642200452,-1.6206336095023,-11.5831336298258));
#33075=CARTESIAN_POINT('Ctrl Pts',(-11.2451027763732,-1.62425012459985,
-11.8390401722566));
#33076=CARTESIAN_POINT('Ctrl Pts',(-11.245499325149,-1.62938835686632,-12.2885988051048));
#33077=CARTESIAN_POINT('Ctrl Pts',(-11.2445889024303,-1.63684237120518,
-13.4353109170186));
#33078=CARTESIAN_POINT('Ctrl Pts',(-11.2395266498228,-1.63217918211705,
-14.6942343328465));
#33079=CARTESIAN_POINT('Ctrl Pts',(-11.2351609777683,-1.62603694400866,
-15.9445922607557));
#33080=CARTESIAN_POINT('Ctrl Pts',(-11.2334936421301,-1.62345795467893,
-16.5687429713417));
#33081=CARTESIAN_POINT('Ctrl Pts',(-11.2327225455089,-1.62227723430756,
-17.067750318547));
#33082=CARTESIAN_POINT('Ctrl Pts',(-11.2325540866687,-1.6220597987632,-17.3172482783649));
#33083=CARTESIAN_POINT('Ctrl Pts',(-11.2325261615434,-1.62207425666605,
-17.5036664428382));
#33084=CARTESIAN_POINT('Ctrl Pts',(-11.2325208137062,-1.62208351508994,
-17.6286085458311));
#33085=CARTESIAN_POINT('Ctrl Pts',(-11.2325612882407,-1.62210073370477,
-17.8776147298047));
#33086=CARTESIAN_POINT('Ctrl Pts',(-11.232671136902,-1.62211043308421,-18.1271358360374));
#33087=CARTESIAN_POINT('Ctrl Pts',(-11.232848152788,-1.62211576375874,-18.3766187541966));
#33088=CARTESIAN_POINT('Ctrl Pts',(-11.2329838221442,-1.62211513012755,
-18.5326539574177));
#33089=CARTESIAN_POINT('Ctrl Pts',(-11.2331070956596,-1.6221125896366,-18.6575054790737));
#33090=CARTESIAN_POINT('Ctrl Pts',(-11.2332395984363,-1.62210818013834,
-18.782388318556));
#33091=CARTESIAN_POINT('Ctrl Pts',(-11.2336409056025,-1.62208945476857,
-19.1259219496441));
#33092=CARTESIAN_POINT('Ctrl Pts',(-11.2344837859616,-1.6220094344919,-19.6886807661217));
#33093=CARTESIAN_POINT('Ctrl Pts',(-11.2363723866999,-1.6217009240143,-20.6909416074719));
#33094=CARTESIAN_POINT('Ctrl Pts',(-11.2391462383464,-1.62084938520113,
-21.9473557243982));
#33095=CARTESIAN_POINT('Ctrl Pts',(-11.2412312975038,-1.61952792207212,
-22.9565995393526));
#33096=CARTESIAN_POINT('Ctrl Pts',(-11.242274432361,-1.61839941643641,-23.5870517203909));
#33097=CARTESIAN_POINT('Ctrl Pts',(-11.2426925129516,-1.61789843605843,
-23.8367914647876));
#33098=CARTESIAN_POINT('Ctrl Pts',(-11.2435586956675,-1.61672265215808,
-24.3368252655553));
#33099=CARTESIAN_POINT('Ctrl Pts',(-11.2451269298127,-1.61425020271206,
-25.2134378024879));
#33100=CARTESIAN_POINT('Ctrl Pts',(-11.2475055060001,-1.60997905946445,
-26.4689342912108));
#33101=CARTESIAN_POINT('Ctrl Pts',(-11.2502268402875,-1.60463449910935,
-27.9765152999299));
#33102=CARTESIAN_POINT('Ctrl Pts',(-11.2518846690841,-1.60184316346082,
-28.9803497799525));
#33103=CARTESIAN_POINT('Ctrl Pts',(-11.2526845529141,-1.6006395775289,-29.5426879338358));
#33104=CARTESIAN_POINT('Ctrl Pts',(-11.2530016388635,-1.60081773392649,
-29.6552622230315));
#33105=CARTESIAN_POINT('Ctrl Pts',(-11.2541316907256,-1.60272031221793,
-29.8896725175522));
#33106=CARTESIAN_POINT('Ctrl Pts',(-11.2573154165258,-1.60982261583138,
-30.301540866585));
#33107=CARTESIAN_POINT('Ctrl Pts',(-11.2674452022504,-1.63593292207713,
-31.14907078036));
#33108=CARTESIAN_POINT('Ctrl Pts',(-11.2829662937318,-1.67867594116351,
-32.1631522498279));
#33109=CARTESIAN_POINT('Ctrl Pts',(-11.2915281314437,-1.70059914198832,
-33.2233457754404));
#33110=CARTESIAN_POINT('Ctrl Pts',(-11.2913372530278,-1.69702533908146,
-34.040796301399));
#33111=CARTESIAN_POINT('Ctrl Pts',(-11.2813003503381,-1.66348397111689,
-34.8810679137723));
#33112=CARTESIAN_POINT('Ctrl Pts',(-11.2656754441518,-1.61374425816922,
-35.4558609216503));
#33113=CARTESIAN_POINT('Ctrl Pts',(-11.2496371955773,-1.56284553931442,
-35.8941482820626));
#33114=CARTESIAN_POINT('Ctrl Pts',(-11.2361268189636,-1.5200304380772,-36.2072998555992));
#33115=CARTESIAN_POINT('Ctrl Pts',(-11.2033119490395,-1.41487719118908,
-36.8046955101422));
#33116=CARTESIAN_POINT('Ctrl Pts',(-11.1324504370696,-1.18653719379417,
-37.8161641760809));
#33117=CARTESIAN_POINT('Ctrl Pts',(-10.9643210506542,-0.626215933228365,
-39.6790476430707));
#33118=CARTESIAN_POINT('Ctrl Pts',(-10.8244131060971,-0.212830624883642,
-41.0275041631862));
#33119=CARTESIAN_POINT('Ctrl Pts',(-10.7745159277284,-0.0923722011974562,
-41.8913882550613));
#33120=CARTESIAN_POINT('Ctrl Pts',(-10.7644262578356,-0.0667960726337613,
-42.100774923633));
#33121=CARTESIAN_POINT('Ctrl Pts',(-10.7521055535479,-0.0383479070046453,
-42.4150659459343));
#33122=CARTESIAN_POINT('Ctrl Pts',(-10.7423454245313,-0.0176547472067045,
-42.7402413431657));
#33123=CARTESIAN_POINT('Ctrl Pts',(-10.7324271418274,2.78979527989668E-5,
-43.183176332304));
#33124=CARTESIAN_POINT('Ctrl Pts',(-10.7251377519842,0.00629930368330282,
-43.7578870145591));
#33125=CARTESIAN_POINT('Ctrl Pts',(-10.722225468076,-0.00301713781191112,
-44.4792267442436));
#33126=CARTESIAN_POINT('Ctrl Pts',(-10.7226678608004,-0.0162766379087752,
-45.1065805339814));
#33127=CARTESIAN_POINT('Ctrl Pts',(-10.723545462882,-0.0242434157495022,
-45.6240842906144));
#33128=CARTESIAN_POINT('Ctrl Pts',(-10.7241700886567,-0.0273378354607701,
-46.0198535950271));
#33129=CARTESIAN_POINT('Ctrl Pts',(-10.7244611701676,-0.0258733857197475,
-46.4232938280841));
#33130=CARTESIAN_POINT('Ctrl Pts',(-10.7240076051067,-0.0154552381350729,
-46.9712845245771));
#33131=CARTESIAN_POINT('Ctrl Pts',(-10.7222645624063,0.00459948307228258,
-47.3936546235918));
#33132=CARTESIAN_POINT('Ctrl Pts',(-10.718999108387,0.0368370176291262,
-47.8231822015646));
#33133=CARTESIAN_POINT('Ctrl Pts',(-10.7168451494989,0.0551515656315621,
-48.0659853261855));
#33134=CARTESIAN_POINT('Ctrl Pts',(-10.7126438701732,0.0947533205243461,
-48.5802163021467));
#33135=CARTESIAN_POINT('Ctrl Pts',(-10.7055740500304,0.167328769646443,
-49.4743468728569));
#33136=CARTESIAN_POINT('Ctrl Pts',(-10.696191178236,0.292518409057621,-50.7801490138078));
#33137=CARTESIAN_POINT('Ctrl Pts',(-10.685966507583,0.505539967513752,-52.3744744198876));
#33138=CARTESIAN_POINT('Ctrl Pts',(-10.6796850250947,0.710589132746706,
-53.4575886581674));
#33139=CARTESIAN_POINT('Ctrl Pts',(-10.6758902888676,0.86539535947085,-54.1404651022306));
#33140=CARTESIAN_POINT('Ctrl Pts',(-10.6743290244131,0.928589158227978,
-54.4101838213268));
#33141=CARTESIAN_POINT('Ctrl Pts',(-10.6711673120377,1.06333532993672,-54.9514724741432));
#33142=CARTESIAN_POINT('Ctrl Pts',(-10.6655572848368,1.31795469515906,-55.8932151703261));
#33143=CARTESIAN_POINT('Ctrl Pts',(-10.6545603915192,1.8979592738655,-57.7615645354719));
#33144=CARTESIAN_POINT('Ctrl Pts',(-10.6471780206085,2.49412918412692,-59.3271216575852));
#33145=CARTESIAN_POINT('Ctrl Pts',(-10.6447300416341,2.9456620163703,-60.417473751051));
#33146=CARTESIAN_POINT('Ctrl Pts',(-10.6444864734455,3.00461178774495,-60.5580565408257));
#33147=CARTESIAN_POINT('Ctrl Pts',(-10.6440810657814,3.12281208563953,-60.8331584712121));
#33148=CARTESIAN_POINT('Ctrl Pts',(-10.6436200824622,3.33621174814075,-61.313592543236));
#33149=CARTESIAN_POINT('Ctrl Pts',(-10.643538445653,3.78141483002328,-62.2592373107269));
#33150=CARTESIAN_POINT('Ctrl Pts',(-10.6448782016157,4.32092352352002,-63.3114408017025));
#33151=CARTESIAN_POINT('Ctrl Pts',(-10.6466814092829,4.86435913111074,-64.3325544290971));
#33152=CARTESIAN_POINT('Ctrl Pts',(-10.6476978523703,5.16688179322271,-64.8949195301645));
#33153=CARTESIAN_POINT('Ctrl Pts',(-10.6483022010011,5.36521976706749,-65.2644093316576));
#33154=CARTESIAN_POINT('Ctrl Pts',(-10.6486804775451,5.49642366290479,-65.5092586775464));
#33155=CARTESIAN_POINT('Ctrl Pts',(-10.6490154796418,5.62591876808531,-65.7518925194187));
#33156=CARTESIAN_POINT('Ctrl Pts',(-10.6492563188143,5.73735950919451,-65.9621141841148));
#33157=CARTESIAN_POINT('Ctrl Pts',(-10.649377241876,5.80045868759503,-66.0816343708117));
#33158=CARTESIAN_POINT('Ctrl Pts',(-10.6495408928145,5.89450845196145,-66.2603135957034));
#33159=CARTESIAN_POINT('Ctrl Pts',(-10.6496390058144,5.97156070475074,-66.4079010048767));
#33160=CARTESIAN_POINT('Ctrl Pts',(-10.6497386183767,6.09728728657649,-66.6507639951798));
#33161=CARTESIAN_POINT('Ctrl Pts',(-10.6498293290638,6.23507055885311,-66.9160539783043));
#33162=CARTESIAN_POINT('Ctrl Pts',(-10.6499677310158,6.50536736913276,-67.4333300460254));
#33163=CARTESIAN_POINT('Ctrl Pts',(-10.6501114230242,6.97884573772282,-68.3321241661668));
#33164=CARTESIAN_POINT('Ctrl Pts',(-10.6500963227376,7.91702070557873,-70.0903209123917));
#33165=CARTESIAN_POINT('Ctrl Pts',(-10.6498795836695,8.71297626916867,-71.566667654021));
#33166=CARTESIAN_POINT('Ctrl Pts',(-10.6499011960763,9.30829482662004,-72.6862697910305));
#33167=CARTESIAN_POINT('Ctrl Pts',(-10.6499047637529,9.44208195132325,-72.9378791448345));
#33168=CARTESIAN_POINT('Ctrl Pts',(-10.649910300367,9.70889818600605,-73.4396768553508));
#33169=CARTESIAN_POINT('Ctrl Pts',(-10.6499144874314,10.0425345294427,-74.0671506210093));
#33170=CARTESIAN_POINT('Ctrl Pts',(-10.6499151827135,10.442516342387,-74.8194073811515));
#33171=CARTESIAN_POINT('Ctrl Pts',(-10.6499111240893,11.2422680992346,-76.3235337653213));
#33172=CARTESIAN_POINT('Ctrl Pts',(-10.6499030565891,11.9084448061482,-77.5764608335406));
#33173=CARTESIAN_POINT('Ctrl Pts',(-10.6499043672714,12.8783648733455,-79.4006205549652));
#33174=CARTESIAN_POINT('Ctrl Pts',(-10.6499050450884,13.3149270582603,-80.2216773804913));
#33175=CARTESIAN_POINT('Ctrl Pts',(-10.6499050450884,13.7514486456498,-81.0426550825896));
#33176=CARTESIAN_POINT('Ctrl Pts',(-8.14412189745736,-0.000152373436558693,
24.8306349266468));
#33177=CARTESIAN_POINT('Ctrl Pts',(-8.14414623195988,-0.000152375382121277,
24.7817556196536));
#33178=CARTESIAN_POINT('Ctrl Pts',(-8.1441717670015,-0.000152392198849738,
24.7328776300862));
#33179=CARTESIAN_POINT('Ctrl Pts',(-8.14447269564718,-0.000151918598724809,
24.1822607486252));
#33180=CARTESIAN_POINT('Ctrl Pts',(-8.14469979318938,-0.000147878987651978,
23.1780515264225));
#33181=CARTESIAN_POINT('Ctrl Pts',(-8.14523667747614,-0.000147765295944936,
21.1694450065643));
#33182=CARTESIAN_POINT('Ctrl Pts',(-8.14723298556225,-0.000137574708599251,
19.6651083293772));
#33183=CARTESIAN_POINT('Ctrl Pts',(-8.15148329064228,-0.000132911415445355,
18.4139794726141));
#33184=CARTESIAN_POINT('Ctrl Pts',(-8.15352302280712,-0.000132173521193853,
17.9111511130494));
#33185=CARTESIAN_POINT('Ctrl Pts',(-8.15864383708089,-0.000129196754508978,
16.9071094951091));
#33186=CARTESIAN_POINT('Ctrl Pts',(-8.16963053348841,-0.000125920397975024,
15.153243554802));
#33187=CARTESIAN_POINT('Ctrl Pts',(-8.18004947280553,-0.000101684712158349,
13.6510767010308));
#33188=CARTESIAN_POINT('Ctrl Pts',(-8.18658467464386,-8.88278457007875E-5,
12.3964004428332));
#33189=CARTESIAN_POINT('Ctrl Pts',(-8.18925923233085,-8.64346045489019E-5,
11.8953895179443));
#33190=CARTESIAN_POINT('Ctrl Pts',(-8.1947078772434,-7.69523185917187E-5,
10.8934820559683));
#33191=CARTESIAN_POINT('Ctrl Pts',(-8.20414480257374,-6.48462924612067E-5,
9.13949375918252));
#33192=CARTESIAN_POINT('Ctrl Pts',(-8.2107091480591,2.93700242304431E-6,
7.63402123554715));
#33193=CARTESIAN_POINT('Ctrl Pts',(-8.21362816021825,3.46121833831947E-5,
6.50030730567718));
#33194=CARTESIAN_POINT('Ctrl Pts',(-8.2139773816664,0.00271505638709518,
6.21868089666948));
#33195=CARTESIAN_POINT('Ctrl Pts',(-8.21366765236856,0.01653627011796,5.68352490005895));
#33196=CARTESIAN_POINT('Ctrl Pts',(-8.21103236130824,0.0566635365252091,
4.76263764161942));
#33197=CARTESIAN_POINT('Ctrl Pts',(-8.20152740606986,0.158430126564625,
3.0271363314686));
#33198=CARTESIAN_POINT('Ctrl Pts',(-8.20073061637961,0.149251458175202,
1.71872219634129));
#33199=CARTESIAN_POINT('Ctrl Pts',(-8.21717066237738,0.0181890322585064,
0.881529631657107));
#33200=CARTESIAN_POINT('Ctrl Pts',(-8.2193040340341,0.00329453289535601,
0.794356070514653));
#33201=CARTESIAN_POINT('Ctrl Pts',(-8.22416980127459,-0.033563900965499,
0.607050496827644));
#33202=CARTESIAN_POINT('Ctrl Pts',(-8.23413279979194,-0.112592668023086,
0.269906771666699));
#33203=CARTESIAN_POINT('Ctrl Pts',(-8.25161317521362,-0.267541466617309,
-0.25065980001266));
#33204=CARTESIAN_POINT('Ctrl Pts',(-8.2760674551824,-0.509570377892601,
-0.926107372523026));
#33205=CARTESIAN_POINT('Ctrl Pts',(-8.31129710119725,-0.885116143113864,
-1.89016358670453));
#33206=CARTESIAN_POINT('Ctrl Pts',(-8.35820655882308,-1.40718620794638,
-3.20511805596597));
#33207=CARTESIAN_POINT('Ctrl Pts',(-8.39167103174164,-1.75864819329131,
-4.39735605748105));
#33208=CARTESIAN_POINT('Ctrl Pts',(-8.4057490725845,-1.90357909164309,-5.19797714431349));
#33209=CARTESIAN_POINT('Ctrl Pts',(-8.41018696867969,-1.95004819727558,
-5.47978199297613));
#33210=CARTESIAN_POINT('Ctrl Pts',(-8.41764518232782,-2.0293328309496,-6.05846771470832));
#33211=CARTESIAN_POINT('Ctrl Pts',(-8.42608946693865,-2.12510790014958,
-7.04372337069025));
#33212=CARTESIAN_POINT('Ctrl Pts',(-8.42835688611333,-2.17335745278486,
-8.4058069611693));
#33213=CARTESIAN_POINT('Ctrl Pts',(-8.42483355820332,-2.16838683398674,
-9.69002623777674));
#33214=CARTESIAN_POINT('Ctrl Pts',(-8.4228693653896,-2.16758867316197,-10.549647857504));
#33215=CARTESIAN_POINT('Ctrl Pts',(-8.42227667941022,-2.1714754449322,-11.0287258129748));
#33216=CARTESIAN_POINT('Ctrl Pts',(-8.4222265668368,-2.17548571011368,-11.2641593891017));
#33217=CARTESIAN_POINT('Ctrl Pts',(-8.4223066588321,-2.17949860847749,-11.4403532700108));
#33218=CARTESIAN_POINT('Ctrl Pts',(-8.42237861265133,-2.18234534725527,
-11.5735122851675));
#33219=CARTESIAN_POINT('Ctrl Pts',(-8.42241335915678,-2.18714051116029,
-11.8308485666504));
#33220=CARTESIAN_POINT('Ctrl Pts',(-8.42226798867896,-2.19385085028673,
-12.2837525929814));
#33221=CARTESIAN_POINT('Ctrl Pts',(-8.42090827535907,-2.20284084437885,
-13.4368375872061));
#33222=CARTESIAN_POINT('Ctrl Pts',(-8.41742083334402,-2.19452611715802,
-14.699424889331));
#33223=CARTESIAN_POINT('Ctrl Pts',(-8.41459096562853,-2.18466983175675,
-15.9491420610126));
#33224=CARTESIAN_POINT('Ctrl Pts',(-8.41351488671319,-2.18063370066728,
-16.5720520403308));
#33225=CARTESIAN_POINT('Ctrl Pts',(-8.41300046580358,-2.17877051369586,
-17.0694513279955));
#33226=CARTESIAN_POINT('Ctrl Pts',(-8.41287266139027,-2.17841281520911,
-17.3179509620184));
#33227=CARTESIAN_POINT('Ctrl Pts',(-8.41283514635732,-2.17841198490692,
-17.5035714183381));
#33228=CARTESIAN_POINT('Ctrl Pts',(-8.4128192890245,-2.17840958154783,-17.6287745384218));
#33229=CARTESIAN_POINT('Ctrl Pts',(-8.41282274470808,-2.1783995227068,-17.8778185403976));
#33230=CARTESIAN_POINT('Ctrl Pts',(-8.41287433890386,-2.17837876830243,
-18.1275208893485));
#33231=CARTESIAN_POINT('Ctrl Pts',(-8.41297294837519,-2.17835392065712,
-18.3770615934934));
#33232=CARTESIAN_POINT('Ctrl Pts',(-8.41305237217696,-2.17833577105845,
-18.5331408135074));
#33233=CARTESIAN_POINT('Ctrl Pts',(-8.4131264249278,-2.17832044242199,-18.6580119473273));
#33234=CARTESIAN_POINT('Ctrl Pts',(-8.41320707340361,-2.17830426803329,
-18.7829114742903));
#33235=CARTESIAN_POINT('Ctrl Pts',(-8.41345624825908,-2.17825882731944,
-19.1264686399524));
#33236=CARTESIAN_POINT('Ctrl Pts',(-8.41400000345279,-2.17817104749403,
-19.6891521495847));
#33237=CARTESIAN_POINT('Ctrl Pts',(-8.41528017288101,-2.17804976165826,
-20.6909497614675));
#33238=CARTESIAN_POINT('Ctrl Pts',(-8.41726103341462,-2.1779744183845,-21.9461768404187));
#33239=CARTESIAN_POINT('Ctrl Pts',(-8.41893477480712,-2.17823712701764,
-22.953825983149));
#33240=CARTESIAN_POINT('Ctrl Pts',(-8.41986349686732,-2.17850502468349,
-23.5830767841885));
#33241=CARTESIAN_POINT('Ctrl Pts',(-8.42024378452539,-2.17862331222871,
-23.8321153579562));
#33242=CARTESIAN_POINT('Ctrl Pts',(-8.42106293419616,-2.17892596672298,
-24.3310626190291));
#33243=CARTESIAN_POINT('Ctrl Pts',(-8.42261468751758,-2.17958483043597,
-25.2061040655729));
#33244=CARTESIAN_POINT('Ctrl Pts',(-8.42511899294663,-2.18087935081873,
-26.4606390371043));
#33245=CARTESIAN_POINT('Ctrl Pts',(-8.42808089250611,-2.1824101925373,-27.9687820656938));
#33246=CARTESIAN_POINT('Ctrl Pts',(-8.42988072285208,-2.1833225916283,-28.9744904395833));
#33247=CARTESIAN_POINT('Ctrl Pts',(-8.43072515641183,-2.18365366003855,
-29.5378159164111));
#33248=CARTESIAN_POINT('Ctrl Pts',(-8.43096689351811,-2.18428588440253,
-29.6460087767788));
#33249=CARTESIAN_POINT('Ctrl Pts',(-8.43167406029457,-2.1876698352998,-29.8750129034852));
#33250=CARTESIAN_POINT('Ctrl Pts',(-8.43346090281294,-2.19874066252348,
-30.2778441726034));
#33251=CARTESIAN_POINT('Ctrl Pts',(-8.43877583514437,-2.2373949958194,-31.1153501423125));
#33252=CARTESIAN_POINT('Ctrl Pts',(-8.44693993544396,-2.30051991094785,
-32.1332707729797));
#33253=CARTESIAN_POINT('Ctrl Pts',(-8.45187694204408,-2.334473844321,-33.2140524330932));
#33254=CARTESIAN_POINT('Ctrl Pts',(-8.4522445888991,-2.33066489370667,-34.0552226771806));
#33255=CARTESIAN_POINT('Ctrl Pts',(-8.44752749223351,-2.28222892522994,
-34.9271681885516));
#33256=CARTESIAN_POINT('Ctrl Pts',(-8.43973025078375,-2.20888269376983,
-35.5269140529488));
#33257=CARTESIAN_POINT('Ctrl Pts',(-8.43168921619344,-2.133704304946,-35.984639162063));
#33258=CARTESIAN_POINT('Ctrl Pts',(-8.42470428825363,-2.06936251403802,
-36.3161971208814));
#33259=CARTESIAN_POINT('Ctrl Pts',(-8.40841115558265,-1.91462768039653,
-36.9382373792022));
#33260=CARTESIAN_POINT('Ctrl Pts',(-8.37476858189967,-1.58581660983551,
-37.9769230783518));
#33261=CARTESIAN_POINT('Ctrl Pts',(-8.30240748369846,-0.811573802930985,
-39.8436351201298));
#33262=CARTESIAN_POINT('Ctrl Pts',(-8.24766419492162,-0.281754963899915,
-41.1725199402397));
#33263=CARTESIAN_POINT('Ctrl Pts',(-8.22703915820806,-0.138584152464493,
-41.9674971713857));
#33264=CARTESIAN_POINT('Ctrl Pts',(-8.22279741361054,-0.106018153825827,
-42.1695350413675));
#33265=CARTESIAN_POINT('Ctrl Pts',(-8.21760452678912,-0.0696723394394581,
-42.4698336926041));
#33266=CARTESIAN_POINT('Ctrl Pts',(-8.21345399549118,-0.0419794705770708,
-42.783383071773));
#33267=CARTESIAN_POINT('Ctrl Pts',(-8.20920443802888,-0.0168922801706015,
-43.2117380270997));
#33268=CARTESIAN_POINT('Ctrl Pts',(-8.2060056324919,-0.00434463815486024,
-43.7719541949028));
#33269=CARTESIAN_POINT('Ctrl Pts',(-8.20454082076387,-0.0104625108048303,
-44.4815998892878));
#33270=CARTESIAN_POINT('Ctrl Pts',(-8.20440922525151,-0.0236201178969525,
-45.1041772238153));
#33271=CARTESIAN_POINT('Ctrl Pts',(-8.20441862179947,-0.0321411125244865,
-45.6207303121886));
#33272=CARTESIAN_POINT('Ctrl Pts',(-8.20434989009874,-0.0356782660657121,
-46.0172516471628));
#33273=CARTESIAN_POINT('Ctrl Pts',(-8.20406992251926,-0.0343648106023225,
-46.4229125033992));
#33274=CARTESIAN_POINT('Ctrl Pts',(-8.20323902185318,-0.0232669902564738,
-46.9758006019662));
#33275=CARTESIAN_POINT('Ctrl Pts',(-8.20188731183341,-0.00111372268798417,
-47.4040701896738));
#33276=CARTESIAN_POINT('Ctrl Pts',(-8.19979619418406,0.0351710604500778,
-47.8406800108478));
#33277=CARTESIAN_POINT('Ctrl Pts',(-8.19836170883178,0.0553133867555958,
-48.0821468140958));
#33278=CARTESIAN_POINT('Ctrl Pts',(-8.19535407046343,0.099077802122036,
-48.596971610594));
#33279=CARTESIAN_POINT('Ctrl Pts',(-8.18979813141032,0.178617138424551,
-49.4900316660884));
#33280=CARTESIAN_POINT('Ctrl Pts',(-8.18131347626536,0.313332652944236,
-50.7942648710663));
#33281=CARTESIAN_POINT('Ctrl Pts',(-8.17141615936791,0.535289599500542,
-52.3844504500429));
#33282=CARTESIAN_POINT('Ctrl Pts',(-8.16568083729471,0.743640919654865,
-53.4639249249685));
#33283=CARTESIAN_POINT('Ctrl Pts',(-8.16260421353783,0.899310397360863,
-54.1442403972218));
#33284=CARTESIAN_POINT('Ctrl Pts',(-8.16135401544335,0.962665926680855,
-54.41276557711));
#33285=CARTESIAN_POINT('Ctrl Pts',(-8.15887544372053,1.09733691858376,-54.9520352187707));
#33286=CARTESIAN_POINT('Ctrl Pts',(-8.15459691068634,1.3507946586784,-55.8907769762969));
#33287=CARTESIAN_POINT('Ctrl Pts',(-8.14657838814605,1.9255036615678,-57.7554882022754));
#33288=CARTESIAN_POINT('Ctrl Pts',(-8.14149181504208,2.51535089116785,-59.3213134096067));
#33289=CARTESIAN_POINT('Ctrl Pts',(-8.13972928395813,2.96457286522012,-60.4132064701784));
#33290=CARTESIAN_POINT('Ctrl Pts',(-8.13955344139843,3.02301727273934,-60.5535137041616));
#33291=CARTESIAN_POINT('Ctrl Pts',(-8.13926470646828,3.14029361968222,-60.8283650932639));
#33292=CARTESIAN_POINT('Ctrl Pts',(-8.13894720952011,3.35193263257086,-61.3083107938966));
#33293=CARTESIAN_POINT('Ctrl Pts',(-8.13894762339317,3.79342717132554,-62.2533982752636));
#33294=CARTESIAN_POINT('Ctrl Pts',(-8.1400365552858,4.32849389946224,-63.3055109143046));
#33295=CARTESIAN_POINT('Ctrl Pts',(-8.14146711027879,4.86804693212373,-64.3270786203418));
#33296=CARTESIAN_POINT('Ctrl Pts',(-8.14226817508642,5.16871692523809,-64.889895156736));
#33297=CARTESIAN_POINT('Ctrl Pts',(-8.14274451908316,5.36601178377058,-65.2597759526672));
#33298=CARTESIAN_POINT('Ctrl Pts',(-8.14304244247713,5.49657582154972,-65.5049110580499));
#33299=CARTESIAN_POINT('Ctrl Pts',(-8.14330765702863,5.62551558736444,-65.7478677462274));
#33300=CARTESIAN_POINT('Ctrl Pts',(-8.14349861608814,5.73655761778692,-65.9584086817351));
#33301=CARTESIAN_POINT('Ctrl Pts',(-8.14359486596038,5.79945465324739,-66.0781220853356));
#33302=CARTESIAN_POINT('Ctrl Pts',(-8.14372550172375,5.89322767828473,-66.2571021403003));
#33303=CARTESIAN_POINT('Ctrl Pts',(-8.1438054888816,5.97010448362115,-66.4049637463919));
#33304=CARTESIAN_POINT('Ctrl Pts',(-8.14388912480341,6.09562186726871,-66.6483134049626));
#33305=CARTESIAN_POINT('Ctrl Pts',(-8.14396545620633,6.2331613153188,-66.9139921069247));
#33306=CARTESIAN_POINT('Ctrl Pts',(-8.14408091872707,6.50319897559478,-67.4320256493946));
#33307=CARTESIAN_POINT('Ctrl Pts',(-8.14420049505799,6.97661293040496,-68.3319171006395));
#33308=CARTESIAN_POINT('Ctrl Pts',(-8.14417979226255,7.9158419811929,-70.0915028523489));
#33309=CARTESIAN_POINT('Ctrl Pts',(-8.14399378791187,8.71296190818585,-71.5675323137367));
#33310=CARTESIAN_POINT('Ctrl Pts',(-8.14401129173376,9.30773813911128,-72.6861798589276));
#33311=CARTESIAN_POINT('Ctrl Pts',(-8.14401378822158,9.44155634426351,-72.9378587433967));
#33312=CARTESIAN_POINT('Ctrl Pts',(-8.14401781863899,9.70835096815867,-73.4396327793342));
#33313=CARTESIAN_POINT('Ctrl Pts',(-8.14402139260452,10.0419982314087,-74.0671403835795));
#33314=CARTESIAN_POINT('Ctrl Pts',(-8.14402217907996,10.441980091082,-74.8193995595811));
#33315=CARTESIAN_POINT('Ctrl Pts',(-8.14401992121061,11.2417489323043,-76.3235460780868));
#33316=CARTESIAN_POINT('Ctrl Pts',(-8.14401659738412,11.9079355425531,-77.5764690921898));
#33317=CARTESIAN_POINT('Ctrl Pts',(-8.1440188815399,12.877844418806,-79.4006130100031));
#33318=CARTESIAN_POINT('Ctrl Pts',(-8.14402005669186,13.3144091843969,-80.2216773875901));
#33319=CARTESIAN_POINT('Ctrl Pts',(-8.14402005669182,13.7509307717864,-81.0426550896885));
#33320=CARTESIAN_POINT('Ctrl Pts',(-5.63798874401576,-0.000197003472309253,
24.8306349854119));
#33321=CARTESIAN_POINT('Ctrl Pts',(-5.63800558191124,-0.000197010017902819,
24.7817556802439));
#33322=CARTESIAN_POINT('Ctrl Pts',(-5.63802322829952,-0.000196997600998546,
24.732877683161));
#33323=CARTESIAN_POINT('Ctrl Pts',(-5.6382321992011,-0.000197727157601966,
24.1822611386521));
#33324=CARTESIAN_POINT('Ctrl Pts',(-5.63839540854526,-0.000203328251643161,
23.1780545711597));
#33325=CARTESIAN_POINT('Ctrl Pts',(-5.63876707035559,-0.000204428222765414,
21.1694483770277));
#33326=CARTESIAN_POINT('Ctrl Pts',(-5.64016391586993,-0.000218427565831332,
19.6651182773234));
#33327=CARTESIAN_POINT('Ctrl Pts',(-5.64311246961886,-0.000224802933236796,
18.4139922902723));
#33328=CARTESIAN_POINT('Ctrl Pts',(-5.64452522473937,-0.000225999139705922,
17.9111644969149));
#33329=CARTESIAN_POINT('Ctrl Pts',(-5.64807365157005,-0.000230617251699585,
16.9071248156262));
#33330=CARTESIAN_POINT('Ctrl Pts',(-5.6556821342335,-0.000236390082593806,
15.1532608344032));
#33331=CARTESIAN_POINT('Ctrl Pts',(-5.66292925317201,-0.000267962939935839,
13.6511084868801));
#33332=CARTESIAN_POINT('Ctrl Pts',(-5.66747180552725,-0.000282218227139333,
12.3964390741229));
#33333=CARTESIAN_POINT('Ctrl Pts',(-5.66932651967778,-0.000283883146473219,
11.895428735672));
#33334=CARTESIAN_POINT('Ctrl Pts',(-5.67311242407095,-0.000293045511818167,
10.8935268493743));
#33335=CARTESIAN_POINT('Ctrl Pts',(-5.67966191248225,-0.000299082491310505,
9.13954002036197));
#33336=CARTESIAN_POINT('Ctrl Pts',(-5.68431080553268,-0.000384941206993508,
7.63411967127975));
#33337=CARTESIAN_POINT('Ctrl Pts',(-5.686372275596,-0.000411482825566298,
6.50039814288972));
#33338=CARTESIAN_POINT('Ctrl Pts',(-5.68684776179194,0.00229630643279153,
6.21845427742025));
#33339=CARTESIAN_POINT('Ctrl Pts',(-5.68786142444616,0.0162632612901432,
5.68295491308527));
#33340=CARTESIAN_POINT('Ctrl Pts',(-5.68971236172501,0.0567615293401514,
4.76167563319915));
#33341=CARTESIAN_POINT('Ctrl Pts',(-5.69297084014264,0.159517117332154,
3.02639313928253));
#33342=CARTESIAN_POINT('Ctrl Pts',(-5.69264654080951,0.149618749208594,
1.72037399230591));
#33343=CARTESIAN_POINT('Ctrl Pts',(-5.68856841900556,0.0173647191069126,
0.885235947772052));
#33344=CARTESIAN_POINT('Ctrl Pts',(-5.68803099617261,0.00238318925849841,
0.798409810767109));
#33345=CARTESIAN_POINT('Ctrl Pts',(-5.68680608971042,-0.0347544439548622,
0.61164864292997));
#33346=CARTESIAN_POINT('Ctrl Pts',(-5.68428941420376,-0.114424015372209,
0.275299005848681));
#33347=CARTESIAN_POINT('Ctrl Pts',(-5.67990871577964,-0.270957526740268,
-0.244611018683231));
#33348=CARTESIAN_POINT('Ctrl Pts',(-5.67369396529163,-0.515273456664773,
-0.919737137559079));
#33349=CARTESIAN_POINT('Ctrl Pts',(-5.6646921537697,-0.894616695793402,
-1.88381123416328));
#33350=CARTESIAN_POINT('Ctrl Pts',(-5.65218739183062,-1.42140596824095,
-3.19924008823192));
#33351=CARTESIAN_POINT('Ctrl Pts',(-5.64245712789792,-1.77696374815495,
-4.3925641794195));
#33352=CARTESIAN_POINT('Ctrl Pts',(-5.63796441630677,-1.92370576951919,
-5.1946090699866));
#33353=CARTESIAN_POINT('Ctrl Pts',(-5.63650687495268,-1.9706510187358,-5.47668455904916));
#33354=CARTESIAN_POINT('Ctrl Pts',(-5.63387712655626,-2.05079010518533,
-6.0560630588307));
#33355=CARTESIAN_POINT('Ctrl Pts',(-5.63037973233777,-2.14756911677532,
-7.04237048376366));
#33356=CARTESIAN_POINT('Ctrl Pts',(-5.62771024023403,-2.19629179135161,
-8.40560259571312));
#33357=CARTESIAN_POINT('Ctrl Pts',(-5.62646453378276,-2.19120634551966,
-9.69018239553766));
#33358=CARTESIAN_POINT('Ctrl Pts',(-5.62553693460616,-2.19025626927096,
-10.5496403261192));
#33359=CARTESIAN_POINT('Ctrl Pts',(-5.62492773711517,-2.19409035070739,
-11.028506356485));
#33360=CARTESIAN_POINT('Ctrl Pts',(-5.62458342773447,-2.19809200746593,
-11.2637947462558));
#33361=CARTESIAN_POINT('Ctrl Pts',(-5.6243036959921,-2.20210252034327,-11.4398681067028));
#33362=CARTESIAN_POINT('Ctrl Pts',(-5.62410483522145,-2.20495370924458,
-11.5730994778588));
#33363=CARTESIAN_POINT('Ctrl Pts',(-5.62372750411003,-2.20974250570501,
-11.8304896121988));
#33364=CARTESIAN_POINT('Ctrl Pts',(-5.62310049238311,-2.21643113870861,
-12.283523795246));
#33365=CARTESIAN_POINT('Ctrl Pts',(-5.62168000244819,-2.22531034670341,
-13.4368678683667));
#33366=CARTESIAN_POINT('Ctrl Pts',(-5.62061026542929,-2.21676141606032,
-14.699629050403));
#33367=CARTESIAN_POINT('Ctrl Pts',(-5.61992998041975,-2.20662324725371,
-15.9492985747393));
#33368=CARTESIAN_POINT('Ctrl Pts',(-5.61970956077904,-2.20251357405667,
-16.5721572080187));
#33369=CARTESIAN_POINT('Ctrl Pts',(-5.61958734393837,-2.20060253110823,
-17.0694810153417));
#33370=CARTESIAN_POINT('Ctrl Pts',(-5.61954956517472,-2.2002384474806,-17.3179365617655));
#33371=CARTESIAN_POINT('Ctrl Pts',(-5.61952801743157,-2.20023584646593,
-17.5035209125398));
#33372=CARTESIAN_POINT('Ctrl Pts',(-5.61952113110232,-2.20023320019289,
-17.6287345805335));
#33373=CARTESIAN_POINT('Ctrl Pts',(-5.61953393535414,-2.20022439388902,
-17.8777776408766));
#33374=CARTESIAN_POINT('Ctrl Pts',(-5.61958764142248,-2.20021267485849,
-18.1274866656909));
#33375=CARTESIAN_POINT('Ctrl Pts',(-5.61967219934989,-2.20019766750374,
-18.377026362966));
#33376=CARTESIAN_POINT('Ctrl Pts',(-5.61973830896478,-2.20018791517279,
-18.5331054168968));
#33377=CARTESIAN_POINT('Ctrl Pts',(-5.61979786202761,-2.20017981841732,
-18.6579753380496));
#33378=CARTESIAN_POINT('Ctrl Pts',(-5.61986172050493,-2.20017160267944,
-18.7828733819617));
#33379=CARTESIAN_POINT('Ctrl Pts',(-5.62005763737625,-2.20015075591428,
-19.1264263327723));
#33380=CARTESIAN_POINT('Ctrl Pts',(-5.62046272300978,-2.2001199750147,-19.6890959425505));
#33381=CARTESIAN_POINT('Ctrl Pts',(-5.62134039297357,-2.20012734742513,
-20.690855324408));
#33382=CARTESIAN_POINT('Ctrl Pts',(-5.62247078887583,-2.20028948776679,
-21.9459931764134));
#33383=CARTESIAN_POINT('Ctrl Pts',(-5.62304153313537,-2.20076782870844,
-22.9535436359179));
#33384=CARTESIAN_POINT('Ctrl Pts',(-5.62311736659782,-2.20119855016699,
-23.5827128224497));
#33385=CARTESIAN_POINT('Ctrl Pts',(-5.62312505609341,-2.20138895511271,
-23.8316904452359));
#33386=CARTESIAN_POINT('Ctrl Pts',(-5.62307863861334,-2.20184988096975,
-24.3305490629185));
#33387=CARTESIAN_POINT('Ctrl Pts',(-5.62284832796686,-2.20283552305635,
-25.2054616107245));
#33388=CARTESIAN_POINT('Ctrl Pts',(-5.6222622772683,-2.20461588646114,-26.4599423345342));
#33389=CARTESIAN_POINT('Ctrl Pts',(-5.62144992063832,-2.20679856145,-27.9681630936482));
#33390=CARTESIAN_POINT('Ctrl Pts',(-5.6211590510458,-2.20797434227957,-28.9740718190661));
#33391=CARTESIAN_POINT('Ctrl Pts',(-5.62111618801636,-2.20844966017214,
-29.5375147504093));
#33392=CARTESIAN_POINT('Ctrl Pts',(-5.62109422172764,-2.20911507239076,
-29.6455549435117));
#33393=CARTESIAN_POINT('Ctrl Pts',(-5.62100876715226,-2.21258346457478,
-29.8743811766298));
#33394=CARTESIAN_POINT('Ctrl Pts',(-5.62075401832145,-2.22382403270066,
-30.2769177522939));
#33395=CARTESIAN_POINT('Ctrl Pts',(-5.61990887107815,-2.26295805170465,
-31.1141259057382));
#33396=CARTESIAN_POINT('Ctrl Pts',(-5.61848957316824,-2.32674809384181,
-32.1322815139189));
#33397=CARTESIAN_POINT('Ctrl Pts',(-5.61781000352031,-2.36116406208853,
-33.2138797468871));
#33398=CARTESIAN_POINT('Ctrl Pts',(-5.61809400321541,-2.35739190047119,
-34.0559545601601));
#33399=CARTESIAN_POINT('Ctrl Pts',(-5.61961452951742,-2.30835269989843,
-34.9291041558053));
#33400=CARTESIAN_POINT('Ctrl Pts',(-5.62177024593562,-2.23404940008006,
-35.529744944464));
#33401=CARTESIAN_POINT('Ctrl Pts',(-5.62393780073057,-2.15796077965923,
-35.9881178443849));
#33402=CARTESIAN_POINT('Ctrl Pts',(-5.62584009583325,-2.09278630793423,
-36.3202547621105));
#33403=CARTESIAN_POINT('Ctrl Pts',(-5.63013513192705,-1.9363345551221,-36.9430040876631));
#33404=CARTESIAN_POINT('Ctrl Pts',(-5.63860506790231,-1.60404305886794,
-37.9824489926659));
#33405=CARTESIAN_POINT('Ctrl Pts',(-5.65541457729167,-0.823249020271413,
-39.8498632334892));
#33406=CARTESIAN_POINT('Ctrl Pts',(-5.66661670520381,-0.28703789039762,
-41.1786802522904));
#33407=CARTESIAN_POINT('Ctrl Pts',(-5.67105654561514,-0.14240251435379,
-41.9710438412748));
#33408=CARTESIAN_POINT('Ctrl Pts',(-5.67202248528354,-0.109518971665621,
-42.1728083600125));
#33409=CARTESIAN_POINT('Ctrl Pts',(-5.67323543706194,-0.0727704952235973,
-42.4725554520429));
#33410=CARTESIAN_POINT('Ctrl Pts',(-5.67424842816243,-0.0447278973882266,
-42.7856337375846));
#33411=CARTESIAN_POINT('Ctrl Pts',(-5.67532096648076,-0.0192377484700357,
-43.2133842460989));
#33412=CARTESIAN_POINT('Ctrl Pts',(-5.67619447869966,-0.0063079848737366,
-43.7729890033109));
#33413=CARTESIAN_POINT('Ctrl Pts',(-5.67662753088596,-0.0121264093254704,
-44.482140388523));
#33414=CARTESIAN_POINT('Ctrl Pts',(-5.67660346780222,-0.0251049264471304,
-45.1045178144991));
#33415=CARTESIAN_POINT('Ctrl Pts',(-5.6764927226138,-0.0335587492382865,
-45.6210550178592));
#33416=CARTESIAN_POINT('Ctrl Pts',(-5.67635643262694,-0.0370325137349412,
-46.0176274785659));
#33417=CARTESIAN_POINT('Ctrl Pts',(-5.67619165632205,-0.035633795839697,
-46.4234041201591));
#33418=CARTESIAN_POINT('Ctrl Pts',(-5.6759795941213,-0.0243845393331214,
-46.9765347575413));
#33419=CARTESIAN_POINT('Ctrl Pts',(-5.67580300544141,-0.00199946540293369,
-47.4050759510626));
#33420=CARTESIAN_POINT('Ctrl Pts',(-5.67571775267112,0.0345851513673987,
-47.8420157886383));
#33421=CARTESIAN_POINT('Ctrl Pts',(-5.67564273379123,0.0548808751941392,
-48.0835009105947));
#33422=CARTESIAN_POINT('Ctrl Pts',(-5.67542062178334,0.098999274407724,
-48.5984489114891));
#33423=CARTESIAN_POINT('Ctrl Pts',(-5.67483381441346,0.17919214459599,-49.4916003161553));
#33424=CARTESIAN_POINT('Ctrl Pts',(-5.67337007871572,0.314922909631311,
-50.7957980320261));
#33425=CARTESIAN_POINT('Ctrl Pts',(-5.67081714031925,0.537881024433923,
-52.3856243686801));
#33426=CARTESIAN_POINT('Ctrl Pts',(-5.66846450176822,0.746623460845851,
-53.4646648158997));
#33427=CARTESIAN_POINT('Ctrl Pts',(-5.66683996713186,0.902366786944092,
-54.1446607528198));
#33428=CARTESIAN_POINT('Ctrl Pts',(-5.66613818814274,0.965739288299476,
-54.4130801179455));
#33429=CARTESIAN_POINT('Ctrl Pts',(-5.66453501303538,1.10040030864196,-54.9521509243576));
#33430=CARTESIAN_POINT('Ctrl Pts',(-5.66128069329804,1.35374995466334,-55.8906029672423));
#33431=CARTESIAN_POINT('Ctrl Pts',(-5.6536193010957,1.92793543307145,-57.7549412003636));
#33432=CARTESIAN_POINT('Ctrl Pts',(-5.64716225372688,2.51720283228602,-59.3207769290211));
#33433=CARTESIAN_POINT('Ctrl Pts',(-5.64455789154054,2.96622528244185,-60.4128272194335));
#33434=CARTESIAN_POINT('Ctrl Pts',(-5.64424507271109,3.02462206702412,-60.553109707374));
#33435=CARTESIAN_POINT('Ctrl Pts',(-5.64365588485913,3.14181292272085,-60.827939914503));
#33436=CARTESIAN_POINT('Ctrl Pts',(-5.64271282607086,3.35329136898542,-61.3078432002741));
#33437=CARTESIAN_POINT('Ctrl Pts',(-5.64114683715443,3.79445349188391,-62.252883979634));
#33438=CARTESIAN_POINT('Ctrl Pts',(-5.63999702692252,4.32913575921044,-63.3049907496339));
#33439=CARTESIAN_POINT('Ctrl Pts',(-5.63920737724254,4.86835251310299,-64.3266002920913));
#33440=CARTESIAN_POINT('Ctrl Pts',(-5.63885055859379,5.16886014394431,-64.8894571013804));
#33441=CARTESIAN_POINT('Ctrl Pts',(-5.6386317481306,5.36606332219433,-65.2593722248099));
#33442=CARTESIAN_POINT('Ctrl Pts',(-5.63848800035496,5.49657044970995,-65.5045323669089));
#33443=CARTESIAN_POINT('Ctrl Pts',(-5.63835259198041,5.62546168731041,-65.7475169610679));
#33444=CARTESIAN_POINT('Ctrl Pts',(-5.63823133523655,5.73646786926492,-65.9580854636632));
#33445=CARTESIAN_POINT('Ctrl Pts',(-5.63816171768633,5.79934662156983,-66.077815500769));
#33446=CARTESIAN_POINT('Ctrl Pts',(-5.63805635071558,5.89309438747521,-66.2568214244471));
#33447=CARTESIAN_POINT('Ctrl Pts',(-5.63796940294333,5.96995542512624,-66.4047063907607));
#33448=CARTESIAN_POINT('Ctrl Pts',(-5.63781800927207,6.0954529938488,-66.6480975667157));
#33449=CARTESIAN_POINT('Ctrl Pts',(-5.63768231546802,6.23297121546627,-66.9138116410786));
#33450=CARTESIAN_POINT('Ctrl Pts',(-5.637479034481,6.50298560865622,-67.4319127266579));
#33451=CARTESIAN_POINT('Ctrl Pts',(-5.63729628543975,6.97639589758447,-68.3319023920043));
#33452=CARTESIAN_POINT('Ctrl Pts',(-5.63743078458553,7.91572142956478,-70.0916119116528));
#33453=CARTESIAN_POINT('Ctrl Pts',(-5.63791663981526,8.71295327982952,-71.5676112934143));
#33454=CARTESIAN_POINT('Ctrl Pts',(-5.63792242673017,9.30768338133656,-72.6861728890823));
#33455=CARTESIAN_POINT('Ctrl Pts',(-5.63792178222381,9.44150440140497,-72.9378580825763));
#33456=CARTESIAN_POINT('Ctrl Pts',(-5.63792140995083,9.70829729496219,-73.4396300814865));
#33457=CARTESIAN_POINT('Ctrl Pts',(-5.63792335705853,10.0419462746335,-74.0671406986579));
#33458=CARTESIAN_POINT('Ctrl Pts',(-5.63792450110527,10.4419285249544,-74.8194001489715));
#33459=CARTESIAN_POINT('Ctrl Pts',(-5.63792772394606,11.2416996338346,-76.3235485176472));
#33460=CARTESIAN_POINT('Ctrl Pts',(-5.63793906758245,11.9078896183025,-77.5764705531983));
#33461=CARTESIAN_POINT('Ctrl Pts',(-5.63794461293377,12.8777987902702,-79.4006124326407));
#33462=CARTESIAN_POINT('Ctrl Pts',(-5.63794746754098,13.3143645759993,-80.22167739341));
#33463=CARTESIAN_POINT('Ctrl Pts',(-5.63794746754101,13.7508861633887,-81.0426550955084));
#33464=CARTESIAN_POINT('Ctrl Pts',(-3.75853532388587,-7.82717008495635E-5,
24.8306348326723));
#33465=CARTESIAN_POINT('Ctrl Pts',(-3.75854654435664,-7.82749362348716E-5,
24.7817555228025));
#33466=CARTESIAN_POINT('Ctrl Pts',(-3.75855831587281,-7.82802977327427E-5,
24.7328775181985));
#33467=CARTESIAN_POINT('Ctrl Pts',(-3.75869715731044,-7.82539305063524E-5,
24.1822610105156));
#33468=CARTESIAN_POINT('Ctrl Pts',(-3.75880238754123,-7.77773261011803E-5,
23.1780551437883));
#33469=CARTESIAN_POINT('Ctrl Pts',(-3.75904944284305,-7.7931664848751E-5,
21.1694489328841));
#33470=CARTESIAN_POINT('Ctrl Pts',(-3.75997170226701,-7.68106373729368E-5,
19.6651207230274));
#33471=CARTESIAN_POINT('Ctrl Pts',(-3.76193324311245,-7.65296069702623E-5,
18.4139955646262));
#33472=CARTESIAN_POINT('Ctrl Pts',(-3.76287426611526,-7.66096606190882E-5,
17.911167619251));
#33473=CARTESIAN_POINT('Ctrl Pts',(-3.76523680827642,-7.66850715270179E-5,
16.9071282930257));
#33474=CARTESIAN_POINT('Ctrl Pts',(-3.77030515875508,-7.72512599819896E-5,
15.1532648847908));
#33475=CARTESIAN_POINT('Ctrl Pts',(-3.77511624071878,-7.47472292143438E-5,
13.6511179057538));
#33476=CARTESIAN_POINT('Ctrl Pts',(-3.77813547303937,-7.31175951349916E-5,
12.3964515094638));
#33477=CARTESIAN_POINT('Ctrl Pts',(-3.77937083065646,-7.27403671319445E-5,
11.8954431352254));
#33478=CARTESIAN_POINT('Ctrl Pts',(-3.78188901434931,-7.14581327677145E-5,
10.8935397134728));
#33479=CARTESIAN_POINT('Ctrl Pts',(-3.78625108065095,-6.87239696068783E-5,
9.13956927306207));
#33480=CARTESIAN_POINT('Ctrl Pts',(-3.78929711946154,-6.07535379212773E-5,
7.63411764796906));
#33481=CARTESIAN_POINT('Ctrl Pts',(-3.79065166883889,-5.22034577220886E-5,
6.50050775733845));
#33482=CARTESIAN_POINT('Ctrl Pts',(-3.79107986193104,0.00252228322518703,
6.22000470746017));
#33483=CARTESIAN_POINT('Ctrl Pts',(-3.79234380964367,0.0158113917461691,
5.68607024174225));
#33484=CARTESIAN_POINT('Ctrl Pts',(-3.79531837082677,0.0544174247292424,
4.76668616845752));
#33485=CARTESIAN_POINT('Ctrl Pts',(-3.80220285402255,0.152587810395906,
3.03036886221659));
#33486=CARTESIAN_POINT('Ctrl Pts',(-3.80176228630631,0.143826217072127,
1.71474782041542));
#33487=CARTESIAN_POINT('Ctrl Pts',(-3.79140440831168,0.016248157303979,
0.870099283591018));
#33488=CARTESIAN_POINT('Ctrl Pts',(-3.79006590320266,0.00167268401214881,
0.781636720070122));
#33489=CARTESIAN_POINT('Ctrl Pts',(-3.78699184695418,-0.0342756137737318,
0.592244840357804));
#33490=CARTESIAN_POINT('Ctrl Pts',(-3.78066302350217,-0.111211123419434,
0.251903829461684));
#33491=CARTESIAN_POINT('Ctrl Pts',(-3.76939533703961,-0.261513074861836,
-0.271663801877638));
#33492=CARTESIAN_POINT('Ctrl Pts',(-3.75359988220739,-0.495283056373455,
-0.94914295080062));
#33493=CARTESIAN_POINT('Ctrl Pts',(-3.73072616249344,-0.857108261975899,
-1.9143557657));
#33494=CARTESIAN_POINT('Ctrl Pts',(-3.70064315115094,-1.35835307823454,
-3.22863941593501));
#33495=CARTESIAN_POINT('Ctrl Pts',(-3.67973778488251,-1.69407181273673,
-4.4157111301945));
#33496=CARTESIAN_POINT('Ctrl Pts',(-3.67085928169629,-1.83212785104798,
-5.210308046637));
#33497=CARTESIAN_POINT('Ctrl Pts',(-3.66793764503103,-1.87653006151095,
-5.4910274303086));
#33498=CARTESIAN_POINT('Ctrl Pts',(-3.66288142323918,-1.95219900130291,
-6.06694545421104));
#33499=CARTESIAN_POINT('Ctrl Pts',(-3.65650523893321,-2.04365923799453,
-7.04821528392791));
#33500=CARTESIAN_POINT('Ctrl Pts',(-3.65264711546065,-2.08974502003478,
-8.4062262755857));
#33501=CARTESIAN_POINT('Ctrl Pts',(-3.65203203181246,-2.08491430156149,
-9.68931684248278));
#33502=CARTESIAN_POINT('Ctrl Pts',(-3.65150826790285,-2.08404876723427,
-10.5495669923731));
#33503=CARTESIAN_POINT('Ctrl Pts',(-3.65096858012834,-2.08772800945087,
-11.0294381603198));
#33504=CARTESIAN_POINT('Ctrl Pts',(-3.65058185043361,-2.09155483800607,
-11.2654142598092));
#33505=CARTESIAN_POINT('Ctrl Pts',(-3.65023458911074,-2.09539087307951,
-11.4420542665395));
#33506=CARTESIAN_POINT('Ctrl Pts',(-3.64999169712714,-2.09810145524411,
-11.5749357706628));
#33507=CARTESIAN_POINT('Ctrl Pts',(-3.64955858697807,-2.10266722483507,
-11.8320568591363));
#33508=CARTESIAN_POINT('Ctrl Pts',(-3.64889746597844,-2.10904587316385,
-12.2844589281418));
#33509=CARTESIAN_POINT('Ctrl Pts',(-3.64768290265879,-2.11754588473787,
-13.4365947109693));
#33510=CARTESIAN_POINT('Ctrl Pts',(-3.64746698996492,-2.10947815317904,
-14.6986500552709));
#33511=CARTESIAN_POINT('Ctrl Pts',(-3.64758001480721,-2.09992789176325,
-15.948456137313));
#33512=CARTESIAN_POINT('Ctrl Pts',(-3.64764941892127,-2.09603249999465,
-16.5715515889072));
#33513=CARTESIAN_POINT('Ctrl Pts',(-3.64767599399056,-2.09422846040575,
-17.0691867471765));
#33514=CARTESIAN_POINT('Ctrl Pts',(-3.64767278213141,-2.09388242091375,
-17.3178339137197));
#33515=CARTESIAN_POINT('Ctrl Pts',(-3.64766195162746,-2.09388021807885,
-17.5035718635503));
#33516=CARTESIAN_POINT('Ctrl Pts',(-3.64766037907709,-2.09387863576372,
-17.628736956136));
#33517=CARTESIAN_POINT('Ctrl Pts',(-3.64767791885066,-2.0938758458656,-17.8777754411049));
#33518=CARTESIAN_POINT('Ctrl Pts',(-3.64772457263836,-2.09387183205052,
-18.127451726039));
#33519=CARTESIAN_POINT('Ctrl Pts',(-3.64779507913674,-2.09386947214827,
-18.3769832632093));
#33520=CARTESIAN_POINT('Ctrl Pts',(-3.6478483308591,-2.09386808188328,-18.5330555957456));
#33521=CARTESIAN_POINT('Ctrl Pts',(-3.64789576041336,-2.09386734399663,
-18.6579232856571));
#33522=CARTESIAN_POINT('Ctrl Pts',(-3.64794615788519,-2.09386665377775,
-18.7828197024514));
#33523=CARTESIAN_POINT('Ctrl Pts',(-3.64809782566923,-2.0938664352779,-19.1263719755194));
#33524=CARTESIAN_POINT('Ctrl Pts',(-3.64840051409532,-2.09386850931672,
-19.6890626879726));
#33525=CARTESIAN_POINT('Ctrl Pts',(-3.64901106867713,-2.09390750623519,
-20.6909211725876));
#33526=CARTESIAN_POINT('Ctrl Pts',(-3.64969208152518,-2.09399894836801,
-21.9463041772876));
#33527=CARTESIAN_POINT('Ctrl Pts',(-3.64979639834935,-2.09420105310877,
-22.9541717024532));
#33528=CARTESIAN_POINT('Ctrl Pts',(-3.64957735467363,-2.09434939667683,
-23.5835820407631));
#33529=CARTESIAN_POINT('Ctrl Pts',(-3.64946154252902,-2.09441198780494,
-23.8327092564764));
#33530=CARTESIAN_POINT('Ctrl Pts',(-3.64913803877753,-2.09456451664979,
-24.3317957111891));
#33531=CARTESIAN_POINT('Ctrl Pts',(-3.648352819248,-2.09488096347744,-25.207038469841));
#33532=CARTESIAN_POINT('Ctrl Pts',(-3.64683626660838,-2.09548696314257,
-26.4617048010875));
#33533=CARTESIAN_POINT('Ctrl Pts',(-3.64488331224232,-2.0961837752456,-27.9697879027271));
#33534=CARTESIAN_POINT('Ctrl Pts',(-3.64395769228688,-2.09662244536148,
-28.9752722261224));
#33535=CARTESIAN_POINT('Ctrl Pts',(-3.6436205019928,-2.09678630431028,-29.5384886302537));
#33536=CARTESIAN_POINT('Ctrl Pts',(-3.64351153512049,-2.0973662734663,-29.6473611136137));
#33537=CARTESIAN_POINT('Ctrl Pts',(-3.64317624760616,-2.10056409426989,
-29.8772090485191));
#33538=CARTESIAN_POINT('Ctrl Pts',(-3.64230927835962,-2.1111057457118,-30.2814499916388));
#33539=CARTESIAN_POINT('Ctrl Pts',(-3.63967466585405,-2.14803998985422,
-31.1205252839991));
#33540=CARTESIAN_POINT('Ctrl Pts',(-3.63572140605777,-2.20828479577518,
-32.1378836654998));
#33541=CARTESIAN_POINT('Ctrl Pts',(-3.63358924140075,-2.2405761068103,-33.2155342515335));
#33542=CARTESIAN_POINT('Ctrl Pts',(-3.63378778424351,-2.23686004340906,
-34.0530834789304));
#33543=CARTESIAN_POINT('Ctrl Pts',(-3.63675381955408,-2.190599093022,-34.9201817981066));
#33544=CARTESIAN_POINT('Ctrl Pts',(-3.64123191036651,-2.12068100214489,
-35.5160745326321));
#33545=CARTESIAN_POINT('Ctrl Pts',(-3.64576438011192,-2.04906134821434,
-35.9707720742832));
#33546=CARTESIAN_POINT('Ctrl Pts',(-3.64965298273566,-1.98788192349195,
-36.2994619330854));
#33547=CARTESIAN_POINT('Ctrl Pts',(-3.65880246984932,-1.84047979358516,
-36.9176012241994));
#33548=CARTESIAN_POINT('Ctrl Pts',(-3.67806204837734,-1.52651468642503,
-37.9518433469515));
#33549=CARTESIAN_POINT('Ctrl Pts',(-3.72086560389792,-0.784570381697561,
-39.8175211185846));
#33550=CARTESIAN_POINT('Ctrl Pts',(-3.75502335684506,-0.272190657553224,
-41.1494732605515));
#33551=CARTESIAN_POINT('Ctrl Pts',(-3.76762193450478,-0.13228232701847,
-41.9554888717754));
#33552=CARTESIAN_POINT('Ctrl Pts',(-3.77018890614804,-0.100794906990536,
-42.1587122714258));
#33553=CARTESIAN_POINT('Ctrl Pts',(-3.77337862406258,-0.0656523899136256,
-42.4612575185149));
#33554=CARTESIAN_POINT('Ctrl Pts',(-3.77595475717398,-0.0390350463462554,
-42.776673888403));
#33555=CARTESIAN_POINT('Ctrl Pts',(-3.7786365989841,-0.0150756310605251,
-43.2073666789962));
#33556=CARTESIAN_POINT('Ctrl Pts',(-3.78072522701561,-0.00346913651286049,
-43.7699070202859));
#33557=CARTESIAN_POINT('Ctrl Pts',(-3.78173732898778,-0.0100179160988367,
-44.4814310562548));
#33558=CARTESIAN_POINT('Ctrl Pts',(-3.78180044511189,-0.0231100159289182,
-45.1047807273984));
#33559=CARTESIAN_POINT('Ctrl Pts',(-3.78166099965021,-0.0314898532548608,
-45.6215024351169));
#33560=CARTESIAN_POINT('Ctrl Pts',(-3.78153156649938,-0.0349108490470552,
-46.0179165001026));
#33561=CARTESIAN_POINT('Ctrl Pts',(-3.78144717600605,-0.0335232889237656,
-46.4232364281124));
#33562=CARTESIAN_POINT('Ctrl Pts',(-3.78149126288203,-0.022464138604499,
-46.975363526501));
#33563=CARTESIAN_POINT('Ctrl Pts',(-3.78179709799868,-0.000576863581530635,
-47.4027053717721));
#33564=CARTESIAN_POINT('Ctrl Pts',(-3.78243277047768,0.0351297799016445,
-47.8382051253742));
#33565=CARTESIAN_POINT('Ctrl Pts',(-3.7828521655432,0.0550254679880845,
-48.0799370747199));
#33566=CARTESIAN_POINT('Ctrl Pts',(-3.78366605684173,0.0982302401516215,
-48.5947359044865));
#33567=CARTESIAN_POINT('Ctrl Pts',(-3.78499798423273,0.176872274547839,
-49.4880650124114));
#33568=CARTESIAN_POINT('Ctrl Pts',(-3.78647580599884,0.310424786308024,
-50.7925895120424));
#33569=CARTESIAN_POINT('Ctrl Pts',(-3.78717568337191,0.531337373178592,
-52.3833317731187));
#33570=CARTESIAN_POINT('Ctrl Pts',(-3.7865819860366,0.739296298888895,-53.4632179152833));
#33571=CARTESIAN_POINT('Ctrl Pts',(-3.78580490188227,0.894839020014008,
-54.1438065235354));
#33572=CARTESIAN_POINT('Ctrl Pts',(-3.78543262539753,0.958171122282076,
-54.4124863225216));
#33573=CARTESIAN_POINT('Ctrl Pts',(-3.78444370602454,1.09283917001359,-54.9520049683496));
#33574=CARTESIAN_POINT('Ctrl Pts',(-3.78216157813114,1.34642076525217,-55.8911232547336));
#33575=CARTESIAN_POINT('Ctrl Pts',(-3.77602584954904,1.92172700273483,-57.7562776592878));
#33576=CARTESIAN_POINT('Ctrl Pts',(-3.77022072522239,2.51236442779873,-59.3220758584305));
#33577=CARTESIAN_POINT('Ctrl Pts',(-3.76779455586239,2.96190521138445,-60.4137989092541));
#33578=CARTESIAN_POINT('Ctrl Pts',(-3.76749222284573,3.02041536309737,-60.5541442225808));
#33579=CARTESIAN_POINT('Ctrl Pts',(-3.76690761672463,3.13781401399604,-60.8290330399708));
#33580=CARTESIAN_POINT('Ctrl Pts',(-3.76591968324598,3.3496899726605,-61.309049494963));
#33581=CARTESIAN_POINT('Ctrl Pts',(-3.76409555893897,3.79169292000971,-62.2542211745589));
#33582=CARTESIAN_POINT('Ctrl Pts',(-3.76236115234085,4.32739169568999,-63.3063512843697));
#33583=CARTESIAN_POINT('Ctrl Pts',(-3.76093648081012,4.86749660007094,-64.3278585369242));
#33584=CARTESIAN_POINT('Ctrl Pts',(-3.76024239649334,5.1684273086147,-64.8906121976067));
#33585=CARTESIAN_POINT('Ctrl Pts',(-3.75982229879937,5.36586845324159,-65.2604378773822));
#33586=CARTESIAN_POINT('Ctrl Pts',(-3.75955278590453,5.49652119911916,-65.505532600228));
#33587=CARTESIAN_POINT('Ctrl Pts',(-3.75930152180481,5.62553933749147,-65.7484431426067));
#33588=CARTESIAN_POINT('Ctrl Pts',(-3.7590947164072,5.73663607593057,-65.9589384493982));
#33589=CARTESIAN_POINT('Ctrl Pts',(-3.75898058555973,5.79956068820915,-66.0786241831879));
#33590=CARTESIAN_POINT('Ctrl Pts',(-3.75881327243508,5.89337112016886,-66.2575611354474));
#33591=CARTESIAN_POINT('Ctrl Pts',(-3.75868316571257,5.97027208588428,-66.405383063182));
#33592=CARTESIAN_POINT('Ctrl Pts',(-3.758477673407,6.09581674659771,-66.648662549422));
#33593=CARTESIAN_POINT('Ctrl Pts',(-3.75829211778717,6.23339093492571,-66.9142887943685));
#33594=CARTESIAN_POINT('Ctrl Pts',(-3.75801448399417,6.50346468227751,-67.4322179601308));
#33595=CARTESIAN_POINT('Ctrl Pts',(-3.75775357067056,6.97689187339913,-68.331958489734));
#33596=CARTESIAN_POINT('Ctrl Pts',(-3.75790811579813,7.91598173799435,-70.0913522764039));
#33597=CARTESIAN_POINT('Ctrl Pts',(-3.75851702956022,8.7129544406287,-71.56741993476));
#33598=CARTESIAN_POINT('Ctrl Pts',(-3.75851139507746,9.30780849071006,-72.6861960657986));
#33599=CARTESIAN_POINT('Ctrl Pts',(-3.75850965202096,9.44162253911425,-72.9378654400856));
#33600=CARTESIAN_POINT('Ctrl Pts',(-3.7585072672047,9.70842045664312,-73.439642572339));
#33601=CARTESIAN_POINT('Ctrl Pts',(-3.75850659091144,10.042067263661,-74.0671451260673));
#33602=CARTESIAN_POINT('Ctrl Pts',(-3.7585068904606,10.4420495799701,-74.8194037887349));
#33603=CARTESIAN_POINT('Ctrl Pts',(-3.75851012699749,11.2418168738129,-76.3235472418929));
#33604=CARTESIAN_POINT('Ctrl Pts',(-3.75851897726527,11.9080053917647,-77.576469362933));
#33605=CARTESIAN_POINT('Ctrl Pts',(-3.75852120334172,12.877917815396,-79.4006144962138));
#33606=CARTESIAN_POINT('Ctrl Pts',(-3.75852234907699,13.3144832846348,-80.2216773890785));
#33607=CARTESIAN_POINT('Ctrl Pts',(-3.75852234907698,13.7510048720243,-81.0426550911768));
#33608=CARTESIAN_POINT('Ctrl Pts',(-1.87922647318657,7.43659936946723E-5,
24.8306346358243));
#33609=CARTESIAN_POINT('Ctrl Pts',(-1.8792320812944,7.43682799464241E-5,
24.781755319639));
#33610=CARTESIAN_POINT('Ctrl Pts',(-1.87923794877265,7.43856257991035E-5,
24.7328772901569));
#33611=CARTESIAN_POINT('Ctrl Pts',(-1.87930788335411,7.39106761634475E-5,
24.1822613292266));
#33612=CARTESIAN_POINT('Ctrl Pts',(-1.87936495452039,6.97862600438643E-5,
23.1780605579904));
#33613=CARTESIAN_POINT('Ctrl Pts',(-1.87948882589249,6.95445524143603E-5,
21.1694547708657));
#33614=CARTESIAN_POINT('Ctrl Pts',(-1.87996099259776,5.92851299646219E-5,
19.6651394211573));
#33615=CARTESIAN_POINT('Ctrl Pts',(-1.88094643808592,5.48594906311521E-5,
18.4140198688397));
#33616=CARTESIAN_POINT('Ctrl Pts',(-1.88141759062512,5.42365496829209E-5,
17.9111924083393));
#33617=CARTESIAN_POINT('Ctrl Pts',(-1.88260171332622,5.1515615193511E-5,
16.9071564758307));
#33618=CARTESIAN_POINT('Ctrl Pts',(-1.8851386273318,4.8840807487355E-5,
15.1532969718806));
#33619=CARTESIAN_POINT('Ctrl Pts',(-1.88756917454291,2.5212297710916E-5,
13.6511807365289));
#33620=CARTESIAN_POINT('Ctrl Pts',(-1.88909132532381,1.31179185919511E-5,
12.3965299246728));
#33621=CARTESIAN_POINT('Ctrl Pts',(-1.88971089815823,1.12234742488184E-5,
11.8955257512763));
#33622=CARTESIAN_POINT('Ctrl Pts',(-1.89097888630937,2.29670390858633E-6,
10.8936285883835));
#33623=CARTESIAN_POINT('Ctrl Pts',(-1.89316912932919,-6.67277562029711E-6,
9.13968656717126));
#33624=CARTESIAN_POINT('Ctrl Pts',(-1.89476488907268,-7.75933543378677E-5,
7.634263797525));
#33625=CARTESIAN_POINT('Ctrl Pts',(-1.89546999666034,-9.98435924221817E-5,
6.50081894633009));
#33626=CARTESIAN_POINT('Ctrl Pts',(-1.89572526873683,0.00230665268363747,
6.22211902701521));
#33627=CARTESIAN_POINT('Ctrl Pts',(-1.89656984995772,0.0147464668667423,
5.6901431042027));
#33628=CARTESIAN_POINT('Ctrl Pts',(-1.89870974110295,0.0509275694207369,
4.77316994900257));
#33629=CARTESIAN_POINT('Ctrl Pts',(-1.90384887013271,0.143249196984895,
3.03555484961679));
#33630=CARTESIAN_POINT('Ctrl Pts',(-1.90386759788697,0.135196680509002,
1.70833859041381));
#33631=CARTESIAN_POINT('Ctrl Pts',(-1.89609045310109,0.0134334976845784,
0.851658950433416));
#33632=CARTESIAN_POINT('Ctrl Pts',(-1.89507277414501,-0.000596206126116792,
0.761097201393625));
#33633=CARTESIAN_POINT('Ctrl Pts',(-1.89274386758357,-0.0350229766227751,
0.568310331140751));
#33634=CARTESIAN_POINT('Ctrl Pts',(-1.88794310623562,-0.108513562227805,
0.222760045781302));
#33635=CARTESIAN_POINT('Ctrl Pts',(-1.87945425802549,-0.251368970401314,
-0.305671681892107));
#33636=CARTESIAN_POINT('Ctrl Pts',(-1.86741465521342,-0.47234244992444,
-0.986225583648586));
#33637=CARTESIAN_POINT('Ctrl Pts',(-1.85007936140568,-0.813435797702823,
-1.95268467358928));
#33638=CARTESIAN_POINT('Ctrl Pts',(-1.82713104757049,-1.28439221945105,
-3.26444308371993));
#33639=CARTESIAN_POINT('Ctrl Pts',(-1.81144354971363,-1.5984732684984,-4.44282707602525));
#33640=CARTESIAN_POINT('Ctrl Pts',(-1.80476245096426,-1.72725980926203,
-5.22829718654077));
#33641=CARTESIAN_POINT('Ctrl Pts',(-1.80253991577537,-1.76890705186197,
-5.50734875644929));
#33642=CARTESIAN_POINT('Ctrl Pts',(-1.79872094345382,-1.83981142184769,
-6.07911225865069));
#33643=CARTESIAN_POINT('Ctrl Pts',(-1.79397191736841,-1.92574635832976,
-7.05450848993233));
#33644=CARTESIAN_POINT('Ctrl Pts',(-1.79134660398458,-1.96941694501554,
-8.40664655582761));
#33645=CARTESIAN_POINT('Ctrl Pts',(-1.7912688089539,-1.96525359414387,-9.68812119753314));
#33646=CARTESIAN_POINT('Ctrl Pts',(-1.79107002876421,-1.96460551414136,
-10.549293763825));
#33647=CARTESIAN_POINT('Ctrl Pts',(-1.79075743910556,-1.96817078064357,
-11.03032083609));
#33648=CARTESIAN_POINT('Ctrl Pts',(-1.79050564371391,-1.97182966370674,
-11.267085603225));
#33649=CARTESIAN_POINT('Ctrl Pts',(-1.79026848438622,-1.97548562812885,
-11.4443732616452));
#33650=CARTESIAN_POINT('Ctrl Pts',(-1.79010312595948,-1.97805319876885,
-11.5768525465978));
#33651=CARTESIAN_POINT('Ctrl Pts',(-1.78981400359038,-1.98239200926529,
-11.83366297907));
#33652=CARTESIAN_POINT('Ctrl Pts',(-1.78939243224564,-1.98847129358254,
-12.2853409495223));
#33653=CARTESIAN_POINT('Ctrl Pts',(-1.78872477134816,-1.99670111738816,
-13.4361160012765));
#33654=CARTESIAN_POINT('Ctrl Pts',(-1.78892194409522,-1.98938784146963,
-14.6974250005926));
#33655=CARTESIAN_POINT('Ctrl Pts',(-1.7892358485117,-1.9805396995022,-15.9474018586027));
#33656=CARTESIAN_POINT('Ctrl Pts',(-1.78938855573791,-1.97693589443852,
-16.5707912522935));
#33657=CARTESIAN_POINT('Ctrl Pts',(-1.78945400749427,-1.97526103685482,
-17.068792009475));
#33658=CARTESIAN_POINT('Ctrl Pts',(-1.78946777988097,-1.97494395888634,
-17.3176657243817));
#33659=CARTESIAN_POINT('Ctrl Pts',(-1.78946661540154,-1.97494499467903,
-17.5035835075773));
#33660=CARTESIAN_POINT('Ctrl Pts',(-1.7894691915749,-1.97494635491117,-17.6286867178594));
#33661=CARTESIAN_POINT('Ctrl Pts',(-1.78948555236713,-1.97495114467567,
-17.8777132092247));
#33662=CARTESIAN_POINT('Ctrl Pts',(-1.78952096602998,-1.97495958507703,
-18.1273468564737));
#33663=CARTESIAN_POINT('Ctrl Pts',(-1.78956735566838,-1.97496935158133,
-18.3768644877724));
#33664=CARTESIAN_POINT('Ctrl Pts',(-1.78960181669949,-1.9749762550401,-18.5329270333045));
#33665=CARTESIAN_POINT('Ctrl Pts',(-1.78963162475722,-1.97498194350401,
-18.6577906642006));
#33666=CARTESIAN_POINT('Ctrl Pts',(-1.78966291596671,-1.97498768563792,
-18.782683892236));
#33667=CARTESIAN_POINT('Ctrl Pts',(-1.78975753412344,-1.97500524550039,
-19.1262339458842));
#33668=CARTESIAN_POINT('Ctrl Pts',(-1.78993935028022,-1.97503357614361,
-19.6889521983325));
#33669=CARTESIAN_POINT('Ctrl Pts',(-1.79029584480078,-1.9750781273811,-20.6909515915249));
#33670=CARTESIAN_POINT('Ctrl Pts',(-1.79064055534606,-1.97505601143599,
-21.9466759565142));
#33671=CARTESIAN_POINT('Ctrl Pts',(-1.79060445085998,-1.97491323922974,
-22.9549969094165));
#33672=CARTESIAN_POINT('Ctrl Pts',(-1.79037559502688,-1.97474017900966,
-23.5847448392945));
#33673=CARTESIAN_POINT('Ctrl Pts',(-1.79026154891338,-1.97465962601369,
-23.8340744749038));
#33674=CARTESIAN_POINT('Ctrl Pts',(-1.78996266815782,-1.97446464689011,
-24.3334733094898));
#33675=CARTESIAN_POINT('Ctrl Pts',(-1.78927381304738,-1.97404218711815,
-25.209165972539));
#33676=CARTESIAN_POINT('Ctrl Pts',(-1.78798170886171,-1.97329878314502,
-26.4641179004378));
#33677=CARTESIAN_POINT('Ctrl Pts',(-1.78632982209942,-1.97235667129645,
-27.9720281857487));
#33678=CARTESIAN_POINT('Ctrl Pts',(-1.78549155115143,-1.97187672496451,
-28.9769975495061));
#33679=CARTESIAN_POINT('Ctrl Pts',(-1.78516656839224,-1.97167625059406,
-29.539906341611));
#33680=CARTESIAN_POINT('Ctrl Pts',(-1.7850666350457,-1.97215941396197,-29.6497164037394));
#33681=CARTESIAN_POINT('Ctrl Pts',(-1.78477169972964,-1.97505395985333,
-29.8807066150062));
#33682=CARTESIAN_POINT('Ctrl Pts',(-1.78402113263626,-1.98480013300052,
-30.2868589688187));
#33683=CARTESIAN_POINT('Ctrl Pts',(-1.78179302898577,-2.01927945684624,
-31.1279979786219));
#33684=CARTESIAN_POINT('Ctrl Pts',(-1.77843455939292,-2.07555131660762,
-32.1444463451454));
#33685=CARTESIAN_POINT('Ctrl Pts',(-1.7765632735973,-2.10549056347651,-33.2177245662806));
#33686=CARTESIAN_POINT('Ctrl Pts',(-1.77660523082701,-2.10175494826061,
-34.0502763097447));
#33687=CARTESIAN_POINT('Ctrl Pts',(-1.77880766198053,-2.05817849987701,
-34.9106733776414));
#33688=CARTESIAN_POINT('Ctrl Pts',(-1.7822325000575,-1.9926391339686,-35.5011482024419));
#33689=CARTESIAN_POINT('Ctrl Pts',(-1.78574196680919,-1.92562867740721,
-35.9515064265878));
#33690=CARTESIAN_POINT('Ctrl Pts',(-1.78873960982218,-1.86856136255701,
-36.2760710728659));
#33691=CARTESIAN_POINT('Ctrl Pts',(-1.79585687226293,-1.73081723039962,
-36.8883400341203));
#33692=CARTESIAN_POINT('Ctrl Pts',(-1.81071819779439,-1.43672452638524,
-37.9152325486312));
#33693=CARTESIAN_POINT('Ctrl Pts',(-1.84411300428762,-0.74008290519004,
-39.776554008902));
#33694=CARTESIAN_POINT('Ctrl Pts',(-1.86996309579029,-0.254721573964913,
-41.1127718926262));
#33695=CARTESIAN_POINT('Ctrl Pts',(-1.87944574652515,-0.120250328587189,
-41.9361856957747));
#33696=CARTESIAN_POINT('Ctrl Pts',(-1.88141687474336,-0.0904963193764836,
-42.1412581804935));
#33697=CARTESIAN_POINT('Ctrl Pts',(-1.88383775239668,-0.057328381547109,
-42.4473311457505));
#33698=CARTESIAN_POINT('Ctrl Pts',(-1.88579098865738,-0.032482726045188,
-42.7656755195937));
#33699=CARTESIAN_POINT('Ctrl Pts',(-1.88780408608839,-0.0104078350965731,
-43.2000369215372));
#33700=CARTESIAN_POINT('Ctrl Pts',(-1.88934964918851,-0.000417930478199928,
-43.766216661788));
#33701=CARTESIAN_POINT('Ctrl Pts',(-1.89005786507775,-0.00781083470753425,
-44.4806607424834));
#33702=CARTESIAN_POINT('Ctrl Pts',(-1.8900503045469,-0.0209520131984904,
-45.1051803940128));
#33703=CARTESIAN_POINT('Ctrl Pts',(-1.88995893058319,-0.029260011726896,
-45.6221161988452));
#33704=CARTESIAN_POINT('Ctrl Pts',(-1.88987679081064,-0.0326211432941866,
-46.0183182336727));
#33705=CARTESIAN_POINT('Ctrl Pts',(-1.88984019143788,-0.0312522604122497,
-46.4230535672428));
#33706=CARTESIAN_POINT('Ctrl Pts',(-1.88994150500147,-0.0204579713078959,
-46.9739112286859));
#33707=CARTESIAN_POINT('Ctrl Pts',(-1.89021927414918,0.000847090578713871,
-47.3997344095905));
#33708=CARTESIAN_POINT('Ctrl Pts',(-1.89079622330981,0.035450677665807,
-47.8334166079678));
#33709=CARTESIAN_POINT('Ctrl Pts',(-1.89118518624509,0.0548291878842356,
-48.0754222563547));
#33710=CARTESIAN_POINT('Ctrl Pts',(-1.8919684497567,0.096849072818417,-48.5899868840785));
#33711=CARTESIAN_POINT('Ctrl Pts',(-1.89331811174698,0.173463964332855,
-49.4834687046147));
#33712=CARTESIAN_POINT('Ctrl Pts',(-1.89500374569028,0.304184643793816,
-50.7883449345947));
#33713=CARTESIAN_POINT('Ctrl Pts',(-1.8963558861006,0.522336541724754,-52.3802914310615));
#33714=CARTESIAN_POINT('Ctrl Pts',(-1.8964105023605,0.729306886905037,-53.4613249704202));
#33715=CARTESIAN_POINT('Ctrl Pts',(-1.89613100861477,0.884610861304433,
-54.1427419720713));
#33716=CARTESIAN_POINT('Ctrl Pts',(-1.89598303975611,0.947891669923935,
-54.411771836144));
#33717=CARTESIAN_POINT('Ctrl Pts',(-1.89551625297565,1.0825818126608,-54.9518990099226));
#33718=CARTESIAN_POINT('Ctrl Pts',(-1.89430851430286,1.33651472026183,-55.8919087552172));
#33719=CARTESIAN_POINT('Ctrl Pts',(-1.89076753071172,1.91341936868272,-57.7581455372565));
#33720=CARTESIAN_POINT('Ctrl Pts',(-1.88722362432661,2.50596526061431,-59.3238337112826));
#33721=CARTESIAN_POINT('Ctrl Pts',(-1.88572660967207,2.95620938582178,-60.4150899796445));
#33722=CARTESIAN_POINT('Ctrl Pts',(-1.88553601853826,3.0148726044652,-60.5555183564978));
#33723=CARTESIAN_POINT('Ctrl Pts',(-1.88516359548367,3.13255149157178,-60.8304824737814));
#33724=CARTESIAN_POINT('Ctrl Pts',(-1.88452291602286,3.34496050530911,-61.3106450471766));
#33725=CARTESIAN_POINT('Ctrl Pts',(-1.88329441022756,3.78808659672977,-62.2559809772548));
#33726=CARTESIAN_POINT('Ctrl Pts',(-1.8820565125292,4.32512291249686,-63.3081334059565));
#33727=CARTESIAN_POINT('Ctrl Pts',(-1.88099241764672,4.86639785683072,-64.3295005770627));
#33728=CARTESIAN_POINT('Ctrl Pts',(-1.8804627043064,5.16788755886044,-64.8921173663213));
#33729=CARTESIAN_POINT('Ctrl Pts',(-1.88014234675638,5.36564326557466,-65.2618246643185));
#33730=CARTESIAN_POINT('Ctrl Pts',(-1.87993629780318,5.49648934849498,-65.5068329550256));
#33731=CARTESIAN_POINT('Ctrl Pts',(-1.87974758568304,5.62567418338341,-65.7496459357718));
#33732=CARTESIAN_POINT('Ctrl Pts',(-1.87959264777368,5.73689111164499,-65.9600447305898));
#33733=CARTESIAN_POINT('Ctrl Pts',(-1.87950787055948,5.79987661251178,-66.0796720507273));
#33734=CARTESIAN_POINT('Ctrl Pts',(-1.87938419873138,5.89377044043449,-66.2585180400154));
#33735=CARTESIAN_POINT('Ctrl Pts',(-1.8792911987843,5.97072364200638,-66.406257209168));
#33736=CARTESIAN_POINT('Ctrl Pts',(-1.87914620246728,6.09633077364163,-66.6493895977556));
#33737=CARTESIAN_POINT('Ctrl Pts',(-1.87901599600879,6.23397804167784,-66.9148991361219));
#33738=CARTESIAN_POINT('Ctrl Pts',(-1.87882043496205,6.5041293622886,-67.4326003206522));
#33739=CARTESIAN_POINT('Ctrl Pts',(-1.87864116952207,6.97757390129021,-68.3320115836156));
#33740=CARTESIAN_POINT('Ctrl Pts',(-1.87875637389118,7.91634431697053,-70.0909885233312));
#33741=CARTESIAN_POINT('Ctrl Pts',(-1.87920310482,8.71296113698193,-71.5671554587218));
#33742=CARTESIAN_POINT('Ctrl Pts',(-1.87920409650289,9.30797701881977,-72.6862204452462));
#33743=CARTESIAN_POINT('Ctrl Pts',(-1.87920288711204,9.4417816722211,-72.937868851734));
#33744=CARTESIAN_POINT('Ctrl Pts',(-1.87920154950468,9.70858596207869,-73.439653172257));
#33745=CARTESIAN_POINT('Ctrl Pts',(-1.87920244898022,10.0422290067306,-74.0671457930824));
#33746=CARTESIAN_POINT('Ctrl Pts',(-1.87920330165399,10.4422110758571,-74.8194038178528));
#33747=CARTESIAN_POINT('Ctrl Pts',(-1.8792068113137,11.2419727933141,-76.3235413741309));
#33748=CARTESIAN_POINT('Ctrl Pts',(-1.87921800986231,11.9081567732661,-77.5764657951134));
#33749=CARTESIAN_POINT('Ctrl Pts',(-1.87922251549513,12.8780717022048,-79.4006164692795));
#33750=CARTESIAN_POINT('Ctrl Pts',(-1.8792248343783,13.3146358968538,-80.2216773916581));
#33751=CARTESIAN_POINT('Ctrl Pts',(-1.87922483437827,13.7511574842433,-81.0426550937565));
#33752=CARTESIAN_POINT('Ctrl Pts',(-7.86816895413843E-6,0.000134138085496685,
24.8306345586402));
#33753=CARTESIAN_POINT('Ctrl Pts',(-7.86837039397705E-6,0.0001341424751082,
24.7817552401123));
#33754=CARTESIAN_POINT('Ctrl Pts',(-7.86758228674821E-6,0.000134149695995169,
24.7328772070671));
#33755=CARTESIAN_POINT('Ctrl Pts',(-7.90367859151917E-6,0.00013411567282899,
24.1822612582853));
#33756=CARTESIAN_POINT('Ctrl Pts',(-8.18809680975969E-6,0.000133513032849035,
23.1780607854083));
#33757=CARTESIAN_POINT('Ctrl Pts',(-8.23189606488739E-6,0.000133804106629631,
21.169454983822));
#33758=CARTESIAN_POINT('Ctrl Pts',(-8.93959770906373E-6,0.00013233366932893,
19.6651404452238));
#33759=CARTESIAN_POINT('Ctrl Pts',(-9.2601353069708E-6,0.000131836478995296,
18.4140212479634));
#33760=CARTESIAN_POINT('Ctrl Pts',(-9.31855293916846E-6,0.000131891105320219,
17.91119370092));
#33761=CARTESIAN_POINT('Ctrl Pts',(-9.53558031351182E-6,0.000131877154863405,
16.9071579078805));
#33762=CARTESIAN_POINT('Ctrl Pts',(-9.81102603618544E-6,0.000132380618664769,
15.1532986547908));
#33763=CARTESIAN_POINT('Ctrl Pts',(-1.13163675539412E-5,0.000128697056927304,
13.6511848101255));
#33764=CARTESIAN_POINT('Ctrl Pts',(-1.20215489539955E-5,0.00012598731728272,
12.3965353750791));
#33765=CARTESIAN_POINT('Ctrl Pts',(-1.21198252440109E-5,0.000125354011049059,
11.8955321306931));
#33766=CARTESIAN_POINT('Ctrl Pts',(-1.25719075545662E-5,0.000122663548405129,
10.893634209687));
#33767=CARTESIAN_POINT('Ctrl Pts',(-1.29806635370252E-5,0.000119128674288264,
9.13969986849073));
#33768=CARTESIAN_POINT('Ctrl Pts',(-1.68084968046005E-5,0.000102911589896075,
7.63426186513583));
#33769=CARTESIAN_POINT('Ctrl Pts',(-1.82403447152679E-5,0.00010109573980971,
6.50086936027134));
#33770=CARTESIAN_POINT('Ctrl Pts',(-1.64601354838555E-5,0.00244662050690851,
6.2228498478194));
#33771=CARTESIAN_POINT('Ctrl Pts',(-6.73044822835249E-6,0.014572420864447,
5.69161192423943));
#33772=CARTESIAN_POINT('Ctrl Pts',(2.07135641908368E-5,0.0498770565337277,
4.77553942507642));
#33773=CARTESIAN_POINT('Ctrl Pts',(9.95496872622605E-5,0.14000092241698,
3.03741192946093));
#33774=CARTESIAN_POINT('Ctrl Pts',(8.35363358727937E-5,0.132494558618385,
1.70571827028138));
#33775=CARTESIAN_POINT('Ctrl Pts',(-4.3165465129633E-5,0.0131276052745993,
0.844409225479565));
#33776=CARTESIAN_POINT('Ctrl Pts',(-5.87456527449067E-5,-0.000678586975984755,
0.753045172446035));
#33777=CARTESIAN_POINT('Ctrl Pts',(-9.40682916947416E-5,-0.0344900533728886,
0.558952015873453));
#33778=CARTESIAN_POINT('Ctrl Pts',(-0.000164093499659093,-0.106614488837571,
0.211381380066455));
#33779=CARTESIAN_POINT('Ctrl Pts',(-0.000283606969796099,-0.246519397169534,
-0.318981240870596));
#33780=CARTESIAN_POINT('Ctrl Pts',(-0.000438074335267664,-0.462725653626534,
-1.00076418485887));
#33781=CARTESIAN_POINT('Ctrl Pts',(-0.00067632928056198,-0.796092318982456,
-1.96767603702569));
#33782=CARTESIAN_POINT('Ctrl Pts',(-0.00104113729596573,-1.25617217791027,
-3.27826183066476));
#33783=CARTESIAN_POINT('Ctrl Pts',(-0.00144925043470265,-1.56238495854328,
-4.45318358255805));
#33784=CARTESIAN_POINT('Ctrl Pts',(-0.00164344066864579,-1.68786141248603,
-5.23520500674852));
#33785=CARTESIAN_POINT('Ctrl Pts',(-0.00169780486768979,-1.72854156947398,
-5.513626473583));
#33786=CARTESIAN_POINT('Ctrl Pts',(-0.00179701682113945,-1.79776427715872,
-6.08382750946227));
#33787=CARTESIAN_POINT('Ctrl Pts',(-0.00191717498362644,-1.88171648309701,
-7.05701935378413));
#33788=CARTESIAN_POINT('Ctrl Pts',(-0.00197726410329787,-1.92440052183823,
-8.40693623429189));
#33789=CARTESIAN_POINT('Ctrl Pts',(-0.00196970659771493,-1.92031956974289,
-9.68777019145027));
#33790=CARTESIAN_POINT('Ctrl Pts',(-0.00196543564596002,-1.91971220554664,
-10.5492737685884));
#33791=CARTESIAN_POINT('Ctrl Pts',(-0.00196716279840418,-1.9232243570222,
-11.0307243359037));
#33792=CARTESIAN_POINT('Ctrl Pts',(-0.0019700711110791,-1.9268200043073,
-11.2677791491987));
#33793=CARTESIAN_POINT('Ctrl Pts',(-0.00197308324111247,-1.93041253094738,
-11.4453057330445));
#33794=CARTESIAN_POINT('Ctrl Pts',(-0.00197588354150194,-1.93292971573111,
-11.5776350827829));
#33795=CARTESIAN_POINT('Ctrl Pts',(-0.00197997062913887,-1.93718924689335,
-11.8343290274479));
#33796=CARTESIAN_POINT('Ctrl Pts',(-0.00198541577020757,-1.94315917627825,
-12.2857350678419));
#33797=CARTESIAN_POINT('Ctrl Pts',(-0.00199021190869098,-1.95125874518291,
-13.435990027481));
#33798=CARTESIAN_POINT('Ctrl Pts',(-0.00197629221165083,-1.94412854859148,
-14.6969941891685));
#33799=CARTESIAN_POINT('Ctrl Pts',(-0.00196013412846356,-1.93551323635508,
-15.9470316019288));
#33800=CARTESIAN_POINT('Ctrl Pts',(-0.00195528042777413,-1.93199060585446,
-16.5705240611153));
#33801=CARTESIAN_POINT('Ctrl Pts',(-0.0019525135633656,-1.93035800022109,
-17.0686604800003));
#33802=CARTESIAN_POINT('Ctrl Pts',(-0.00195230352912211,-1.93004766012124,
-17.3176175926851));
#33803=CARTESIAN_POINT('Ctrl Pts',(-0.00195233573781056,-1.93004894171476,
-17.5036021570554));
#33804=CARTESIAN_POINT('Ctrl Pts',(-0.00195236553761999,-1.93005065707797,
-17.628681641473));
#33805=CARTESIAN_POINT('Ctrl Pts',(-0.00195222219453429,-1.93005739523279,
-17.877702982022));
#33806=CARTESIAN_POINT('Ctrl Pts',(-0.00195260067372203,-1.93006735831943,
-18.1273192668479));
#33807=CARTESIAN_POINT('Ctrl Pts',(-0.00195239498154048,-1.93008052775035,
-18.3768312531958));
#33808=CARTESIAN_POINT('Ctrl Pts',(-0.00195238244644089,-1.93008945422298,
-18.5328897673755));
#33809=CARTESIAN_POINT('Ctrl Pts',(-0.00195228565643687,-1.93009698291304,
-18.6577517412467));
#33810=CARTESIAN_POINT('Ctrl Pts',(-0.00195212946204278,-1.93010456739087,
-18.7826436765513));
#33811=CARTESIAN_POINT('Ctrl Pts',(-0.00195265544136155,-1.93012668860778,
-19.1261923033247));
#33812=CARTESIAN_POINT('Ctrl Pts',(-0.00195299924847534,-1.93016069924505,
-19.6889203191277));
#33813=CARTESIAN_POINT('Ctrl Pts',(-0.0019628499729974,-1.93020222093941,
-20.6909711259829));
#33814=CARTESIAN_POINT('Ctrl Pts',(-0.00197359275882038,-1.93013298869328,
-21.9468251921027));
#33815=CARTESIAN_POINT('Ctrl Pts',(-0.00200870222067299,-1.92987326196219,
-22.9553165950121));
#33816=CARTESIAN_POINT('Ctrl Pts',(-0.00202556675274397,-1.92958934005298,
-23.5851939129496));
#33817=CARTESIAN_POINT('Ctrl Pts',(-0.00203145635328623,-1.92945901432285,
-23.8346016612358));
#33818=CARTESIAN_POINT('Ctrl Pts',(-0.00204696141433901,-1.92914542303968,
-24.3341202973898));
#33819=CARTESIAN_POINT('Ctrl Pts',(-0.00207837479126103,-1.92846700729011,
-25.2099864486648));
#33820=CARTESIAN_POINT('Ctrl Pts',(-0.00215156754501358,-1.92728229243832,
-26.4650381951777));
#33821=CARTESIAN_POINT('Ctrl Pts',(-0.00222333586556621,-1.92577926784895,
-27.9728776779655));
#33822=CARTESIAN_POINT('Ctrl Pts',(-0.00228055085845308,-1.92502813324683,
-28.9776299813488));
#33823=CARTESIAN_POINT('Ctrl Pts',(-0.002298177987237,-1.92470980210758,
-29.5404151696509));
#33824=CARTESIAN_POINT('Ctrl Pts',(-0.00230130766395741,-1.92516042605284,
-29.6505728721337));
#33825=CARTESIAN_POINT('Ctrl Pts',(-0.00230978503821261,-1.92795253854498,
-29.8819857404979));
#33826=CARTESIAN_POINT('Ctrl Pts',(-0.00233059546001059,-1.93743770191964,
-30.288842694958));
#33827=CARTESIAN_POINT('Ctrl Pts',(-0.00239052663365571,-1.97110017924892,
-31.1307375695758));
#33828=CARTESIAN_POINT('Ctrl Pts',(-0.00248975575594169,-2.02609596226747,
-32.1468124521085));
#33829=CARTESIAN_POINT('Ctrl Pts',(-0.00255393362773429,-2.05528304965543,
-33.2184453682104));
#33830=CARTESIAN_POINT('Ctrl Pts',(-0.00255607068676999,-2.05156741016729,
-34.0491340814343));
#33831=CARTESIAN_POINT('Ctrl Pts',(-0.00248991705472534,-2.00898197987319,
-34.9070215761246));
#33832=CARTESIAN_POINT('Ctrl Pts',(-0.0023793876735871,-1.94501401488239,
-35.4954627611981));
#33833=CARTESIAN_POINT('Ctrl Pts',(-0.00226892854331357,-1.87962048862466,
-35.9441896793407));
#33834=CARTESIAN_POINT('Ctrl Pts',(-0.00216704516292421,-1.8240010896022,
-36.2672021766089));
#33835=CARTESIAN_POINT('Ctrl Pts',(-0.00195357476185786,-1.68961350158174,
-36.8772308283305));
#33836=CARTESIAN_POINT('Ctrl Pts',(-0.00155117525253687,-1.40258216824729,
-37.9012275834125));
#33837=CARTESIAN_POINT('Ctrl Pts',(-0.000952370227631846,-0.721863588740229,
-39.7604638106087));
#33838=CARTESIAN_POINT('Ctrl Pts',(-0.000618816224572059,-0.247226512287369,
-41.0986235843677));
#33839=CARTESIAN_POINT('Ctrl Pts',(-0.000457042263932061,-0.115183321968809,
-41.9287308981079));
#33840=CARTESIAN_POINT('Ctrl Pts',(-0.000425764461784592,-0.0860929365982914,
-42.1345110983509));
#33841=CARTESIAN_POINT('Ctrl Pts',(-0.000383611275539338,-0.0537133742847068,
-42.4419305296188));
#33842=CARTESIAN_POINT('Ctrl Pts',(-0.000348398037189352,-0.0295622812038002,
-42.7613877270058));
#33843=CARTESIAN_POINT('Ctrl Pts',(-0.000307974476746251,-0.00823942687768989,
-43.1971433320679));
#33844=CARTESIAN_POINT('Ctrl Pts',(-0.000271596152705288,0.00109993840456285,
-43.7647049359353));
#33845=CARTESIAN_POINT('Ctrl Pts',(-0.000241129946027054,-0.00666211470508639,
-44.4802635490114));
#33846=CARTESIAN_POINT('Ctrl Pts',(-0.000218092509743048,-0.0198790964273407,
-45.105238504849));
#33847=CARTESIAN_POINT('Ctrl Pts',(-0.000210848210031528,-0.0281666779737864,
-45.6222574130482));
#33848=CARTESIAN_POINT('Ctrl Pts',(-0.000203131619834829,-0.0315153753063813,
-46.0183819397791));
#33849=CARTESIAN_POINT('Ctrl Pts',(-0.000192990095033107,-0.0301650435608711,
-46.422899151946));
#33850=CARTESIAN_POINT('Ctrl Pts',(-0.000179976946274749,-0.0194765785343918,
-46.9732794940509));
#33851=CARTESIAN_POINT('Ctrl Pts',(-0.000152921065464157,0.00157914786618924,
-47.3985344890977));
#33852=CARTESIAN_POINT('Ctrl Pts',(-0.000130616097718489,0.0357606605654795,
-47.8315319828244));
#33853=CARTESIAN_POINT('Ctrl Pts',(-0.000115589656268732,0.0549381457458591,
-48.0736438273212));
#33854=CARTESIAN_POINT('Ctrl Pts',(-8.29538197244078E-5,0.0965018439824387,
-48.5881247084077));
#33855=CARTESIAN_POINT('Ctrl Pts',(-1.89201302580575E-5,0.172330139091039,
-49.4816721346524));
#33856=CARTESIAN_POINT('Ctrl Pts',(0.000104768315615061,0.301924242134264,
-50.786702156654));
#33857=CARTESIAN_POINT('Ctrl Pts',(0.000218759891771719,0.519013310827141,
-52.3791099138675));
#33858=CARTESIAN_POINT('Ctrl Pts',(0.000287059711293618,0.725574522676222,
-53.4605852128649));
#33859=CARTESIAN_POINT('Ctrl Pts',(0.000304880749959895,0.880778148203204,
-54.14231167573));
#33860=CARTESIAN_POINT('Ctrl Pts',(0.000309049917928886,0.944038711403875,
-54.4114723712317));
#33861=CARTESIAN_POINT('Ctrl Pts',(0.000313322841748133,1.07873450151376,
-54.9518265359057));
#33862=CARTESIAN_POINT('Ctrl Pts',(0.000314429842083324,1.3327900865459,
-55.8921728030728));
#33863=CARTESIAN_POINT('Ctrl Pts',(0.000284882742374926,1.91027806491778,
-57.7588207333756));
#33864=CARTESIAN_POINT('Ctrl Pts',(0.000237836621859263,2.50353264792865,
-59.3244902541145));
#33865=CARTESIAN_POINT('Ctrl Pts',(0.000214874912799959,2.95403965973707,
-60.4155795542004));
#33866=CARTESIAN_POINT('Ctrl Pts',(0.000211500358311257,3.01275985071423,
-60.5560389550589));
#33867=CARTESIAN_POINT('Ctrl Pts',(0.000204780571771536,3.13054311258116,
-60.8310316498565));
#33868=CARTESIAN_POINT('Ctrl Pts',(0.000191193440495367,3.34315184314077,
-61.3112496976771));
#33869=CARTESIAN_POINT('Ctrl Pts',(0.000162043330489063,3.78669936896942,
-62.2566494682892));
#33870=CARTESIAN_POINT('Ctrl Pts',(0.000118672692779613,4.32424582620751,
-63.3088124541968));
#33871=CARTESIAN_POINT('Ctrl Pts',(8.17628259240602E-5,4.86596465270228,
-64.3301283776222));
#33872=CARTESIAN_POINT('Ctrl Pts',(6.44246275231492E-5,5.16766507371822,
-64.8926939205394));
#33873=CARTESIAN_POINT('Ctrl Pts',(5.42269208335611E-5,5.36553930207075,
-65.262356915369));
#33874=CARTESIAN_POINT('Ctrl Pts',(4.83012049103832E-5,5.49645773933371,
-65.5073328453505));
#33875=CARTESIAN_POINT('Ctrl Pts',(4.1628878654448E-5,5.62570604049499,
-65.7501091651644));
#33876=CARTESIAN_POINT('Ctrl Pts',(3.72381543414075E-5,5.73696806356847,
-65.9604718020035));
#33877=CARTESIAN_POINT('Ctrl Pts',(3.48749553043657E-5,5.7999764236035,
-66.0800772441846));
#33878=CARTESIAN_POINT('Ctrl Pts',(3.15955711106227E-5,5.89390147861976,
-66.2588891870182));
#33879=CARTESIAN_POINT('Ctrl Pts',(2.84193281057929E-5,5.97087483489673,
-66.4065971904426));
#33880=CARTESIAN_POINT('Ctrl Pts',(2.44817438210786E-5,6.09650571081662,
-66.6496744393032));
#33881=CARTESIAN_POINT('Ctrl Pts',(2.04986805459089E-5,6.23418093562956,
-66.9151401191057));
#33882=CARTESIAN_POINT('Ctrl Pts',(1.48718372786516E-5,6.5043619711416,
-67.4327557777686));
#33883=CARTESIAN_POINT('Ctrl Pts',(6.62261016059817E-6,6.97781566951045,
-68.332042634089));
#33884=CARTESIAN_POINT('Ctrl Pts',(4.48053439701293E-6,7.91646970425133,
-70.0908617665458));
#33885=CARTESIAN_POINT('Ctrl Pts',(4.20848049135385E-6,8.71295983512131,
-71.5670614909078));
#33886=CARTESIAN_POINT('Ctrl Pts',(6.84354616859567E-7,9.30803814757989,
-72.6862328888755));
#33887=CARTESIAN_POINT('Ctrl Pts',(5.68114809718481E-7,9.44183934535038,
-72.9378734208353));
#33888=CARTESIAN_POINT('Ctrl Pts',(2.05586755580999E-7,9.70864620119544,
-73.4396602737137));
#33889=CARTESIAN_POINT('Ctrl Pts',(-7.21239062929604E-7,10.0422883693543,
-74.0671487882584));
#33890=CARTESIAN_POINT('Ctrl Pts',(-1.11438109418972E-6,10.442270567524,
-74.8194063862324));
#33891=CARTESIAN_POINT('Ctrl Pts',(-1.71035629119184E-6,11.2420305551737,
-76.3235414328312));
#33892=CARTESIAN_POINT('Ctrl Pts',(-4.32945481586382E-6,11.9082144683072,
-77.5764655497178));
#33893=CARTESIAN_POINT('Ctrl Pts',(-6.05635545269383E-6,12.8781314087794,
-79.4006176028791));
#33894=CARTESIAN_POINT('Ctrl Pts',(-6.94521695860565E-6,13.314695659481,
-80.2216773934557));
#33895=CARTESIAN_POINT('Ctrl Pts',(-6.94521697867286E-6,13.7512172468705,
-81.0426550955541));
#33896=CARTESIAN_POINT('Ctrl Pts',(1.87922065701991,7.61596117959377E-5,
24.8306346333771));
#33897=CARTESIAN_POINT('Ctrl Pts',(1.87922626560681,7.61620135603957E-5,
24.7817553171342));
#33898=CARTESIAN_POINT('Ctrl Pts',(1.87923216025948,7.61760040173549E-5,
24.7328772886127));
#33899=CARTESIAN_POINT('Ctrl Pts',(1.87930120315869,7.58194923152649E-5,
24.1822612927019));
#33900=CARTESIAN_POINT('Ctrl Pts',(1.87935079445246,7.26740057884463E-5,
23.1780602344503));
#33901=CARTESIAN_POINT('Ctrl Pts',(1.87947388483842,7.25425928646775E-5,
21.169454415134));
#33902=CARTESIAN_POINT('Ctrl Pts',(1.87992747111033,6.47238710413929E-5,
19.6651383523929));
#33903=CARTESIAN_POINT('Ctrl Pts',(1.88090486185821,6.13733892703204E-5,
18.4140184893336));
#33904=CARTESIAN_POINT('Ctrl Pts',(1.88137478720441,6.09217268373628E-5,
17.9111909771165));
#33905=CARTESIAN_POINT('Ctrl Pts',(1.88255374297555,5.89108913871656E-5,
16.9071548405334));
#33906=CARTESIAN_POINT('Ctrl Pts',(1.88508516688353,5.70155313945553E-5,
15.1532951221729));
#33907=CARTESIAN_POINT('Ctrl Pts',(1.88747375765592,3.89855064059539E-5,
13.651177276246));
#33908=CARTESIAN_POINT('Ctrl Pts',(1.8889753781808,2.96207864364287E-5,
12.3965256878489));
#33909=CARTESIAN_POINT('Ctrl Pts',(1.88959196096303,2.81242245297611E-5,
11.8955214044168));
#33910=CARTESIAN_POINT('Ctrl Pts',(1.8908457391163,2.10877770421448E-5,
10.893623706362));
#33911=CARTESIAN_POINT('Ctrl Pts',(1.89302201588768,1.3952629727407E-5,
9.13968114018261));
#33912=CARTESIAN_POINT('Ctrl Pts',(1.89449907752566,-4.11353129124917E-5,
7.63425381206281));
#33913=CARTESIAN_POINT('Ctrl Pts',(1.89515906367933,-5.7372725229025E-5,
6.50080706358199));
#33914=CARTESIAN_POINT('Ctrl Pts',(1.89540762219618,0.0023494898295555,
6.22210496316194));
#33915=CARTESIAN_POINT('Ctrl Pts',(1.89622309817872,0.0147904875425885,
5.69012664502278));
#33916=CARTESIAN_POINT('Ctrl Pts',(1.89824710817307,0.0509794365844755,
4.77314810156052));
#33917=CARTESIAN_POINT('Ctrl Pts',(1.90315893713563,0.143311521409256,3.0355352845081));
#33918=CARTESIAN_POINT('Ctrl Pts',(1.90277046926461,0.135314710798477,1.70830615109979));
#33919=CARTESIAN_POINT('Ctrl Pts',(1.89514572110263,0.0135512360379868,
0.851649839357737));
#33920=CARTESIAN_POINT('Ctrl Pts',(1.89416706532207,-0.000481487034814646,
0.761093637132466));
#33921=CARTESIAN_POINT('Ctrl Pts',(1.89191197327707,-0.0349124265759622,
0.568317371434498));
#33922=CARTESIAN_POINT('Ctrl Pts',(1.88726269607664,-0.108411282795717,
0.222787915872012));
#33923=CARTESIAN_POINT('Ctrl Pts',(1.87891203932446,-0.251263790050898,
-0.305614290368038));
#33924=CARTESIAN_POINT('Ctrl Pts',(1.8672190151571,-0.472266342518573,-0.986136213316851));
#33925=CARTESIAN_POINT('Ctrl Pts',(1.85019799115212,-0.813392882796135,
-1.95256231630457));
#33926=CARTESIAN_POINT('Ctrl Pts',(1.82794512867848,-1.28446993438294,-3.26430893703937));
#33927=CARTESIAN_POINT('Ctrl Pts',(1.81272281017777,-1.59859453901927,-4.44274312874163));
#33928=CARTESIAN_POINT('Ctrl Pts',(1.80638910274363,-1.7273997721369,-5.22825505005266));
#33929=CARTESIAN_POINT('Ctrl Pts',(1.80427869767207,-1.76905831655269,-5.50731245895802));
#33930=CARTESIAN_POINT('Ctrl Pts',(1.80065184481023,-1.83997895086455,-6.07909111574944));
#33931=CARTESIAN_POINT('Ctrl Pts',(1.79607620867608,-1.92592867677439,-7.05450472650263));
#33932=CARTESIAN_POINT('Ctrl Pts',(1.79334543307704,-1.96958741569615,-8.40665558072903));
#33933=CARTESIAN_POINT('Ctrl Pts',(1.79301141822182,-1.96539730646951,-9.68813059631163));
#33934=CARTESIAN_POINT('Ctrl Pts',(1.79274419096131,-1.96474439193333,-10.5492997925194));
#33935=CARTESIAN_POINT('Ctrl Pts',(1.79241023005762,-1.96830968052557,-11.0303231475472));
#33936=CARTESIAN_POINT('Ctrl Pts',(1.79215465822465,-1.97196962659183,-11.2670853827026));
#33937=CARTESIAN_POINT('Ctrl Pts',(1.79192032589268,-1.97562733286965,-11.4443710457125));
#33938=CARTESIAN_POINT('Ctrl Pts',(1.79175912918206,-1.9781959777931,-11.5768517128996));
#33939=CARTESIAN_POINT('Ctrl Pts',(1.79147608617423,-1.98253698716417,-11.8336633529133));
#33940=CARTESIAN_POINT('Ctrl Pts',(1.79105482303264,-1.98861872995816,-12.2853438149451));
#33941=CARTESIAN_POINT('Ctrl Pts',(1.79033442655468,-1.99684810126393,-13.4361224209512));
#33942=CARTESIAN_POINT('Ctrl Pts',(1.79037559992281,-1.98952102095365,-14.6974307834233));
#33943=CARTESIAN_POINT('Ctrl Pts',(1.79063171507148,-1.98067118531168,-15.9474082220266));
#33944=CARTESIAN_POINT('Ctrl Pts',(1.79073917055929,-1.97706320348729,-16.5707963211281));
#33945=CARTESIAN_POINT('Ctrl Pts',(1.79079316205804,-1.97538781040393,-17.0687964452538));
#33946=CARTESIAN_POINT('Ctrl Pts',(1.79079992984237,-1.97507008585841,-17.3176695608236));
#33947=CARTESIAN_POINT('Ctrl Pts',(1.79079700457479,-1.97507098594446,-17.5035869553218));
#33948=CARTESIAN_POINT('Ctrl Pts',(1.79079820480672,-1.97507223472088,-17.6286902970982));
#33949=CARTESIAN_POINT('Ctrl Pts',(1.79081303643941,-1.97507694677315,-17.8777168846834));
#33950=CARTESIAN_POINT('Ctrl Pts',(1.7908423737458,-1.97508492772897,-18.1273505684258));
#33951=CARTESIAN_POINT('Ctrl Pts',(1.7908870071724,-1.97509460752825,-18.3768683685547));
#33952=CARTESIAN_POINT('Ctrl Pts',(1.79091958228694,-1.97510139113122,-18.5329310092027));
#33953=CARTESIAN_POINT('Ctrl Pts',(1.7909485715885,-1.97510703421114,-18.6577947414661));
#33954=CARTESIAN_POINT('Ctrl Pts',(1.79097929787607,-1.97511272116633,-18.7826880802208));
#33955=CARTESIAN_POINT('Ctrl Pts',(1.79106851433894,-1.97513010281441,-19.1262383518251));
#33956=CARTESIAN_POINT('Ctrl Pts',(1.7912440182103,-1.97515778890431,-19.6889570515333));
#33957=CARTESIAN_POINT('Ctrl Pts',(1.79156652620716,-1.97520162435307,-20.6909569831857));
#33958=CARTESIAN_POINT('Ctrl Pts',(1.79190032472266,-1.97517555483402,-21.9466829676396));
#33959=CARTESIAN_POINT('Ctrl Pts',(1.79181893930524,-1.97502933168004,-22.9550048537654));
#33960=CARTESIAN_POINT('Ctrl Pts',(1.79160011312644,-1.97485112618095,-23.5847540984166));
#33961=CARTESIAN_POINT('Ctrl Pts',(1.79149584037637,-1.974767994845,-23.8340852761802));
#33962=CARTESIAN_POINT('Ctrl Pts',(1.79121783036047,-1.97456755508006,-24.3334861354704));
#33963=CARTESIAN_POINT('Ctrl Pts',(1.79057296578653,-1.97413291472412,-25.2091818472031));
#33964=CARTESIAN_POINT('Ctrl Pts',(1.78932843181765,-1.97337654638549,-26.4641335002892));
#33965=CARTESIAN_POINT('Ctrl Pts',(1.7877667392985,-1.97241463979719,-27.9720406937298));
#33966=CARTESIAN_POINT('Ctrl Pts',(1.78696631713144,-1.97193620457676,-28.9770024271066));
#33967=CARTESIAN_POINT('Ctrl Pts',(1.78666350274049,-1.97173369920145,-29.5399069473805));
#33968=CARTESIAN_POINT('Ctrl Pts',(1.78657098731778,-1.97221656613458,-29.6497131023628));
#33969=CARTESIAN_POINT('Ctrl Pts',(1.78629442080549,-1.9751112788456,-29.8806978494081));
#33970=CARTESIAN_POINT('Ctrl Pts',(1.7855939429116,-1.98486158926284,-30.2868406514868));
#33971=CARTESIAN_POINT('Ctrl Pts',(1.78349968794802,-2.01935510224964,-31.1279669106716));
#33972=CARTESIAN_POINT('Ctrl Pts',(1.78043296885725,-2.07565946440525,-32.1444103650944));
#33973=CARTESIAN_POINT('Ctrl Pts',(1.77875938834126,-2.10561496942114,-33.2176998689347));
#33974=CARTESIAN_POINT('Ctrl Pts',(1.77884649386387,-2.10188115948581,-34.0502677224308));
#33975=CARTESIAN_POINT('Ctrl Pts',(1.78097744958609,-2.05830577735026,-34.9106860529736));
#33976=CARTESIAN_POINT('Ctrl Pts',(1.78422692571106,-1.99276232309771,-35.5011821085368));
#33977=CARTESIAN_POINT('Ctrl Pts',(1.78750554178346,-1.92573953974817,-35.9515615389986));
#33978=CARTESIAN_POINT('Ctrl Pts',(1.79029021991389,-1.86866336738416,-36.276149755922));
#33979=CARTESIAN_POINT('Ctrl Pts',(1.79691647755597,-1.73088180147094,-36.8884573580224));
#33980=CARTESIAN_POINT('Ctrl Pts',(1.8111128882931,-1.43672381918429,-37.9153989559922));
#33981=CARTESIAN_POINT('Ctrl Pts',(1.84323794506374,-0.739869809114935,
-39.7767029410827));
#33982=CARTESIAN_POINT('Ctrl Pts',(1.86947535510397,-0.254607037277298,
-41.1128294039107));
#33983=CARTESIAN_POINT('Ctrl Pts',(1.87899508576981,-0.120158475357969,
-41.9361875204854));
#33984=CARTESIAN_POINT('Ctrl Pts',(1.88089764189098,-0.0904014568632321,
-42.1412540027529));
#33985=CARTESIAN_POINT('Ctrl Pts',(1.88326412278239,-0.057233445228627,
-42.4473182514808));
#33986=CARTESIAN_POINT('Ctrl Pts',(1.88516231205803,-0.032387317552159,
-42.7656567863243));
#33987=CARTESIAN_POINT('Ctrl Pts',(1.88713894608345,-0.0103148900108803,
-43.2000120944421));
#33988=CARTESIAN_POINT('Ctrl Pts',(1.88867239674863,-0.000330444911487711,
-43.7661869076419));
#33989=CARTESIAN_POINT('Ctrl Pts',(1.88943137570746,-0.00773447396790047,
-44.4806273744286));
#33990=CARTESIAN_POINT('Ctrl Pts',(1.88952521953819,-0.0208897500709426,
-45.1051458260789));
#33991=CARTESIAN_POINT('Ctrl Pts',(1.88943909368804,-0.0292027843404737,
-45.6220800031513));
#33992=CARTESIAN_POINT('Ctrl Pts',(1.88937202606144,-0.0325689471320249,
-46.0182813039979));
#33993=CARTESIAN_POINT('Ctrl Pts',(1.88935229353195,-0.0312056430228143,
-46.4230162698549));
#33994=CARTESIAN_POINT('Ctrl Pts',(1.88944668290529,-0.0204177420640209,
-46.9738736665184));
#33995=CARTESIAN_POINT('Ctrl Pts',(1.88977797873393,0.000877657567567272,
-47.3996979493288));
#33996=CARTESIAN_POINT('Ctrl Pts',(1.89033911609484,0.0354747851842442,
-47.8333811257174));
#33997=CARTESIAN_POINT('Ctrl Pts',(1.89071470667213,0.0548501897799582,
-48.0753819531635));
#33998=CARTESIAN_POINT('Ctrl Pts',(1.89146761287879,0.0968621047481274,
-48.5899412044517));
#33999=CARTESIAN_POINT('Ctrl Pts',(1.89277126953455,0.173459077297203,-49.4834146851367));
#34000=CARTESIAN_POINT('Ctrl Pts',(1.89449745127194,0.304140752206121,-50.7882896551614));
#34001=CARTESIAN_POINT('Ctrl Pts',(1.89579350141421,0.522243515316254,-52.3802470077318));
#34002=CARTESIAN_POINT('Ctrl Pts',(1.89593212526715,0.729188120289724,-53.461300559368));
#34003=CARTESIAN_POINT('Ctrl Pts',(1.89567407999173,0.884486289122258,-54.1427309942361));
#34004=CARTESIAN_POINT('Ctrl Pts',(1.8955253537994,0.947765356447221,-54.4117640933295));
#34005=CARTESIAN_POINT('Ctrl Pts',(1.89506593219007,1.0824539958618,-54.9518980607266));
#34006=CARTESIAN_POINT('Ctrl Pts',(1.8939009228576,1.33638837878062,-55.8919177460886));
#34007=CARTESIAN_POINT('Ctrl Pts',(1.89049136136924,1.91330971648247,-57.7581672374045));
#34008=CARTESIAN_POINT('Ctrl Pts',(1.88706535826581,2.50588183666261,-59.3238564112775));
#34009=CARTESIAN_POINT('Ctrl Pts',(1.88561817574945,2.95613587497698,-60.4151086469192));
#34010=CARTESIAN_POINT('Ctrl Pts',(1.88543527559833,3.01480092392394,-60.5555376788414));
#34011=CARTESIAN_POINT('Ctrl Pts',(1.88507824362982,3.13248322009135,-60.830502284115));
#34012=CARTESIAN_POINT('Ctrl Pts',(1.8844607487485,3.34489889769905,-61.310665724608));
#34013=CARTESIAN_POINT('Ctrl Pts',(1.88328108508382,3.78803882885241,-62.2560020211235));
#34014=CARTESIAN_POINT('Ctrl Pts',(1.88206459657106,4.32509239194982,-63.3081532507657));
#34015=CARTESIAN_POINT('Ctrl Pts',(1.88103553773681,4.86638112300206,-64.3295185491561));
#34016=CARTESIAN_POINT('Ctrl Pts',(1.88053102808851,5.1678768730388,-64.8921339858536));
#34017=CARTESIAN_POINT('Ctrl Pts',(1.88022675171844,5.3656359116224,-65.2618402500252));
#34018=CARTESIAN_POINT('Ctrl Pts',(1.88003357553327,5.49648391025698,-65.5068478162644));
#34019=CARTESIAN_POINT('Ctrl Pts',(1.87985097591106,5.62567062746725,-65.7496599480654));
#34020=CARTESIAN_POINT('Ctrl Pts',(1.87970493381329,5.73688874252341,-65.9600579521806));
#34021=CARTESIAN_POINT('Ctrl Pts',(1.87962492948782,5.79987484390888,-66.079684794079));
#34022=CARTESIAN_POINT('Ctrl Pts',(1.87950863690349,5.89376947121256,-66.2585300435357));
#34023=CARTESIAN_POINT('Ctrl Pts',(1.87941758530446,5.97072330512786,-66.4062684787644));
#34024=CARTESIAN_POINT('Ctrl Pts',(1.87927867663299,6.09633110207486,-66.64939961239));
#34025=CARTESIAN_POINT('Ctrl Pts',(1.87915208151063,6.23397919347889,-66.9149080623945));
#34026=CARTESIAN_POINT('Ctrl Pts',(1.87896352134001,6.50413138058693,-67.4326071669248));
#34027=CARTESIAN_POINT('Ctrl Pts',(1.87877816093101,6.97757667318536,-68.3320150970721));
#34028=CARTESIAN_POINT('Ctrl Pts',(1.8788680390831,7.91634487377019,-70.0909875251694));
#34029=CARTESIAN_POINT('Ctrl Pts',(1.87924656738061,8.71295995044206,-71.567154267523));
#34030=CARTESIAN_POINT('Ctrl Pts',(1.87923337319213,9.30797784656764,-72.6862215632396));
#34031=CARTESIAN_POINT('Ctrl Pts',(1.87923193113062,9.44178242559873,-72.9378697596276));
#34032=CARTESIAN_POINT('Ctrl Pts',(1.87922940657654,9.70858682183065,-73.4396541033119));
#34033=CARTESIAN_POINT('Ctrl Pts',(1.87922645837445,10.0422299603181,-74.0671465227276));
#34034=CARTESIAN_POINT('Ctrl Pts',(1.87922558503116,10.4422120792725,-74.8194044878806));
#34035=CARTESIAN_POINT('Ctrl Pts',(1.87922606073315,11.2419738247468,-76.3235419027106));
#34036=CARTESIAN_POINT('Ctrl Pts',(1.87922464770105,11.9081581569989,-77.5764660419606));
#34037=CARTESIAN_POINT('Ctrl Pts',(1.87922138294482,12.8780733791962,-79.4006165956265));
#34038=CARTESIAN_POINT('Ctrl Pts',(1.8792197023166,13.3146376913136,-80.2216773930927));
#34039=CARTESIAN_POINT('Ctrl Pts',(1.87921970231659,13.7511592787031,-81.042655095191));
#34040=CARTESIAN_POINT('Ctrl Pts',(4.38494444132642,-0.000133734827608889,
24.8306349039861));
#34041=CARTESIAN_POINT('Ctrl Pts',(4.38495753146493,-0.00013374032887973,
24.7817555964521));
#34042=CARTESIAN_POINT('Ctrl Pts',(4.38497125731604,-0.000133744552648744,
24.7328775966515));
#34043=CARTESIAN_POINT('Ctrl Pts',(4.38513347473583,-0.000133864397380097,
24.1822610347766));
#34044=CARTESIAN_POINT('Ctrl Pts',(4.3852582468995,-0.000134433697096954,
23.1780545188473));
#34045=CARTESIAN_POINT('Ctrl Pts',(4.38554667014594,-0.000134855584066727,
21.1694482846898));
#34046=CARTESIAN_POINT('Ctrl Pts',(4.38662762097494,-0.000136376740863039,
19.6651183959319));
#34047=CARTESIAN_POINT('Ctrl Pts',(4.38891822538359,-0.000137371987590711,
18.41399250541));
#34048=CARTESIAN_POINT('Ctrl Pts',(4.3900163968666,-0.000137730298437801,
17.9111645886437));
#34049=CARTESIAN_POINT('Ctrl Pts',(4.39277406888475,-0.000138809563126842,
16.907124878646));
#34050=CARTESIAN_POINT('Ctrl Pts',(4.3986885227367,-0.000140770907664884,
15.1532609539057));
#34051=CARTESIAN_POINT('Ctrl Pts',(4.40431300958534,-0.000144270691794568,
13.651109619525));
#34052=CARTESIAN_POINT('Ctrl Pts',(4.4078411305582,-0.00014522718386964,
12.39644086798));
#34053=CARTESIAN_POINT('Ctrl Pts',(4.4092832051397,-0.000145137964999622,
11.8954314878313));
#34054=CARTESIAN_POINT('Ctrl Pts',(4.41222508668909,-0.000145387654091127,
10.8935279540275));
#34055=CARTESIAN_POINT('Ctrl Pts',(4.41731809368509,-0.000143543800937141,
9.13954994961948));
#34056=CARTESIAN_POINT('Ctrl Pts',(4.42090548426581,-0.000150527145067114,
7.63410559711367));
#34057=CARTESIAN_POINT('Ctrl Pts',(4.42249863000223,-0.000147353245287479,
6.50044700529247));
#34058=CARTESIAN_POINT('Ctrl Pts',(4.42299616630408,0.00248284197451034,
6.21934256026946));
#34059=CARTESIAN_POINT('Ctrl Pts',(4.42445914823768,0.0160554202489226,
5.6847549980432));
#34060=CARTESIAN_POINT('Ctrl Pts',(4.42790007773388,0.0554580633367147,
4.76457601399349));
#34061=CARTESIAN_POINT('Ctrl Pts',(4.43584107924143,0.155572358940781,3.0286903083529));
#34062=CARTESIAN_POINT('Ctrl Pts',(4.43543312462318,0.146415497950293,1.71703744849467));
#34063=CARTESIAN_POINT('Ctrl Pts',(4.4235845204549,0.0168898128865376,0.876374772474017));
#34064=CARTESIAN_POINT('Ctrl Pts',(4.42204892079727,0.00214081928892977,
0.78860210460576));
#34065=CARTESIAN_POINT('Ctrl Pts',(4.4185311781697,-0.0343048651997382,
0.60032047710926));
#34066=CARTESIAN_POINT('Ctrl Pts',(4.41130252706129,-0.112371934479805,
0.261667363808621));
#34067=CARTESIAN_POINT('Ctrl Pts',(4.39851668321994,-0.265181268990898,
-0.260360024829797));
#34068=CARTESIAN_POINT('Ctrl Pts',(4.3805994085879,-0.503172644073552,-0.93691151551543));
#34069=CARTESIAN_POINT('Ctrl Pts',(4.35467542905104,-0.871862859368354,
-1.90182031569792));
#34070=CARTESIAN_POINT('Ctrl Pts',(4.32024185028443,-1.38292737347823,-3.21699911158908));
#34071=CARTESIAN_POINT('Ctrl Pts',(4.29559179121607,-1.72574738134475,-4.40684408194398));
#34072=CARTESIAN_POINT('Ctrl Pts',(4.28494920984687,-1.86685375632645,-5.20438075326181));
#34073=CARTESIAN_POINT('Ctrl Pts',(4.28149639120192,-1.91214565680086,-5.48564350309126));
#34074=CARTESIAN_POINT('Ctrl Pts',(4.27549161115425,-1.98936167253877,-6.06291218185832));
#34075=CARTESIAN_POINT('Ctrl Pts',(4.26796048132989,-2.08262140259452,-7.04610453435813));
#34076=CARTESIAN_POINT('Ctrl Pts',(4.26350476705694,-2.12952827711346,-8.40605252302899));
#34077=CARTESIAN_POINT('Ctrl Pts',(4.26290160138965,-2.12453036670742,-9.68968775091903));
#34078=CARTESIAN_POINT('Ctrl Pts',(4.26233004431676,-2.1235993642786,-10.5496387643383));
#34079=CARTESIAN_POINT('Ctrl Pts',(4.26172062194488,-2.12731348831879,-11.0291331838308));
#34080=CARTESIAN_POINT('Ctrl Pts',(4.26127901825024,-2.13119193174928,-11.2648521645087));
#34081=CARTESIAN_POINT('Ctrl Pts',(4.26088060468755,-2.1350823139462,-11.4412807325406));
#34082=CARTESIAN_POINT('Ctrl Pts',(4.26059750053618,-2.13783715675781,-11.5742931051035));
#34083=CARTESIAN_POINT('Ctrl Pts',(4.26009539343274,-2.14247157126928,-11.8315148074345));
#34084=CARTESIAN_POINT('Ctrl Pts',(4.25933127536179,-2.1489410967831,-12.2841524738275));
#34085=CARTESIAN_POINT('Ctrl Pts',(4.25794700299552,-2.15752446875554,-13.4367348500518));
#34086=CARTESIAN_POINT('Ctrl Pts',(4.25774924560805,-2.14923093736645,-14.6990441605346));
#34087=CARTESIAN_POINT('Ctrl Pts',(4.257898891459,-2.13944675254938,-15.9487908781029));
#34088=CARTESIAN_POINT('Ctrl Pts',(4.25798947493779,-2.1354625341751,-16.5717918598142));
#34089=CARTESIAN_POINT('Ctrl Pts',(4.25802180761526,-2.13361607940448,-17.069305966523));
#34090=CARTESIAN_POINT('Ctrl Pts',(4.25801831252641,-2.13326166550583,-17.3178788519545));
#34091=CARTESIAN_POINT('Ctrl Pts',(4.25800523628165,-2.13325861396676,-17.5035575132461));
#34092=CARTESIAN_POINT('Ctrl Pts',(4.25800303403809,-2.13325625333121,-17.6287430664321));
#34093=CARTESIAN_POINT('Ctrl Pts',(4.25802247592092,-2.1332510321176,-17.877785314546));
#34094=CARTESIAN_POINT('Ctrl Pts',(4.25807533223794,-2.13324369231377,-18.1274759620926));
#34095=CARTESIAN_POINT('Ctrl Pts',(4.25815578201396,-2.13323742070418,-18.3770116479716));
#34096=CARTESIAN_POINT('Ctrl Pts',(4.25821655397436,-2.13323347698379,-18.5330869888321));
#34097=CARTESIAN_POINT('Ctrl Pts',(4.2582707462992,-2.13323068283773,-18.6579557153899));
#34098=CARTESIAN_POINT('Ctrl Pts',(4.25832845323534,-2.13322798751371,-18.7828528356388));
#34099=CARTESIAN_POINT('Ctrl Pts',(4.25850066708906,-2.13322198399732,-19.1264052228547));
#34100=CARTESIAN_POINT('Ctrl Pts',(4.25884627993172,-2.13321684857528,-19.6890852084046));
#34101=CARTESIAN_POINT('Ctrl Pts',(4.25952647816828,-2.13325378494267,-20.6908951968342));
#34102=CARTESIAN_POINT('Ctrl Pts',(4.2602843313177,-2.13339493823762,-21.9461580058192));
#34103=CARTESIAN_POINT('Ctrl Pts',(4.26033098793204,-2.13372045578471,-22.9538712271591));
#34104=CARTESIAN_POINT('Ctrl Pts',(4.26004237114559,-2.133993612134,-23.5831634906123));
#34105=CARTESIAN_POINT('Ctrl Pts',(4.25989601774496,-2.13411302553283,-23.8322171555192));
#34106=CARTESIAN_POINT('Ctrl Pts',(4.2594892722799,-2.13440115952288,-24.3311913273362));
#34107=CARTESIAN_POINT('Ctrl Pts',(4.2585180312423,-2.13500677200017,-25.2062722948472));
#34108=CARTESIAN_POINT('Ctrl Pts',(4.25661156107835,-2.13611445719196,-26.4608432571924));
#34109=CARTESIAN_POINT('Ctrl Pts',(4.25421514420097,-2.13743125211775,-27.9689958353944));
#34110=CARTESIAN_POINT('Ctrl Pts',(4.25301855845424,-2.13818538230176,-28.9746783685956));
#34111=CARTESIAN_POINT('Ctrl Pts',(4.252594337193,-2.13848119146963,-29.5380129894862));
#34112=CARTESIAN_POINT('Ctrl Pts',(4.25246494386027,-2.13909508958004,-29.6465829713314));
#34113=CARTESIAN_POINT('Ctrl Pts',(4.25207003987882,-2.14239521561274,-29.8760648068341));
#34114=CARTESIAN_POINT('Ctrl Pts',(4.25104839864593,-2.15319445238582,-30.2796942725863));
#34115=CARTESIAN_POINT('Ctrl Pts',(4.24794966511473,-2.19091521088286,-31.1181176652429));
#34116=CARTESIAN_POINT('Ctrl Pts',(4.24321206419763,-2.25241329623747,-32.135797088019));
#34117=CARTESIAN_POINT('Ctrl Pts',(4.24060853356921,-2.28545836031402,-33.2148794748876));
#34118=CARTESIAN_POINT('Ctrl Pts',(4.24082448438597,-2.28175122961546,-34.0540552676246));
#34119=CARTESIAN_POINT('Ctrl Pts',(4.24437157033838,-2.23460163035187,-34.9233354941886));
#34120=CARTESIAN_POINT('Ctrl Pts',(4.24977549528951,-2.16323890794728,-35.5209805461277));
#34121=CARTESIAN_POINT('Ctrl Pts',(4.25525670096684,-2.09011394025412,-35.9770689509718));
#34122=CARTESIAN_POINT('Ctrl Pts',(4.26000233546485,-2.02758438872165,-36.3070700362323));
#34123=CARTESIAN_POINT('Ctrl Pts',(4.27103057364325,-1.87705461603904,-36.9270605674051));
#34124=CARTESIAN_POINT('Ctrl Pts',(4.29385848486922,-1.55664513660238,-37.9636207856555));
#34125=CARTESIAN_POINT('Ctrl Pts',(4.34311304510202,-0.800125491514468,
-39.8308322541445));
#34126=CARTESIAN_POINT('Ctrl Pts',(4.38119483574206,-0.278451825361257,
-41.1616575831691));
#34127=CARTESIAN_POINT('Ctrl Pts',(4.39548516377524,-0.136693188783896,
-41.9619869949894));
#34128=CARTESIAN_POINT('Ctrl Pts',(4.39842520476576,-0.104631661251257,
-42.1646065536608));
#34129=CARTESIAN_POINT('Ctrl Pts',(4.40208173363288,-0.0688288777778128,
-42.4659900876119));
#34130=CARTESIAN_POINT('Ctrl Pts',(4.40504729703054,-0.0416183495331478,
-42.7804374760604));
#34131=CARTESIAN_POINT('Ctrl Pts',(4.4081429290184,-0.0170206407560294,
-43.2099117875883));
#34132=CARTESIAN_POINT('Ctrl Pts',(4.41057027474141,-0.00485691508605945,
-43.77123943215));
#34133=CARTESIAN_POINT('Ctrl Pts',(4.4117742870394,-0.0110935056786064,
-44.4817888698965));
#34134=CARTESIAN_POINT('Ctrl Pts',(4.41188659105624,-0.024134170747513,
-45.1047465724255));
#34135=CARTESIAN_POINT('Ctrl Pts',(4.41175636241589,-0.0325221901227191,
-45.6214015911291));
#34136=CARTESIAN_POINT('Ctrl Pts',(4.41163173721691,-0.0359483457055346,
-46.0178897568402));
#34137=CARTESIAN_POINT('Ctrl Pts',(4.41156042456205,-0.0345379690853276,
-46.4234084111503));
#34138=CARTESIAN_POINT('Ctrl Pts',(4.41164198332398,-0.0233685406918769,
-46.975965217637));
#34139=CARTESIAN_POINT('Ctrl Pts',(4.41202937942913,-0.00125959827215216,
-47.4038163878187));
#34140=CARTESIAN_POINT('Ctrl Pts',(4.41278495644332,0.0348396358383206,
-47.8399267824656));
#34141=CARTESIAN_POINT('Ctrl Pts',(4.4132838759114,0.0549196106208449,-48.0815831819142));
#34142=CARTESIAN_POINT('Ctrl Pts',(4.41425913138979,0.0985496371173923,
-48.5964805029828));
#34143=CARTESIAN_POINT('Ctrl Pts',(4.41587201080464,0.177932520964587,-49.4897871839858));
#34144=CARTESIAN_POINT('Ctrl Pts',(4.41774428372684,0.312552417560597,-50.7942048465594));
#34145=CARTESIAN_POINT('Ctrl Pts',(4.41871611176856,0.534548942698696,-52.3845058858798));
#34146=CARTESIAN_POINT('Ctrl Pts',(4.41811880571771,0.742912336433342,-53.4639470870333));
#34147=CARTESIAN_POINT('Ctrl Pts',(4.41723188071979,0.898550865422039,-54.1442117798183));
#34148=CARTESIAN_POINT('Ctrl Pts',(4.41680184496303,0.961905712297198,-54.41276250448));
#34149=CARTESIAN_POINT('Ctrl Pts',(4.4156507935149,1.09657035164313,-54.9520528656041));
#34150=CARTESIAN_POINT('Ctrl Pts',(4.41298531917194,1.35002999176865,-55.8908387686135));
#34151=CARTESIAN_POINT('Ctrl Pts',(4.40577743472443,1.92474191344074,-57.755588741959));
#34152=CARTESIAN_POINT('Ctrl Pts',(4.39894561258167,2.51469589787006,-59.3214284512625));
#34153=CARTESIAN_POINT('Ctrl Pts',(4.39608239703651,2.96398234750693,-60.4133254990442));
#34154=CARTESIAN_POINT('Ctrl Pts',(4.39572420020829,3.02243441040618,-60.5536403951176));
#34155=CARTESIAN_POINT('Ctrl Pts',(4.39503159740573,3.13972743028378,-60.8285020826318));
#34156=CARTESIAN_POINT('Ctrl Pts',(4.39385789835129,3.35140393735138,-61.3084658780271));
#34157=CARTESIAN_POINT('Ctrl Pts',(4.39168537592052,3.79298878201076,-62.2535803239954));
#34158=CARTESIAN_POINT('Ctrl Pts',(4.38959734540799,4.3281999379598,-63.3057043206065));
#34159=CARTESIAN_POINT('Ctrl Pts',(4.38788098922377,4.86787702280524,-64.3272637172959));
#34160=CARTESIAN_POINT('Ctrl Pts',(4.38704573394525,5.16860177178643,-64.8900676807838));
#34161=CARTESIAN_POINT('Ctrl Pts',(4.38654071275671,5.36592715697807,-65.2599366680509));
#34162=CARTESIAN_POINT('Ctrl Pts',(4.38621762817815,5.49650820835829,-65.5050630813914));
#34163=CARTESIAN_POINT('Ctrl Pts',(4.38591471255685,5.62546575748379,-65.7480091109017));
#34164=CARTESIAN_POINT('Ctrl Pts',(4.38566703852788,5.73651809548135,-65.9585397229399));
#34165=CARTESIAN_POINT('Ctrl Pts',(4.38553044241807,5.79942023400714,-66.0782468295102));
#34166=CARTESIAN_POINT('Ctrl Pts',(4.38533047147116,5.89319979678333,-66.2572170941181));
#34167=CARTESIAN_POINT('Ctrl Pts',(4.38517400334211,5.97008206126848,-66.4050691863734));
#34168=CARTESIAN_POINT('Ctrl Pts',(4.38492849824558,6.09560395288787,-66.6484025458349));
#34169=CARTESIAN_POINT('Ctrl Pts',(4.38470615525269,6.23315175334774,-66.9140716153702));
#34170=CARTESIAN_POINT('Ctrl Pts',(4.38437396671341,6.50319749318971,-67.4320845675039));
#34171=CARTESIAN_POINT('Ctrl Pts',(4.38405715027776,6.97662108137445,-68.331945776566));
#34172=CARTESIAN_POINT('Ctrl Pts',(4.38423359111322,7.91583209385217,-70.0914928447299));
#34173=CARTESIAN_POINT('Ctrl Pts',(4.38494215631249,8.71294426216148,-71.5675208905616));
#34174=CARTESIAN_POINT('Ctrl Pts',(4.38493000258167,9.30774093474432,-72.6861891777452));
#34175=CARTESIAN_POINT('Ctrl Pts',(4.38492777760085,9.44155851431508,-72.9378663168809));
#34176=CARTESIAN_POINT('Ctrl Pts',(4.38492441286894,9.70835430006309,-73.4396407360582));
#34177=CARTESIAN_POINT('Ctrl Pts',(4.38492215877831,10.0420032022086,-74.0671467503144));
#34178=CARTESIAN_POINT('Ctrl Pts',(4.38492189125759,10.4419859347932,-74.8194055694887));
#34179=CARTESIAN_POINT('Ctrl Pts',(4.38492474424574,11.2417558570399,-76.3235510600817));
#34180=CARTESIAN_POINT('Ctrl Pts',(4.38493101488265,11.9079483102949,-77.5764715046922));
#34181=CARTESIAN_POINT('Ctrl Pts',(4.38493092127123,12.8778611632279,-79.4006140082112));
#34182=CARTESIAN_POINT('Ctrl Pts',(4.38493087314377,13.3144278324901,-80.2216773891645));
#34183=CARTESIAN_POINT('Ctrl Pts',(4.38493087314375,13.7509494198795,-81.0426550912629));
#34184=CARTESIAN_POINT('Ctrl Pts',(6.89104910298435,-0.00024498498954306,
24.8306350459706));
#34185=CARTESIAN_POINT('Ctrl Pts',(6.89106969042788,-0.000244992005475219,
24.7817557429577));
#34186=CARTESIAN_POINT('Ctrl Pts',(6.89109126507086,-0.000244999363845071,
24.7328777610462));
#34187=CARTESIAN_POINT('Ctrl Pts',(6.8913468151815,-0.000245085668324933,
24.1822608050565));
#34188=CARTESIAN_POINT('Ctrl Pts',(6.89154686940115,-0.000245309193916475,
23.1780506245846));
#34189=CARTESIAN_POINT('Ctrl Pts',(6.89200170238563,-0.000245943228249708,
21.1694440815797));
#34190=CARTESIAN_POINT('Ctrl Pts',(6.89371055321136,-0.000246501152717097,
19.6651049165689));
#34191=CARTESIAN_POINT('Ctrl Pts',(6.89731549185056,-0.000246902951521312,
18.4139749758576));
#34192=CARTESIAN_POINT('Ctrl Pts',(6.89904265364457,-0.000247155807051646,
17.9111466962113));
#34193=CARTESIAN_POINT('Ctrl Pts',(6.90338100601535,-0.000247888007577191,
16.9071045316924));
#34194=CARTESIAN_POINT('Ctrl Pts',(6.91268284218105,-0.000249412304973884,
15.1532378243496));
#34195=CARTESIAN_POINT('Ctrl Pts',(6.92154441509678,-0.000249921414807475,
13.6510643636072));
#34196=CARTESIAN_POINT('Ctrl Pts',(6.92709720790588,-0.000248609121187243,
12.3963845191955));
#34197=CARTESIAN_POINT('Ctrl Pts',(6.92936390855178,-0.000247823935322427,
11.8953717842346));
#34198=CARTESIAN_POINT('Ctrl Pts',(6.93399085127207,-0.000245912721741659,
10.8934648715124));
#34199=CARTESIAN_POINT('Ctrl Pts',(6.941993501733,-0.000240364403368093,
9.13946216763256));
#34200=CARTESIAN_POINT('Ctrl Pts',(6.94768031383367,-0.000237808466911361,
7.6340098511879));
#34201=CARTESIAN_POINT('Ctrl Pts',(6.95020094821363,-0.000230555480565149,
6.50020032101587));
#34202=CARTESIAN_POINT('Ctrl Pts',(6.95063684985277,0.00256165266826663,
6.21737010967138));
#34203=CARTESIAN_POINT('Ctrl Pts',(6.95110846856475,0.0169490906205031,
5.68090711620389));
#34204=CARTESIAN_POINT('Ctrl Pts',(6.95109368914234,0.0586645200695752,
4.75843655621655));
#34205=CARTESIAN_POINT('Ctrl Pts',(6.94892115892448,0.16424761237392,3.02377943901819));
#34206=CARTESIAN_POINT('Ctrl Pts',(6.94863380234148,0.154198492166273,1.72337900750542));
#34207=CARTESIAN_POINT('Ctrl Pts',(6.95342525135404,0.0192222826723204,
0.894091270258636));
#34208=CARTESIAN_POINT('Ctrl Pts',(6.95402987640926,0.00398319776505293,
0.808286238370748));
#34209=CARTESIAN_POINT('Ctrl Pts',(6.95541606875165,-0.0338837478143756,
0.623174343735704));
#34210=CARTESIAN_POINT('Ctrl Pts',(6.95824164768107,-0.115240968906443,
0.289354562987173));
#34211=CARTESIAN_POINT('Ctrl Pts',(6.96327163986587,-0.275499286305752,
-0.22816704014749));
#34212=CARTESIAN_POINT('Ctrl Pts',(6.97013009679123,-0.526548360153427,
-0.901612116200544));
#34213=CARTESIAN_POINT('Ctrl Pts',(6.98007564991511,-0.917055970967649,
-1.8645931081793));
#34214=CARTESIAN_POINT('Ctrl Pts',(6.9928688616949,-1.46101102771583,-3.18020351604593));
#34215=CARTESIAN_POINT('Ctrl Pts',(7.00181798897999,-1.8298425877256,-4.37745688997694));
#34216=CARTESIAN_POINT('Ctrl Pts',(7.00534376182817,-1.98247267596028,-5.1844399667158));
#34217=CARTESIAN_POINT('Ctrl Pts',(7.00641136561573,-2.0311953057056,-5.46739474082408));
#34218=CARTESIAN_POINT('Ctrl Pts',(7.00811865174563,-2.11444031578616,-6.04904983182828));
#34219=CARTESIAN_POINT('Ctrl Pts',(7.0097862660601,-2.21489225562981,-7.03866839639272));
#34220=CARTESIAN_POINT('Ctrl Pts',(7.00935572239978,-2.26528901955801,-8.4053192817156));
#34221=CARTESIAN_POINT('Ctrl Pts',(7.00725330740455,-2.25981898315895,-9.6908323666209));
#34222=CARTESIAN_POINT('Ctrl Pts',(7.00589690781737,-2.25878825103757,-10.5497523725835));
#34223=CARTESIAN_POINT('Ctrl Pts',(7.00529225341263,-2.26273389699714,-11.0279436565139));
#34224=CARTESIAN_POINT('Ctrl Pts',(7.00506881584601,-2.26686517166806,-11.2627708989377));
#34225=CARTESIAN_POINT('Ctrl Pts',(7.00493595031213,-2.27100964632756,-11.4384651606442));
#34226=CARTESIAN_POINT('Ctrl Pts',(7.00484836839363,-2.2739661211869,-11.5719308075916));
#34227=CARTESIAN_POINT('Ctrl Pts',(7.00463561274481,-2.27892706711406,-11.8295019931928));
#34228=CARTESIAN_POINT('Ctrl Pts',(7.00419443918313,-2.28585201946081,-12.2829590322349));
#34229=CARTESIAN_POINT('Ctrl Pts',(7.00275050857491,-2.29500391100284,-13.4371000127244));
#34230=CARTESIAN_POINT('Ctrl Pts',(7.00059379503007,-2.28604358714452,-14.7003011504045));
#34231=CARTESIAN_POINT('Ctrl Pts',(6.99890853765602,-2.275516690094,-15.949893638767));
#34232=CARTESIAN_POINT('Ctrl Pts',(6.99830005957763,-2.27123437456408,-16.5725928132207));
#34233=CARTESIAN_POINT('Ctrl Pts',(6.99799068376282,-2.26925031404122,-17.0697162473411));
#34234=CARTESIAN_POINT('Ctrl Pts',(6.99790913550761,-2.26886914319229,-17.3180464092085));
#34235=CARTESIAN_POINT('Ctrl Pts',(6.99787713820796,-2.26886529890116,-17.5035309910445));
#34236=CARTESIAN_POINT('Ctrl Pts',(6.9978639032166,-2.26886101581699,-17.6287753544509));
#34237=CARTESIAN_POINT('Ctrl Pts',(6.99786698761888,-2.26884742862941,-17.8778210848774));
#34238=CARTESIAN_POINT('Ctrl Pts',(6.99791421698644,-2.26882538596002,-18.1275501541622));
#34239=CARTESIAN_POINT('Ctrl Pts',(6.99799850102396,-2.26880018709046,-18.3770960467612));
#34240=CARTESIAN_POINT('Ctrl Pts',(6.9980664450061,-2.26878287323182,-18.5331800437488));
#34241=CARTESIAN_POINT('Ctrl Pts',(6.99812909445171,-2.26876872466669,-18.6580522536357));
#34242=CARTESIAN_POINT('Ctrl Pts',(6.9981972425833,-2.26875429147753,-18.7829523317202));
#34243=CARTESIAN_POINT('Ctrl Pts',(6.99840638378703,-2.26871451756231,-19.1265081948758));
#34244=CARTESIAN_POINT('Ctrl Pts',(6.99886006536309,-2.26864996988756,-19.6891706427572));
#34245=CARTESIAN_POINT('Ctrl Pts',(6.9998822485617,-2.26860388774605,-20.6908816494304));
#34246=CARTESIAN_POINT('Ctrl Pts',(7.00139967900657,-2.26874994953288,-21.945896967966));
#34247=CARTESIAN_POINT('Ctrl Pts',(7.00247309280133,-2.26933126992684,-22.9532794742794));
#34248=CARTESIAN_POINT('Ctrl Pts',(7.0029887564633,-2.26988649050958,-23.5823240349596));
#34249=CARTESIAN_POINT('Ctrl Pts',(7.00319420804157,-2.27013392172621,-23.8312307536037));
#34250=CARTESIAN_POINT('Ctrl Pts',(7.00360398344485,-2.27073812005696,-24.3299781180718));
#34251=CARTESIAN_POINT('Ctrl Pts',(7.00432709632794,-2.27203490661507,-25.2047311211729));
#34252=CARTESIAN_POINT('Ctrl Pts',(7.0053274540055,-2.27441233558042,-26.4591008069716));
#34253=CARTESIAN_POINT('Ctrl Pts',(7.00653584994815,-2.27733928484868,-27.9673691521971));
#34254=CARTESIAN_POINT('Ctrl Pts',(7.00726581201525,-2.27895576084736,-28.9734445269011));
#34255=CARTESIAN_POINT('Ctrl Pts',(7.00768741812352,-2.27959993181941,-29.5369717835662));
#34256=CARTESIAN_POINT('Ctrl Pts',(7.00780073972456,-2.28031670425964,-29.6444420501042));
#34257=CARTESIAN_POINT('Ctrl Pts',(7.00809766792642,-2.28396009662537,-29.8725594838599));
#34258=CARTESIAN_POINT('Ctrl Pts',(7.00877793961808,-2.29569033419828,-30.2739083653757));
#34259=CARTESIAN_POINT('Ctrl Pts',(7.0106802705156,-2.33639039519754,-31.1097812419148));
#34260=CARTESIAN_POINT('Ctrl Pts',(7.01341229050687,-2.4028184112436,-32.1283655105824));
#34261=CARTESIAN_POINT('Ctrl Pts',(7.01520429698212,-2.43879053088795,-33.2125950918116));
#34262=CARTESIAN_POINT('Ctrl Pts',(7.01557655242834,-2.43498485314343,-34.057735891391));
#34263=CARTESIAN_POINT('Ctrl Pts',(7.01439623030718,-2.38406503985142,-34.9349685769412));
#34264=CARTESIAN_POINT('Ctrl Pts',(7.0122274136511,-2.30676299171889,-35.5388148177783));
#34265=CARTESIAN_POINT('Ctrl Pts',(7.00998652770148,-2.22756133212805,-35.9996792004172));
#34266=CARTESIAN_POINT('Ctrl Pts',(7.00803909756502,-2.15962539500237,-36.3341747691404));
#34267=CARTESIAN_POINT('Ctrl Pts',(7.00347015250425,-1.99681681609787,-36.9600450235213));
#34268=CARTESIAN_POINT('Ctrl Pts',(6.9937431091387,-1.65190985969706,-38.002830542361));
#34269=CARTESIAN_POINT('Ctrl Pts',(6.97235829764089,-0.844341899209787,
-39.8703584526267));
#34270=CARTESIAN_POINT('Ctrl Pts',(6.95472791598771,-0.294406849577237,
-41.1965525582491));
#34271=CARTESIAN_POINT('Ctrl Pts',(6.94817137872906,-0.147220927628577,
-41.9802784413025));
#34272=CARTESIAN_POINT('Ctrl Pts',(6.94688299772939,-0.113472013097866,
-42.1811165076733));
#34273=CARTESIAN_POINT('Ctrl Pts',(6.94530724703268,-0.0757730453484783,
-42.4791089023079));
#34274=CARTESIAN_POINT('Ctrl Pts',(6.94407239284371,-0.0468827358548862,
-42.7907295132023));
#34275=CARTESIAN_POINT('Ctrl Pts',(6.9428166037123,-0.0205159884065598,
-43.2166553393947));
#34276=CARTESIAN_POINT('Ctrl Pts',(6.94188917056371,-0.00686498021950975,
-43.7744463599481));
#34277=CARTESIAN_POINT('Ctrl Pts',(6.94143803507245,-0.0123781368730491,
-44.4821346690289));
#34278=CARTESIAN_POINT('Ctrl Pts',(6.9412937478431,-0.0254512748617087,
-45.1039146783508));
#34279=CARTESIAN_POINT('Ctrl Pts',(6.9411669417653,-0.0340160506748517,
-45.6203215595853));
#34280=CARTESIAN_POINT('Ctrl Pts',(6.94100001408149,-0.0375857210191279,
-46.0169793624786));
#34281=CARTESIAN_POINT('Ctrl Pts',(6.94071683255022,-0.0362515468378396,
-46.4230240405838));
#34282=CARTESIAN_POINT('Ctrl Pts',(6.94012770127554,-0.0249707453746474,
-46.9767511611614));
#34283=CARTESIAN_POINT('Ctrl Pts',(6.93935359805737,-0.00240539020963474,
-47.4060205652198));
#34284=CARTESIAN_POINT('Ctrl Pts',(6.93828715749912,0.0346278594182365,
-47.843830926901));
#34285=CARTESIAN_POINT('Ctrl Pts',(6.93753780765541,0.0551177747709163,
-48.0851115474941));
#34286=CARTESIAN_POINT('Ctrl Pts',(6.9359028464867,0.0996744565208953,-48.6000854844173));
#34287=CARTESIAN_POINT('Ctrl Pts',(6.93271869400548,0.180558930246471,-49.4930326775486));
#34288=CARTESIAN_POINT('Ctrl Pts',(6.92746024155021,0.317107244885934,-50.7970279095856));
#34289=CARTESIAN_POINT('Ctrl Pts',(6.92077978587043,0.540751777371533,-52.3864353473554));
#34290=CARTESIAN_POINT('Ctrl Pts',(6.91657371441663,0.749687557481511,-53.4652019487692));
#34291=CARTESIAN_POINT('Ctrl Pts',(6.91418410317824,0.905493783202333,-54.1449974000241));
#34292=CARTESIAN_POINT('Ctrl Pts',(6.9131924896337,0.968874942190495,-54.4132984129917));
#34293=CARTESIAN_POINT('Ctrl Pts',(6.91113670604855,1.10352176270923,-54.9521794482773));
#34294=CARTESIAN_POINT('Ctrl Pts',(6.90738506736453,1.35675544402263,-55.8903497025829));
#34295=CARTESIAN_POINT('Ctrl Pts',(6.89968460661885,1.93045977921322,-57.7543508921274));
#34296=CARTESIAN_POINT('Ctrl Pts',(6.89408348717811,2.5191883577489,-59.3202380645919));
#34297=CARTESIAN_POINT('Ctrl Pts',(6.89195135839285,2.96800306623196,-60.4124402356466));
#34298=CARTESIAN_POINT('Ctrl Pts',(6.89171429919799,3.0263514212361,-60.5526931378033));
#34299=CARTESIAN_POINT('Ctrl Pts',(6.89128991775844,3.1434538716825,-60.8274949565257));
#34300=CARTESIAN_POINT('Ctrl Pts',(6.89068359683782,3.35476527656681,-61.3073433604132));
#34301=CARTESIAN_POINT('Ctrl Pts',(6.88995074751437,3.79557181295857,-62.252317471277));
#34302=CARTESIAN_POINT('Ctrl Pts',(6.88995917391789,4.32983562181616,-63.3044054893138));
#34303=CARTESIAN_POINT('Ctrl Pts',(6.89032196427239,4.86867416564934,-64.3260586974247));
#34304=CARTESIAN_POINT('Ctrl Pts',(6.89056898535275,5.16899624846297,-64.888961970895));
#34305=CARTESIAN_POINT('Ctrl Pts',(6.89071316539118,5.3660945447526,-65.2589185090952));
#34306=CARTESIAN_POINT('Ctrl Pts',(6.89080140524194,5.49653604670366,-65.5041091394283));
#34307=CARTESIAN_POINT('Ctrl Pts',(6.89087358680562,5.62537294269141,-65.7471279716458));
#34308=CARTESIAN_POINT('Ctrl Pts',(6.89091630878653,5.73633849640408,-65.9577307770876));
#34309=CARTESIAN_POINT('Ctrl Pts',(6.89093386030419,5.79919670625669,-66.0774815963281));
#34310=CARTESIAN_POINT('Ctrl Pts',(6.89095285967377,5.89291617543268,-66.2565199375178));
#34311=CARTESIAN_POINT('Ctrl Pts',(6.89095225893861,5.96976082905929,-66.4044339259934));
#34312=CARTESIAN_POINT('Ctrl Pts',(6.89092434227999,6.0952381855696,-66.6478771407354));
#34313=CARTESIAN_POINT('Ctrl Pts',(6.89089907668696,6.23273250392706,-66.9136308044214));
#34314=CARTESIAN_POINT('Ctrl Pts',(6.89086260692432,6.50272160355848,-67.4318102360639));
#34315=CARTESIAN_POINT('Ctrl Pts',(6.89083129094997,6.97613109832236,-68.3319099789933));
#34316=CARTESIAN_POINT('Ctrl Pts',(6.8908723959093,7.91557235664225,-70.09175669196));
#34317=CARTESIAN_POINT('Ctrl Pts',(6.89097650851583,8.71294015020471,-71.5677124890261));
#34318=CARTESIAN_POINT('Ctrl Pts',(6.89098028167908,9.30761950729522,-72.6861721206043));
#34319=CARTESIAN_POINT('Ctrl Pts',(6.89098108645138,9.44144384808963,-72.9378643900992));
#34320=CARTESIAN_POINT('Ctrl Pts',(6.89098226445106,9.70823498149448,-73.4396336082364));
#34321=CARTESIAN_POINT('Ctrl Pts',(6.89098289537523,10.0418864481601,-74.06714673629));
#34322=CARTESIAN_POINT('Ctrl Pts',(6.89098290635027,10.4418692957198,-74.8194059925143));
#34323=CARTESIAN_POINT('Ctrl Pts',(6.89098170197776,11.2416431420624,-76.3235556962517));
#34324=CARTESIAN_POINT('Ctrl Pts',(6.89097877132087,11.9078384197489,-77.5764742851218));
#34325=CARTESIAN_POINT('Ctrl Pts',(6.89097842229583,12.8777491700385,-79.4006126633289));
#34326=CARTESIAN_POINT('Ctrl Pts',(6.89097824243373,13.3143166100287,-80.2216774058681));
#34327=CARTESIAN_POINT('Ctrl Pts',(6.89097824243374,13.7508381974181,-81.0426551079665));
#34328=CARTESIAN_POINT('Ctrl Pts',(9.39709574952983,9.85060074434863E-5,
24.8306346021324));
#34329=CARTESIAN_POINT('Ctrl Pts',(9.39712382476148,9.85139203122644E-5,
24.7817552849976));
#34330=CARTESIAN_POINT('Ctrl Pts',(9.39715326797429,9.85273671940927E-5,
24.7328772539229));
#34331=CARTESIAN_POINT('Ctrl Pts',(9.3975010314311,9.84518919665791E-5,
24.1822613028827));
#34332=CARTESIAN_POINT('Ctrl Pts',(9.39776786851327,9.71467296369741E-5,
23.1780607007944));
#34333=CARTESIAN_POINT('Ctrl Pts',(9.39838786334986,9.73630010883039E-5,
21.1694549086907));
#34334=CARTESIAN_POINT('Ctrl Pts',(9.40070301825327,9.44172580033674E-5,
19.6651399776767));
#34335=CARTESIAN_POINT('Ctrl Pts',(9.40561179634645,9.38961761531635E-5,
18.4140206008922));
#34336=CARTESIAN_POINT('Ctrl Pts',(9.40796582390437,9.41854221663634E-5,
17.9111930870781));
#34337=CARTESIAN_POINT('Ctrl Pts',(9.41387706883776,9.4553365822232E-5,
16.9071572294501));
#34338=CARTESIAN_POINT('Ctrl Pts',(9.42655591655234,9.64268787003325E-5,
15.1532978757182));
#34339=CARTESIAN_POINT('Ctrl Pts',(9.43860374245195,9.06259428207321E-5,
13.651182963467));
#34340=CARTESIAN_POINT('Ctrl Pts',(9.44615688123903,8.73069875527575E-5,
12.396532862185));
#34341=CARTESIAN_POINT('Ctrl Pts',(9.4492444542645,8.69671991073794E-5,
11.895529349549));
#34342=CARTESIAN_POINT('Ctrl Pts',(9.4555398926741,8.41326905260385E-5,
10.8936312703422));
#34343=CARTESIAN_POINT('Ctrl Pts',(9.46643626337659,8.15860255114301E-5,
9.13969528076933));
#34344=CARTESIAN_POINT('Ctrl Pts',(9.47408873909819,5.54737107715689E-5,
7.6342584301987));
#34345=CARTESIAN_POINT('Ctrl Pts',(9.47748675819484,5.05234838685672E-5,
6.50085628110018));
#34346=CARTESIAN_POINT('Ctrl Pts',(9.47774676872149,0.00240407033145399,
6.22271251698896));
#34347=CARTESIAN_POINT('Ctrl Pts',(9.47663442596991,0.0145821795353661,
5.69133854372974));
#34348=CARTESIAN_POINT('Ctrl Pts',(9.4713534496034,0.0500243802638127,4.77508614954621));
#34349=CARTESIAN_POINT('Ctrl Pts',(9.45435632175483,0.140714471638447,3.03710695773964));
#34350=CARTESIAN_POINT('Ctrl Pts',(9.45372533458491,0.133068046649489,1.70611532398695));
#34351=CARTESIAN_POINT('Ctrl Pts',(9.48257740876507,0.0130386069436019,
0.845828636693778));
#34352=CARTESIAN_POINT('Ctrl Pts',(9.48630876393063,-0.000847748246050882,
0.754632089069898));
#34353=CARTESIAN_POINT('Ctrl Pts',(9.49486024241688,-0.0348148210482442,
0.560836824164949));
#34354=CARTESIAN_POINT('Ctrl Pts',(9.51244192469342,-0.107173781897646,
0.213757548909062));
#34355=CARTESIAN_POINT('Ctrl Pts',(9.54365652214872,-0.247172970664451,
-0.316122472084849));
#34356=CARTESIAN_POINT('Ctrl Pts',(9.58741988734466,-0.462822748651149,
-0.997961801831015));
#34357=CARTESIAN_POINT('Ctrl Pts',(9.65058012985507,-0.794350751155283,
-1.96586121105861));
#34358=CARTESIAN_POINT('Ctrl Pts',(9.73329874184328,-1.24970822682561,-3.27944088196305));
#34359=CARTESIAN_POINT('Ctrl Pts',(9.78933424622287,-1.54945484288796,-4.4560485225065));
#34360=CARTESIAN_POINT('Ctrl Pts',(9.81231789269538,-1.67175810583986,-5.23755586899791));
#34361=CARTESIAN_POINT('Ctrl Pts',(9.81975763370998,-1.71146137288016,-5.51594462977292));
#34362=CARTESIAN_POINT('Ctrl Pts',(9.83219696761995,-1.77894269056047,-6.08582494629925));
#34363=CARTESIAN_POINT('Ctrl Pts',(9.84658949085487,-1.86080320713964,-7.05828794318947));
#34364=CARTESIAN_POINT('Ctrl Pts',(9.85146478888084,-1.90278098250614,-8.40712935793198));
#34365=CARTESIAN_POINT('Ctrl Pts',(9.84696453471149,-1.89943818623475,-9.68764951150679));
#34366=CARTESIAN_POINT('Ctrl Pts',(9.84450263709722,-1.89922786536826,-10.549318186832));
#34367=CARTESIAN_POINT('Ctrl Pts',(9.84396945193637,-1.9028474624947,-11.030981263349));
#34368=CARTESIAN_POINT('Ctrl Pts',(9.84411071223977,-1.90644026244215,-11.2681837624333));
#34369=CARTESIAN_POINT('Ctrl Pts',(9.84441122490759,-1.91000441977411,-11.4458336189714));
#34370=CARTESIAN_POINT('Ctrl Pts',(9.84463107530365,-1.91249319772449,-11.5780920335527));
#34371=CARTESIAN_POINT('Ctrl Pts',(9.84490733911212,-1.91672407923323,-11.8347330068637));
#34372=CARTESIAN_POINT('Ctrl Pts',(9.84507523283692,-1.92268918027574,-12.2860098066065));
#34373=CARTESIAN_POINT('Ctrl Pts',(9.84400431113743,-1.93100390233827,-13.4360093674867));
#34374=CARTESIAN_POINT('Ctrl Pts',(9.83969839554375,-1.92457337722949,-14.6968539115163));
#34375=CARTESIAN_POINT('Ctrl Pts',(9.8360140155241,-1.91654013277157,-15.9468962665494));
#34376=CARTESIAN_POINT('Ctrl Pts',(9.83462020824012,-1.9132362729513,-16.5704247665775));
#34377=CARTESIAN_POINT('Ctrl Pts',(9.83396171319717,-1.91170774015949,-17.0686125869906));
#34378=CARTESIAN_POINT('Ctrl Pts',(9.83381192550018,-1.91142187832722,-17.317602341319));
#34379=CARTESIAN_POINT('Ctrl Pts',(9.83377912208015,-1.91142942347021,-17.5036135228565));
#34380=CARTESIAN_POINT('Ctrl Pts',(9.8337683516608,-1.91143332817741,-17.6286923495811));
#34381=CARTESIAN_POINT('Ctrl Pts',(9.83378925148769,-1.91143666779512,-17.877722086886));
#34382=CARTESIAN_POINT('Ctrl Pts',(9.8338690691644,-1.91143235734373,-18.1273414666358));
#34383=CARTESIAN_POINT('Ctrl Pts',(9.8340050059961,-1.91142124231706,-18.3768574556843));
#34384=CARTESIAN_POINT('Ctrl Pts',(9.83411137207806,-1.91141112487478,-18.5329174549527));
#34385=CARTESIAN_POINT('Ctrl Pts',(9.8342089902123,-1.91140120730261,-18.6577804903151));
#34386=CARTESIAN_POINT('Ctrl Pts',(9.83431464188427,-1.91138991853604,-18.7826732285614));
#34387=CARTESIAN_POINT('Ctrl Pts',(9.83463598146339,-1.91135465577494,-19.1262231260297));
#34388=CARTESIAN_POINT('Ctrl Pts',(9.83532550903627,-1.91126593733576,-19.6889483271403));
#34389=CARTESIAN_POINT('Ctrl Pts',(9.83689315628327,-1.91103332471521,-20.6909798403928));
#34390=CARTESIAN_POINT('Ctrl Pts',(9.83928212534762,-1.91055958819307,-21.9467826019539));
#34391=CARTESIAN_POINT('Ctrl Pts',(9.84116764454534,-1.91001418058634,-22.955204818448));
#34392=CARTESIAN_POINT('Ctrl Pts',(9.8421933054474,-1.90959220114503,-23.5850311524326));
#34393=CARTESIAN_POINT('Ctrl Pts',(9.84261393218004,-1.9094071339158,-23.8344089360016));
#34394=CARTESIAN_POINT('Ctrl Pts',(9.84350382388819,-1.90898251807467,-24.3338811135346));
#34395=CARTESIAN_POINT('Ctrl Pts',(9.8451725829466,-1.90810399481636,-25.2096813987555));
#34396=CARTESIAN_POINT('Ctrl Pts',(9.84775195150598,-1.90661928666474,-26.4646920808429));
#34397=CARTESIAN_POINT('Ctrl Pts',(9.85082969349042,-1.90472362092078,-27.9725650153342));
#34398=CARTESIAN_POINT('Ctrl Pts',(9.85260536859806,-1.90372500288613,-28.9773843873838));
#34399=CARTESIAN_POINT('Ctrl Pts',(9.85347022616558,-1.90327567303515,-29.5402360386186));
#34400=CARTESIAN_POINT('Ctrl Pts',(9.85376439664258,-1.90368429194054,-29.6505702179668));
#34401=CARTESIAN_POINT('Ctrl Pts',(9.85472331033051,-1.90634343794854,-29.8822173878728));
#34402=CARTESIAN_POINT('Ctrl Pts',(9.85729641826308,-1.91547380118253,-30.2894705601969));
#34403=CARTESIAN_POINT('Ctrl Pts',(9.86529427154334,-1.94801673142762,-31.1318876565905));
#34404=CARTESIAN_POINT('Ctrl Pts',(9.87755736457791,-2.00113995963799,-32.1479794298922));
#34405=CARTESIAN_POINT('Ctrl Pts',(9.88458332930815,-2.02914796194555,-33.2187160361868));
#34406=CARTESIAN_POINT('Ctrl Pts',(9.8846505448229,-2.02540533054684,-34.0482843286969));
#34407=CARTESIAN_POINT('Ctrl Pts',(9.87678603945088,-1.98416420939679,-34.9047570982295));
#34408=CARTESIAN_POINT('Ctrl Pts',(9.86434714101142,-1.92228483706194,-35.4923457190805));
#34409=CARTESIAN_POINT('Ctrl Pts',(9.85161255446927,-1.85892275316106,-35.9406210300452));
#34410=CARTESIAN_POINT('Ctrl Pts',(9.84072169333682,-1.80507065302535,-36.2632421397352));
#34411=CARTESIAN_POINT('Ctrl Pts',(9.81484982650837,-1.67442270398369,-36.8733766663579));
#34412=CARTESIAN_POINT('Ctrl Pts',(9.7600581790089,-1.39404280255062,-37.8990108669212));
#34413=CARTESIAN_POINT('Ctrl Pts',(9.63659735888789,-0.722613497645318,
-39.7639201836366));
#34414=CARTESIAN_POINT('Ctrl Pts',(9.53816382801678,-0.248912727847852,
-41.1021642167714));
#34415=CARTESIAN_POINT('Ctrl Pts',(9.50217064222597,-0.116651839270521,
-41.9305954513151));
#34416=CARTESIAN_POINT('Ctrl Pts',(9.49487857746734,-0.0874975350060252,
-42.1362059880072));
#34417=CARTESIAN_POINT('Ctrl Pts',(9.48594038761699,-0.0549897319655466,
-42.4433074274479));
#34418=CARTESIAN_POINT('Ctrl Pts',(9.47883283572487,-0.0307036412911002,
-42.7625139069713));
#34419=CARTESIAN_POINT('Ctrl Pts',(9.4715738737315,-0.00920915185482917,
-43.1979630713915));
#34420=CARTESIAN_POINT('Ctrl Pts',(9.46617075949442,0.00030125175059658,
-43.7652339495534));
#34421=CARTESIAN_POINT('Ctrl Pts',(9.46386173516898,-0.00733827689215994,
-44.4805653014695));
#34422=CARTESIAN_POINT('Ctrl Pts',(9.46394450808348,-0.0204975884789352,
-45.1054543111399));
#34423=CARTESIAN_POINT('Ctrl Pts',(9.46435067476216,-0.0287494965312834,
-45.6224691455761));
#34424=CARTESIAN_POINT('Ctrl Pts',(9.46459707476204,-0.0320676494958033,
-46.0186216064772));
#34425=CARTESIAN_POINT('Ctrl Pts',(9.46456526055404,-0.0306772902459179,
-46.4231979182499));
#34426=CARTESIAN_POINT('Ctrl Pts',(9.46386003704854,-0.0199159967342241,
-46.9736983984273));
#34427=CARTESIAN_POINT('Ctrl Pts',(9.46224277548488,0.00123271037981269,
-47.3990882005854));
#34428=CARTESIAN_POINT('Ctrl Pts',(9.45947300888553,0.0355427847841118,
-47.8322468349079));
#34429=CARTESIAN_POINT('Ctrl Pts',(9.45761404741026,0.0547904732236308,
-48.0743676862649));
#34430=CARTESIAN_POINT('Ctrl Pts',(9.45387130200266,0.0965200563031265,
-48.5889071297665));
#34431=CARTESIAN_POINT('Ctrl Pts',(9.44729751772116,0.172672927165151,-49.4824938544509));
#34432=CARTESIAN_POINT('Ctrl Pts',(9.43800296747507,0.302828721577757,-50.7874940600758));
#34433=CARTESIAN_POINT('Ctrl Pts',(9.42760104368089,0.520617671817749,-52.3796782186102));
#34434=CARTESIAN_POINT('Ctrl Pts',(9.42148449284729,0.727489544375616,-53.4608837581059));
#34435=CARTESIAN_POINT('Ctrl Pts',(9.41801653726967,0.882776450636743,-54.1424217070253));
#34436=CARTESIAN_POINT('Ctrl Pts',(9.41660018054459,0.946065112992808,-54.4115221367208));
#34437=CARTESIAN_POINT('Ctrl Pts',(9.41377399906611,1.0807879654595,-54.9517633279573));
#34438=CARTESIAN_POINT('Ctrl Pts',(9.40885840442797,1.33482818349171,-55.891951541443));
#34439=CARTESIAN_POINT('Ctrl Pts',(9.39951864609365,1.91208396809229,-57.7584288631972));
#34440=CARTESIAN_POINT('Ctrl Pts',(9.39355010701788,2.50502947097712,-59.3241279180903));
#34441=CARTESIAN_POINT('Ctrl Pts',(9.39156343535068,2.95537803265398,-60.415272793405));
#34442=CARTESIAN_POINT('Ctrl Pts',(9.39136735927576,3.0140632876918,-60.5557152480889));
#34443=CARTESIAN_POINT('Ctrl Pts',(9.3910492684304,3.1317814670137,-60.8306909163205));
#34444=CARTESIAN_POINT('Ctrl Pts',(9.39071295906558,3.34426521613766,-61.3108788866971));
#34445=CARTESIAN_POINT('Ctrl Pts',(9.39078821554258,3.7875443137992,-62.2562486506828));
#34446=CARTESIAN_POINT('Ctrl Pts',(9.39213953428988,4.3247693680003,-63.3084130369635));
#34447=CARTESIAN_POINT('Ctrl Pts',(9.39388778754442,4.86620950375434,-64.3297613140723));
#34448=CARTESIAN_POINT('Ctrl Pts',(9.39486435610099,5.16777800376065,-64.8923576658369));
#34449=CARTESIAN_POINT('Ctrl Pts',(9.39544586818117,5.36557938810239,-65.2620471351256));
#34450=CARTESIAN_POINT('Ctrl Pts',(9.39581056127253,5.49645330380412,-65.5070425816499));
#34451=CARTESIAN_POINT('Ctrl Pts',(9.39613415269145,5.62566425274362,-65.7498409109864));
#34452=CARTESIAN_POINT('Ctrl Pts',(9.39636931187523,5.73689993095036,-65.9602257093019));
#34453=CARTESIAN_POINT('Ctrl Pts',(9.39648826638796,5.79989522799455,-66.0798446515712));
#34454=CARTESIAN_POINT('Ctrl Pts',(9.39665040100374,5.8938026825324,-66.2586777183794));
#34455=CARTESIAN_POINT('Ctrl Pts',(9.39674981576714,5.97076589573635,-66.4064051929983));
#34456=CARTESIAN_POINT('Ctrl Pts',(9.39685726595448,6.09638583511326,-66.6495173501779));
#34457=CARTESIAN_POINT('Ctrl Pts',(9.39695467963757,6.2340448976683,-66.9150063715849));
#34458=CARTESIAN_POINT('Ctrl Pts',(9.39710259783481,6.50421003572679,-67.4326708346839));
#34459=CARTESIAN_POINT('Ctrl Pts',(9.39725124719125,6.97766078616841,-68.3320276092932));
#34460=CARTESIAN_POINT('Ctrl Pts',(9.39721704222952,7.91638427079446,-70.0909389565235));
#34461=CARTESIAN_POINT('Ctrl Pts',(9.39695920064004,8.71295332911861,-71.5671178811821));
#34462=CARTESIAN_POINT('Ctrl Pts',(9.39697619655444,9.30799708286968,-72.686226807902));
#34463=CARTESIAN_POINT('Ctrl Pts',(9.39697930001536,9.44180033126638,-72.9378719364681));
#34464=CARTESIAN_POINT('Ctrl Pts',(9.39698400304045,9.70860585557645,-73.4396573013827));
#34465=CARTESIAN_POINT('Ctrl Pts',(9.39698710758693,10.0422490477591,-74.067148102403));
#34466=CARTESIAN_POINT('Ctrl Pts',(9.39698746336443,10.4422314152469,-74.8194059221752));
#34467=CARTESIAN_POINT('Ctrl Pts',(9.39698343039283,11.2419928422341,-76.3235423766373));
#34468=CARTESIAN_POINT('Ctrl Pts',(9.39697452470082,11.9081784818574,-77.5764661824382));
#34469=CARTESIAN_POINT('Ctrl Pts',(9.39697457998603,12.8780952426034,-79.4006170546344));
#34470=CARTESIAN_POINT('Ctrl Pts',(9.39697460873377,13.3146600052307,-80.2216773745254));
#34471=CARTESIAN_POINT('Ctrl Pts',(9.39697460873379,13.7511815926202,-81.0426550766237));
#34472=CARTESIAN_POINT('Ctrl Pts',(11.5895003465238,0.000421249146080626,
24.8306341860236));
#34473=CARTESIAN_POINT('Ctrl Pts',(11.5895349558891,0.000421265971284107,
24.7817548555947));
#34474=CARTESIAN_POINT('Ctrl Pts',(11.5895712425403,0.000421288380151196,
24.732876758355));
#34475=CARTESIAN_POINT('Ctrl Pts',(11.590000249277,0.000421335496354015,
24.1822624226437));
#34476=CARTESIAN_POINT('Ctrl Pts',(11.5903315807401,0.000420438478241857,
23.1780764140684));
#34477=CARTESIAN_POINT('Ctrl Pts',(11.5910956631355,0.000421514181210609,
21.1694719372929));
#34478=CARTESIAN_POINT('Ctrl Pts',(11.59395600421,0.000419556677115865,
19.6651937504487));
#34479=CARTESIAN_POINT('Ctrl Pts',(11.6000108331372,0.000419595016915984,
18.4140903993403));
#34480=CARTESIAN_POINT('Ctrl Pts',(11.6029134738436,0.000420193598292942,
17.911264557871));
#34481=CARTESIAN_POINT('Ctrl Pts',(11.610202940336,0.000421505558988271,
16.9072385975303));
#34482=CARTESIAN_POINT('Ctrl Pts',(11.6258359918673,0.000425254069881499,
15.1533902639501));
#34483=CARTESIAN_POINT('Ctrl Pts',(11.6407048266074,0.000420578030577308,
13.6513622787079));
#34484=CARTESIAN_POINT('Ctrl Pts',(11.65002661683,0.000415634117589493,
12.3967550004797));
#34485=CARTESIAN_POINT('Ctrl Pts',(11.6538355348768,0.000414271683788634,
11.8957647331824));
#34486=CARTESIAN_POINT('Ctrl Pts',(11.6616052574914,0.00040872892343895,
10.89387820218));
#34487=CARTESIAN_POINT('Ctrl Pts',(11.6750512732423,0.000399384798179506,
9.14004403088222));
#34488=CARTESIAN_POINT('Ctrl Pts',(11.6845336306305,0.000369136692087825,
7.63462505162104));
#34489=CARTESIAN_POINT('Ctrl Pts',(11.6887426152279,0.000360629362696536,
6.50185638510926));
#34490=CARTESIAN_POINT('Ctrl Pts',(11.6889829938694,0.00204940874441417,
6.23104218068182));
#34491=CARTESIAN_POINT('Ctrl Pts',(11.6871933797293,0.0108499136959918,
5.70761822167393));
#34492=CARTESIAN_POINT('Ctrl Pts',(11.6794103159137,0.0366529171734025,
4.80116829281341));
#34493=CARTESIAN_POINT('Ctrl Pts',(11.6551428675138,0.103926667440031,3.05766827252427));
#34494=CARTESIAN_POINT('Ctrl Pts',(11.6544067577611,0.0997159897208348,
1.67957314750907));
#34495=CARTESIAN_POINT('Ctrl Pts',(11.6956884426168,0.00524533581804662,
0.76907608223799));
#34496=CARTESIAN_POINT('Ctrl Pts',(11.7010331324381,-0.00612686295736921,
0.669109293389778));
#34497=CARTESIAN_POINT('Ctrl Pts',(11.7133419918826,-0.033295340217515,
0.460962228982755));
#34498=CARTESIAN_POINT('Ctrl Pts',(11.7388026574533,-0.0904451889914446,
0.0914601360013011));
#34499=CARTESIAN_POINT('Ctrl Pts',(11.7846067217235,-0.197828873089581,
-0.460490590649874));
#34500=CARTESIAN_POINT('Ctrl Pts',(11.8492755833482,-0.35785312251849,-1.15772429267139));
#34501=CARTESIAN_POINT('Ctrl Pts',(11.9422531726328,-0.597449389264225,
-2.13404256300419));
#34502=CARTESIAN_POINT('Ctrl Pts',(12.0600747368333,-0.915142274293143,
-3.43977101294881));
#34503=CARTESIAN_POINT('Ctrl Pts',(12.1317881784433,-1.11347752640962,-4.57760409191073));
#34504=CARTESIAN_POINT('Ctrl Pts',(12.1598433026514,-1.19302471328253,-5.31855920096231));
#34505=CARTESIAN_POINT('Ctrl Pts',(12.169366898184,-1.21964202475537,-5.58971844115356));
#34506=CARTESIAN_POINT('Ctrl Pts',(12.1849416948029,-1.26453163793054,-6.14133750050855));
#34507=CARTESIAN_POINT('Ctrl Pts',(12.2030002467654,-1.31956548681415,-7.0879167372753));
#34508=CARTESIAN_POINT('Ctrl Pts',(12.2090841204405,-1.34885175444332,-8.41047338620064));
#34509=CARTESIAN_POINT('Ctrl Pts',(12.2033198192615,-1.34791613453023,-9.68356162650418));
#34510=CARTESIAN_POINT('Ctrl Pts',(12.2001610304695,-1.3485209109719,-10.5492284134047));
#34511=CARTESIAN_POINT('Ctrl Pts',(12.199565240339,-1.35141229690972,-11.0359749983344));
#34512=CARTESIAN_POINT('Ctrl Pts',(12.1998293163945,-1.35407559411239,-11.2766596539298));
#34513=CARTESIAN_POINT('Ctrl Pts',(12.2002966711747,-1.35667249736963,-11.4571774087692));
#34514=CARTESIAN_POINT('Ctrl Pts',(12.200602535717,-1.35843107697228,-11.5876611958586));
#34515=CARTESIAN_POINT('Ctrl Pts',(12.2010332957154,-1.36147606105468,-11.8429321527371));
#34516=CARTESIAN_POINT('Ctrl Pts',(12.2014008783385,-1.36582617024926,-12.2909985688009));
#34517=CARTESIAN_POINT('Ctrl Pts',(12.2005528795049,-1.37230550341324,-13.4348799242311));
#34518=CARTESIAN_POINT('Ctrl Pts',(12.1958185922034,-1.36885998545949,-14.692157276302));
#34519=CARTESIAN_POINT('Ctrl Pts',(12.1916526864696,-1.36400843945851,-15.9427077708804));
#34520=CARTESIAN_POINT('Ctrl Pts',(12.1900893000376,-1.36197258417533,-16.5673646493878));
#34521=CARTESIAN_POINT('Ctrl Pts',(12.1893597741114,-1.36103431008563,-17.0670389593229));
#34522=CARTESIAN_POINT('Ctrl Pts',(12.1892071133706,-1.36086730651945,-17.316956074871));
#34523=CARTESIAN_POINT('Ctrl Pts',(12.1891850913752,-1.36088367403509,-17.5037103865457));
#34524=CARTESIAN_POINT('Ctrl Pts',(12.1891860726778,-1.36089370079563,-17.6285722135397));
#34525=CARTESIAN_POINT('Ctrl Pts',(12.1892466645591,-1.36091024622022,-17.8775969971028));
#34526=CARTESIAN_POINT('Ctrl Pts',(12.1893903663723,-1.3609200070653,-18.1270748121356));
#34527=CARTESIAN_POINT('Ctrl Pts',(12.1896069748992,-1.3609210606696,-18.3765523507506));
#34528=CARTESIAN_POINT('Ctrl Pts',(12.1897706375991,-1.36091754738905,-18.5325779604253));
#34529=CARTESIAN_POINT('Ctrl Pts',(12.1899173027073,-1.36091196273073,-18.6574255762084));
#34530=CARTESIAN_POINT('Ctrl Pts',(12.1900741058559,-1.36090430584617,-18.7823042848857));
#34531=CARTESIAN_POINT('Ctrl Pts',(12.1905441675585,-1.36087613957535,-19.1258297086731));
#34532=CARTESIAN_POINT('Ctrl Pts',(12.1915123396548,-1.36077757925637,-19.6885889384576));
#34533=CARTESIAN_POINT('Ctrl Pts',(12.1935748924666,-1.36042389655417,-20.690890665205));
#34534=CARTESIAN_POINT('Ctrl Pts',(12.1964140789255,-1.35950880721579,-21.9474356554848));
#34535=CARTESIAN_POINT('Ctrl Pts',(12.1980823823026,-1.35811531701347,-22.9568678500849));
#34536=CARTESIAN_POINT('Ctrl Pts',(12.1986778233842,-1.35694704435592,-23.5874635626913));
#34537=CARTESIAN_POINT('Ctrl Pts',(12.1988951249704,-1.35642925560143,-23.8372801898254));
#34538=CARTESIAN_POINT('Ctrl Pts',(12.1992557838325,-1.35521683352075,-24.3374364321954));
#34539=CARTESIAN_POINT('Ctrl Pts',(12.1997222650968,-1.35268582991751,-25.2142287410768));
#34540=CARTESIAN_POINT('Ctrl Pts',(12.1999918287177,-1.3483298012673,-26.469843102847));
#34541=CARTESIAN_POINT('Ctrl Pts',(12.2001331733731,-1.3430080053085,-27.9774101168199));
#34542=CARTESIAN_POINT('Ctrl Pts',(12.2002979616086,-1.34021231189827,-28.9810214667866));
#34543=CARTESIAN_POINT('Ctrl Pts',(12.2005179979553,-1.33902294947022,-29.5433690165917));
#34544=CARTESIAN_POINT('Ctrl Pts',(12.2007155568601,-1.33913234315464,-29.6579343007927));
#34545=CARTESIAN_POINT('Ctrl Pts',(12.2016183131347,-1.34064013032727,-29.894857818671));
#34546=CARTESIAN_POINT('Ctrl Pts',(12.2044109963861,-1.34640703943498,-30.3109049420008));
#34547=CARTESIAN_POINT('Ctrl Pts',(12.2138037264528,-1.36780107507898,-31.1631350360708));
#34548=CARTESIAN_POINT('Ctrl Pts',(12.2282678471616,-1.40267735858772,-32.1756131064741));
#34549=CARTESIAN_POINT('Ctrl Pts',(12.2359281634714,-1.42035992478456,-33.2268804247612));
#34550=CARTESIAN_POINT('Ctrl Pts',(12.235382686702,-1.41727505453408,-34.0340411863746));
#34551=CARTESIAN_POINT('Ctrl Pts',(12.2254752043518,-1.38978026876474,-34.8603776714585));
#34552=CARTESIAN_POINT('Ctrl Pts',(12.2104691370127,-1.34925733430161,-35.4236498731343));
#34553=CARTESIAN_POINT('Ctrl Pts',(12.1951752297892,-1.30790111826445,-35.8524630983525));
#34554=CARTESIAN_POINT('Ctrl Pts',(12.1825211824852,-1.27333639386323,-36.1563718706145));
#34555=CARTESIAN_POINT('Ctrl Pts',(12.1512525619581,-1.1880725012926,-36.7400470871197));
#34556=CARTESIAN_POINT('Ctrl Pts',(12.0823704341283,-1.00177550927921,-37.7333136575194));
#34557=CARTESIAN_POINT('Ctrl Pts',(11.912067166079,-0.539417026971565,-39.5844202785541));
#34558=CARTESIAN_POINT('Ctrl Pts',(11.7643012553191,-0.183649155381337,
-40.9505201179462));
#34559=CARTESIAN_POINT('Ctrl Pts',(11.7132560199656,-0.0769147300689789,
-41.8530590205573));
#34560=CARTESIAN_POINT('Ctrl Pts',(11.7030577355911,-0.0549797254856127,
-42.0664949301454));
#34561=CARTESIAN_POINT('Ctrl Pts',(11.6906565557908,-0.0307525519755015,
-42.3883700308207));
#34562=CARTESIAN_POINT('Ctrl Pts',(11.6809257359326,-0.0136401693481867,
-42.7197339938335));
#34563=CARTESIAN_POINT('Ctrl Pts',(11.6711343612843,0.000378588213563514,
-43.170388084499));
#34564=CARTESIAN_POINT('Ctrl Pts',(11.6641582404438,0.003870671157017,-43.7527445567746));
#34565=CARTESIAN_POINT('Ctrl Pts',(11.6618085968409,-0.00627095441501176,
-44.4803624481653));
#34566=CARTESIAN_POINT('Ctrl Pts',(11.6628519722898,-0.0187202388324247,
-45.1104330869402));
#34567=CARTESIAN_POINT('Ctrl Pts',(11.6643176229784,-0.0256880940942903,
-45.6286559926594));
#34568=CARTESIAN_POINT('Ctrl Pts',(11.665417654692,-0.0279705948420053,
-46.0242224672143));
#34569=CARTESIAN_POINT('Ctrl Pts',(11.6662197469886,-0.0257940182038288,
-46.4267149613217));
#34570=CARTESIAN_POINT('Ctrl Pts',(11.6664945399492,-0.0148137185444308,
-46.9724562252043));
#34571=CARTESIAN_POINT('Ctrl Pts',(11.6653371442479,0.00499710263825592,
-47.3920033430256));
#34572=CARTESIAN_POINT('Ctrl Pts',(11.6626865579812,0.0360646717714845,
-47.8180888050839));
#34573=CARTESIAN_POINT('Ctrl Pts',(11.6609970542061,0.0540060645333786,
-48.0621584055523));
#34574=CARTESIAN_POINT('Ctrl Pts',(11.6579125669985,0.0928044846859556,
-48.5768198708537));
#34575=CARTESIAN_POINT('Ctrl Pts',(11.6531862216885,0.16443908310244,-49.4725388962503));
#34576=CARTESIAN_POINT('Ctrl Pts',(11.6477776932751,0.289023855935045,-50.7794141693277));
#34577=CARTESIAN_POINT('Ctrl Pts',(11.6417051597372,0.501721528728834,-52.3744925130066));
#34578=CARTESIAN_POINT('Ctrl Pts',(11.6368682309341,0.706544305032596,-53.4574473486582));
#34579=CARTESIAN_POINT('Ctrl Pts',(11.6332778401015,0.86106650825881,-54.1400827334346));
#34580=CARTESIAN_POINT('Ctrl Pts',(11.631747464244,0.924228189408537,-54.4100019188139));
#34581=CARTESIAN_POINT('Ctrl Pts',(11.6284383863139,1.05893209788025,-54.9514885117027));
#34582=CARTESIAN_POINT('Ctrl Pts',(11.6220936677995,1.31365760989207,-55.893593887579));
#34583=CARTESIAN_POINT('Ctrl Pts',(11.6081597107898,1.89428780354141,-57.7622977018779));
#34584=CARTESIAN_POINT('Ctrl Pts',(11.5972576739243,2.49130687345031,-59.3278233751766));
#34585=CARTESIAN_POINT('Ctrl Pts',(11.5932461563346,2.94318498687134,-60.4180302768753));
#34586=CARTESIAN_POINT('Ctrl Pts',(11.5927990424572,3.002203182863,-60.5586409281497));
#34587=CARTESIAN_POINT('Ctrl Pts',(11.5919848816902,3.12053101962373,-60.833766518273));
#34588=CARTESIAN_POINT('Ctrl Pts',(11.5907857315375,3.33417256712251,-61.3142431871049));
#34589=CARTESIAN_POINT('Ctrl Pts',(11.5891815844952,3.77988417078737,-62.2599187917617));
#34590=CARTESIAN_POINT('Ctrl Pts',(11.5887569117294,4.31997925913707,-63.3121003364946));
#34591=CARTESIAN_POINT('Ctrl Pts',(11.5889649652932,4.86391151043664,-64.3331503596558));
#34592=CARTESIAN_POINT('Ctrl Pts',(11.5891777174056,5.16666562729302,-64.8954629679139));
#34593=CARTESIAN_POINT('Ctrl Pts',(11.5892979571789,5.36513161334473,-65.264909254195));
#34594=CARTESIAN_POINT('Ctrl Pts',(11.5893689104412,5.49641360042041,-65.5097267921224));
#34595=CARTESIAN_POINT('Ctrl Pts',(11.589417857095,5.62597475449768,-65.7523254738009));
#34596=CARTESIAN_POINT('Ctrl Pts',(11.5894326263675,5.73746232256607,-65.9625116689282));
#34597=CARTESIAN_POINT('Ctrl Pts',(11.5894312284362,5.80058491029846,-66.082010275755));
#34598=CARTESIAN_POINT('Ctrl Pts',(11.5894186243491,5.89466641583682,-66.2606557110124));
#34599=CARTESIAN_POINT('Ctrl Pts',(11.5893837333011,5.97173763063546,-66.4082123733179));
#34600=CARTESIAN_POINT('Ctrl Pts',(11.5892865435401,6.09748576135826,-66.6510196056842));
#34601=CARTESIAN_POINT('Ctrl Pts',(11.5891983703341,6.23529702121285,-66.9162681907086));
#34602=CARTESIAN_POINT('Ctrl Pts',(11.5890696535673,6.50562214135505,-67.4334602383677));
#34603=CARTESIAN_POINT('Ctrl Pts',(11.588952931312,6.97910540105887,-68.3321328965063));
#34604=CARTESIAN_POINT('Ctrl Pts',(11.5890635559689,7.91715809051001,-70.0901682506227));
#34605=CARTESIAN_POINT('Ctrl Pts',(11.5893843546621,8.71297649813509,-71.5665593860804));
#34606=CARTESIAN_POINT('Ctrl Pts',(11.5893882636949,9.30835753260348,-72.6862749620062));
#34607=CARTESIAN_POINT('Ctrl Pts',(11.5893894963938,9.44214102812561,-72.9378761916324));
#34608=CARTESIAN_POINT('Ctrl Pts',(11.5893911749115,9.70895971908889,-73.4396767585204));
#34609=CARTESIAN_POINT('Ctrl Pts',(11.5893916578803,10.0425945061019,-74.0671471010587));
#34610=CARTESIAN_POINT('Ctrl Pts',(11.5893914474645,10.4425761394456,-74.8194037472044));
#34611=CARTESIAN_POINT('Ctrl Pts',(11.5893891715325,11.2423255426347,-76.3235281075312));
#34612=CARTESIAN_POINT('Ctrl Pts',(11.5893829173179,11.9085001528643,-77.5764577736852));
#34613=CARTESIAN_POINT('Ctrl Pts',(11.5893813335251,12.8784211622576,-79.4006208947267));
#34614=CARTESIAN_POINT('Ctrl Pts',(11.5893805197922,13.3149827504299,-80.2216774359031));
#34615=CARTESIAN_POINT('Ctrl Pts',(11.5893805197922,13.7515043378194,-81.0426551380014));
#34616=CARTESIAN_POINT('Ctrl Pts',(14.0944631116312,0.000239315415103097,
24.8306344290317));
#34617=CARTESIAN_POINT('Ctrl Pts',(14.0945051703635,0.000239310373125806,
24.7817551065899));
#34618=CARTESIAN_POINT('Ctrl Pts',(14.094549283557,0.000239308494718214,
24.7328769301283));
#34619=CARTESIAN_POINT('Ctrl Pts',(14.0950700886175,0.000239130724081029,
24.1822656284498));
#34620=CARTESIAN_POINT('Ctrl Pts',(14.0954676202415,0.000238294797979617,
23.1781042478625));
#34621=CARTESIAN_POINT('Ctrl Pts',(14.0963939340577,0.000238593416326289,
21.169502605));
#34622=CARTESIAN_POINT('Ctrl Pts',(14.0998586839277,0.000235783298849487,
19.6652856273898));
#34623=CARTESIAN_POINT('Ctrl Pts',(14.1072148356599,0.000232983959125036,
18.4142089765319));
#34624=CARTESIAN_POINT('Ctrl Pts',(14.1107427068927,0.00023202792923821,
17.9113877798041));
#34625=CARTESIAN_POINT('Ctrl Pts',(14.1196006764428,0.000229423541213125,
16.907379540741));
#34626=CARTESIAN_POINT('Ctrl Pts',(14.1386011789869,0.000224523189695424,
15.1535492780035));
#34627=CARTESIAN_POINT('Ctrl Pts',(14.1566536268648,0.000214244067486069,
13.6516594845658));
#34628=CARTESIAN_POINT('Ctrl Pts',(14.1679809427275,0.000207077916971663,
12.3971158810473));
#34629=CARTESIAN_POINT('Ctrl Pts',(14.1726133672633,0.000204695620792798,
11.8961428873256));
#34630=CARTESIAN_POINT('Ctrl Pts',(14.1820601727929,0.000198134753947263,
10.8942756519075));
#34631=CARTESIAN_POINT('Ctrl Pts',(14.1984197580504,0.000187296246933722,
9.14058768641498));
#34632=CARTESIAN_POINT('Ctrl Pts',(14.2098938545934,0.000163375509298961,
7.63525678927255));
#34633=CARTESIAN_POINT('Ctrl Pts',(14.2149923557477,0.000155107245014959,
6.50340589673276));
#34634=CARTESIAN_POINT('Ctrl Pts',(14.215505664609,0.000961838336879548,
6.24294842492752));
#34635=CARTESIAN_POINT('Ctrl Pts',(14.214494741344,0.00520287161040355,
5.73074485996725));
#34636=CARTESIAN_POINT('Ctrl Pts',(14.208472871761,0.0177970441974879,4.83834267556141));
#34637=CARTESIAN_POINT('Ctrl Pts',(14.1882723930367,0.0514117428276515,
3.08651160205499));
#34638=CARTESIAN_POINT('Ctrl Pts',(14.1870202056287,0.0504889425535852,
1.64352233320098));
#34639=CARTESIAN_POINT('Ctrl Pts',(14.2222965127537,-0.00105218817305978,
0.65884157414066));
#34640=CARTESIAN_POINT('Ctrl Pts',(14.2268798643112,-0.00758097557180187,
0.545811031676352));
#34641=CARTESIAN_POINT('Ctrl Pts',(14.2374646281445,-0.0227769719229255,
0.315844136561766));
#34642=CARTESIAN_POINT('Ctrl Pts',(14.2594646628206,-0.0543499942763772,
-0.0887617804289952));
#34643=CARTESIAN_POINT('Ctrl Pts',(14.29940595502,-0.111800663915594,-0.677724198690524));
#34644=CARTESIAN_POINT('Ctrl Pts',(14.3563852189701,-0.193695842118945,
-1.40127978883877));
#34645=CARTESIAN_POINT('Ctrl Pts',(14.438257220335,-0.311431996465603,-2.38958521327673));
#34646=CARTESIAN_POINT('Ctrl Pts',(14.5400067851163,-0.458336815684018,
-3.66964344286333));
#34647=CARTESIAN_POINT('Ctrl Pts',(14.5973641928648,-0.543987179230505,
-4.7410559036543));
#34648=CARTESIAN_POINT('Ctrl Pts',(14.6189747978427,-0.577967613166301,
-5.42511263803678));
#34649=CARTESIAN_POINT('Ctrl Pts',(14.6266712537219,-0.589946057792036,
-5.68610831669644));
#34650=CARTESIAN_POINT('Ctrl Pts',(14.6388917659254,-0.610003749620148,
-6.21288609120711));
#34651=CARTESIAN_POINT('Ctrl Pts',(14.6527014652724,-0.635210361922765,
-7.12556047241501));
#34652=CARTESIAN_POINT('Ctrl Pts',(14.6557197938956,-0.649738254045434,
-8.4149020244448));
#34653=CARTESIAN_POINT('Ctrl Pts',(14.6487675087243,-0.650689112584959,
-9.67872412606275));
#34654=CARTESIAN_POINT('Ctrl Pts',(14.6449804595606,-0.65169415946043,-10.5495371614848));
#34655=CARTESIAN_POINT('Ctrl Pts',(14.6440223013186,-0.653390173386025,
-11.0427651834159));
#34656=CARTESIAN_POINT('Ctrl Pts',(14.6440935479156,-0.654782110586744,
-11.2878771507872));
#34657=CARTESIAN_POINT('Ctrl Pts',(14.644410748038,-0.656098167934278,-11.4720377844606));
#34658=CARTESIAN_POINT('Ctrl Pts',(14.644596826737,-0.656954171553811,-11.6003216120659));
#34659=CARTESIAN_POINT('Ctrl Pts',(14.6448506490134,-0.65846059666502,-11.8539261484059));
#34660=CARTESIAN_POINT('Ctrl Pts',(14.6450078304074,-0.660620745336611,
-12.2980494275863));
#34661=CARTESIAN_POINT('Ctrl Pts',(14.6441144207941,-0.663938980749091,
-13.4344334651777));
#34662=CARTESIAN_POINT('Ctrl Pts',(14.6403828036926,-0.66250451342443,-14.6872309086493));
#34663=CARTESIAN_POINT('Ctrl Pts',(14.6371980784744,-0.660296369796018,
-15.9381573936582));
#34664=CARTESIAN_POINT('Ctrl Pts',(14.6360059921958,-0.65935859603253,-16.5640543178105));
#34665=CARTESIAN_POINT('Ctrl Pts',(14.635462637249,-0.658922651127044,-17.0654182024739));
#34666=CARTESIAN_POINT('Ctrl Pts',(14.635352481037,-0.658845427413407,-17.316400499451));
#34667=CARTESIAN_POINT('Ctrl Pts',(14.6353417591257,-0.658853429342191,
-17.5040152635562));
#34668=CARTESIAN_POINT('Ctrl Pts',(14.6353571064953,-0.658854724164119,
-17.6287585220641));
#34669=CARTESIAN_POINT('Ctrl Pts',(14.6354719377722,-0.658840559604473,
-17.8779376136121));
#34670=CARTESIAN_POINT('Ctrl Pts',(14.6357009996904,-0.658803757903174,
-18.1274062923526));
#34671=CARTESIAN_POINT('Ctrl Pts',(14.6360285153936,-0.658745667646573,
-18.3769412078243));
#34672=CARTESIAN_POINT('Ctrl Pts',(14.6362692312006,-0.658701461788393,
-18.5329793145762));
#34673=CARTESIAN_POINT('Ctrl Pts',(14.6364814865989,-0.658661504375778,
-18.6578404208514));
#34674=CARTESIAN_POINT('Ctrl Pts',(14.6367059358736,-0.658618534443917,
-18.7827285092989));
#34675=CARTESIAN_POINT('Ctrl Pts',(14.6373687437213,-0.658490720845063,
-19.1262718546939));
#34676=CARTESIAN_POINT('Ctrl Pts',(14.6386717472663,-0.658222632735348,
-19.6890094189946));
#34677=CARTESIAN_POINT('Ctrl Pts',(14.6411978702278,-0.657659795614467,
-20.6911364612033));
#34678=CARTESIAN_POINT('Ctrl Pts',(14.6439798247638,-0.656868696869042,
-21.9471940091887));
#34679=CARTESIAN_POINT('Ctrl Pts',(14.6441686157926,-0.656448414793447,
-22.9559680415154));
#34680=CARTESIAN_POINT('Ctrl Pts',(14.6431430916204,-0.656300061609959,
-23.5860567718861));
#34681=CARTESIAN_POINT('Ctrl Pts',(14.6426229433556,-0.656246471252463,
-23.8355925193941));
#34682=CARTESIAN_POINT('Ctrl Pts',(14.6411775215826,-0.65615890474012,-24.3353020723151));
#34683=CARTESIAN_POINT('Ctrl Pts',(14.6377218693294,-0.656040548619147,
-25.2114694865791));
#34684=CARTESIAN_POINT('Ctrl Pts',(14.630931002644,-0.655932213546865,-26.4666335432331));
#34685=CARTESIAN_POINT('Ctrl Pts',(14.6223146384926,-0.655668239594834,
-27.9745595516146));
#34686=CARTESIAN_POINT('Ctrl Pts',(14.6179171860164,-0.655445702698336,
-28.9786726424719));
#34687=CARTESIAN_POINT('Ctrl Pts',(14.6162837788159,-0.655294134551463,
-29.5419272467765));
#34688=CARTESIAN_POINT('Ctrl Pts',(14.6160526186354,-0.655431598986769,
-29.6618678131118));
#34689=CARTESIAN_POINT('Ctrl Pts',(14.616077382021,-0.656336226474451,-29.9056909605988));
#34690=CARTESIAN_POINT('Ctrl Pts',(14.617272582571,-0.659413701806968,-30.3331582640928));
#34691=CARTESIAN_POINT('Ctrl Pts',(14.6232727430873,-0.670210520658779,
-31.1983989008025));
#34692=CARTESIAN_POINT('Ctrl Pts',(14.6337803186591,-0.687008466127124,
-32.2067891285952));
#34693=CARTESIAN_POINT('Ctrl Pts',(14.6387619758346,-0.695431285875479,
-33.2344469506228));
#34694=CARTESIAN_POINT('Ctrl Pts',(14.6374425383742,-0.694208271454865,
-34.0143290999874));
#34695=CARTESIAN_POINT('Ctrl Pts',(14.6287348608639,-0.681999141243495,
-34.8034317094201));
#34696=CARTESIAN_POINT('Ctrl Pts',(14.6163979205044,-0.664066380160658,
-35.3354422613335));
#34697=CARTESIAN_POINT('Ctrl Pts',(14.6040256480247,-0.645869465357065,
-35.7381142952021));
#34698=CARTESIAN_POINT('Ctrl Pts',(14.5941965503113,-0.631098851807827,
-36.0162513416395));
#34699=CARTESIAN_POINT('Ctrl Pts',(14.5692778703312,-0.593921211685036,
-36.5604144990715));
#34700=CARTESIAN_POINT('Ctrl Pts',(14.5136952188433,-0.511016907625734,
-37.4982534980529));
#34701=CARTESIAN_POINT('Ctrl Pts',(14.3688154380279,-0.296013867944767,
-39.3038417030766));
#34702=CARTESIAN_POINT('Ctrl Pts',(14.2412748366334,-0.103913541802183,
-40.7308966430827));
#34703=CARTESIAN_POINT('Ctrl Pts',(14.2007198503395,-0.041093094070166,
-41.7462840081312));
#34704=CARTESIAN_POINT('Ctrl Pts',(14.1926845082915,-0.0295996644645384,
-41.9714637433589));
#34705=CARTESIAN_POINT('Ctrl Pts',(14.1831712501751,-0.0177873381933792,
-42.3151913299676));
#34706=CARTESIAN_POINT('Ctrl Pts',(14.175954585427,-0.0109313467580231,
-42.6642712761484));
#34707=CARTESIAN_POINT('Ctrl Pts',(14.1690727655943,-0.00731900968447937,
-43.1369985049661));
#34708=CARTESIAN_POINT('Ctrl Pts',(14.1649874111451,-0.0113324728833667,
-43.7412301831783));
#34709=CARTESIAN_POINT('Ctrl Pts',(14.1653540359968,-0.0230281051507635,
-44.4870156367657));
#34710=CARTESIAN_POINT('Ctrl Pts',(14.168437914655,-0.0323762303982092,
-45.1252156814221));
#34711=CARTESIAN_POINT('Ctrl Pts',(14.1715872552744,-0.0356362457752205,
-45.645851223175));
#34712=CARTESIAN_POINT('Ctrl Pts',(14.1740599557543,-0.0349179086061656,
-46.0411583115204));
#34713=CARTESIAN_POINT('Ctrl Pts',(14.1763997595407,-0.0299574615799581,
-46.4413118080271));
#34714=CARTESIAN_POINT('Ctrl Pts',(14.1790129891584,-0.0162060290324866,
-46.9811770540874));
#34715=CARTESIAN_POINT('Ctrl Pts',(14.1800566255083,0.00387885879804714,
-47.3931509835375));
#34716=CARTESIAN_POINT('Ctrl Pts',(14.1799839193984,0.0328654514553911,
-47.8099162855327));
#34717=CARTESIAN_POINT('Ctrl Pts',(14.1801699126152,0.050442263674094,-48.0585622102138));
#34718=CARTESIAN_POINT('Ctrl Pts',(14.1813949791877,0.0887586200856952,
-48.5757443673385));
#34719=CARTESIAN_POINT('Ctrl Pts',(14.1854212572758,0.161526430360534,-49.4778028225827));
#34720=CARTESIAN_POINT('Ctrl Pts',(14.1945592362753,0.291531467721919,-50.7883928435346));
#34721=CARTESIAN_POINT('Ctrl Pts',(14.2042550733362,0.513009107213242,-52.3831151560713));
#34722=CARTESIAN_POINT('Ctrl Pts',(14.2051663413128,0.721191364602573,-53.4616910628258));
#34723=CARTESIAN_POINT('Ctrl Pts',(14.2025787229755,0.875692912286117,-54.1407068771491));
#34724=CARTESIAN_POINT('Ctrl Pts',(14.2012739081521,0.939052912013921,-54.4104195310996));
#34725=CARTESIAN_POINT('Ctrl Pts',(14.1976254729671,1.07375873756196,-54.9508991578226));
#34726=CARTESIAN_POINT('Ctrl Pts',(14.1889001249657,1.3280120419816,-55.8918948767622));
#34727=CARTESIAN_POINT('Ctrl Pts',(14.1647212737922,1.90595529360788,-57.7590647206015));
#34728=CARTESIAN_POINT('Ctrl Pts',(14.1415184678372,2.49993288989735,-59.3250783966603));
#34729=CARTESIAN_POINT('Ctrl Pts',(14.131970141928,2.95077088735296,-60.4160582227018));
#34730=CARTESIAN_POINT('Ctrl Pts',(14.1307710836269,3.00955831636239,-60.5565771168024));
#34731=CARTESIAN_POINT('Ctrl Pts',(14.1284534374888,3.12746976575313,-60.831640867667));
#34732=CARTESIAN_POINT('Ctrl Pts',(14.1245188339413,3.3403348058412,-61.3119979220487));
#34733=CARTESIAN_POINT('Ctrl Pts',(14.1172208409135,3.7844632034876,-62.2576103132215));
#34734=CARTESIAN_POINT('Ctrl Pts',(14.1101772483488,4.32279535372546,-63.3099087432315));
#34735=CARTESIAN_POINT('Ctrl Pts',(14.1043800409819,4.86523831329963,-64.331189455735));
#34736=CARTESIAN_POINT('Ctrl Pts',(14.1015589331006,5.16728968206662,-64.8936695292806));
#34737=CARTESIAN_POINT('Ctrl Pts',(14.0998535271436,5.36536341095623,-65.2632505212294));
#34738=CARTESIAN_POINT('Ctrl Pts',(14.0987631670646,5.49640348952483,-65.5081634934525));
#34739=CARTESIAN_POINT('Ctrl Pts',(14.097740478461,5.62575958346341,-65.750870239036));
#34740=CARTESIAN_POINT('Ctrl Pts',(14.0969055959606,5.737097329896,-65.9611607932242));
#34741=CARTESIAN_POINT('Ctrl Pts',(14.0964453913745,5.80014387688518,-66.0807225592858));
#34742=CARTESIAN_POINT('Ctrl Pts',(14.0957720260039,5.894120752074,-66.2594662298233));
#34743=CARTESIAN_POINT('Ctrl Pts',(14.0952453994318,5.97112719209651,-66.4071136441018));
#34744=CARTESIAN_POINT('Ctrl Pts',(14.094420702844,6.09679499953658,-66.6500823173283));
#34745=CARTESIAN_POINT('Ctrl Pts',(14.0936733266644,6.2345195842633,-66.9154735311475));
#34746=CARTESIAN_POINT('Ctrl Pts',(14.0925563499899,6.50475175827377,-67.4329375581774));
#34747=CARTESIAN_POINT('Ctrl Pts',(14.0914884899755,6.97822414671521,-68.3320177551548));
#34748=CARTESIAN_POINT('Ctrl Pts',(14.0920786701469,7.91667658554508,-70.0905855126675));
#34749=CARTESIAN_POINT('Ctrl Pts',(14.0944616232842,8.71295349364137,-71.5668686173992));
#34750=CARTESIAN_POINT('Ctrl Pts',(14.0944203771024,9.30813886155358,-72.6862306066469));
#34751=CARTESIAN_POINT('Ctrl Pts',(14.0944129266693,9.44193414211487,-72.9378583214016));
#34752=CARTESIAN_POINT('Ctrl Pts',(14.094401644644,9.70874540476567,-73.4396508401897));
#34753=CARTESIAN_POINT('Ctrl Pts',(14.094393790156,10.0423867401557,-74.067135425168));
#34754=CARTESIAN_POINT('Ctrl Pts',(14.0943927400073,10.442369684355,-74.8193939097495));
#34755=CARTESIAN_POINT('Ctrl Pts',(14.094401938375,11.2421279686844,-76.3235272219561));
#34756=CARTESIAN_POINT('Ctrl Pts',(14.0944215158371,11.9083145311271,-77.576458354187));
#34757=CARTESIAN_POINT('Ctrl Pts',(14.0944204190697,12.8782355883391,-79.4006165662628));
#34758=CARTESIAN_POINT('Ctrl Pts',(14.0944198510847,13.3148007666061,-80.2216772868161));
#34759=CARTESIAN_POINT('Ctrl Pts',(14.0944198510847,13.7513223539956,-81.0426549889144));
#34760=CARTESIAN_POINT('Ctrl Pts',(16.9134010704912,-0.00101211290211373,
24.8306360281983));
#34761=CARTESIAN_POINT('Ctrl Pts',(16.9134515851132,-0.00101216298668399,
24.7817567553152));
#34762=CARTESIAN_POINT('Ctrl Pts',(16.9135045614701,-0.00101221733777369,
24.7328785600789));
#34763=CARTESIAN_POINT('Ctrl Pts',(16.9141302683925,-0.00101277382828913,
24.1822701699722));
#34764=CARTESIAN_POINT('Ctrl Pts',(16.9146093969652,-0.00101336582011031,
23.1781289778484));
#34765=CARTESIAN_POINT('Ctrl Pts',(16.9157222684248,-0.00101635417976157,
21.1695304690424));
#34766=CARTESIAN_POINT('Ctrl Pts',(16.919887647335,-0.00101909292100717,
19.6653620532305));
#34767=CARTESIAN_POINT('Ctrl Pts',(16.9287242477762,-0.00102394440616367,
18.4143064981284));
#34768=CARTESIAN_POINT('Ctrl Pts',(16.9329616521634,-0.00102672623135195,
17.9114915242589));
#34769=CARTESIAN_POINT('Ctrl Pts',(16.9436018359616,-0.00103395784223769,
16.9074991314347));
#34770=CARTESIAN_POINT('Ctrl Pts',(16.9664240149538,-0.00104977486294956,
15.1536831036689));
#34771=CARTESIAN_POINT('Ctrl Pts',(16.9881142952943,-0.00105774583357663,
13.6518945109012));
#34772=CARTESIAN_POINT('Ctrl Pts',(17.0017205179854,-0.00105612070077724,
12.3973905181308));
#34773=CARTESIAN_POINT('Ctrl Pts',(17.00728354403,-0.00105509932350135,
11.8964263867371));
#34774=CARTESIAN_POINT('Ctrl Pts',(17.0186292831805,-0.00104972614985391,
10.8945690573246));
#34775=CARTESIAN_POINT('Ctrl Pts',(17.038273396033,-0.00103592836115452,
9.14098616641578));
#34776=CARTESIAN_POINT('Ctrl Pts',(17.0520731254646,-0.00101141481218296,
7.63574208026637));
#34777=CARTESIAN_POINT('Ctrl Pts',(17.0582013852299,-0.00100031734776509,
6.50459176410634));
#34778=CARTESIAN_POINT('Ctrl Pts',(17.0592472161264,-0.000807859651648968,
6.25190653752823));
#34779=CARTESIAN_POINT('Ctrl Pts',(17.0602873551709,0.000198982466678631,
5.74812435408048));
#34780=CARTESIAN_POINT('Ctrl Pts',(17.0598280761885,0.00321326207857862,
4.86635425594689));
#34781=CARTESIAN_POINT('Ctrl Pts',(17.0535730927932,0.0112852006322439,
3.10810905803595));
#34782=CARTESIAN_POINT('Ctrl Pts',(17.0521709339728,0.0112998091967429,
1.61686178593503));
#34783=CARTESIAN_POINT('Ctrl Pts',(17.0653475382084,-0.0016525451973971,
0.575295319315679));
#34784=CARTESIAN_POINT('Ctrl Pts',(17.0670550137546,-0.00333319431329617,
0.452234021601371));
#34785=CARTESIAN_POINT('Ctrl Pts',(17.0709941824522,-0.00720646393610515,
0.205334822652025));
#34786=CARTESIAN_POINT('Ctrl Pts',(17.0791668908371,-0.015235953441166,
-0.226906573901212));
#34787=CARTESIAN_POINT('Ctrl Pts',(17.093976404849,-0.0297392650086584,
-0.846084503850126));
#34788=CARTESIAN_POINT('Ctrl Pts',(17.1150350693186,-0.0503005092990941,
-1.59187825505627));
#34789=CARTESIAN_POINT('Ctrl Pts',(17.1452781567032,-0.079676674057784,
-2.59060025215715));
#34790=CARTESIAN_POINT('Ctrl Pts',(17.1828830449709,-0.116026267737767,
-3.84795045468806));
#34791=CARTESIAN_POINT('Ctrl Pts',(17.20367526053,-0.13689468150225,-4.86553318329858));
#34792=CARTESIAN_POINT('Ctrl Pts',(17.2108571856803,-0.145209364453794,
-5.5058282838844));
#34793=CARTESIAN_POINT('Ctrl Pts',(17.2133370193797,-0.148277992537555,
-5.75901501432666));
#34794=CARTESIAN_POINT('Ctrl Pts',(17.2168625181439,-0.153461595669578,
-6.26684228454734));
#34795=CARTESIAN_POINT('Ctrl Pts',(17.2196570823651,-0.160268540870484,
-7.15387174200375));
#34796=CARTESIAN_POINT('Ctrl Pts',(17.2161957907094,-0.164846610753823,
-8.41831375137636));
#34797=CARTESIAN_POINT('Ctrl Pts',(17.2086652847334,-0.165894483071219,
-9.67542171650664));
#34798=CARTESIAN_POINT('Ctrl Pts',(17.204344428868,-0.166484237745355,-10.5503473101162));
#34799=CARTESIAN_POINT('Ctrl Pts',(17.202591260253,-0.167023235471124,-11.0486030835193));
#34800=CARTESIAN_POINT('Ctrl Pts',(17.2020271185242,-0.167400366556015,
-11.2971269343835));
#34801=CARTESIAN_POINT('Ctrl Pts',(17.2017475472665,-0.167740422767266,
-11.48409458387));
#34802=CARTESIAN_POINT('Ctrl Pts',(17.2015524547536,-0.16794943888993,-11.610846864052));
#34803=CARTESIAN_POINT('Ctrl Pts',(17.2011370054641,-0.168295419965447,
-11.8633836146047));
#34804=CARTESIAN_POINT('Ctrl Pts',(17.2003497396288,-0.168720501775088,
-12.3048501423687));
#34805=CARTESIAN_POINT('Ctrl Pts',(17.1980759356503,-0.168991746416044,
-13.4361686515847));
#34806=CARTESIAN_POINT('Ctrl Pts',(17.195166342771,-0.16748464734297,-14.6856322936344));
#34807=CARTESIAN_POINT('Ctrl Pts',(17.1929427647513,-0.166025264204655,
-15.936236513704));
#34808=CARTESIAN_POINT('Ctrl Pts',(17.192091582413,-0.165457473599947,-16.5626055131858));
#34809=CARTESIAN_POINT('Ctrl Pts',(17.1916233913902,-0.165193040786199,
-17.0647803125105));
#34810=CARTESIAN_POINT('Ctrl Pts',(17.1914677453772,-0.165139481591272,
-17.3162986549023));
#34811=CARTESIAN_POINT('Ctrl Pts',(17.1913850731145,-0.165134236199292,
-17.5043622594433));
#34812=CARTESIAN_POINT('Ctrl Pts',(17.191348644696,-0.16512106484283,-17.6292564913955));
#34813=CARTESIAN_POINT('Ctrl Pts',(17.1913446759282,-0.165061999303678,
-17.8787680895582));
#34814=CARTESIAN_POINT('Ctrl Pts',(17.1914332508204,-0.164961471165937,
-18.1284650671892));
#34815=CARTESIAN_POINT('Ctrl Pts',(17.1916038734292,-0.164828811201584,
-18.3781744105982));
#34816=CARTESIAN_POINT('Ctrl Pts',(17.1917401349492,-0.164736014496021,
-18.5342875656331));
#34817=CARTESIAN_POINT('Ctrl Pts',(17.1918657123936,-0.164656910754746,
-18.6591925189444));
#34818=CARTESIAN_POINT('Ctrl Pts',(17.1920016369369,-0.164574886043304,
-18.7841123853212));
#34819=CARTESIAN_POINT('Ctrl Pts',(17.1924117324506,-0.164345436637,-19.1276903432311));
#34820=CARTESIAN_POINT('Ctrl Pts',(17.1932699185797,-0.163941364873975,
-19.6902183631619));
#34821=CARTESIAN_POINT('Ctrl Pts',(17.1949883319485,-0.163455992169393,
-20.691191527286));
#34822=CARTESIAN_POINT('Ctrl Pts',(17.1969478648271,-0.163637135736605,
-21.9444203752336));
#34823=CARTESIAN_POINT('Ctrl Pts',(17.1969970314627,-0.165760114789861,
-22.9494207069731));
#34824=CARTESIAN_POINT('Ctrl Pts',(17.1961696538154,-0.167927488336689,
-23.576699079459));
#34825=CARTESIAN_POINT('Ctrl Pts',(17.1957545684123,-0.16889756834329,-23.824580657638));
#34826=CARTESIAN_POINT('Ctrl Pts',(17.1946012022147,-0.171294332463981,
-24.3217271026583));
#34827=CARTESIAN_POINT('Ctrl Pts',(17.1918508109013,-0.176506695480344,
-25.194230216388));
#34828=CARTESIAN_POINT('Ctrl Pts',(17.1864385424517,-0.186161713891325,
-26.4470593020611));
#34829=CARTESIAN_POINT('Ctrl Pts',(17.179693734892,-0.198235214341492,-27.9566636321236));
#34830=CARTESIAN_POINT('Ctrl Pts',(17.1764096119066,-0.204826586355265,
-28.9647261094821));
#34831=CARTESIAN_POINT('Ctrl Pts',(17.1753272541737,-0.207458681419564,
-29.5313529950025));
#34832=CARTESIAN_POINT('Ctrl Pts',(17.1751445967002,-0.208063086582707,
-29.6554266700394));
#34833=CARTESIAN_POINT('Ctrl Pts',(17.1749891798098,-0.209424878074251,
-29.9049026660955));
#34834=CARTESIAN_POINT('Ctrl Pts',(17.1752153459553,-0.212141967300124,
-30.3416243728318));
#34835=CARTESIAN_POINT('Ctrl Pts',(17.1772652557581,-0.21852268673992,-31.2180724911193));
#34836=CARTESIAN_POINT('Ctrl Pts',(17.1814166304052,-0.226246158720518,
-32.2247964553449));
#34837=CARTESIAN_POINT('Ctrl Pts',(17.1837242446055,-0.230889730583628,
-33.2358402786202));
#34838=CARTESIAN_POINT('Ctrl Pts',(17.1836212786991,-0.231969424975495,
-33.9959253124533));
#34839=CARTESIAN_POINT('Ctrl Pts',(17.180761376691,-0.229833784540344,-34.7575837027073));
#34840=CARTESIAN_POINT('Ctrl Pts',(17.1764123040643,-0.22565813026792,-35.2662106297554));
#34841=CARTESIAN_POINT('Ctrl Pts',(17.1719958652942,-0.221245152351467,
-35.6490605845432));
#34842=CARTESIAN_POINT('Ctrl Pts',(17.16849832909,-0.217712347575618,-35.9073148872236));
#34843=CARTESIAN_POINT('Ctrl Pts',(17.1596174202635,-0.208535106444459,
-36.420556897512));
#34844=CARTESIAN_POINT('Ctrl Pts',(17.1398262512644,-0.187586376473583,
-37.3140101396874));
#34845=CARTESIAN_POINT('Ctrl Pts',(17.0889808123628,-0.131047673218112,
-39.0817287769171));
#34846=CARTESIAN_POINT('Ctrl Pts',(17.0454414315167,-0.0761651363072375,
-40.5684528421309));
#34847=CARTESIAN_POINT('Ctrl Pts',(17.0318850438195,-0.0539912644416674,
-41.6732315274097));
#34848=CARTESIAN_POINT('Ctrl Pts',(17.0292214004439,-0.0505667957516916,
-41.907605347663));
#34849=CARTESIAN_POINT('Ctrl Pts',(17.0261376777833,-0.0483916202365658,
-42.2683784749758));
#34850=CARTESIAN_POINT('Ctrl Pts',(17.0238733039162,-0.0487778072880304,
-42.6312292904252));
#34851=CARTESIAN_POINT('Ctrl Pts',(17.0218305108725,-0.0518242957205186,
-43.1211998751754));
#34852=CARTESIAN_POINT('Ctrl Pts',(17.0208767056471,-0.0589310512847072,
-43.7427738125955));
#34853=CARTESIAN_POINT('Ctrl Pts',(17.0215749943808,-0.0675708651721102,
-44.5035932800172));
#34854=CARTESIAN_POINT('Ctrl Pts',(17.0230941742369,-0.0703394841680138,
-45.1492707441048));
#34855=CARTESIAN_POINT('Ctrl Pts',(17.0244855042361,-0.0670859480560476,
-45.6728939699293));
#34856=CARTESIAN_POINT('Ctrl Pts',(17.0255376111403,-0.0611357074905208,
-46.0689460167095));
#34857=CARTESIAN_POINT('Ctrl Pts',(17.0265051171325,-0.050916701376646,
-46.4683351154574));
#34858=CARTESIAN_POINT('Ctrl Pts',(17.0275494830201,-0.0305908520694293,
-47.0051754871332));
#34859=CARTESIAN_POINT('Ctrl Pts',(17.0279485298638,-0.00651356267870405,
-47.4125881784468));
#34860=CARTESIAN_POINT('Ctrl Pts',(17.027871025413,0.0250247472743915,-47.823537087381));
#34861=CARTESIAN_POINT('Ctrl Pts',(17.0279445204245,0.0453507766221093,
-48.0785047352768));
#34862=CARTESIAN_POINT('Ctrl Pts',(17.0284901041219,0.0901937661096688,
-48.6012889715114));
#34863=CARTESIAN_POINT('Ctrl Pts',(17.0302587584616,0.177593175442441,-49.5132589892957));
#34864=CARTESIAN_POINT('Ctrl Pts',(17.0337291862979,0.33360895778891,-50.8277687101996));
#34865=CARTESIAN_POINT('Ctrl Pts',(17.0351310915789,0.582883041778303,-52.4149695324514));
#34866=CARTESIAN_POINT('Ctrl Pts',(17.0318463451629,0.80031213472367,-53.4799784868388));
#34867=CARTESIAN_POINT('Ctrl Pts',(17.0277490187653,0.955439440182285,-54.1483596116179));
#34868=CARTESIAN_POINT('Ctrl Pts',(17.0258424488058,1.01918280988269,-54.4157872537986));
#34869=CARTESIAN_POINT('Ctrl Pts',(17.0211461857495,1.15344357491875,-54.951209548359));
#34870=CARTESIAN_POINT('Ctrl Pts',(17.0109087247023,1.40479153071745,-55.8853439606409));
#34871=CARTESIAN_POINT('Ctrl Pts',(16.984753882311,1.97014456173065,-57.7437500515642));
#34872=CARTESIAN_POINT('Ctrl Pts',(16.9606180598848,2.5494463143456,-59.3108745233488));
#34873=CARTESIAN_POINT('Ctrl Pts',(16.950361723684,2.9949772413804,-60.4057342821153));
#34874=CARTESIAN_POINT('Ctrl Pts',(16.9491073046583,3.05259874766688,-60.5455884776621));
#34875=CARTESIAN_POINT('Ctrl Pts',(16.9466853619297,3.16838014856612,-60.8200491397828));
#34876=CARTESIAN_POINT('Ctrl Pts',(16.942620918488,3.37717852163246,-61.299217702888));
#34877=CARTESIAN_POINT('Ctrl Pts',(16.9352294511537,3.81272231434839,-62.2434288889346));
#34878=CARTESIAN_POINT('Ctrl Pts',(16.9283406644973,4.34066707435569,-63.2954579139722));
#34879=CARTESIAN_POINT('Ctrl Pts',(16.9228040541019,4.87398964320674,-64.3178341147752));
#34880=CARTESIAN_POINT('Ctrl Pts',(16.920141194956,5.17167860343828,-64.8814124517947));
#34881=CARTESIAN_POINT('Ctrl Pts',(16.9185301080169,5.36729007332549,-65.2519469242985));
#34882=CARTESIAN_POINT('Ctrl Pts',(16.9175003525531,5.49682016376608,-65.4975540875435));
#34883=CARTESIAN_POINT('Ctrl Pts',(16.9165269998,5.62485777415317,-65.7410500677168));
#34884=CARTESIAN_POINT('Ctrl Pts',(16.9157288893456,5.73524940179998,-65.9521145711583));
#34885=CARTESIAN_POINT('Ctrl Pts',(16.9152866444826,5.79781536441384,-66.0721439981323));
#34886=CARTESIAN_POINT('Ctrl Pts',(16.9146373118575,5.89113377149035,-66.2516144809089));
#34887=CARTESIAN_POINT('Ctrl Pts',(16.9141213623647,5.96771782117635,-66.3999258533314));
#34888=CARTESIAN_POINT('Ctrl Pts',(16.9133049693211,6.09288052949987,-66.6440651452324));
#34889=CARTESIAN_POINT('Ctrl Pts',(16.9125662700127,6.23002422703788,-66.9103980955905));
#34890=CARTESIAN_POINT('Ctrl Pts',(16.9114683668413,6.49963646627558,-67.4296844202676));
#34891=CARTESIAN_POINT('Ctrl Pts',(16.9104262500859,6.97294614154424,-68.3314056845011));
#34892=CARTESIAN_POINT('Ctrl Pts',(16.9110520933701,7.91390854629592,-70.0932822293166));
#34893=CARTESIAN_POINT('Ctrl Pts',(16.9134073097484,8.71293266517356,-71.5688689618016));
#34894=CARTESIAN_POINT('Ctrl Pts',(16.9133674206332,9.30682319629896,-72.6859786116366));
#34895=CARTESIAN_POINT('Ctrl Pts',(16.9133622712192,9.44069244288629,-72.9377707805658));
#34896=CARTESIAN_POINT('Ctrl Pts',(16.9133536603917,9.70745196172853,-73.4395069259972));
#34897=CARTESIAN_POINT('Ctrl Pts',(16.9133456322856,10.0411163676074,-74.0670749356618));
#34898=CARTESIAN_POINT('Ctrl Pts',(16.9133436988121,10.4410973824441,-74.8193396278468));
#34899=CARTESIAN_POINT('Ctrl Pts',(16.9133478951202,11.2408916722415,-76.3235221726316));
#34900=CARTESIAN_POINT('Ctrl Pts',(16.913352509992,11.9070907868733,-77.5764604690554));
#34901=CARTESIAN_POINT('Ctrl Pts',(16.9133463396528,12.876981812635,-79.4005947887978));
#34902=CARTESIAN_POINT('Ctrl Pts',(16.9133431703429,13.3135497833338,-80.2216775335791));
#34903=CARTESIAN_POINT('Ctrl Pts',(16.9133431703429,13.7500713707233,-81.0426552356776));
#34904=CARTESIAN_POINT('Ctrl Pts',(19.7346230857497,-0.000642953111401741,
24.8306355395365));
#34905=CARTESIAN_POINT('Ctrl Pts',(19.7346821167419,-0.000642934736490794,
24.781756252557));
#34906=CARTESIAN_POINT('Ctrl Pts',(19.7347440260616,-0.000642913768523213,
24.7328780189341));
#34907=CARTESIAN_POINT('Ctrl Pts',(19.7354751641474,-0.000642741727641322,
24.1822702714333));
#34908=CARTESIAN_POINT('Ctrl Pts',(19.7360360872234,-0.000643517082627163,
23.1781357609119));
#34909=CARTESIAN_POINT('Ctrl Pts',(19.7373409930261,-0.000644592940470209,
21.169537608259));
#34910=CARTESIAN_POINT('Ctrl Pts',(19.7422073080115,-0.000644228994501214,
19.6653856082875));
#34911=CARTESIAN_POINT('Ctrl Pts',(19.7525254976372,-0.000639085395243651,
18.4143370820647));
#34912=CARTESIAN_POINT('Ctrl Pts',(19.7574741046864,-0.000636573362535956,
17.9115221213179));
#34913=CARTESIAN_POINT('Ctrl Pts',(19.7699008328156,-0.000630633018027315,
16.9075337937884));
#34914=CARTESIAN_POINT('Ctrl Pts',(19.79655504348,-0.000617266269918687,
15.1537233398426));
#34915=CARTESIAN_POINT('Ctrl Pts',(19.821875349484,-0.000605020852467982,
13.6519770448393));
#34916=CARTESIAN_POINT('Ctrl Pts',(19.8377436350961,-0.000592969546270982,
12.3974956126268));
#34917=CARTESIAN_POINT('Ctrl Pts',(19.8442301715107,-0.000587175138563672,
11.8965382478349));
#34918=CARTESIAN_POINT('Ctrl Pts',(19.8574528580582,-0.000574554883993074,
10.8946893215832));
#34919=CARTESIAN_POINT('Ctrl Pts',(19.8803358682593,-0.00054875605103042,
9.14114851187957));
#34920=CARTESIAN_POINT('Ctrl Pts',(19.8963889971374,-0.000536768765242916,
7.63592840905772));
#34921=CARTESIAN_POINT('Ctrl Pts',(19.9035179481799,-0.000530587930652473,
6.50502163852959));
#34922=CARTESIAN_POINT('Ctrl Pts',(19.9049801590683,-0.000553432928634556,
6.25511760243307));
#34923=CARTESIAN_POINT('Ctrl Pts',(19.9074770795704,-0.000679949177192419,
5.75435183526716));
#34924=CARTESIAN_POINT('Ctrl Pts',(19.9107964265407,-0.00106714628387842,
4.87638767184662));
#34925=CARTESIAN_POINT('Ctrl Pts',(19.9138001065816,-0.00209765951886981,
3.11587427664056));
#34926=CARTESIAN_POINT('Ctrl Pts',(19.9121023976492,-0.00212305173409241,
1.60724231122929));
#34927=CARTESIAN_POINT('Ctrl Pts',(19.9107191795177,-0.000458589584695931,
0.545455546299319));
#34928=CARTESIAN_POINT('Ctrl Pts',(19.910536721583,-0.000240879410105755,
0.418856935719241));
#34929=CARTESIAN_POINT('Ctrl Pts',(19.9101056334482,0.000263531734119996,
0.165994698487929));
#34930=CARTESIAN_POINT('Ctrl Pts',(19.9091827300556,0.00131805171169694,
-0.275935387072352));
#34931=CARTESIAN_POINT('Ctrl Pts',(19.9074245102459,0.00323972576446598,
-0.905606226749042));
#34932=CARTESIAN_POINT('Ctrl Pts',(19.9047108946236,0.00602030268412137,
-1.65908800201351));
#34933=CARTESIAN_POINT('Ctrl Pts',(19.9004523608938,0.01002517504186,-2.66149121249902));
#34934=CARTESIAN_POINT('Ctrl Pts',(19.8941653858529,0.0150642551577006,
-3.91142926653451));
#34935=CARTESIAN_POINT('Ctrl Pts',(19.8888148939253,0.0178887851550629,
-4.91030040063366));
#34936=CARTESIAN_POINT('Ctrl Pts',(19.8856001260017,0.0189503528382262,
-5.53506672615536));
#34937=CARTESIAN_POINT('Ctrl Pts',(19.8842625781479,0.019331232340815,-5.78557007654373));
#34938=CARTESIAN_POINT('Ctrl Pts',(19.881420005471,0.0199225557911846,-6.28673777410555));
#34939=CARTESIAN_POINT('Ctrl Pts',(19.8760732500074,0.020557544334544,-7.16470056012135));
#34940=CARTESIAN_POINT('Ctrl Pts',(19.86775437564,0.0205928311815489,-8.42014679737612));
#34941=CARTESIAN_POINT('Ctrl Pts',(19.8595226870973,0.0201745887778942,
-9.67457783212885));
#34942=CARTESIAN_POINT('Ctrl Pts',(19.8543205682205,0.0200185830632958,
-10.5506646481595));
#34943=CARTESIAN_POINT('Ctrl Pts',(19.8515839106785,0.0200193520216717,
-11.0505094359074));
#34944=CARTESIAN_POINT('Ctrl Pts',(19.8503064139383,0.020058521840743,-11.3001384889717));
#34945=CARTESIAN_POINT('Ctrl Pts',(19.8493831115964,0.02010609406382,-11.4880183077322));
#34946=CARTESIAN_POINT('Ctrl Pts',(19.848759579533,0.0201389662794458,-11.6141131856583));
#34947=CARTESIAN_POINT('Ctrl Pts',(19.8475035865337,0.0202088783303024,
-11.8660900631704));
#34948=CARTESIAN_POINT('Ctrl Pts',(19.8452901371666,0.0203402429399956,
-12.3063138185554));
#34949=CARTESIAN_POINT('Ctrl Pts',(19.8395963739657,0.0207155104692084,
-13.4352543682579));
#34950=CARTESIAN_POINT('Ctrl Pts',(19.8337233195694,0.0211892187478554,
-14.6834171900175));
#34951=CARTESIAN_POINT('Ctrl Pts',(19.8296973929213,0.021535321909794,-15.9343304218055));
#34952=CARTESIAN_POINT('Ctrl Pts',(19.828262623613,0.0216592588011182,-16.5612150515869));
#34953=CARTESIAN_POINT('Ctrl Pts',(19.827532909389,0.021717998410105,-17.0640315108058));
#34954=CARTESIAN_POINT('Ctrl Pts',(19.8273188497013,0.0217327140511073,
-17.3159473892265));
#34955=CARTESIAN_POINT('Ctrl Pts',(19.8272197499129,0.0217373640412579,
-17.5043252928702));
#34956=CARTESIAN_POINT('Ctrl Pts',(19.8271645940149,0.021743742715054,-17.6290672580878));
#34957=CARTESIAN_POINT('Ctrl Pts',(19.8270963895439,0.0217716370272419,
-17.8785042386958));
#34958=CARTESIAN_POINT('Ctrl Pts',(19.8270927400091,0.0218191141612584,
-18.1280752129324));
#34959=CARTESIAN_POINT('Ctrl Pts',(19.8271554676397,0.0218804577107381,
-18.3777251690563));
#34960=CARTESIAN_POINT('Ctrl Pts',(19.82722294071,0.0219235473964778,-18.5338030361248));
#34961=CARTESIAN_POINT('Ctrl Pts',(19.8272940849153,0.021960136806743,-18.658689553547));
#34962=CARTESIAN_POINT('Ctrl Pts',(19.8273765552953,0.021998026722338,-18.7835940973741));
#34963=CARTESIAN_POINT('Ctrl Pts',(19.8276539168662,0.0221052563178028,
-19.1271513721223));
#34964=CARTESIAN_POINT('Ctrl Pts',(19.8283688675522,0.0222941765936138,
-19.689739383064));
#34965=CARTESIAN_POINT('Ctrl Pts',(19.8304691154989,0.0225287937954849,
-20.6911098412784));
#34966=CARTESIAN_POINT('Ctrl Pts',(19.8346284038769,0.0224225988438274,
-21.9452964756393));
#34967=CARTESIAN_POINT('Ctrl Pts',(19.8398820955914,0.0213428595161395,
-22.9516036161008));
#34968=CARTESIAN_POINT('Ctrl Pts',(19.8437546466324,0.0202230855359422,
-23.5798476343222));
#34969=CARTESIAN_POINT('Ctrl Pts',(19.84542658254,0.0197138857317108,-23.8282650337369));
#34970=CARTESIAN_POINT('Ctrl Pts',(19.8492992870015,0.0184781981973547,
-24.3262507423293));
#34971=CARTESIAN_POINT('Ctrl Pts',(19.857267766854,0.015824936416586,-25.1999679111835));
#34972=CARTESIAN_POINT('Ctrl Pts',(19.8711374113828,0.0111859737214354,
-26.4535682981818));
#34973=CARTESIAN_POINT('Ctrl Pts',(19.8882621349692,0.00576243781980644,
-27.9627331221817));
#34974=CARTESIAN_POINT('Ctrl Pts',(19.8978645033397,0.00308643285001822,
-28.9694055740695));
#34975=CARTESIAN_POINT('Ctrl Pts',(19.9020476452313,0.00202842531119992,
-29.5351389851221));
#34976=CARTESIAN_POINT('Ctrl Pts',(19.9029598655213,0.00179395500155851,
-29.660711242041));
#34977=CARTESIAN_POINT('Ctrl Pts',(19.9047368949606,0.00136864071316774,
-29.9119673822201));
#34978=CARTESIAN_POINT('Ctrl Pts',(19.9077264104863,0.00071936380440862,
-30.3516893036152));
#34979=CARTESIAN_POINT('Ctrl Pts',(19.9132380639417,-0.000244003107841386,
-31.2313376651581));
#34980=CARTESIAN_POINT('Ctrl Pts',(19.9185788054482,-0.000796108407126999,
-32.2363666896278));
#34981=CARTESIAN_POINT('Ctrl Pts',(19.9231699515195,-0.00130293714163212,
-33.2400982545545));
#34982=CARTESIAN_POINT('Ctrl Pts',(19.926287582346,-0.00178506957046058,
-33.9919628075564));
#34983=CARTESIAN_POINT('Ctrl Pts',(19.9291537330895,-0.00247603470082823,
-34.7425267762971));
#34984=CARTESIAN_POINT('Ctrl Pts',(19.930921520269,-0.00316109123277813,
-35.2418837084394));
#34985=CARTESIAN_POINT('Ctrl Pts',(19.932212815312,-0.00379711533894955,
-35.6169656511168));
#34986=CARTESIAN_POINT('Ctrl Pts',(19.9331201298407,-0.00430080901852659,
-35.8676312652858));
#34987=CARTESIAN_POINT('Ctrl Pts',(19.9350542554739,-0.00559418401298511,
-36.3690027760414));
#34988=CARTESIAN_POINT('Ctrl Pts',(19.9385694048054,-0.00841243403087586,
-37.2453622153362));
#34989=CARTESIAN_POINT('Ctrl Pts',(19.9450600062419,-0.0153862358953072,
-38.9978150636203));
#34990=CARTESIAN_POINT('Ctrl Pts',(19.9457014876814,-0.0193132523885131,
-40.50342730423));
#34991=CARTESIAN_POINT('Ctrl Pts',(19.9405912460554,-0.0175424815871379,
-41.6396344433984));
#34992=CARTESIAN_POINT('Ctrl Pts',(19.939417941721,-0.0180609024665847,
-41.8773427901699));
#34993=CARTESIAN_POINT('Ctrl Pts',(19.9374487737961,-0.0209480616663699,
-42.2441269452064));
#34994=CARTESIAN_POINT('Ctrl Pts',(19.9352664823961,-0.0254730253434529,
-42.611783774443));
#34995=CARTESIAN_POINT('Ctrl Pts',(19.9320404046982,-0.0329960094720893,
-43.1076484405979));
#34996=CARTESIAN_POINT('Ctrl Pts',(19.9273834522402,-0.0438998692360093,
-43.7349078281428));
#34997=CARTESIAN_POINT('Ctrl Pts',(19.920645793495,-0.0550409518824901,
-44.5001571844784));
#34998=CARTESIAN_POINT('Ctrl Pts',(19.9139481025105,-0.058917689892779,
-45.1474411022027));
#34999=CARTESIAN_POINT('Ctrl Pts',(19.9079109430792,-0.0563763703496538,
-45.6711601971578));
#35000=CARTESIAN_POINT('Ctrl Pts',(19.9030063055532,-0.0510379740403673,
-46.0666739926564));
#35001=CARTESIAN_POINT('Ctrl Pts',(19.8977111471374,-0.041636222220782,
-46.4649218026843));
#35002=CARTESIAN_POINT('Ctrl Pts',(19.8901265591865,-0.0228219799811086,
-46.9994538907081));
#35003=CARTESIAN_POINT('Ctrl Pts',(19.8837762659454,-0.00066810850759029,
-47.4042332401222));
#35004=CARTESIAN_POINT('Ctrl Pts',(19.877004516628,0.0282497019994057,-47.8120475821032));
#35005=CARTESIAN_POINT('Ctrl Pts',(19.8720730452078,0.0469490572617378,
-48.0669242890347));
#35006=CARTESIAN_POINT('Ctrl Pts',(19.8608461763039,0.0882600632253731,
-48.5886303230491));
#35007=CARTESIAN_POINT('Ctrl Pts',(19.8381971947123,0.169269250258146,-49.4998005116595));
#35008=CARTESIAN_POINT('Ctrl Pts',(19.8005116026619,0.316415072387404,-50.8144923814608));
#35009=CARTESIAN_POINT('Ctrl Pts',(19.7571232499412,0.558733185701103,-52.4044613455247));
#35010=CARTESIAN_POINT('Ctrl Pts',(19.7354326536812,0.774332347196781,-53.4727165621296));
#35011=CARTESIAN_POINT('Ctrl Pts',(19.7259938964815,0.929292946652962,-54.1436236906726));
#35012=CARTESIAN_POINT('Ctrl Pts',(19.722378034875,0.993021295346837,-54.4118453951711));
#35013=CARTESIAN_POINT('Ctrl Pts',(19.7158892867674,1.1275509880106,-54.9488036427376));
#35014=CARTESIAN_POINT('Ctrl Pts',(19.7063490604149,1.37998863274845,-55.8852205667512));
#35015=CARTESIAN_POINT('Ctrl Pts',(19.6938101649099,1.94940883769124,-57.7468499435128));
#35016=CARTESIAN_POINT('Ctrl Pts',(19.6917179920513,2.53343609922751,-59.3144488274368));
#35017=CARTESIAN_POINT('Ctrl Pts',(19.6921472074124,2.98058714663305,-60.408320468436));
#35018=CARTESIAN_POINT('Ctrl Pts',(19.6923302411128,3.03855380157463,-60.5484454487465));
#35019=CARTESIAN_POINT('Ctrl Pts',(19.6928896930775,3.15496837800988,-60.8232006982505));
#35020=CARTESIAN_POINT('Ctrl Pts',(19.6944621969898,3.36498448187706,-61.3029405460856));
#35021=CARTESIAN_POINT('Ctrl Pts',(19.699547978084,3.80312264363572,-62.2479633131678));
#35022=CARTESIAN_POINT('Ctrl Pts',(19.708472488342,4.33433639755622,-63.3003758582488));
#35023=CARTESIAN_POINT('Ctrl Pts',(19.7178062533734,4.87058092910209,-64.3225010121906));
#35024=CARTESIAN_POINT('Ctrl Pts',(19.7227363601189,5.16968125139723,-64.8857202902664));
#35025=CARTESIAN_POINT('Ctrl Pts',(19.7256892775882,5.3660993240338,-65.2559282740194));
#35026=CARTESIAN_POINT('Ctrl Pts',(19.7275529269646,5.4961236312018,-65.5012946526292));
#35027=CARTESIAN_POINT('Ctrl Pts',(19.7292494930669,5.62460530306604,-65.7445154007033));
#35028=CARTESIAN_POINT('Ctrl Pts',(19.7305409820397,5.73531536293809,-65.9553101543504));
#35029=CARTESIAN_POINT('Ctrl Pts',(19.7312200009703,5.79804464979269,-66.0751771047758));
#35030=CARTESIAN_POINT('Ctrl Pts',(19.7321763080164,5.89158788007909,-66.2543957286631));
#35031=CARTESIAN_POINT('Ctrl Pts',(19.7328433165431,5.96832407956894,-66.402477667768));
#35032=CARTESIAN_POINT('Ctrl Pts',(19.7337361677523,6.09367212132328,-66.64621744546));
#35033=CARTESIAN_POINT('Ctrl Pts',(19.7345472830898,6.23102804903925,-66.9122358782964));
#35034=CARTESIAN_POINT('Ctrl Pts',(19.7357637525657,6.50088493107782,-67.4309132821684));
#35035=CARTESIAN_POINT('Ctrl Pts',(19.73696023581,6.97433195159225,-68.3317564250992));
#35036=CARTESIAN_POINT('Ctrl Pts',(19.7364841334505,7.91461052110222,-70.0925538466961));
#35037=CARTESIAN_POINT('Ctrl Pts',(19.7341525791219,8.71285882012307,-71.568314545697));
#35038=CARTESIAN_POINT('Ctrl Pts',(19.7342536478909,9.30719870643568,-72.6861159988526));
#35039=CARTESIAN_POINT('Ctrl Pts',(19.7342693216236,9.4410471924085,-72.9378486651355));
#35040=CARTESIAN_POINT('Ctrl Pts',(19.734294087738,9.70782792197631,-73.4395913415074));
#35041=CARTESIAN_POINT('Ctrl Pts',(19.73431380359,10.0414888140811,-74.0671184098798));
#35042=CARTESIAN_POINT('Ctrl Pts',(19.7343174844631,10.4414675358527,-74.8193699085516));
#35043=CARTESIAN_POINT('Ctrl Pts',(19.7343007359239,11.241238470148,-76.3235214394896));
#35044=CARTESIAN_POINT('Ctrl Pts',(19.7342702208829,11.9074313046534,-77.5764535976686));
#35045=CARTESIAN_POINT('Ctrl Pts',(19.7342790380661,12.8773505355511,-79.4006103950861));
#35046=CARTESIAN_POINT('Ctrl Pts',(19.7342835685967,13.3139183378821,-80.221677090073));
#35047=CARTESIAN_POINT('Ctrl Pts',(19.7342835685968,13.7504399252715,-81.0426547921714));
#35048=CARTESIAN_POINT('Ctrl Pts',(22.5540683561216,0.00218147413889375,
24.8306318837938));
#35049=CARTESIAN_POINT('Ctrl Pts',(22.554135708553,0.0021816069582444,24.781752480719));
#35050=CARTESIAN_POINT('Ctrl Pts',(22.5542063449766,0.00218174482895129,
24.7328741280427));
#35051=CARTESIAN_POINT('Ctrl Pts',(22.5550405516681,0.00218343279774944,
24.1822650476588));
#35052=CARTESIAN_POINT('Ctrl Pts',(22.5556808204131,0.00218653523452655,
23.1781290012419));
#35053=CARTESIAN_POINT('Ctrl Pts',(22.5571704372049,0.00219387923828822,
21.1695284782211));
#35054=CARTESIAN_POINT('Ctrl Pts',(22.5627227814794,0.00220569836013384,
19.6653768549175));
#35055=CARTESIAN_POINT('Ctrl Pts',(22.5744942562184,0.00222185508179394,
18.4143286693318));
#35056=CARTESIAN_POINT('Ctrl Pts',(22.5801396960068,0.00223007976877095,
17.9115066393623));
#35057=CARTESIAN_POINT('Ctrl Pts',(22.5943159820712,0.00225185213321563,
16.9075134210456));
#35058=CARTESIAN_POINT('Ctrl Pts',(22.6247225788558,0.00229799248967236,
15.153703473283));
#35059=CARTESIAN_POINT('Ctrl Pts',(22.6536089727913,0.00233443368688111,
13.6519813201694));
#35060=CARTESIAN_POINT('Ctrl Pts',(22.6717145277981,0.00234043481082431,
12.3975308629626));
#35061=CARTESIAN_POINT('Ctrl Pts',(22.679115594771,0.00234074687208769,
11.8965860813863));
#35062=CARTESIAN_POINT('Ctrl Pts',(22.6942029354826,0.00233563010780471,
10.8947553295711));
#35063=CARTESIAN_POINT('Ctrl Pts',(22.7203138747303,0.00231381924858082,
9.14123354533352));
#35064=CARTESIAN_POINT('Ctrl Pts',(22.7386363554764,0.00228962747677265,
7.63600350836706));
#35065=CARTESIAN_POINT('Ctrl Pts',(22.7467772039179,0.00227689513963197,
6.5050900642413));
#35066=CARTESIAN_POINT('Ctrl Pts',(22.7485221996124,0.00223748350450178,
6.25533927343516));
#35067=CARTESIAN_POINT('Ctrl Pts',(22.7517687074826,0.00204041652177819,
5.75473880201197));
#35068=CARTESIAN_POINT('Ctrl Pts',(22.756746021602,0.00145805657110865,
4.87698664852411));
#35069=CARTESIAN_POINT('Ctrl Pts',(22.7633409013492,-9.50353224288473E-5,
3.11633965161738));
#35070=CARTESIAN_POINT('Ctrl Pts',(22.7614298458992,-0.000101851369145884,
1.60673369886307));
#35071=CARTESIAN_POINT('Ctrl Pts',(22.754755687708,0.00237657533938654,
0.543821997324392));
#35072=CARTESIAN_POINT('Ctrl Pts',(22.7538849752791,0.00269824982403687,
0.417040370789071));
#35073=CARTESIAN_POINT('Ctrl Pts',(22.7518618090786,0.00344090667788074,
0.163862775610429));
#35074=CARTESIAN_POINT('Ctrl Pts',(22.7476225754754,0.00498369006181879,
-0.278579310015945));
#35075=CARTESIAN_POINT('Ctrl Pts',(22.7398195734886,0.00778723782990159,
-0.908804588765807));
#35076=CARTESIAN_POINT('Ctrl Pts',(22.7284275590651,0.0117866394648969,
-1.6626456912705));
#35077=CARTESIAN_POINT('Ctrl Pts',(22.7115977999302,0.0175719377185294,
-2.66510680565334));
#35078=CARTESIAN_POINT('Ctrl Pts',(22.6894237529051,0.0248789730569118,
-3.91437002671321));
#35079=CARTESIAN_POINT('Ctrl Pts',(22.6746279323472,0.0292114700920186,
-4.91228617641643));
#35080=CARTESIAN_POINT('Ctrl Pts',(22.6675562993878,0.0309313882324642,
-5.5364254127196));
#35081=CARTESIAN_POINT('Ctrl Pts',(22.6647896390813,0.0315766094374004,
-5.78702766260291));
#35082=CARTESIAN_POINT('Ctrl Pts',(22.6594992216835,0.0327005225668863,
-6.28815877217012));
#35083=CARTESIAN_POINT('Ctrl Pts',(22.6508460117802,0.0342590482256434,
-7.16606874547671));
#35084=CARTESIAN_POINT('Ctrl Pts',(22.6400133172493,0.0354626555877318,
-8.42107398284687));
#35085=CARTESIAN_POINT('Ctrl Pts',(22.6307092367043,0.0357005865857655,
-9.67465683280276));
#35086=CARTESIAN_POINT('Ctrl Pts',(22.6247301929899,0.0355672907810145,
-10.5498966593995));
#35087=CARTESIAN_POINT('Ctrl Pts',(22.6214297571352,0.0354360409498412,
-11.0491879677433));
#35088=CARTESIAN_POINT('Ctrl Pts',(22.6198116453495,0.0353568730948748,
-11.2985176495465));
#35089=CARTESIAN_POINT('Ctrl Pts',(22.6186028341508,0.0352940820780271,
-11.4861565312266));
#35090=CARTESIAN_POINT('Ctrl Pts',(22.6177874524816,0.0352378259324908,
-11.611867847455));
#35091=CARTESIAN_POINT('Ctrl Pts',(22.6161496709671,0.035072157733957,-11.8632532885014));
#35092=CARTESIAN_POINT('Ctrl Pts',(22.6132752194428,0.0346523606763489,
-12.3024953421541));
#35093=CARTESIAN_POINT('Ctrl Pts',(22.6059441579138,0.0330017977772016,
-13.4295791077051));
#35094=CARTESIAN_POINT('Ctrl Pts',(22.598602354385,0.030057379385193,-14.677520602664));
#35095=CARTESIAN_POINT('Ctrl Pts',(22.5939390070843,0.0277608272128385,
-15.9301343469425));
#35096=CARTESIAN_POINT('Ctrl Pts',(22.592426221169,0.0269196020107557,-16.5583233401281));
#35097=CARTESIAN_POINT('Ctrl Pts',(22.5918052172197,0.0265202899207708,
-17.0624557535612));
#35098=CARTESIAN_POINT('Ctrl Pts',(22.591704598448,0.026425712580917,-17.3151272795674));
#35099=CARTESIAN_POINT('Ctrl Pts',(22.5917144447763,0.0264002013132958,
-17.5040742508018));
#35100=CARTESIAN_POINT('Ctrl Pts',(22.5917487630321,0.0263702963468637,
-17.6282069779701));
#35101=CARTESIAN_POINT('Ctrl Pts',(22.5919252031847,0.0262575873912922,
-17.8771189025034));
#35102=CARTESIAN_POINT('Ctrl Pts',(22.5922557762722,0.0260765632870242,
-18.1261007585217));
#35103=CARTESIAN_POINT('Ctrl Pts',(22.5927310220947,0.0258508062393998,
-18.3754317061234));
#35104=CARTESIAN_POINT('Ctrl Pts',(22.5930852523955,0.0256949150880551,
-18.5313488908643));
#35105=CARTESIAN_POINT('Ctrl Pts',(22.5934018269883,0.0255643923002756,
-18.6561552304994));
#35106=CARTESIAN_POINT('Ctrl Pts',(22.5937398083511,0.0254310783739573,
-18.7810025555363));
#35107=CARTESIAN_POINT('Ctrl Pts',(22.5947569696741,0.0250516744836173,
-19.1245123719922));
#35108=CARTESIAN_POINT('Ctrl Pts',(22.5968697909726,0.0244272748524223,
-19.6876037237825));
#35109=CARTESIAN_POINT('Ctrl Pts',(22.6016928063477,0.023736309273104,-20.6915355013246));
#35110=CARTESIAN_POINT('Ctrl Pts',(22.6092220907402,0.0246838664602423,
-21.9520496006516));
#35111=CARTESIAN_POINT('Ctrl Pts',(22.6159651125159,0.0292734278575275,
-22.966722303222));
#35112=CARTESIAN_POINT('Ctrl Pts',(22.6200050894728,0.0340288155052018,
-23.6012568386363));
#35113=CARTESIAN_POINT('Ctrl Pts',(22.6216960539806,0.0361924278746453,
-23.8534746245936));
#35114=CARTESIAN_POINT('Ctrl Pts',(22.6254141445623,0.0414336069590376,
-24.3573247228981));
#35115=CARTESIAN_POINT('Ctrl Pts',(22.6326435229306,0.0527088136412557,
-25.2394652019242));
#35116=CARTESIAN_POINT('Ctrl Pts',(22.6443106503046,0.0727322552410105,
-26.4984118526265));
#35117=CARTESIAN_POINT('Ctrl Pts',(22.6577636488587,0.0972434087164042,
-28.0039143274124));
#35118=CARTESIAN_POINT('Ctrl Pts',(22.6648986224874,0.109910840772038,-29.0011715067303));
#35119=CARTESIAN_POINT('Ctrl Pts',(22.667906150243,0.115058735797627,-29.5597546137854));
#35120=CARTESIAN_POINT('Ctrl Pts',(22.6685373980379,0.116221209894467,-29.6853423185855));
#35121=CARTESIAN_POINT('Ctrl Pts',(22.6696760198942,0.118507809722523,-29.935698806095));
#35122=CARTESIAN_POINT('Ctrl Pts',(22.6713694335329,0.12242392958844,-30.3742436235447));
#35123=CARTESIAN_POINT('Ctrl Pts',(22.6737257579926,0.129834840657116,-31.2509365971211));
#35124=CARTESIAN_POINT('Ctrl Pts',(22.6749011413929,0.136936610672894,-32.2522134124557));
#35125=CARTESIAN_POINT('Ctrl Pts',(22.6761981716237,0.141970330127987,-33.2514988088751));
#35126=CARTESIAN_POINT('Ctrl Pts',(22.6776431338712,0.144534674572906,-33.9997484962132));
#35127=CARTESIAN_POINT('Ctrl Pts',(22.6800043956835,0.145645822770892,-34.7463847821545));
#35128=CARTESIAN_POINT('Ctrl Pts',(22.6824604269127,0.145311856209713,-35.2429076455261));
#35129=CARTESIAN_POINT('Ctrl Pts',(22.6847454964563,0.144612206113386,-35.6157555666383));
#35130=CARTESIAN_POINT('Ctrl Pts',(22.6865345137926,0.143935748993521,-35.8647138062475));
#35131=CARTESIAN_POINT('Ctrl Pts',(22.6909948954712,0.141825139239321,-36.3629355945598));
#35132=CARTESIAN_POINT('Ctrl Pts',(22.7007211017334,0.136319998449124,-37.2340753087831));
#35133=CARTESIAN_POINT('Ctrl Pts',(22.7247187730148,0.11964407152272,-38.9777466279288));
#35134=CARTESIAN_POINT('Ctrl Pts',(22.7420439175246,0.100879259671926,-40.4797501482002));
#35135=CARTESIAN_POINT('Ctrl Pts',(22.742174398847,0.0900117196293994,-41.6152353076556));
#35136=CARTESIAN_POINT('Ctrl Pts',(22.7419947456864,0.0868629477186161,
-41.8530396771713));
#35137=CARTESIAN_POINT('Ctrl Pts',(22.7411588868783,0.0798734920793458,
-42.2195939742537));
#35138=CARTESIAN_POINT('Ctrl Pts',(22.7397815779615,0.0711701094471297,
-42.586859208967));
#35139=CARTESIAN_POINT('Ctrl Pts',(22.737263822772,0.0578805058533532,-43.081875181358));
#35140=CARTESIAN_POINT('Ctrl Pts',(22.7329120829938,0.0393414645107835,
-43.7075346067066));
#35141=CARTESIAN_POINT('Ctrl Pts',(22.7259867352306,0.0180490019609267,
-44.4699595380308));
#35142=CARTESIAN_POINT('Ctrl Pts',(22.7189754097439,0.00461976903386266,
-45.1141309663419));
#35143=CARTESIAN_POINT('Ctrl Pts',(22.7127423271767,-0.00138856537622484,
-45.6349447941414));
#35144=CARTESIAN_POINT('Ctrl Pts',(22.7077745025803,-0.00293648720720613,
-46.0280483924158));
#35145=CARTESIAN_POINT('Ctrl Pts',(22.702539756329,-0.000952767527570727,
-46.4236679472298));
#35146=CARTESIAN_POINT('Ctrl Pts',(22.695248106512,0.00715860064351331,
-46.9544003416955));
#35147=CARTESIAN_POINT('Ctrl Pts',(22.6894368964206,0.0203671438046086,
-47.3560146155071));
#35148=CARTESIAN_POINT('Ctrl Pts',(22.6834694544482,0.039481350339373,-47.7603227791904));
#35149=CARTESIAN_POINT('Ctrl Pts',(22.6791422427141,0.0512307024465059,
-48.0075015017657));
#35150=CARTESIAN_POINT('Ctrl Pts',(22.6692324211024,0.0763142779141968,
-48.5191761118809));
#35151=CARTESIAN_POINT('Ctrl Pts',(22.6491107551827,0.124158552493288,-49.416497872572));
#35152=CARTESIAN_POINT('Ctrl Pts',(22.6148657729272,0.215268103806751,-50.7276117444274));
#35153=CARTESIAN_POINT('Ctrl Pts',(22.5746907034547,0.395225833157523,-52.3372310364046));
#35154=CARTESIAN_POINT('Ctrl Pts',(22.5555260121924,0.588228809792435,-53.4345630297578));
#35155=CARTESIAN_POINT('Ctrl Pts',(22.5480884581515,0.74030785136882,-54.1276488294856));
#35156=CARTESIAN_POINT('Ctrl Pts',(22.5452460751718,0.803140727604942,-54.4022021073488));
#35157=CARTESIAN_POINT('Ctrl Pts',(22.5404938550578,0.938793274403183,-54.9516189864557));
#35158=CARTESIAN_POINT('Ctrl Pts',(22.5341958029479,1.19920161828228,-55.9053975612708));
#35159=CARTESIAN_POINT('Ctrl Pts',(22.5281267758728,1.80275630578089,-57.7881154594452));
#35160=CARTESIAN_POINT('Ctrl Pts',(22.528583603618,2.42533038851665,-59.35130068497));
#35161=CARTESIAN_POINT('Ctrl Pts',(22.528532377079,2.88493160586583,-60.4337308314408));
#35162=CARTESIAN_POINT('Ctrl Pts',(22.5287259190148,2.94571920325708,-60.5750505472678));
#35163=CARTESIAN_POINT('Ctrl Pts',(22.5291677879915,3.06720147455161,-60.850552993609));
#35164=CARTESIAN_POINT('Ctrl Pts',(22.5303403340556,3.28675165509904,-61.3319382132006));
#35165=CARTESIAN_POINT('Ctrl Pts',(22.5338469167794,3.74449224051456,-62.2782340020111));
#35166=CARTESIAN_POINT('Ctrl Pts',(22.5397048431139,4.29830979361861,-63.3298919614451));
#35167=CARTESIAN_POINT('Ctrl Pts',(22.5457174570534,4.85400363670458,-64.3492239718143));
#35168=CARTESIAN_POINT('Ctrl Pts',(22.5488714298889,5.16234868040809,-64.9101497756193));
#35169=CARTESIAN_POINT('Ctrl Pts',(22.5507492352918,5.36397377145835,-65.2784630670283));
#35170=CARTESIAN_POINT('Ctrl Pts',(22.551931627265,5.49720250657446,-65.5224660380437));
#35171=CARTESIAN_POINT('Ctrl Pts',(22.5530001707,5.6284580866325,-65.7641630999649));
#35172=CARTESIAN_POINT('Ctrl Pts',(22.5538074203757,5.74118426524144,-65.9734681757563));
#35173=CARTESIAN_POINT('Ctrl Pts',(22.5542291325583,5.8049417377464,-66.0924361240013));
#35174=CARTESIAN_POINT('Ctrl Pts',(22.5548200729008,5.89990121284972,-66.2702572205141));
#35175=CARTESIAN_POINT('Ctrl Pts',(22.5552240851311,5.97754530004697,-66.4170687212062));
#35176=CARTESIAN_POINT('Ctrl Pts',(22.5557509286219,6.10401749845465,-66.6585493188342));
#35177=CARTESIAN_POINT('Ctrl Pts',(22.5562022351456,6.24252186488589,-66.922501445448));
#35178=CARTESIAN_POINT('Ctrl Pts',(22.5568282241031,6.51358133221557,-67.4373154524345));
#35179=CARTESIAN_POINT('Ctrl Pts',(22.5572574572638,6.98704795492337,-68.3324605421028));
#35180=CARTESIAN_POINT('Ctrl Pts',(22.5560808670878,7.92134723887345,-70.0860597307467));
#35181=CARTESIAN_POINT('Ctrl Pts',(22.5537908216693,8.71315752530691,-71.5635641333792));
#35182=CARTESIAN_POINT('Ctrl Pts',(22.5536221564192,9.3102139919392,-72.6864389144413));
#35183=CARTESIAN_POINT('Ctrl Pts',(22.5535880143634,9.44388849338344,-72.9378363622075));
#35184=CARTESIAN_POINT('Ctrl Pts',(22.5535378432735,9.71076529731538,-73.4397479822456));
#35185=CARTESIAN_POINT('Ctrl Pts',(22.5535059689553,10.0443610125397,-74.0671478108037));
#35186=CARTESIAN_POINT('Ctrl Pts',(22.5535030828491,10.444355436008,-74.8194294880936));
#35187=CARTESIAN_POINT('Ctrl Pts',(22.5535484575473,11.2440931997388,-76.3235325103929));
#35188=CARTESIAN_POINT('Ctrl Pts',(22.5536517783583,11.9102687075601,-77.5764681404427));
#35189=CARTESIAN_POINT('Ctrl Pts',(22.5536551658664,12.8801832338076,-79.4006231145849));
#35190=CARTESIAN_POINT('Ctrl Pts',(22.5536569200915,13.3167425765319,-80.2216775136107));
#35191=CARTESIAN_POINT('Ctrl Pts',(22.5536569200916,13.7532641639214,-81.0426552157089));
#35192=CARTESIAN_POINT('Ctrl Pts',(25.3681329014818,0.00175512325942154,
24.8306327114547));
#35193=CARTESIAN_POINT('Ctrl Pts',(25.3682084066264,0.00175506440139837,
24.7817533351788));
#35194=CARTESIAN_POINT('Ctrl Pts',(25.3682875944382,0.00175500320257746,
24.73287501414));
#35195=CARTESIAN_POINT('Ctrl Pts',(25.369222751594,0.00175425231120099,
24.1822661052121));
#35196=CARTESIAN_POINT('Ctrl Pts',(25.3699366350458,0.00175478425630212,
23.1781287518567));
#35197=CARTESIAN_POINT('Ctrl Pts',(25.3715957331742,0.00175722934477583,
21.1695289275335));
#35198=CARTESIAN_POINT('Ctrl Pts',(25.3778196824431,0.00175189404505957,
19.6653756524456));
#35199=CARTESIAN_POINT('Ctrl Pts',(25.3910342840048,0.00173499406283094,
18.4143272223797));
#35200=CARTESIAN_POINT('Ctrl Pts',(25.3973705443932,0.00172725455765711,
17.9115074792048));
#35201=CARTESIAN_POINT('Ctrl Pts',(25.4132791906795,0.00170817665878482,
16.9075149255972));
#35202=CARTESIAN_POINT('Ctrl Pts',(25.4474027842317,0.00166701913903138,
15.1537022583482));
#35203=CARTESIAN_POINT('Ctrl Pts',(25.4798405615858,0.00162111906728065,
13.6519650344697));
#35204=CARTESIAN_POINT('Ctrl Pts',(25.5002106904973,0.00158271977166255,
12.3975021657436));
#35205=CARTESIAN_POINT('Ctrl Pts',(25.5085421434162,0.00156602110601469,
11.8965526321469));
#35206=CARTESIAN_POINT('Ctrl Pts',(25.5255401762533,0.00152790014427616,
10.8947155709491));
#35207=CARTESIAN_POINT('Ctrl Pts',(25.5549874499801,0.00145470426919707,
9.14118230153193));
#35208=CARTESIAN_POINT('Ctrl Pts',(25.5756768333846,0.00139107439095266,
7.6359531409517));
#35209=CARTESIAN_POINT('Ctrl Pts',(25.5848715252591,0.00136281688660175,
6.50500245926613));
#35210=CARTESIAN_POINT('Ctrl Pts',(25.5868291161923,0.00135878771456196,
6.25475796638462));
#35211=CARTESIAN_POINT('Ctrl Pts',(25.5904255824825,0.00135700379304369,
5.75362379308219));
#35212=CARTESIAN_POINT('Ctrl Pts',(25.5958355797972,0.0013658411947461,
4.87519816783808));
#35213=CARTESIAN_POINT('Ctrl Pts',(25.6027324835524,0.00141374342985738,
3.11496398695253));
#35214=CARTESIAN_POINT('Ctrl Pts',(25.6006135930905,0.00139356100729972,
1.60842266632563));
#35215=CARTESIAN_POINT('Ctrl Pts',(25.5940653731096,0.00126840919376977,
0.549146222454319));
#35216=CARTESIAN_POINT('Ctrl Pts',(25.5932108642366,0.00125246996428166,
0.423005443203523));
#35217=CARTESIAN_POINT('Ctrl Pts',(25.5912223975216,0.0012154047501728,
0.170912548170089));
#35218=CARTESIAN_POINT('Ctrl Pts',(25.5870494140617,0.00113907015926919,
-0.269752289290245));
#35219=CARTESIAN_POINT('Ctrl Pts',(25.5793481002059,0.000999773781648224,
-0.898012224905597));
#35220=CARTESIAN_POINT('Ctrl Pts',(25.5680685042275,0.00081869072994828,
-1.65037512844969));
#35221=CARTESIAN_POINT('Ctrl Pts',(25.5513318271299,0.000564796045184066,
-2.65209276473023));
#35222=CARTESIAN_POINT('Ctrl Pts',(25.5290937037836,0.00028358619712762,
-3.90273938444517));
#35223=CARTESIAN_POINT('Ctrl Pts',(25.5139658455212,0.000143314572967394,
-4.90412568224005));
#35224=CARTESIAN_POINT('Ctrl Pts',(25.5066066317116,0.000113426011848074,
-5.53110188175309));
#35225=CARTESIAN_POINT('Ctrl Pts',(25.5036835254715,0.000114260159312473,
-5.78214345065753));
#35226=CARTESIAN_POINT('Ctrl Pts',(25.4979434853451,0.000157626732065502,
-6.2844308036127));
#35227=CARTESIAN_POINT('Ctrl Pts',(25.4882144756133,0.000320708389550938,
-7.16391082866169));
#35228=CARTESIAN_POINT('Ctrl Pts',(25.4754245271312,0.000690105851062742,
-8.42056581874819));
#35229=CARTESIAN_POINT('Ctrl Pts',(25.4646628399057,0.000930460627113542,
-9.67481228885));
#35230=CARTESIAN_POINT('Ctrl Pts',(25.4584799010143,0.000871282544065464,
-10.5500525215716));
#35231=CARTESIAN_POINT('Ctrl Pts',(25.4553746220341,0.000748308381848376,
-11.0492006290456));
#35232=CARTESIAN_POINT('Ctrl Pts',(25.4539712258333,0.00065353868288205,
-11.2984104554626));
#35233=CARTESIAN_POINT('Ctrl Pts',(25.4529730997057,0.000568068219536715,
-11.4859485564007));
#35234=CARTESIAN_POINT('Ctrl Pts',(25.452326132432,0.000502308203846308,
-11.6118537768369));
#35235=CARTESIAN_POINT('Ctrl Pts',(25.4511248493894,0.000339436248003312,
-11.8634638331684));
#35236=CARTESIAN_POINT('Ctrl Pts',(25.4492572720771,-2.13177763458417E-5,
-12.3031350879559));
#35237=CARTESIAN_POINT('Ctrl Pts',(25.4455733009429,-0.00127151211373016,
-13.4310595204373));
#35238=CARTESIAN_POINT('Ctrl Pts',(25.4442696957111,-0.00324028611677037,
-14.6793284460138));
#35239=CARTESIAN_POINT('Ctrl Pts',(25.4442188319478,-0.00469418068542391,
-15.9315714498161));
#35240=CARTESIAN_POINT('Ctrl Pts',(25.4443718553869,-0.00519040400416343,
-16.5594233238429));
#35241=CARTESIAN_POINT('Ctrl Pts',(25.444535750671,-0.00540381450733151,
-17.063191775564));
#35242=CARTESIAN_POINT('Ctrl Pts',(25.4446148166108,-0.0054358285895357,
-17.3156504373223));
#35243=CARTESIAN_POINT('Ctrl Pts',(25.4446703968559,-0.00543021020626045,
-17.5044367377568));
#35244=CARTESIAN_POINT('Ctrl Pts',(25.4447702572895,-0.00543876491614813,
-17.6287772188686));
#35245=CARTESIAN_POINT('Ctrl Pts',(25.4452033779121,-0.00548455064734357,
-17.8778862518301));
#35246=CARTESIAN_POINT('Ctrl Pts',(25.4459484732348,-0.00556518895829205,
-18.1270891705938));
#35247=CARTESIAN_POINT('Ctrl Pts',(25.4469513666631,-0.00566934587467172,
-18.3765573041242));
#35248=CARTESIAN_POINT('Ctrl Pts',(25.4476695073721,-0.00573957025722995,
-18.5325489822974));
#35249=CARTESIAN_POINT('Ctrl Pts',(25.4482921792919,-0.0057975462711501,
-18.6573999809797));
#35250=CARTESIAN_POINT('Ctrl Pts',(25.448943962461,-0.00585579423744788,
-18.7822849044884));
#35251=CARTESIAN_POINT('Ctrl Pts',(25.4508407251618,-0.00601388244252327,
-19.1258655044693));
#35252=CARTESIAN_POINT('Ctrl Pts',(25.4544128386284,-0.00623383029622586,
-19.6888923083069));
#35253=CARTESIAN_POINT('Ctrl Pts',(25.4607136401172,-0.00621497217796829,
-20.6921962973884));
#35254=CARTESIAN_POINT('Ctrl Pts',(25.4659070379412,-0.00488152850010207,
-21.950908820203));
#35255=CARTESIAN_POINT('Ctrl Pts',(25.4617334310053,-0.00136543214013412,
-22.9630575020273));
#35256=CARTESIAN_POINT('Ctrl Pts',(25.4548895692197,0.00193924301537645,
-23.5956290011506));
#35257=CARTESIAN_POINT('Ctrl Pts',(25.451682010114,0.00341722181846537,
-23.8468144058512));
#35258=CARTESIAN_POINT('Ctrl Pts',(25.4435054679934,0.00701771022553986,
-24.3489788833278));
#35259=CARTESIAN_POINT('Ctrl Pts',(25.4251966044907,0.0147766336876126,
-25.2286345451861));
#35260=CARTESIAN_POINT('Ctrl Pts',(25.3911009360267,0.0290385074477614,
-26.4856458523038));
#35261=CARTESIAN_POINT('Ctrl Pts',(25.3486156498219,0.0471068872725806,
-27.9915651436109));
#35262=CARTESIAN_POINT('Ctrl Pts',(25.3263690740992,0.0568900860452525,
-28.9911557795488));
#35263=CARTESIAN_POINT('Ctrl Pts',(25.3175812742222,0.0607584266492917,
-29.5516223804273));
#35264=CARTESIAN_POINT('Ctrl Pts',(25.3156293787246,0.061592916379088,-29.6769343510659));
#35265=CARTESIAN_POINT('Ctrl Pts',(25.3117385973929,0.0632320080383922,
-29.9271772256254));
#35266=CARTESIAN_POINT('Ctrl Pts',(25.3049829328802,0.0660034853406051,
-30.365428785787));
#35267=CARTESIAN_POINT('Ctrl Pts',(25.2919218208384,0.0711141872250324,
-31.2421328820492));
#35268=CARTESIAN_POINT('Ctrl Pts',(25.2789764183782,0.0758345991570889,
-32.244390638728));
#35269=CARTESIAN_POINT('Ctrl Pts',(25.2700163853228,0.0790603100313161,
-33.2458396436738));
#35270=CARTESIAN_POINT('Ctrl Pts',(25.2657798433522,0.0806436515990896,
-33.996278996021));
#35271=CARTESIAN_POINT('Ctrl Pts',(25.2644794704812,0.0813586561400045,
-34.745678118443));
#35272=CARTESIAN_POINT('Ctrl Pts',(25.2659042009034,0.081188793023538,-35.2444190767083));
#35273=CARTESIAN_POINT('Ctrl Pts',(25.2679651629538,0.080793461154485,-35.6190947913638));
#35274=CARTESIAN_POINT('Ctrl Pts',(25.2698038021904,0.0804011451233684,
-35.8696786868496));
#35275=CARTESIAN_POINT('Ctrl Pts',(25.2751350616424,0.0791410965171598,
-36.3705619577952));
#35276=CARTESIAN_POINT('Ctrl Pts',(25.2882912666579,0.0758383373910412,
-37.2456130265893));
#35277=CARTESIAN_POINT('Ctrl Pts',(25.3263009832524,0.0655881685321379,
-38.9934148472535));
#35278=CARTESIAN_POINT('Ctrl Pts',(25.3660237714869,0.0537048238599824,
-40.4924681546936));
#35279=CARTESIAN_POINT('Ctrl Pts',(25.3868173702797,0.0461422196979259,
-41.6233324791523));
#35280=CARTESIAN_POINT('Ctrl Pts',(25.3912373871007,0.0436140991761894,
-41.860221123796));
#35281=CARTESIAN_POINT('Ctrl Pts',(25.3973700983514,0.0374224242567952,
-42.2256358743637));
#35282=CARTESIAN_POINT('Ctrl Pts',(25.4031185807571,0.0293769893550175,
-42.5920052031964));
#35283=CARTESIAN_POINT('Ctrl Pts',(25.4103981796825,0.0168179227951479,
-43.0861397328003));
#35284=CARTESIAN_POINT('Ctrl Pts',(25.4190295780276,-0.00101099563237717,
-43.7112799075222));
#35285=CARTESIAN_POINT('Ctrl Pts',(25.4294620202946,-0.021554817131394,
-44.4739945711385));
#35286=CARTESIAN_POINT('Ctrl Pts',(25.4389209355737,-0.0342398653924662,
-45.1191659333761));
#35287=CARTESIAN_POINT('Ctrl Pts',(25.4473581299803,-0.0393363436383698,
-45.641235380365));
#35288=CARTESIAN_POINT('Ctrl Pts',(25.4542390415722,-0.0400471293213535,
-46.0355131625125));
#35289=CARTESIAN_POINT('Ctrl Pts',(25.4617820786829,-0.0370233890860234,
-46.4325422982045));
#35290=CARTESIAN_POINT('Ctrl Pts',(25.472856685772,-0.0271478199940004,
-46.9654673795409));
#35291=CARTESIAN_POINT('Ctrl Pts',(25.4825121168589,-0.0122484618405171,
-47.3690991664361));
#35292=CARTESIAN_POINT('Ctrl Pts',(25.493267506116,0.00907138186284126,
-47.7756692098869));
#35293=CARTESIAN_POINT('Ctrl Pts',(25.501211784735,0.0220973664887757,-48.0244308258799));
#35294=CARTESIAN_POINT('Ctrl Pts',(25.5199370045213,0.050323927401844,-48.5388691091687));
#35295=CARTESIAN_POINT('Ctrl Pts',(25.5588730890254,0.104697561159238,-49.440270598891));
#35296=CARTESIAN_POINT('Ctrl Pts',(25.6257355173962,0.208531107070698,-50.7555447682703));
#35297=CARTESIAN_POINT('Ctrl Pts',(25.7002509619933,0.409804400073271,-52.3671232960966));
#35298=CARTESIAN_POINT('Ctrl Pts',(25.728247498021,0.618019263522986,-53.4624325198976));
#35299=CARTESIAN_POINT('Ctrl Pts',(25.7334600658104,0.778437845763766,-54.1532441424037));
#35300=CARTESIAN_POINT('Ctrl Pts',(25.7349319083926,0.845541179631897,-54.4301320189739));
#35301=CARTESIAN_POINT('Ctrl Pts',(25.7347380859195,0.989797646729615,-54.9813031273514));
#35302=CARTESIAN_POINT('Ctrl Pts',(25.7272770131462,1.26607155773159,-55.9368281010095));
#35303=CARTESIAN_POINT('Ctrl Pts',(25.689298194883,1.89943737823761,-57.8135359681924));
#35304=CARTESIAN_POINT('Ctrl Pts',(25.6372206757203,2.53221269783963,-59.3618236532249));
#35305=CARTESIAN_POINT('Ctrl Pts',(25.6070393087952,2.98348633857783,-60.4301512945906));
#35306=CARTESIAN_POINT('Ctrl Pts',(25.6026691806258,3.0428503469781,-60.5693675812764));
#35307=CARTESIAN_POINT('Ctrl Pts',(25.5937983070444,3.16122724568963,-60.8412878946237));
#35308=CARTESIAN_POINT('Ctrl Pts',(25.5770435088133,3.37426564143506,-61.3171444820579));
#35309=CARTESIAN_POINT('Ctrl Pts',(25.5403294318885,3.81589521074941,-62.2556527357861));
#35310=CARTESIAN_POINT('Ctrl Pts',(25.4946976885163,4.34756025896486,-63.3039212552564));
#35311=CARTESIAN_POINT('Ctrl Pts',(25.4520398017056,4.88310998404356,-64.3237077519025));
#35312=CARTESIAN_POINT('Ctrl Pts',(25.4302032332109,5.18182040324868,-64.8863115932198));
#35313=CARTESIAN_POINT('Ctrl Pts',(25.4170265395301,5.37814378610955,-65.2563773576763));
#35314=CARTESIAN_POINT('Ctrl Pts',(25.4086409738142,5.50815980319325,-65.5017282449367));
#35315=CARTESIAN_POINT('Ctrl Pts',(25.4009045103152,5.63673168239466,-65.7450459230475));
#35316=CARTESIAN_POINT('Ctrl Pts',(25.394791660978,5.74763464779616,-65.9560398076997));
#35317=CARTESIAN_POINT('Ctrl Pts',(25.3914997534428,5.81051079104281,-66.0760542003117));
#35318=CARTESIAN_POINT('Ctrl Pts',(25.3867697623633,5.90431188593719,-66.2555271536956));
#35319=CARTESIAN_POINT('Ctrl Pts',(25.3832757638548,5.9813493352091,-66.4038965917702));
#35320=CARTESIAN_POINT('Ctrl Pts',(25.3781612478994,6.10730883680973,-66.6481876229862));
#35321=CARTESIAN_POINT('Ctrl Pts',(25.3734177864175,6.24427381811155,-66.9130325327389));
#35322=CARTESIAN_POINT('Ctrl Pts',(25.3660745822116,6.51358274593333,-67.4305557185275));
#35323=CARTESIAN_POINT('Ctrl Pts',(25.3582211469451,6.98514738255385,-68.3293237287385));
#35324=CARTESIAN_POINT('Ctrl Pts',(25.3580816655429,7.92020785558271,-70.0882057983418));
#35325=CARTESIAN_POINT('Ctrl Pts',(25.3693194658115,8.7143382475515,-71.5650278595612));
#35326=CARTESIAN_POINT('Ctrl Pts',(25.3681462159118,9.30898734236341,-72.685199163973));
#35327=CARTESIAN_POINT('Ctrl Pts',(25.367917096413,9.44269738110703,-72.9370229943887));
#35328=CARTESIAN_POINT('Ctrl Pts',(25.3675776648242,9.70941010015701,-73.4391576681312));
#35329=CARTESIAN_POINT('Ctrl Pts',(25.3673528745007,10.0430572274069,-74.0670009234832));
#35330=CARTESIAN_POINT('Ctrl Pts',(25.3673284253758,10.4431899420131,-74.819578242019));
#35331=CARTESIAN_POINT('Ctrl Pts',(25.367623027978,11.2434153013325,-76.324130100766));
#35332=CARTESIAN_POINT('Ctrl Pts',(25.3682779859034,11.9100659430314,-77.5769082849159));
#35333=CARTESIAN_POINT('Ctrl Pts',(25.368278431672,12.8796456096317,-79.4004200089946));
#35334=CARTESIAN_POINT('Ctrl Pts',(25.3682785991074,13.3163163216665,-80.2216769343914));
#35335=CARTESIAN_POINT('Ctrl Pts',(25.3682785991072,13.752837909056,-81.0426546364897));
#35336=CARTESIAN_POINT('Ctrl Pts',(27.7155278763841,-0.00393385284186832,
24.8306394904181));
#35337=CARTESIAN_POINT('Ctrl Pts',(27.7156106041345,-0.00393416938080131,
24.7817603293108));
#35338=CARTESIAN_POINT('Ctrl Pts',(27.7156973673394,-0.00393450211927658,
24.7328822274878));
#35339=CARTESIAN_POINT('Ctrl Pts',(27.716721963321,-0.00393838859547021,
24.182275835805));
#35340=CARTESIAN_POINT('Ctrl Pts',(27.717503441855,-0.00394355052081269,
23.1781418767792));
#35341=CARTESIAN_POINT('Ctrl Pts',(27.7193195511872,-0.00395770727941399,
21.1695464036031));
#35342=CARTESIAN_POINT('Ctrl Pts',(27.7261385733133,-0.00398305457749233,
19.6653929760623));
#35343=CARTESIAN_POINT('Ctrl Pts',(27.7406198960983,-0.00402582649965188,
18.414344021376));
#35344=CARTESIAN_POINT('Ctrl Pts',(27.7475639508972,-0.00404747964383108,
17.9115374502442));
#35345=CARTESIAN_POINT('Ctrl Pts',(27.7649993287739,-0.00410367701289973,
16.9075543253637));
#35346=CARTESIAN_POINT('Ctrl Pts',(27.8023983213515,-0.00422371392205734,
15.1537415029734));
#35347=CARTESIAN_POINT('Ctrl Pts',(27.8379460185578,-0.00432156848241613,
13.6519620075462));
#35348=CARTESIAN_POINT('Ctrl Pts',(27.8602632773443,-0.00435458583941141,
12.3974424140735));
#35349=CARTESIAN_POINT('Ctrl Pts',(27.8693910229039,-0.00436493508005512,
11.8964697298276));
#35350=CARTESIAN_POINT('Ctrl Pts',(27.8880124740053,-0.00437568075665919,
10.8945992424429));
#35351=CARTESIAN_POINT('Ctrl Pts',(27.9202693857805,-0.00437277336843283,
9.14103287468171));
#35352=CARTESIAN_POINT('Ctrl Pts',(27.942922372983,-0.00434869611805563,
7.63582414935623));
#35353=CARTESIAN_POINT('Ctrl Pts',(27.9529816133133,-0.0043349081756363,
6.50489909332326));
#35354=CARTESIAN_POINT('Ctrl Pts',(27.9550904561317,-0.00431925130350027,
6.25451764743701));
#35355=CARTESIAN_POINT('Ctrl Pts',(27.9588519820389,-0.00424701392688201,
5.75323897220658));
#35356=CARTESIAN_POINT('Ctrl Pts',(27.9642492028057,-0.00403750286507426,
4.87463059887487));
#35357=CARTESIAN_POINT('Ctrl Pts',(27.9703983457841,-0.00348262153394864,
3.11451716859049));
#35358=CARTESIAN_POINT('Ctrl Pts',(27.9680330925388,-0.00344023067093111,
1.60884636308336));
#35359=CARTESIAN_POINT('Ctrl Pts',(27.9630586530823,-0.00424528887266004,
0.550558997922009));
#35360=CARTESIAN_POINT('Ctrl Pts',(27.9624086450966,-0.0043499597142107,
0.424586029884561));
#35361=CARTESIAN_POINT('Ctrl Pts',(27.9608907300847,-0.00459286025227315,
0.172776845081321));
#35362=CARTESIAN_POINT('Ctrl Pts',(27.957692878994,-0.00510026698762377,
-0.267430351903845));
#35363=CARTESIAN_POINT('Ctrl Pts',(27.9517513083943,-0.00602934778227967,
-0.895200587868783));
#35364=CARTESIAN_POINT('Ctrl Pts',(27.9429819494069,-0.00736901072906046,
-1.64721018097085));
#35365=CARTESIAN_POINT('Ctrl Pts',(27.9298477572099,-0.00931740432985499,
-2.64876001923851));
#35366=CARTESIAN_POINT('Ctrl Pts',(27.9121217457491,-0.0117945338553188,
-3.89973019267382));
#35367=CARTESIAN_POINT('Ctrl Pts',(27.8995090785445,-0.0132557468094068,
-4.9019715887432));
#35368=CARTESIAN_POINT('Ctrl Pts',(27.8930349152043,-0.0138297519450205,
-5.52964563288159));
#35369=CARTESIAN_POINT('Ctrl Pts',(27.8904180812731,-0.0140601142080389,
-5.780437898808));
#35370=CARTESIAN_POINT('Ctrl Pts',(27.8851124581628,-0.0145173344259218,
-6.28262787103353));
#35371=CARTESIAN_POINT('Ctrl Pts',(27.875725454074,-0.0152837624433052,
-7.16201194286542));
#35372=CARTESIAN_POINT('Ctrl Pts',(27.8625139385489,-0.0161506201033615,
-8.41929816585113));
#35373=CARTESIAN_POINT('Ctrl Pts',(27.8508862565949,-0.0163576458403922,
-9.67501482097612));
#35374=CARTESIAN_POINT('Ctrl Pts',(27.8442716872927,-0.0159714395871801,
-10.5517788288946));
#35375=CARTESIAN_POINT('Ctrl Pts',(27.8410266987454,-0.0155721145169628,
-11.0519335897028));
#35376=CARTESIAN_POINT('Ctrl Pts',(27.8395988846676,-0.0153087597685989,
-11.3016901654378));
#35377=CARTESIAN_POINT('Ctrl Pts',(27.8386031475785,-0.0150845863514239,
-11.4896701473081));
#35378=CARTESIAN_POINT('Ctrl Pts',(27.837967769797,-0.014912003675546,-11.6163073222506));
#35379=CARTESIAN_POINT('Ctrl Pts',(27.8368262603536,-0.0144846864311702,
-11.8690358141286));
#35380=CARTESIAN_POINT('Ctrl Pts',(27.8351498853946,-0.0135375479306688,
-12.3105590020318));
#35381=CARTESIAN_POINT('Ctrl Pts',(27.8323064470357,-0.0102443343565817,
-13.4419288100555));
#35382=CARTESIAN_POINT('Ctrl Pts',(27.8324069463981,-0.00499426391876198,
-14.6904514807044));
#35383=CARTESIAN_POINT('Ctrl Pts',(27.8324832190777,-0.00107387732498213,
-15.9392029541057));
#35384=CARTESIAN_POINT('Ctrl Pts',(27.8322371672579,0.000304516178078215,
-16.5644082550696));
#35385=CARTESIAN_POINT('Ctrl Pts',(27.8317057618377,0.000906063691328227,
-17.0655127643589));
#35386=CARTESIAN_POINT('Ctrl Pts',(27.8312997053129,0.00101604259468865,
-17.3164424452256));
#35387=CARTESIAN_POINT('Ctrl Pts',(27.8309339665234,0.00101659999667262,
-17.5040710809957));
#35388=CARTESIAN_POINT('Ctrl Pts',(27.8307228356329,0.00104583334236606,
-17.6294604138463));
#35389=CARTESIAN_POINT('Ctrl Pts',(27.830410768655,0.00118037429640018,
-17.8793920992222));
#35390=CARTESIAN_POINT('Ctrl Pts',(27.8302444974371,0.00141827279767814,
-18.1295378971104));
#35391=CARTESIAN_POINT('Ctrl Pts',(27.8301871488947,0.00171258365097112,
-18.3794552586451));
#35392=CARTESIAN_POINT('Ctrl Pts',(27.8301887369512,0.00191364338468692,
-18.5356582031945));
#35393=CARTESIAN_POINT('Ctrl Pts',(27.8302079147249,0.0020789458745374,
-18.6605904464526));
#35394=CARTESIAN_POINT('Ctrl Pts',(27.8302373476539,0.00224571909714837,
-18.7855154584377));
#35395=CARTESIAN_POINT('Ctrl Pts',(27.8303558545768,0.00270723948490729,
-19.1290061737529));
#35396=CARTESIAN_POINT('Ctrl Pts',(27.8306773007071,0.00338746134337307,
-19.6908470469758));
#35397=CARTESIAN_POINT('Ctrl Pts',(27.8308588116303,0.00358852653968433,
-20.6890802452549));
#35398=CARTESIAN_POINT('Ctrl Pts',(27.8288808501303,0.000456470933084654,
-21.9360876156402));
#35399=CARTESIAN_POINT('Ctrl Pts',(27.821832683648,-0.00854233090364024,
-22.9332360638372));
#35400=CARTESIAN_POINT('Ctrl Pts',(27.8146537172427,-0.0170501805523391,
-23.5546173623963));
#35401=CARTESIAN_POINT('Ctrl Pts',(27.8113777751593,-0.0208561464693165,
-23.7986271585001));
#35402=CARTESIAN_POINT('Ctrl Pts',(27.8033019918199,-0.0300516119524009,
-24.2899600801057));
#35403=CARTESIAN_POINT('Ctrl Pts',(27.7857542022908,-0.0496849425336436,
-25.1542089073046));
#35404=CARTESIAN_POINT('Ctrl Pts',(27.7543748471676,-0.0845146120712593,
-26.4023025252781));
#35405=CARTESIAN_POINT('Ctrl Pts',(27.7174388846653,-0.126663579853726,
-27.9166945666629));
#35406=CARTESIAN_POINT('Ctrl Pts',(27.7004166352905,-0.148482904650703,
-28.9349257067696));
#35407=CARTESIAN_POINT('Ctrl Pts',(27.6948542233149,-0.157190087608495,
-29.5092422475926));
#35408=CARTESIAN_POINT('Ctrl Pts',(27.6936345431008,-0.159080801738769,
-29.6346285463885));
#35409=CARTESIAN_POINT('Ctrl Pts',(27.691264706659,-0.162783190872688,-29.8867589803176));
#35410=CARTESIAN_POINT('Ctrl Pts',(27.6873298225248,-0.16901547033627,-30.3275681171679));
#35411=CARTESIAN_POINT('Ctrl Pts',(27.680482994079,-0.180454499214935,-31.2104816765876));
#35412=CARTESIAN_POINT('Ctrl Pts',(27.6758378390379,-0.190954387007905,
-32.2204659203817));
#35413=CARTESIAN_POINT('Ctrl Pts',(27.6760328730208,-0.198361068611184,
-33.2308349292764));
#35414=CARTESIAN_POINT('Ctrl Pts',(27.6790154457573,-0.202235372088996,
-33.9884291090496));
#35415=CARTESIAN_POINT('Ctrl Pts',(27.6852693481341,-0.204317459123181,
-34.745514565451));
#35416=CARTESIAN_POINT('Ctrl Pts',(27.6919010382722,-0.204407326281904,
-35.249717218533));
#35417=CARTESIAN_POINT('Ctrl Pts',(27.6979241250912,-0.203944476816674,
-35.6286417414824));
#35418=CARTESIAN_POINT('Ctrl Pts',(27.7024562249202,-0.203472746778721,
-35.8823404494921));
#35419=CARTESIAN_POINT('Ctrl Pts',(27.7133274010445,-0.201882737834755,
-36.3889814167889));
#35420=CARTESIAN_POINT('Ctrl Pts',(27.7366196682698,-0.197448353427203,
-37.2735023505669));
#35421=CARTESIAN_POINT('Ctrl Pts',(27.7965248219601,-0.181978851313276,
-39.0372131646583));
#35422=CARTESIAN_POINT('Ctrl Pts',(27.8577782633427,-0.157797010592176,
-40.545514585732));
#35423=CARTESIAN_POINT('Ctrl Pts',(27.8956018334961,-0.134531942823141,
-41.6810303600698));
#35424=CARTESIAN_POINT('Ctrl Pts',(27.903761259723,-0.130667056236929,-41.9171031268057));
#35425=CARTESIAN_POINT('Ctrl Pts',(27.9156475993859,-0.126965301462498,
-42.2829138338868));
#35426=CARTESIAN_POINT('Ctrl Pts',(27.9272547782387,-0.124974790747706,
-42.6499725926779));
#35427=CARTESIAN_POINT('Ctrl Pts',(27.9425023899414,-0.123664606083567,
-43.1461020545497));
#35428=CARTESIAN_POINT('Ctrl Pts',(27.9613809979822,-0.123027792205116,
-43.7753169177318));
#35429=CARTESIAN_POINT('Ctrl Pts',(27.9845771199602,-0.118435365113253,
-44.545694783705));
#35430=CARTESIAN_POINT('Ctrl Pts',(28.0050528544863,-0.106634821138297,
-45.1995497251918));
#35431=CARTESIAN_POINT('Ctrl Pts',(28.0225406446347,-0.0893354422462611,
-45.729822479714));
#35432=CARTESIAN_POINT('Ctrl Pts',(28.0362989127611,-0.0716272099567747,
-46.1309291427025));
#35433=CARTESIAN_POINT('Ctrl Pts',(28.0507914761749,-0.0483595244083412,
-46.5354140463417));
#35434=CARTESIAN_POINT('Ctrl Pts',(28.0712128334668,-0.00879431783632524,
-47.0790793048288));
#35435=CARTESIAN_POINT('Ctrl Pts',(28.0878498794627,0.0318081545271698,
-47.4915893744711));
#35436=CARTESIAN_POINT('Ctrl Pts',(28.1055592638943,0.0815659363833794,
-47.9077561120951));
#35437=CARTESIAN_POINT('Ctrl Pts',(28.1188418354446,0.115297825002333,-48.1753761014028));
#35438=CARTESIAN_POINT('Ctrl Pts',(28.1493598687048,0.191566326899808,-48.7149396128666));
#35439=CARTESIAN_POINT('Ctrl Pts',(28.2113220874215,0.344705652707654,-49.6511595987853));
#35440=CARTESIAN_POINT('Ctrl Pts',(28.3112761493627,0.617893217392755,-50.9746068171927));
#35441=CARTESIAN_POINT('Ctrl Pts',(28.4097812738316,1.00886628162702,-52.5319378166776));
#35442=CARTESIAN_POINT('Ctrl Pts',(28.4390786440405,1.28767941036866,-53.552314578807));
#35443=CARTESIAN_POINT('Ctrl Pts',(28.4403749025846,1.46043255501218,-54.187964888863));
#35444=CARTESIAN_POINT('Ctrl Pts',(28.4389318054096,1.53300109764453,-54.4528958189231));
#35445=CARTESIAN_POINT('Ctrl Pts',(28.4312020513412,1.68004052263621,-54.9775443276195));
#35446=CARTESIAN_POINT('Ctrl Pts',(28.4053868143613,1.94588833285434,-55.8966092099976));
#35447=CARTESIAN_POINT('Ctrl Pts',(28.3162447976202,2.50764073843331,-57.7248393212858));
#35448=CARTESIAN_POINT('Ctrl Pts',(28.2091691509567,3.04002742409168,-59.2686626610434));
#35449=CARTESIAN_POINT('Ctrl Pts',(28.1493298592453,3.43444480648254,-60.3423774514013));
#35450=CARTESIAN_POINT('Ctrl Pts',(28.1416132495178,3.48323051822477,-60.4752311183287));
#35451=CARTESIAN_POINT('Ctrl Pts',(28.1255647390676,3.58128135589683,-60.7394082384028));
#35452=CARTESIAN_POINT('Ctrl Pts',(28.0955889856453,3.75532904521311,-61.2019343267608));
#35453=CARTESIAN_POINT('Ctrl Pts',(28.0296287411644,4.11229247223529,-62.1238604209113));
#35454=CARTESIAN_POINT('Ctrl Pts',(27.9461522198004,4.54104063594089,-63.1688325671928));
#35455=CARTESIAN_POINT('Ctrl Pts',(27.8669587469973,4.98745796642251,-64.1991496102626));
#35456=CARTESIAN_POINT('Ctrl Pts',(27.826380770832,5.24407774535702,-64.7725770283981));
#35457=CARTESIAN_POINT('Ctrl Pts',(27.8019337923344,5.41695386520446,-65.1520284576054));
#35458=CARTESIAN_POINT('Ctrl Pts',(27.7863902342801,5.53263278391158,-65.4042259418254));
#35459=CARTESIAN_POINT('Ctrl Pts',(27.7720769394183,5.64893176063813,-65.6552881250302));
#35460=CARTESIAN_POINT('Ctrl Pts',(27.7607817580091,5.75109744567071,-65.8738983477784));
#35461=CARTESIAN_POINT('Ctrl Pts',(27.7547015495567,5.80958162100798,-65.9985129337661));
#35462=CARTESIAN_POINT('Ctrl Pts',(27.7459661258242,5.89740668233722,-66.1851344259272));
#35463=CARTESIAN_POINT('Ctrl Pts',(27.7395146314148,5.97078045415491,-66.3400046904007));
#35464=CARTESIAN_POINT('Ctrl Pts',(27.7300438427688,6.09251013412725,-66.59573563328));
#35465=CARTESIAN_POINT('Ctrl Pts',(27.7213616823757,6.22361047539017,-66.8678269235341));
#35466=CARTESIAN_POINT('Ctrl Pts',(27.7081078774019,6.48628712014753,-67.4006280009251));
#35467=CARTESIAN_POINT('Ctrl Pts',(27.6944680391957,6.95376801043905,-68.3208241954038));
#35468=CARTESIAN_POINT('Ctrl Pts',(27.6959663569651,7.90413467785139,-70.1072879225436));
#35469=CARTESIAN_POINT('Ctrl Pts',(27.7174181757263,8.71791680473499,-71.5789932925461));
#35470=CARTESIAN_POINT('Ctrl Pts',(27.7156266075869,9.30124239502026,-72.6817383151479));
#35471=CARTESIAN_POINT('Ctrl Pts',(27.7152842047099,9.4354274875904,-72.9352364610077));
#35472=CARTESIAN_POINT('Ctrl Pts',(27.7147734692249,9.70157307813676,-73.4374478690909));
#35473=CARTESIAN_POINT('Ctrl Pts',(27.7144402769229,10.0354711469673,-74.0665268595069));
#35474=CARTESIAN_POINT('Ctrl Pts',(27.7144063687065,10.4358528450057,-74.8196553989177));
#35475=CARTESIAN_POINT('Ctrl Pts',(27.7148556365495,11.2371667797637,-76.325264132285));
#35476=CARTESIAN_POINT('Ctrl Pts',(27.7158522161718,11.9048293991325,-77.5777501015528));
#35477=CARTESIAN_POINT('Ctrl Pts',(27.7158562496574,12.8737109173691,-79.3999540031939));
#35478=CARTESIAN_POINT('Ctrl Pts',(27.7158606407362,13.3106272082791,-80.2216754077889));
#35479=CARTESIAN_POINT('Ctrl Pts',(27.7158606407362,13.7471487956685,-81.0426531098874));
#35480=CARTESIAN_POINT('Ctrl Pts',(29.6002100937378,-0.00570612383640002,
24.8306405759807));
#35481=CARTESIAN_POINT('Ctrl Pts',(29.6002989001342,-0.00570624884174762,
24.78176144937));
#35482=CARTESIAN_POINT('Ctrl Pts',(29.6003920380491,-0.00570637939760055,
24.7328833808383));
#35483=CARTESIAN_POINT('Ctrl Pts',(29.6014919216698,-0.00570793470053486,
24.1822774476937));
#35484=CARTESIAN_POINT('Ctrl Pts',(29.6023342893883,-0.00571269138779538,
23.1781454826973));
#35485=CARTESIAN_POINT('Ctrl Pts',(29.6042940170815,-0.00572583877534936,
21.1695502348416));
#35486=CARTESIAN_POINT('Ctrl Pts',(29.6116140134114,-0.00573620328390793,
19.6653954329726));
#35487=CARTESIAN_POINT('Ctrl Pts',(29.6271419186231,-0.00574044368796074,
18.414344917972));
#35488=CARTESIAN_POINT('Ctrl Pts',(29.6345892733583,-0.00574358245359698,
17.9115396664595));
#35489=CARTESIAN_POINT('Ctrl Pts',(29.6532908087813,-0.00575338624565161,
16.9075582711688));
#35490=CARTESIAN_POINT('Ctrl Pts',(29.6934046812983,-0.00577316241557398,
15.1537490041529));
#35491=CARTESIAN_POINT('Ctrl Pts',(29.7315107250221,-0.00577400371802316,
13.6519691858614));
#35492=CARTESIAN_POINT('Ctrl Pts',(29.7553945730525,-0.005741119949668,
12.3974430625798));
#35493=CARTESIAN_POINT('Ctrl Pts',(29.7651585260561,-0.00572368866968957,
11.896467784163));
#35494=CARTESIAN_POINT('Ctrl Pts',(29.7850637534519,-0.00567597881962372,
10.8945934236694));
#35495=CARTESIAN_POINT('Ctrl Pts',(29.8195144423163,-0.00556760762166768,
9.14102402407729));
#35496=CARTESIAN_POINT('Ctrl Pts',(29.8436795735494,-0.00546919741555448,
7.63581886876459));
#35497=CARTESIAN_POINT('Ctrl Pts',(29.8544057770259,-0.00542299840893521,
6.50490484182837));
#35498=CARTESIAN_POINT('Ctrl Pts',(29.8566388765318,-0.00540546234814099,
6.25458913080819));
#35499=CARTESIAN_POINT('Ctrl Pts',(29.8605682245575,-0.00534762537235711,
5.75338201666123));
#35500=CARTESIAN_POINT('Ctrl Pts',(29.8660787804742,-0.00520160560400977,
4.87486360767608));
#35501=CARTESIAN_POINT('Ctrl Pts',(29.8719697289,-0.00483948820640255,3.11469817291051));
#35502=CARTESIAN_POINT('Ctrl Pts',(29.869397961577,-0.0048114235087629,
1.60862425262526));
#35503=CARTESIAN_POINT('Ctrl Pts',(29.8650606763383,-0.00528875922251774,
0.549858267814596));
#35504=CARTESIAN_POINT('Ctrl Pts',(29.8644924991081,-0.00535056658702854,
0.423799297997487));
#35505=CARTESIAN_POINT('Ctrl Pts',(29.8631629038045,-0.00549418155172073,
0.171845739387263));
#35506=CARTESIAN_POINT('Ctrl Pts',(29.8603537126289,-0.00579390989457697,
-0.268597214816478));
#35507=CARTESIAN_POINT('Ctrl Pts',(29.8551149833809,-0.00634414333367143,
-0.896625607696168));
#35508=CARTESIAN_POINT('Ctrl Pts',(29.8473318446249,-0.00713040017255807,
-1.64883440985916));
#35509=CARTESIAN_POINT('Ctrl Pts',(29.835605595992,-0.00827613585702751,
-2.65049840535369));
#35510=CARTESIAN_POINT('Ctrl Pts',(29.8195877687245,-0.00972986558144148,
-3.90132680824059));
#35511=CARTESIAN_POINT('Ctrl Pts',(29.8078771861049,-0.0106079211921739,
-4.9031065281976));
#35512=CARTESIAN_POINT('Ctrl Pts',(29.8016893369936,-0.010963391753219,
-5.53037655675497));
#35513=CARTESIAN_POINT('Ctrl Pts',(29.7991956095894,-0.0111189600917785,
-5.78105177583071));
#35514=CARTESIAN_POINT('Ctrl Pts',(29.7941598437616,-0.0114712860324365,
-6.28301816895253));
#35515=CARTESIAN_POINT('Ctrl Pts',(29.7852703682728,-0.012158172617904,
-7.16210355326741));
#35516=CARTESIAN_POINT('Ctrl Pts',(29.7726228250825,-0.0131147854172198,
-8.41918825799379));
#35517=CARTESIAN_POINT('Ctrl Pts',(29.7607845675514,-0.0134483008526966,
-9.67500973180304));
#35518=CARTESIAN_POINT('Ctrl Pts',(29.7533079155556,-0.0130400411815235,
-10.5520040880199));
#35519=CARTESIAN_POINT('Ctrl Pts',(29.7493231299057,-0.01257931399796,-11.052338128805));
#35520=CARTESIAN_POINT('Ctrl Pts',(29.7474353170481,-0.0122651127567208,
-11.3021987660583));
#35521=CARTESIAN_POINT('Ctrl Pts',(29.7460566259942,-0.0119943543122567,
-11.4902662304204));
#35522=CARTESIAN_POINT('Ctrl Pts',(29.7451348168513,-0.0117821177244601,
-11.6170598970885));
#35523=CARTESIAN_POINT('Ctrl Pts',(29.7433122662121,-0.0112517730943604,
-11.8700207133685));
#35524=CARTESIAN_POINT('Ctrl Pts',(29.7401807944409,-0.0100653661808592,
-12.311918431288));
#35525=CARTESIAN_POINT('Ctrl Pts',(29.7324582218323,-0.00590550545204358,
-13.4439117837114));
#35526=CARTESIAN_POINT('Ctrl Pts',(29.7250466443676,0.000623289411662867,
-14.6921479165137));
#35527=CARTESIAN_POINT('Ctrl Pts',(29.7194556385609,0.00502339709455761,
-15.9396896263156));
#35528=CARTESIAN_POINT('Ctrl Pts',(29.7171528919325,0.00638833162455389,
-16.5640736481404));
#35529=CARTESIAN_POINT('Ctrl Pts',(29.7156637887129,0.00676695964046818,
-17.0644084781654));
#35530=CARTESIAN_POINT('Ctrl Pts',(29.7150340955089,0.00669424293120357,
-17.3149143689853));
#35531=CARTESIAN_POINT('Ctrl Pts',(29.7146138519149,0.00652709518728442,
-17.5022173432018));
#35532=CARTESIAN_POINT('Ctrl Pts',(29.7143264146382,0.00642164488428857,
-17.6274847142069));
#35533=CARTESIAN_POINT('Ctrl Pts',(29.7137256018092,0.00626720074023811,
-17.8771353260958));
#35534=CARTESIAN_POINT('Ctrl Pts',(29.7130842190378,0.00617674100949031,
-18.1270372465979));
#35535=CARTESIAN_POINT('Ctrl Pts',(29.7124460673569,0.00611433711372318,
-18.3767246179939));
#35536=CARTESIAN_POINT('Ctrl Pts',(29.712047395045,0.00608229662135253,
-18.5327935609526));
#35537=CARTESIAN_POINT('Ctrl Pts',(29.7117343091275,0.00605607845166938,
-18.6576230389906));
#35538=CARTESIAN_POINT('Ctrl Pts',(29.7114255053145,0.00602857561386291,
-18.782448723037));
#35539=CARTESIAN_POINT('Ctrl Pts',(29.7105856794882,0.00594243490906421,
-19.1256744595573));
#35540=CARTESIAN_POINT('Ctrl Pts',(29.7093569756374,0.00568593401260037,
-19.6871396016039));
#35541=CARTESIAN_POINT('Ctrl Pts',(29.7080087336263,0.00417192491291634,
-20.6847928678057));
#35542=CARTESIAN_POINT('Ctrl Pts',(29.7087982191887,-0.00112163915555453,
-21.9310851831672));
#35543=CARTESIAN_POINT('Ctrl Pts',(29.7139850254477,-0.0122670608579555,
-22.9276090155673));
#35544=CARTESIAN_POINT('Ctrl Pts',(29.7194119080898,-0.0224053888038508,
-23.548634519785));
#35545=CARTESIAN_POINT('Ctrl Pts',(29.7217664646152,-0.0269248482588539,
-23.7911111990818));
#35546=CARTESIAN_POINT('Ctrl Pts',(29.7272503068371,-0.0380593889693665,
-24.2806287192842));
#35547=CARTESIAN_POINT('Ctrl Pts',(29.7387592909759,-0.062226793790845,
-25.1423683057187));
#35548=CARTESIAN_POINT('Ctrl Pts',(29.7596607464096,-0.105749834326537,
-26.3902395876224));
#35549=CARTESIAN_POINT('Ctrl Pts',(29.7890543841874,-0.158476650180068,
-27.9092333040972));
#35550=CARTESIAN_POINT('Ctrl Pts',(29.8093101555645,-0.183628753409201,
-28.9340113861485));
#35551=CARTESIAN_POINT('Ctrl Pts',(29.8204946969917,-0.192072165295886,
-29.5129698492737));
#35552=CARTESIAN_POINT('Ctrl Pts',(29.8229722322911,-0.193866686645311,
-29.6384331626403));
#35553=CARTESIAN_POINT('Ctrl Pts',(29.8278919393808,-0.197330745845292,
-29.8913006822493));
#35554=CARTESIAN_POINT('Ctrl Pts',(29.8364146617225,-0.202940840499442,
-30.3332238844636));
#35555=CARTESIAN_POINT('Ctrl Pts',(29.8533485531302,-0.212312140634371,
-31.2189730912166));
#35556=CARTESIAN_POINT('Ctrl Pts',(29.873222181893,-0.217983824509602,-32.2329556173296));
#35557=CARTESIAN_POINT('Ctrl Pts',(29.8954103194336,-0.217222257306601,
-33.2482347387287));
#35558=CARTESIAN_POINT('Ctrl Pts',(29.9136435426566,-0.213057285220415,
-34.0099224273251));
#35559=CARTESIAN_POINT('Ctrl Pts',(29.9338055008375,-0.204823505354437,
-34.7715069329928));
#35560=CARTESIAN_POINT('Ctrl Pts',(29.9488407513319,-0.196378497002392,
-35.2789820981113));
#35561=CARTESIAN_POINT('Ctrl Pts',(29.9608608438713,-0.188819591402007,
-35.6604624402291));
#35562=CARTESIAN_POINT('Ctrl Pts',(29.9692936010343,-0.18335102815823,-35.915679061952));
#35563=CARTESIAN_POINT('Ctrl Pts',(29.9874908722616,-0.170850653216882,
-36.4253425766179));
#35564=CARTESIAN_POINT('Ctrl Pts',(30.0223072141217,-0.144947484904871,
-37.3148844095339));
#35565=CARTESIAN_POINT('Ctrl Pts',(30.100325464607,-0.0782827314807047,
-39.0876043893815));
#35566=CARTESIAN_POINT('Ctrl Pts',(30.1687343584942,0.000719127292588034,
-40.6023724685504));
#35567=CARTESIAN_POINT('Ctrl Pts',(30.2080583406784,0.0666362462407528,
-41.7418518157352));
#35568=CARTESIAN_POINT('Ctrl Pts',(30.2167140524775,0.0793717304027045,
-41.9777259748089));
#35569=CARTESIAN_POINT('Ctrl Pts',(30.2292099403697,0.0967553830352084,
-42.3441373781403));
#35570=CARTESIAN_POINT('Ctrl Pts',(30.2413254660434,0.112512992435887,-42.7119145187934));
#35571=CARTESIAN_POINT('Ctrl Pts',(30.2569693086651,0.132565735837706,-43.2095398905444));
#35572=CARTESIAN_POINT('Ctrl Pts',(30.2756372878933,0.157432667124367,-43.8413320000696));
#35573=CARTESIAN_POINT('Ctrl Pts',(30.2967247796072,0.193037461349602,-44.6159223094752));
#35574=CARTESIAN_POINT('Ctrl Pts',(30.3132192490903,0.232789029516669,-45.2740518150012));
#35575=CARTESIAN_POINT('Ctrl Pts',(30.3256359826119,0.274056483815724,-45.8079455044184));
#35576=CARTESIAN_POINT('Ctrl Pts',(30.3345612437144,0.310583052433669,-46.2118950495979));
#35577=CARTESIAN_POINT('Ctrl Pts',(30.3430579940097,0.353569674361366,-46.6192737502179));
#35578=CARTESIAN_POINT('Ctrl Pts',(30.353711866588,0.420723951037079,-47.1668036671869));
#35579=CARTESIAN_POINT('Ctrl Pts',(30.3609668156114,0.483431121928524,-47.5821347560762));
#35580=CARTESIAN_POINT('Ctrl Pts',(30.3674690616424,0.556484599912766,-48.0012328869044));
#35581=CARTESIAN_POINT('Ctrl Pts',(30.3723163449793,0.60922824910479,-48.2828209099944));
#35582=CARTESIAN_POINT('Ctrl Pts',(30.3833730441837,0.726570719937063,-48.8378186704525));
#35583=CARTESIAN_POINT('Ctrl Pts',(30.4050881001414,0.959498388023445,-49.7922951178013));
#35584=CARTESIAN_POINT('Ctrl Pts',(30.4360609436282,1.34705064834406,-51.1074078461644));
#35585=CARTESIAN_POINT('Ctrl Pts',(30.4569223855284,1.82982481176224,-52.6165998976898));
#35586=CARTESIAN_POINT('Ctrl Pts',(30.4525459065398,2.11955233242534,-53.5805979983041));
#35587=CARTESIAN_POINT('Ctrl Pts',(30.4403000101703,2.27815765531267,-54.1716093252403));
#35588=CARTESIAN_POINT('Ctrl Pts',(30.432735890706,2.34416941058513,-54.4230251518103));
#35589=CARTESIAN_POINT('Ctrl Pts',(30.4136112348139,2.47157031309743,-54.9216083177821));
#35590=CARTESIAN_POINT('Ctrl Pts',(30.3684069581331,2.68928140342694,-55.8039465899849));
#35591=CARTESIAN_POINT('Ctrl Pts',(30.2415291238702,3.11258624593874,-57.5867140656665));
#35592=CARTESIAN_POINT('Ctrl Pts',(30.1002208360485,3.50765107649709,-59.1391076348399));
#35593=CARTESIAN_POINT('Ctrl Pts',(30.0251249611869,3.84005238168457,-60.2381524787919));
#35594=CARTESIAN_POINT('Ctrl Pts',(30.0163721182157,3.87864932191528,-60.3659328037547));
#35595=CARTESIAN_POINT('Ctrl Pts',(29.9981933064438,3.95727247694841,-60.6251189253043));
#35596=CARTESIAN_POINT('Ctrl Pts',(29.9655464703264,4.09550572043887,-61.0778962302091));
#35597=CARTESIAN_POINT('Ctrl Pts',(29.8971217556328,4.37816350489105,-61.9875267268624));
#35598=CARTESIAN_POINT('Ctrl Pts',(29.8160872524673,4.71961990354699,-63.0303865845481));
#35599=CARTESIAN_POINT('Ctrl Pts',(29.7413689014789,5.08847429459405,-64.0726429042806));
#35600=CARTESIAN_POINT('Ctrl Pts',(29.7035172061765,5.30736914621276,-64.6576470039614));
#35601=CARTESIAN_POINT('Ctrl Pts',(29.680707169744,5.45856492187508,-65.0468473336499));
#35602=CARTESIAN_POINT('Ctrl Pts',(29.6661934302272,5.56078387914126,-65.3060644005528));
#35603=CARTESIAN_POINT('Ctrl Pts',(29.6527755459062,5.66520903499327,-65.5649233293135));
#35604=CARTESIAN_POINT('Ctrl Pts',(29.6421101614254,5.75856118215573,-65.7910134859799));
#35605=CARTESIAN_POINT('Ctrl Pts',(29.6363364245003,5.81248486888892,-65.9200874000455));
#35606=CARTESIAN_POINT('Ctrl Pts',(29.6280041870977,5.89395736346093,-66.113579136086));
#35607=CARTESIAN_POINT('Ctrl Pts',(29.6217565785856,5.96308461558392,-66.2745581212124));
#35608=CARTESIAN_POINT('Ctrl Pts',(29.612413901581,6.0792941599492,-66.5408461079343));
#35609=CARTESIAN_POINT('Ctrl Pts',(29.6038932231889,6.20472440432365,-66.8215903272585));
#35610=CARTESIAN_POINT('Ctrl Pts',(29.5910146048047,6.46050135730378,-67.3706075763046));
#35611=CARTESIAN_POINT('Ctrl Pts',(29.5780658698442,6.92422326566066,-68.3135400697311));
#35612=CARTESIAN_POINT('Ctrl Pts',(29.5803465546603,7.89115824189205,-70.1267298299807));
#35613=CARTESIAN_POINT('Ctrl Pts',(29.6013021167182,8.72542547986538,-71.5935063992352));
#35614=CARTESIAN_POINT('Ctrl Pts',(29.5997390704358,9.2976740218444,-72.6785697945003));
#35615=CARTESIAN_POINT('Ctrl Pts',(29.5994345993365,9.4323604289187,-72.9336723885517));
#35616=CARTESIAN_POINT('Ctrl Pts',(29.5989838213741,9.69797488227456,-73.435839448843));
#35617=CARTESIAN_POINT('Ctrl Pts',(29.5986845091741,10.0321181096191,-74.0660328586202));
#35618=CARTESIAN_POINT('Ctrl Pts',(29.5986520948479,10.4326930518429,-74.819598742444));
#35619=CARTESIAN_POINT('Ctrl Pts',(29.5990423700363,11.2349229683723,-76.3261145564624));
#35620=CARTESIAN_POINT('Ctrl Pts',(29.5999052687731,11.9034263089648,-77.5783970633848));
#35621=CARTESIAN_POINT('Ctrl Pts',(29.5999024700786,12.8717351076972,-79.3995546363377));
#35622=CARTESIAN_POINT('Ctrl Pts',(29.5999011496128,13.3088569590276,-80.2216783074562));
#35623=CARTESIAN_POINT('Ctrl Pts',(29.5999011496129,13.745378546417,-81.0426560095546));
#35624=CARTESIAN_POINT('Ctrl Pts',(31.0171866232326,-0.00299204424446314,
24.8306373191774));
#35625=CARTESIAN_POINT('Ctrl Pts',(31.0172800374408,-0.00299175195389374,
24.7817580900798));
#35626=CARTESIAN_POINT('Ctrl Pts',(31.0173780076597,-0.00299144622876444,
24.7328799158363));
#35627=CARTESIAN_POINT('Ctrl Pts',(31.0185349571666,-0.00298779232615199,
24.1822728181405));
#35628=CARTESIAN_POINT('Ctrl Pts',(31.0194242644657,-0.00298701896593174,
23.1781407180979));
#35629=CARTESIAN_POINT('Ctrl Pts',(31.0214952096736,-0.0029872921198035,
21.169542798472));
#35630=CARTESIAN_POINT('Ctrl Pts',(31.029194999137,-0.00296246222206313,
19.6653857519563));
#35631=CARTESIAN_POINT('Ctrl Pts',(31.0455122304153,-0.00289957867720278,
18.4143334371842));
#35632=CARTESIAN_POINT('Ctrl Pts',(31.0533392075379,-0.00286986433034777,
17.9115212109908));
#35633=CARTESIAN_POINT('Ctrl Pts',(31.0729958361359,-0.0027956849546429,
16.907535608882));
#35634=CARTESIAN_POINT('Ctrl Pts',(31.1151570483659,-0.00263552471530198,
15.1537304867153));
#35635=CARTESIAN_POINT('Ctrl Pts',(31.1551908943919,-0.00247432632475043,
13.6519762098179));
#35636=CARTESIAN_POINT('Ctrl Pts',(31.1802515164793,-0.00235944594013484,
12.3974782675912));
#35637=CARTESIAN_POINT('Ctrl Pts',(31.1904926330016,-0.00231080546792335,
11.8965147288727));
#35638=CARTESIAN_POINT('Ctrl Pts',(31.2113586077952,-0.00220612306289779,
10.8946572774833));
#35639=CARTESIAN_POINT('Ctrl Pts',(31.2474478081631,-0.00201365744969911,
9.14110480766528));
#35640=CARTESIAN_POINT('Ctrl Pts',(31.2727401436192,-0.00186903671229844,
7.63588960317416));
#35641=CARTESIAN_POINT('Ctrl Pts',(31.2839672924156,-0.00180566320929945,
6.50496387401208));
#35642=CARTESIAN_POINT('Ctrl Pts',(31.2862988414548,-0.00179111271627116,
6.25472622040602));
#35643=CARTESIAN_POINT('Ctrl Pts',(31.2903812975918,-0.00176082906178743,
5.75360134193579));
#35644=CARTESIAN_POINT('Ctrl Pts',(31.2960570243148,-0.00170698473366819,
4.87518683510538));
#35645=CARTESIAN_POINT('Ctrl Pts',(31.301972124276,-0.00161246329748242,
3.11495098143548));
#35646=CARTESIAN_POINT('Ctrl Pts',(31.2992403549997,-0.00161384079096441,
1.60838932949574));
#35647=CARTESIAN_POINT('Ctrl Pts',(31.2950393056685,-0.00170936156091001,
0.549047151704652));
#35648=CARTESIAN_POINT('Ctrl Pts',(31.2944887558957,-0.00172172143893924,
0.422887489995395));
#35649=CARTESIAN_POINT('Ctrl Pts',(31.2931984938341,-0.00175049760823538,
0.170763124126403));
#35650=CARTESIAN_POINT('Ctrl Pts',(31.2904683982893,-0.00181071082727286,
-0.269959669295347));
#35651=CARTESIAN_POINT('Ctrl Pts',(31.2853649746126,-0.00192254888288488,
-0.898298554812866));
#35652=CARTESIAN_POINT('Ctrl Pts',(31.2777684919425,-0.00208464034506392,
-1.65074301382481));
#35653=CARTESIAN_POINT('Ctrl Pts',(31.2662973694254,-0.0023259096128296,
-2.65253152566603));
#35654=CARTESIAN_POINT('Ctrl Pts',(31.2505760830858,-0.0026417561311629,
-3.90315870134114));
#35655=CARTESIAN_POINT('Ctrl Pts',(31.2389823001759,-0.00285192107937762,
-4.90440181540127));
#35656=CARTESIAN_POINT('Ctrl Pts',(31.2327966858658,-0.00295087232972535,
-5.53123792318891));
#35657=CARTESIAN_POINT('Ctrl Pts',(31.2303236229937,-0.00299944518517874,
-5.78202002293138));
#35658=CARTESIAN_POINT('Ctrl Pts',(31.225391374235,-0.00312588674535756,
-6.28399733300269));
#35659=CARTESIAN_POINT('Ctrl Pts',(31.2167989280666,-0.00340425233937084,
-7.16308358740321));
#35660=CARTESIAN_POINT('Ctrl Pts',(31.2046634006741,-0.00385283489059006,
-8.41981571843076));
#35661=CARTESIAN_POINT('Ctrl Pts',(31.192760038336,-0.00407574900706089,
-9.67490155539903));
#35662=CARTESIAN_POINT('Ctrl Pts',(31.184576129495,-0.003962792679451,-10.5511513249466));
#35663=CARTESIAN_POINT('Ctrl Pts',(31.1799452252549,-0.00379956597116409,
-11.0509969797361));
#35664=CARTESIAN_POINT('Ctrl Pts',(31.1776468697959,-0.00368176937487282,
-11.3005933523199));
#35665=CARTESIAN_POINT('Ctrl Pts',(31.1759217329085,-0.00357798355857695,
-11.4884477295729));
#35666=CARTESIAN_POINT('Ctrl Pts',(31.1747307640991,-0.00349601556723211,
-11.6148890942837));
#35667=CARTESIAN_POINT('Ctrl Pts',(31.1722364279941,-0.00327958682477642,
-11.8673074536642));
#35668=CARTESIAN_POINT('Ctrl Pts',(31.1676106338369,-0.00277616568156974,
-12.3083010607177));
#35669=CARTESIAN_POINT('Ctrl Pts',(31.1547118667396,-0.000960816288891971,
-13.4385717099228));
#35670=CARTESIAN_POINT('Ctrl Pts',(31.1393834657479,0.00201370407255788,
-14.6866895026391));
#35671=CARTESIAN_POINT('Ctrl Pts',(31.1288818117628,0.00396512956716421,
-15.9359205297263));
#35672=CARTESIAN_POINT('Ctrl Pts',(31.1253471619125,0.00449851534797558,
-16.5615504263016));
#35673=CARTESIAN_POINT('Ctrl Pts',(31.123813009011,0.00454494116123564,
-17.0631003642246));
#35674=CARTESIAN_POINT('Ctrl Pts',(31.1235321706078,0.00442294582556831,
-17.3142932229386));
#35675=CARTESIAN_POINT('Ctrl Pts',(31.1235178775408,0.00426874304661423,
-17.502099921976));
#35676=CARTESIAN_POINT('Ctrl Pts',(31.1234883913472,0.00418007425389375,
-17.6265784319385));
#35677=CARTESIAN_POINT('Ctrl Pts',(31.1233659176513,0.00395307306701036,
-17.8754407324593));
#35678=CARTESIAN_POINT('Ctrl Pts',(31.1231861318757,0.00367710873470516,
-18.1244853654518));
#35679=CARTESIAN_POINT('Ctrl Pts',(31.1229959777868,0.00332690480317081,
-18.3736241718446));
#35680=CARTESIAN_POINT('Ctrl Pts',(31.1228892610535,0.00308002734341012,
-18.5293970678065));
#35681=CARTESIAN_POINT('Ctrl Pts',(31.1228170511343,0.00286282586100117,
-18.6540461903583));
#35682=CARTESIAN_POINT('Ctrl Pts',(31.1227567187964,0.00263235993411028,
-18.7787192621887));
#35683=CARTESIAN_POINT('Ctrl Pts',(31.1226559341866,0.00195365178629543,
-19.1216563816462));
#35684=CARTESIAN_POINT('Ctrl Pts',(31.1229441836729,0.000533712239019911,
-19.68336488423));
#35685=CARTESIAN_POINT('Ctrl Pts',(31.1261109527912,-0.00285231282776662,
-20.6835784311914));
#35686=CARTESIAN_POINT('Ctrl Pts',(31.1377230351493,-0.00868577361617233,
-21.9374302792362));
#35687=CARTESIAN_POINT('Ctrl Pts',(31.1602385963435,-0.014065553654675,
-22.9445900629422));
#35688=CARTESIAN_POINT('Ctrl Pts',(31.1797508256719,-0.0172592242312334,
-23.5734793564911));
#35689=CARTESIAN_POINT('Ctrl Pts',(31.1882333981687,-0.0187590953521933,
-23.8193969122014));
#35690=CARTESIAN_POINT('Ctrl Pts',(31.2078655307222,-0.0224443650309819,
-24.314803704475));
#35691=CARTESIAN_POINT('Ctrl Pts',(31.2483979655463,-0.0301709904708716,
-25.1850798180763));
#35692=CARTESIAN_POINT('Ctrl Pts',(31.3192510621073,-0.0421576005802248,
-26.4397119259467));
#35693=CARTESIAN_POINT('Ctrl Pts',(31.4105442678541,-0.0490727090890887,
-27.958767976614));
#35694=CARTESIAN_POINT('Ctrl Pts',(31.4656991678369,-0.0437895376736689,
-28.9784359331697));
#35695=CARTESIAN_POINT('Ctrl Pts',(31.4920969623829,-0.036835621476926,
-29.5530483523592));
#35696=CARTESIAN_POINT('Ctrl Pts',(31.4979193479439,-0.0352906090957437,
-29.6784470123789));
#35697=CARTESIAN_POINT('Ctrl Pts',(31.5093943242123,-0.0320515077944978,
-29.9307145964565));
#35698=CARTESIAN_POINT('Ctrl Pts',(31.5290623113824,-0.026038521043076,
-30.3719366101199));
#35699=CARTESIAN_POINT('Ctrl Pts',(31.5668943942862,-0.0123207761499249,
-31.2564232518502));
#35700=CARTESIAN_POINT('Ctrl Pts',(31.6075126695474,0.00816049901412967,
-32.2698118697941));
#35701=CARTESIAN_POINT('Ctrl Pts',(31.6470161171525,0.0356857649896198,
-33.285012417737));
#35702=CARTESIAN_POINT('Ctrl Pts',(31.6764611302861,0.0604146604395156,
-34.0469117290958));
#35703=CARTESIAN_POINT('Ctrl Pts',(31.7061338079151,0.0897085824578493,
-34.8089853898741));
#35704=CARTESIAN_POINT('Ctrl Pts',(31.7263006112609,0.112683191082764,-35.316954376036));
#35705=CARTESIAN_POINT('Ctrl Pts',(31.7416977032748,0.131411147765765,-35.698841734656));
#35706=CARTESIAN_POINT('Ctrl Pts',(31.7522103743375,0.14440488890183,-35.9538749156084));
#35707=CARTESIAN_POINT('Ctrl Pts',(31.7738532824062,0.172180260359674,-36.4633985114814));
#35708=CARTESIAN_POINT('Ctrl Pts',(31.8129445351975,0.225103674084826,-37.3525870810542));
#35709=CARTESIAN_POINT('Ctrl Pts',(31.8926538715873,0.346789697405608,-39.1246789072447));
#35710=CARTESIAN_POINT('Ctrl Pts',(31.9522857829168,0.471316329837971,-40.6395337378253));
#35711=CARTESIAN_POINT('Ctrl Pts',(31.9818045876848,0.56827802006083,-41.7793140646381));
#35712=CARTESIAN_POINT('Ctrl Pts',(31.9885951174029,0.587669054701669,-42.0158666289406));
#35713=CARTESIAN_POINT('Ctrl Pts',(31.9980821327246,0.615086545272046,-42.3828188587321));
#35714=CARTESIAN_POINT('Ctrl Pts',(32.0071087518599,0.640791292565634,-42.7510825055653));
#35715=CARTESIAN_POINT('Ctrl Pts',(32.0183226475649,0.67403479725514,-43.249063143809));
#35716=CARTESIAN_POINT('Ctrl Pts',(32.0307682837515,0.715153783936835,-43.8808613990902));
#35717=CARTESIAN_POINT('Ctrl Pts',(32.042620373242,0.769682862548015,-44.6546381777675));
#35718=CARTESIAN_POINT('Ctrl Pts',(32.0494012967017,0.824467495919128,-45.3113909381642));
#35719=CARTESIAN_POINT('Ctrl Pts',(32.0526342092818,0.877055401355374,-45.843709339823));
#35720=CARTESIAN_POINT('Ctrl Pts',(32.0538325537096,0.921699636222757,-46.2462780366077));
#35721=CARTESIAN_POINT('Ctrl Pts',(32.0536974250961,0.972370016102763,-46.6520717026781));
#35722=CARTESIAN_POINT('Ctrl Pts',(32.051603455164,1.04907493013307,-47.197270800761));
#35723=CARTESIAN_POINT('Ctrl Pts',(32.0476327337414,1.11819982422158,-47.6105991423849));
#35724=CARTESIAN_POINT('Ctrl Pts',(32.0418554401568,1.19697063345933,-48.0278371428771));
#35725=CARTESIAN_POINT('Ctrl Pts',(32.0370093390979,1.2552571080079,-48.3153661676004));
#35726=CARTESIAN_POINT('Ctrl Pts',(32.0269492025836,1.38395180559172,-48.8756501702507));
#35727=CARTESIAN_POINT('Ctrl Pts',(32.0073796248885,1.63820497082836,-49.8362698327807));
#35728=CARTESIAN_POINT('Ctrl Pts',(31.9760030483103,2.05155110483119,-51.1465206922891));
#35729=CARTESIAN_POINT('Ctrl Pts',(31.9345223527777,2.54042952179378,-52.6333826654537));
#35730=CARTESIAN_POINT('Ctrl Pts',(31.9018911272374,2.80866824949851,-53.5658649239555));
#35731=CARTESIAN_POINT('Ctrl Pts',(31.8771846719511,2.94341900039249,-54.1295428104592));
#35732=CARTESIAN_POINT('Ctrl Pts',(31.8648175905742,2.99807320889389,-54.3697618998694));
#35733=CARTESIAN_POINT('Ctrl Pts',(31.8360856950958,3.09901795679906,-54.8483308358366));
#35734=CARTESIAN_POINT('Ctrl Pts',(31.7742711480597,3.26112727366891,-55.7010632445142));
#35735=CARTESIAN_POINT('Ctrl Pts',(31.6145810013345,3.54756645215416,-57.4480884546376));
#35736=CARTESIAN_POINT('Ctrl Pts',(31.4495654705191,3.82266725475589,-59.0165294959396));
#35737=CARTESIAN_POINT('Ctrl Pts',(31.367770953786,4.10638844852506,-60.1476588478776));
#35738=CARTESIAN_POINT('Ctrl Pts',(31.3585136584601,4.13772508255956,-60.2730723916295));
#35739=CARTESIAN_POINT('Ctrl Pts',(31.3397740472031,4.20257802447826,-60.5312989229257));
#35740=CARTESIAN_POINT('Ctrl Pts',(31.3075710473081,4.31634468200943,-60.9812009781816));
#35741=CARTESIAN_POINT('Ctrl Pts',(31.2449622958405,4.55065839947622,-61.8889297924662));
#35742=CARTESIAN_POINT('Ctrl Pts',(31.1794385244147,4.83839904044304,-62.9350100374388));
#35743=CARTESIAN_POINT('Ctrl Pts',(31.122726763293,5.15907701218947,-63.987551271028));
#35744=CARTESIAN_POINT('Ctrl Pts',(31.0946368142613,5.354039507125,-64.5807134970563));
#35745=CARTESIAN_POINT('Ctrl Pts',(31.0776806560438,5.49111596067101,-64.976348444816));
#35746=CARTESIAN_POINT('Ctrl Pts',(31.0668597264748,5.58444985936914,-65.2401034842792));
#35747=CARTESIAN_POINT('Ctrl Pts',(31.0567803435495,5.68084257221062,-65.5038761735702));
#35748=CARTESIAN_POINT('Ctrl Pts',(31.0486362195788,5.76800749574544,-65.734567400679));
#35749=CARTESIAN_POINT('Ctrl Pts',(31.0441788183548,5.81865115456034,-65.8663542619541));
#35750=CARTESIAN_POINT('Ctrl Pts',(31.0376906710409,5.89546615139976,-66.063997660731));
#35751=CARTESIAN_POINT('Ctrl Pts',(31.0327000962336,5.96127690314123,-66.2286057948698));
#35752=CARTESIAN_POINT('Ctrl Pts',(31.0250025050703,6.07281901289687,-66.5011152840611));
#35753=CARTESIAN_POINT('Ctrl Pts',(31.0179956380395,6.19437698960279,-66.7887030109143));
#35754=CARTESIAN_POINT('Ctrl Pts',(31.0074757471655,6.44513738098736,-67.3493144180915));
#35755=CARTESIAN_POINT('Ctrl Pts',(30.997085233629,6.906412501861,-68.3087923116582));
#35756=CARTESIAN_POINT('Ctrl Pts',(30.999493056306,7.8855409231497,-70.1403049410983));
#35757=CARTESIAN_POINT('Ctrl Pts',(31.0168899440058,8.73456822280869,-71.6038226179437));
#35758=CARTESIAN_POINT('Ctrl Pts',(31.0158700282441,9.29917548368328,-72.6764093602891));
#35759=CARTESIAN_POINT('Ctrl Pts',(31.0156385115126,9.43422564243663,-72.9326071116161));
#35760=CARTESIAN_POINT('Ctrl Pts',(31.0153112276913,9.69948548811709,-73.4346939262143));
#35761=CARTESIAN_POINT('Ctrl Pts',(31.0150889569634,10.0338049752592,-74.0656234388318));
#35762=CARTESIAN_POINT('Ctrl Pts',(31.0150636577838,10.4344948303806,-74.8194510270631));
#35763=CARTESIAN_POINT('Ctrl Pts',(31.0153438539892,11.2372986599713,-76.3265451457017));
#35764=CARTESIAN_POINT('Ctrl Pts',(31.0159819351073,11.9063383399868,-77.578742348905));
#35765=CARTESIAN_POINT('Ctrl Pts',(31.0159924606929,12.8743106021264,-79.3992882081553));
#35766=CARTESIAN_POINT('Ctrl Pts',(31.015991633413,13.3115662212557,-80.2216742641514));
#35767=CARTESIAN_POINT('Ctrl Pts',(31.0159916334131,13.7480878086451,-81.0426519662498));
#35768=CARTESIAN_POINT('Ctrl Pts',(32.4375725283096,0.00612073677650567,
24.8306303773195));
#35769=CARTESIAN_POINT('Ctrl Pts',(32.4376704492468,0.00612173323859073,
24.781750928448));
#35770=CARTESIAN_POINT('Ctrl Pts',(32.4377731465535,0.00612277784268754,
24.732872528879));
#35771=CARTESIAN_POINT('Ctrl Pts',(32.438985886721,0.0061351289779464,24.1822628969437));
#35772=CARTESIAN_POINT('Ctrl Pts',(32.4399193830562,0.00614560068208076,
23.1781289417908));
#35773=CARTESIAN_POINT('Ctrl Pts',(32.4420948130036,0.00617032469026516,
21.1695259205625));
#35774=CARTESIAN_POINT('Ctrl Pts',(32.4501651077224,0.00625264801595857,
19.6653663333986));
#35775=CARTESIAN_POINT('Ctrl Pts',(32.467261250398,0.00642226561136431,
18.4143123354664));
#35776=CARTESIAN_POINT('Ctrl Pts',(32.4754620024458,0.00650459012566578,
17.9114868513781));
#35777=CARTESIAN_POINT('Ctrl Pts',(32.4960567542474,0.00671318284351931,
16.9074925722283));
#35778=CARTESIAN_POINT('Ctrl Pts',(32.540229806681,0.0071610401825099,15.1536918206885));
#35779=CARTESIAN_POINT('Ctrl Pts',(32.5821659779686,0.0075747936488959,
13.6519837245366));
#35780=CARTESIAN_POINT('Ctrl Pts',(32.6084134956282,0.00781133248939808,
12.3975410538733));
#35781=CARTESIAN_POINT('Ctrl Pts',(32.6191392183056,0.00790562449951455,
11.8966003565388));
#35782=CARTESIAN_POINT('Ctrl Pts',(32.6409890710773,0.00808999154332186,
10.8947764919162));
#35783=CARTESIAN_POINT('Ctrl Pts',(32.6787755656417,0.00839256724841023,
9.14125760874515));
#35784=CARTESIAN_POINT('Ctrl Pts',(32.7052468202478,0.00858448180949316,
7.63602490847467));
#35785=CARTESIAN_POINT('Ctrl Pts',(32.7170051004007,0.00866427690422162,
6.50506873960121));
#35786=CARTESIAN_POINT('Ctrl Pts',(32.7194476626338,0.00867657290767804,
6.25489858217397));
#35787=CARTESIAN_POINT('Ctrl Pts',(32.723724156199,0.00868237884311895,
5.7538424239641));
#35788=CARTESIAN_POINT('Ctrl Pts',(32.7296680260123,0.008651717567273,4.87551538707216));
#35789=CARTESIAN_POINT('Ctrl Pts',(32.7358654941957,0.00849526231436584,
3.11521304601986));
#35790=CARTESIAN_POINT('Ctrl Pts',(32.7330050923788,0.00842882889151111,
1.60822825847469));
#35791=CARTESIAN_POINT('Ctrl Pts',(32.7286287931558,0.00863352408019025,
0.548390972029742));
#35792=CARTESIAN_POINT('Ctrl Pts',(32.7280556012293,0.00866031411611293,
0.422146457370445));
#35793=CARTESIAN_POINT('Ctrl Pts',(32.7267103229818,0.00872296322295062,
0.169878000266251));
#35794=CARTESIAN_POINT('Ctrl Pts',(32.7238611536692,0.00885483901651413,
-0.271079661633083));
#35795=CARTESIAN_POINT('Ctrl Pts',(32.7185257185815,0.00909719910768501,
-0.89967508832505));
#35796=CARTESIAN_POINT('Ctrl Pts',(32.7105872595901,0.00944673870218814,
-1.65231437353842));
#35797=CARTESIAN_POINT('Ctrl Pts',(32.698591518813,0.00995047629065278,
-2.65420250676402));
#35798=CARTESIAN_POINT('Ctrl Pts',(32.6821693413152,0.0105775487649706,
-3.9046733867623));
#35799=CARTESIAN_POINT('Ctrl Pts',(32.6700718046237,0.0109227635378567,
-4.90546860538031));
#35800=CARTESIAN_POINT('Ctrl Pts',(32.6636503115398,0.0110412576361191,
-5.53195733759867));
#35801=CARTESIAN_POINT('Ctrl Pts',(32.6611026206047,0.0111029208113027,
-5.78307151337921));
#35802=CARTESIAN_POINT('Ctrl Pts',(32.6560786904651,0.0112707827624278,
-6.28532116522749));
#35803=CARTESIAN_POINT('Ctrl Pts',(32.6474492938381,0.0116453384518062,
-7.16474040450405));
#35804=CARTESIAN_POINT('Ctrl Pts',(32.6353941325091,0.0122156502770102,
-8.42102129578186));
#35805=CARTESIAN_POINT('Ctrl Pts',(32.6232792542869,0.0123006655414279,
-9.67459864505452));
#35806=CARTESIAN_POINT('Ctrl Pts',(32.6145352572378,0.0118326570992625,
-10.5491928952008));
#35807=CARTESIAN_POINT('Ctrl Pts',(32.6094313904953,0.0113765141786167,
-11.0479256199958));
#35808=CARTESIAN_POINT('Ctrl Pts',(32.6068351489801,0.011080033509664,-11.2969138483581));
#35809=CARTESIAN_POINT('Ctrl Pts',(32.604862964816,0.0108284854691137,-11.4842693213742));
#35810=CARTESIAN_POINT('Ctrl Pts',(32.6034581502333,0.0106345574586929,
-11.6096889651575));
#35811=CARTESIAN_POINT('Ctrl Pts',(32.6003606096668,0.0101420129158296,
-11.860601970361));
#35812=CARTESIAN_POINT('Ctrl Pts',(32.5942538989981,0.00903576810677099,
-12.2991065557788));
#35813=CARTESIAN_POINT('Ctrl Pts',(32.5757932155024,0.00517063181383277,
-13.4249465396148));
#35814=CARTESIAN_POINT('Ctrl Pts',(32.5516633096074,-0.00076474121200517,
-14.6733009245517));
#35815=CARTESIAN_POINT('Ctrl Pts',(32.5380545352075,-0.00459324500449539,
-15.9284346040029));
#35816=CARTESIAN_POINT('Ctrl Pts',(32.5350003375435,-0.00565654912437246,
-16.5584041406639));
#35817=CARTESIAN_POINT('Ctrl Pts',(32.5355910795788,-0.00581636820274184,
-17.0643083481665));
#35818=CARTESIAN_POINT('Ctrl Pts',(32.5369915996141,-0.00562287815735871,
-17.3179877292813));
#35819=CARTESIAN_POINT('Ctrl Pts',(32.5385075377801,-0.00536457972547619,
-17.5076988195231));
#35820=CARTESIAN_POINT('Ctrl Pts',(32.5395516516621,-0.00526975227129406,
-17.6311265404471));
#35821=CARTESIAN_POINT('Ctrl Pts',(32.5418300401125,-0.00518431464235082,
-17.8795060413966));
#35822=CARTESIAN_POINT('Ctrl Pts',(32.5443808293887,-0.00525827931732753,
-18.1278998449213));
#35823=CARTESIAN_POINT('Ctrl Pts',(32.5472860436008,-0.00540480712456201,
-18.3770110834493));
#35824=CARTESIAN_POINT('Ctrl Pts',(32.5492427809058,-0.00551399113095648,
-18.5328476680375));
#35825=CARTESIAN_POINT('Ctrl Pts',(32.5509033290443,-0.00560164294745968,
-18.6576559792242));
#35826=CARTESIAN_POINT('Ctrl Pts',(32.5526266366226,-0.00568581122353676,
-18.7825370683472));
#35827=CARTESIAN_POINT('Ctrl Pts',(32.5576121159634,-0.00590691263338564,
-19.1262829157936));
#35828=CARTESIAN_POINT('Ctrl Pts',(32.5672340253502,-0.00599570887245065,
-19.6905177021123));
#35829=CARTESIAN_POINT('Ctrl Pts',(32.5890910784554,-0.00413567925224601,
-20.6984784042354));
#35830=CARTESIAN_POINT('Ctrl Pts',(32.6260269114473,0.00445448628603799,
-21.9672178731562));
#35831=CARTESIAN_POINT('Ctrl Pts',(32.6688510646589,0.0221318845874462,
-22.9920195822445));
#35832=CARTESIAN_POINT('Ctrl Pts',(32.7012102272047,0.0385324406427145,
-23.634396489595));
#35833=CARTESIAN_POINT('Ctrl Pts',(32.715031917855,0.0455217649744831,-23.8880348573153));
#35834=CARTESIAN_POINT('Ctrl Pts',(32.7465170742004,0.0616196840009675,
-24.3957111275666));
#35835=CARTESIAN_POINT('Ctrl Pts',(32.8105415409616,0.0952581051992893,
-25.2842461053142));
#35836=CARTESIAN_POINT('Ctrl Pts',(32.9210591618046,0.159762402551823,-26.5530608107758));
#35837=CARTESIAN_POINT('Ctrl Pts',(33.0589337037139,0.25910958635653,-28.0695863386293));
#35838=CARTESIAN_POINT('Ctrl Pts',(33.136796739872,0.330867870485165,-29.0725964140342));
#35839=CARTESIAN_POINT('Ctrl Pts',(33.1725279620985,0.368669790118915,-29.6338337416282));
#35840=CARTESIAN_POINT('Ctrl Pts',(33.1803870386095,0.377025613103238,-29.759044228272));
#35841=CARTESIAN_POINT('Ctrl Pts',(33.1957438638766,0.393733031112438,-30.0093990829174));
#35842=CARTESIAN_POINT('Ctrl Pts',(33.2217030508958,0.422957178392457,-30.4481178470327));
#35843=CARTESIAN_POINT('Ctrl Pts',(33.2702186084373,0.481524710545981,-31.3272291279453));
#35844=CARTESIAN_POINT('Ctrl Pts',(33.3188327155682,0.5498143672729,-32.3352499388375));
#35845=CARTESIAN_POINT('Ctrl Pts',(33.3627484758732,0.621597850833921,-33.3452623854794));
#35846=CARTESIAN_POINT('Ctrl Pts',(33.3938233587234,0.677804083201993,-34.1034748355415));
#35847=CARTESIAN_POINT('Ctrl Pts',(33.4234183964842,0.73715538275439,-34.8619437154264));
#35848=CARTESIAN_POINT('Ctrl Pts',(33.4424931158544,0.779237276920695,-35.3676000913595));
#35849=CARTESIAN_POINT('Ctrl Pts',(33.4567175399219,0.81197947781779,-35.7477541739545));
#35850=CARTESIAN_POINT('Ctrl Pts',(33.4663254823227,0.834162056159859,-36.0010457997609));
#35851=CARTESIAN_POINT('Ctrl Pts',(33.4855665553264,0.879653442348478,-36.5075046045366));
#35852=CARTESIAN_POINT('Ctrl Pts',(33.518976770033,0.962053734946922,-37.3914520772919));
#35853=CARTESIAN_POINT('Ctrl Pts',(33.5824998346805,1.13533938921436,-39.1543029953479));
#35854=CARTESIAN_POINT('Ctrl Pts',(33.6228063368028,1.29268351555625,-40.6638351678756));
#35855=CARTESIAN_POINT('Ctrl Pts',(33.637460801882,1.40823476310828,-41.8007123511776));
#35856=CARTESIAN_POINT('Ctrl Pts',(33.6411996738958,1.43179248615386,-42.0387259261224));
#35857=CARTESIAN_POINT('Ctrl Pts',(33.6461063511285,1.46536011018525,-42.4061764186738));
#35858=CARTESIAN_POINT('Ctrl Pts',(33.6506102473115,1.49707490134403,-42.7747444908318));
#35859=CARTESIAN_POINT('Ctrl Pts',(33.6557553728041,1.5380045112777,-43.2721482774162));
#35860=CARTESIAN_POINT('Ctrl Pts',(33.6604262132191,1.58789030168531,-43.9018736202697));
#35861=CARTESIAN_POINT('Ctrl Pts',(33.6622567248897,1.65073055016276,-44.6708978424729));
#35862=CARTESIAN_POINT('Ctrl Pts',(33.6598108879441,1.70982232506804,-45.3219908902517));
#35863=CARTESIAN_POINT('Ctrl Pts',(33.6548067440503,1.76380021439561,-45.8487647704021));
#35864=CARTESIAN_POINT('Ctrl Pts',(33.649419920791,1.80832894359961,-46.2467602469543));
#35865=CARTESIAN_POINT('Ctrl Pts',(33.6422362058874,1.85759769357008,-46.6475979770163));
#35866=CARTESIAN_POINT('Ctrl Pts',(33.6299889594092,1.93059838524708,-47.1857555957972));
#35867=CARTESIAN_POINT('Ctrl Pts',(33.61768960664,1.99458607735694,-47.5934589947759));
#35868=CARTESIAN_POINT('Ctrl Pts',(33.6027138623418,2.0665714935698,-48.0050566158937));
#35869=CARTESIAN_POINT('Ctrl Pts',(33.5905238784982,2.12049129158493,-48.2930096977021));
#35870=CARTESIAN_POINT('Ctrl Pts',(33.5641889649566,2.2394387576737,-48.8517379400952));
#35871=CARTESIAN_POINT('Ctrl Pts',(33.5121412511527,2.47469649448957,-49.8106673127384));
#35872=CARTESIAN_POINT('Ctrl Pts',(33.4296895252064,2.8540314627126,-51.116041684853));
#35873=CARTESIAN_POINT('Ctrl Pts',(33.3323497449342,3.28708577780795,-52.5895297498466));
#35874=CARTESIAN_POINT('Ctrl Pts',(33.2724679931295,3.50437584515634,-53.5024828340018));
#35875=CARTESIAN_POINT('Ctrl Pts',(33.2353734282258,3.603793727542,-54.048495646057));
#35876=CARTESIAN_POINT('Ctrl Pts',(33.2186887677575,3.64206286670646,-54.2765843642304));
#35877=CARTESIAN_POINT('Ctrl Pts',(33.1812690437434,3.70762601944653,-54.736104266661));
#35878=CARTESIAN_POINT('Ctrl Pts',(33.1052759700434,3.79981335244846,-55.5599817959337));
#35879=CARTESIAN_POINT('Ctrl Pts',(32.9199074710695,3.92750431317271,-57.275958678648));
#35880=CARTESIAN_POINT('Ctrl Pts',(32.7437274613203,4.07114128831046,-58.8721394454319));
#35881=CARTESIAN_POINT('Ctrl Pts',(32.6639824581932,4.30556649985029,-60.0493336085321));
#35882=CARTESIAN_POINT('Ctrl Pts',(32.6550523999368,4.33055841229675,-60.174987850211));
#35883=CARTESIAN_POINT('Ctrl Pts',(32.63768717107,4.38337873383551,-60.4366839407282));
#35884=CARTESIAN_POINT('Ctrl Pts',(32.6095138887291,4.47691107068816,-60.8910885081208));
#35885=CARTESIAN_POINT('Ctrl Pts',(32.5608295965856,4.67430312186353,-61.8088050207747));
#35886=CARTESIAN_POINT('Ctrl Pts',(32.5207812011383,4.92588842360142,-62.8654352013746));
#35887=CARTESIAN_POINT('Ctrl Pts',(32.4910556698706,5.21535938673554,-63.9289579808857));
#35888=CARTESIAN_POINT('Ctrl Pts',(32.4772375701882,5.39473052547573,-64.5283020847092));
#35889=CARTESIAN_POINT('Ctrl Pts',(32.4688275698169,5.52227196815787,-64.9280978430035));
#35890=CARTESIAN_POINT('Ctrl Pts',(32.4634077760578,5.60949149135347,-65.1946257634481));
#35891=CARTESIAN_POINT('Ctrl Pts',(32.4582349635776,5.70012474893571,-65.4611844737283));
#35892=CARTESIAN_POINT('Ctrl Pts',(32.4538496347377,5.78259031628741,-65.6943019960171));
#35893=CARTESIAN_POINT('Ctrl Pts',(32.4513753260859,5.83064584969686,-65.8274717215964));
#35894=CARTESIAN_POINT('Ctrl Pts',(32.4476902372352,5.90367903832255,-66.0271877027392));
#35895=CARTESIAN_POINT('Ctrl Pts',(32.4446685092354,5.96653900293033,-66.1935103058364));
#35896=CARTESIAN_POINT('Ctrl Pts',(32.4396698964425,6.07351165788405,-66.4689006508914));
#35897=CARTESIAN_POINT('Ctrl Pts',(32.4351018946248,6.19225514219894,-66.7627262695961));
#35898=CARTESIAN_POINT('Ctrl Pts',(32.4283028677017,6.43897617099595,-67.332382514625));
#35899=CARTESIAN_POINT('Ctrl Pts',(32.4217165914204,6.89862124151141,-68.3053596401035));
#35900=CARTESIAN_POINT('Ctrl Pts',(32.4236746454016,7.88786118882068,-70.1508134268032));
#35901=CARTESIAN_POINT('Ctrl Pts',(32.435278994445,8.74876384190553,-71.6120343198423));
#35902=CARTESIAN_POINT('Ctrl Pts',(32.435038763498,9.30747710662932,-72.6747612841359));
#35903=CARTESIAN_POINT('Ctrl Pts',(32.4349002184836,9.44282627201533,-72.9317827884244));
#35904=CARTESIAN_POINT('Ctrl Pts',(32.4347384980485,9.70782501925712,-73.4337510341519));
#35905=CARTESIAN_POINT('Ctrl Pts',(32.4346157241301,10.042276972751,-74.0652069607757));
#35906=CARTESIAN_POINT('Ctrl Pts',(32.4345986484725,10.4430286253234,-74.819189488878));
#35907=CARTESIAN_POINT('Ctrl Pts',(32.434728949116,11.2461960650344,-76.3266732241031));
#35908=CARTESIAN_POINT('Ctrl Pts',(32.4350650841433,11.9155592004831,-77.5788728671257));
#35909=CARTESIAN_POINT('Ctrl Pts',(32.435094458272,12.8833188081073,-79.3990793477341));
#35910=CARTESIAN_POINT('Ctrl Pts',(32.4350926663251,13.3206560018545,-80.2216501046058));
#35911=CARTESIAN_POINT('Ctrl Pts',(32.4350926663252,13.757177589244,-81.042627806704));
#35912=CARTESIAN_POINT('Ctrl Pts',(34.3348665008137,0.0296348787660989,
24.8306202558209));
#35913=CARTESIAN_POINT('Ctrl Pts',(34.3349702061934,0.029637068735487,24.7817404888869));
#35914=CARTESIAN_POINT('Ctrl Pts',(34.3350789693011,0.0296393640675755,
24.7328617643363));
#35915=CARTESIAN_POINT('Ctrl Pts',(34.3363633825367,0.0296665120963467,
24.1822484301607));
#35916=CARTESIAN_POINT('Ctrl Pts',(34.337350759526,0.0296933097880433,23.1781110319428));
#35917=CARTESIAN_POINT('Ctrl Pts',(34.3396499777359,0.0297587991764213,
21.1695008410527));
#35918=CARTESIAN_POINT('Ctrl Pts',(34.3481981529855,0.0299396228229842,
19.6653379702371));
#35919=CARTESIAN_POINT('Ctrl Pts',(34.3663127117265,0.0302934347281393,
18.4142822305806));
#35920=CARTESIAN_POINT('Ctrl Pts',(34.3750003475134,0.0304658073261087,
17.9114388071362));
#35921=CARTESIAN_POINT('Ctrl Pts',(34.3968154838019,0.0309034790139605,
16.907432448917));
#35922=CARTESIAN_POINT('Ctrl Pts',(34.4436049017858,0.0318414145430069,
15.1536361704964));
#35923=CARTESIAN_POINT('Ctrl Pts',(34.4880473484764,0.0326934662284305,
13.6519888957546));
#35924=CARTESIAN_POINT('Ctrl Pts',(34.5158961770517,0.0331547802921301,
12.397621207677));
#35925=CARTESIAN_POINT('Ctrl Pts',(34.5272788503318,0.0333352448613346,
11.8967116582713));
#35926=CARTESIAN_POINT('Ctrl Pts',(34.5504784914328,0.033677032523816,10.8949340302363));
#35927=CARTESIAN_POINT('Ctrl Pts',(34.5906219851948,0.0342144269964047,
9.14146183505485));
#35928=CARTESIAN_POINT('Ctrl Pts',(34.6187852923028,0.034531507353301,7.63620565117921));
#35929=CARTESIAN_POINT('Ctrl Pts',(34.6313071543681,0.0346614975994032,
6.50520241718005));
#35930=CARTESIAN_POINT('Ctrl Pts',(34.6339101122789,0.0346805129074275,
6.25507094287352));
#35931=CARTESIAN_POINT('Ctrl Pts',(34.6384775201399,0.0346848860572032,
5.75405063514034));
#35932=CARTESIAN_POINT('Ctrl Pts',(34.6448529888665,0.034618796147095,4.87576992215105));
#35933=CARTESIAN_POINT('Ctrl Pts',(34.6515912826497,0.0343121150855791,
3.11541901871874));
#35934=CARTESIAN_POINT('Ctrl Pts',(34.6486547883739,0.0341545534559291,
1.60818548078039));
#35935=CARTESIAN_POINT('Ctrl Pts',(34.6439423833365,0.0344775417838192,
0.548062255281211));
#35936=CARTESIAN_POINT('Ctrl Pts',(34.6433235709926,0.0345201216650427,
0.421770541410198));
#35937=CARTESIAN_POINT('Ctrl Pts',(34.6418698505304,0.0346199270201468,
0.169421305589011));
#35938=CARTESIAN_POINT('Ctrl Pts',(34.6387866018264,0.0348308422103272,
-0.271667565664166));
#35939=CARTESIAN_POINT('Ctrl Pts',(34.6330112099306,0.0352194887939851,
-0.900405073948883));
#35940=CARTESIAN_POINT('Ctrl Pts',(34.6244098621842,0.0357828305244157,
-1.65315227382485));
#35941=CARTESIAN_POINT('Ctrl Pts',(34.6114362072505,0.0365964720905593,
-2.65509310379257));
#35942=CARTESIAN_POINT('Ctrl Pts',(34.5937070812663,0.0376214045821537,
-3.90548388247732));
#35943=CARTESIAN_POINT('Ctrl Pts',(34.5807623271108,0.0381958727371875,
-4.90603699346939));
#35944=CARTESIAN_POINT('Ctrl Pts',(34.5739306797211,0.0384004064543149,
-5.53236276681657));
#35945=CARTESIAN_POINT('Ctrl Pts',(34.5712035777894,0.0385355389098031,
-5.78398927199619));
#35946=CARTESIAN_POINT('Ctrl Pts',(34.5657823899225,0.0389715066872898,
-6.28674790375234));
#35947=CARTESIAN_POINT('Ctrl Pts',(34.5563821271522,0.0400579145688246,
-7.16680494613018));
#35948=CARTESIAN_POINT('Ctrl Pts',(34.5432213468392,0.0418916352723083,
-8.42263682791367));
#35949=CARTESIAN_POINT('Ctrl Pts',(34.5304281853659,0.0423755989149951,
-9.67418519311426));
#35950=CARTESIAN_POINT('Ctrl Pts',(34.5216736231272,0.0410948990578466,
-10.5464833526537));
#35951=CARTESIAN_POINT('Ctrl Pts',(34.5167287269536,0.0397704858090913,
-11.0436474668148));
#35952=CARTESIAN_POINT('Ctrl Pts',(34.5142776957149,0.0388885449217639,
-11.2917836956804));
#35953=CARTESIAN_POINT('Ctrl Pts',(34.512438749955,0.0381334687157137,-11.4784120208249));
#35954=CARTESIAN_POINT('Ctrl Pts',(34.5110693944478,0.0375076169622718,
-11.6015276034163));
#35955=CARTESIAN_POINT('Ctrl Pts',(34.5078499703665,0.0358175810326835,
-11.849203928751));
#35956=CARTESIAN_POINT('Ctrl Pts',(34.5010910795936,0.03181512375827,-12.2823387512624));
#35957=CARTESIAN_POINT('Ctrl Pts',(34.4792962544431,0.0171493363518133,
-13.3990847781187));
#35958=CARTESIAN_POINT('Ctrl Pts',(34.4501747289077,-0.00563669577787649,
-14.6505064305469));
#35959=CARTESIAN_POINT('Ctrl Pts',(34.4402911621688,-0.0163880090013641,
-15.9220705631234));
#35960=CARTESIAN_POINT('Ctrl Pts',(34.4421816827344,-0.0172553614217765,
-16.5633264679564));
#35961=CARTESIAN_POINT('Ctrl Pts',(34.4489435583318,-0.0142978400379119,
-17.0800094717923));
#35962=CARTESIAN_POINT('Ctrl Pts',(34.4542793572371,-0.0114392291676308,
-17.3396666946536));
#35963=CARTESIAN_POINT('Ctrl Pts',(34.4590621679773,-0.00872845323497167,
-17.5339367992568));
#35964=CARTESIAN_POINT('Ctrl Pts',(34.4624250714993,-0.00693217023133912,
-17.6568219591938));
#35965=CARTESIAN_POINT('Ctrl Pts',(34.4699245154061,-0.00339418588522034,
-17.9063737364449));
#35966=CARTESIAN_POINT('Ctrl Pts',(34.4785499941884,0.000139553048910618,
-18.1554151286434));
#35967=CARTESIAN_POINT('Ctrl Pts',(34.4881981477845,0.00374441972305012,
-18.4058266429038));
#35968=CARTESIAN_POINT('Ctrl Pts',(34.4946424647782,0.00605320969936596,
-18.5624954125497));
#35969=CARTESIAN_POINT('Ctrl Pts',(34.5000341941741,0.00794431257695288,
-18.688069890545));
#35970=CARTESIAN_POINT('Ctrl Pts',(34.5055811412055,0.00986886720126,-18.8137530033974));
#35971=CARTESIAN_POINT('Ctrl Pts',(34.5214679358394,0.0153379856010082,
-19.1599197917746));
#35972=CARTESIAN_POINT('Ctrl Pts',(34.5507640173886,0.0253466481217635,
-19.7292428735243));
#35973=CARTESIAN_POINT('Ctrl Pts',(34.6108128715338,0.0490990947697404,
-20.7501383806793));
#35974=CARTESIAN_POINT('Ctrl Pts',(34.6988121604481,0.0959009703686677,
-22.0439214278242));
#35975=CARTESIAN_POINT('Ctrl Pts',(34.7768065662565,0.16854409880932,-23.0992880475148));
#35976=CARTESIAN_POINT('Ctrl Pts',(34.8247270237116,0.230398196361508,-23.7634141199022));
#35977=CARTESIAN_POINT('Ctrl Pts',(34.8445161595343,0.257282454815504,-24.0322039773686));
#35978=CARTESIAN_POINT('Ctrl Pts',(34.8866107950697,0.31890337558203,-24.5626599722539));
#35979=CARTESIAN_POINT('Ctrl Pts',(34.9654040907167,0.445760973026535,-25.4840804706916));
#35980=CARTESIAN_POINT('Ctrl Pts',(35.0836114628791,0.668955182248936,-26.7718438871875));
#35981=CARTESIAN_POINT('Ctrl Pts',(35.2107424432564,0.959877924312591,-28.2700879809425));
#35982=CARTESIAN_POINT('Ctrl Pts',(35.2756202929575,1.13589941731545,-29.2363892005653));
#35983=CARTESIAN_POINT('Ctrl Pts',(35.3049350040518,1.22055555336939,-29.7712659446889));
#35984=CARTESIAN_POINT('Ctrl Pts',(35.311152113083,1.23966678302167,-29.8954325847102));
#35985=CARTESIAN_POINT('Ctrl Pts',(35.3231424719885,1.27717133207363,-30.141072757404));
#35986=CARTESIAN_POINT('Ctrl Pts',(35.3427475768565,1.34168941918445,-30.5731204623188));
#35987=CARTESIAN_POINT('Ctrl Pts',(35.3770722102907,1.46610252274959,-31.4386112933145));
#35988=CARTESIAN_POINT('Ctrl Pts',(35.4070489402869,1.59963645464085,-32.4333294077523));
#35989=CARTESIAN_POINT('Ctrl Pts',(35.4312403420351,1.72847555459606,-33.4310363885322));
#35990=CARTESIAN_POINT('Ctrl Pts',(35.4472477001023,1.8238550384678,-34.1806796044288));
#35991=CARTESIAN_POINT('Ctrl Pts',(35.4619111545767,1.91895541470026,-34.9312137346278));
#35992=CARTESIAN_POINT('Ctrl Pts',(35.4712334901812,1.98293013095225,-35.4319905802502));
#35993=CARTESIAN_POINT('Ctrl Pts',(35.478233773719,2.03153925195565,-35.808572373394));
#35994=CARTESIAN_POINT('Ctrl Pts',(35.4830531735356,2.06392218397385,-36.0584646920786));
#35995=CARTESIAN_POINT('Ctrl Pts',(35.4926802077051,2.12861386739761,-36.5589901333385));
#35996=CARTESIAN_POINT('Ctrl Pts',(35.5094871138481,2.24105474199066,-37.4330062845498));
#35997=CARTESIAN_POINT('Ctrl Pts',(35.5408576479142,2.46234762716514,-39.1789748004921));
#35998=CARTESIAN_POINT('Ctrl Pts',(35.5572421876025,2.64112381329902,-40.6782951369843));
#35999=CARTESIAN_POINT('Ctrl Pts',(35.5567624571101,2.76578051166555,-41.8093748197993));
#36000=CARTESIAN_POINT('Ctrl Pts',(35.5571853301886,2.79177993029111,-42.0496317037747));
#36001=CARTESIAN_POINT('Ctrl Pts',(35.5573263029132,2.82889503479657,-42.4176035690288));
#36002=CARTESIAN_POINT('Ctrl Pts',(35.5572386302164,2.86409255204442,-42.7863815460673));
#36003=CARTESIAN_POINT('Ctrl Pts',(35.5564822691865,2.90921026862981,-43.2824239859168));
#36004=CARTESIAN_POINT('Ctrl Pts',(35.5541893094433,2.96307988572064,-43.9082524122556));
#36005=CARTESIAN_POINT('Ctrl Pts',(35.5482826496532,3.02703653127083,-44.6689075116179));
#36006=CARTESIAN_POINT('Ctrl Pts',(35.5398959644219,3.08256710346372,-45.3102081014407));
#36007=CARTESIAN_POINT('Ctrl Pts',(35.5305831733313,3.13009686860969,-45.8276045672095));
#36008=CARTESIAN_POINT('Ctrl Pts',(35.5221159032968,3.16774298696779,-46.2178189894755));
#36009=CARTESIAN_POINT('Ctrl Pts',(35.512004132919,3.20784441258354,-46.6101715258913));
#36010=CARTESIAN_POINT('Ctrl Pts',(35.4960988966223,3.26521600069479,-47.1362032751428));
#36011=CARTESIAN_POINT('Ctrl Pts',(35.4811021734307,3.31335286374751,-47.5338839460087));
#36012=CARTESIAN_POINT('Ctrl Pts',(35.4635967259766,3.36607212993744,-47.9351749220645));
#36013=CARTESIAN_POINT('Ctrl Pts',(35.4494898736546,3.4056746116725,-48.2179946905193));
#36014=CARTESIAN_POINT('Ctrl Pts',(35.4182032525292,3.49275120818139,-48.7674332494914));
#36015=CARTESIAN_POINT('Ctrl Pts',(35.3545447183938,3.6640815037813,-49.7144307196596));
#36016=CARTESIAN_POINT('Ctrl Pts',(35.2471415986055,3.93550743444783,-51.0097126548988));
#36017=CARTESIAN_POINT('Ctrl Pts',(35.1102158736415,4.22549151210901,-52.4694949292696));
#36018=CARTESIAN_POINT('Ctrl Pts',(35.0224921908637,4.34893489480374,-53.3657555146103));
#36019=CARTESIAN_POINT('Ctrl Pts',(34.9712095732623,4.39391473679624,-53.8990101827058));
#36020=CARTESIAN_POINT('Ctrl Pts',(34.9500808458707,4.40684644048079,-54.1095680986356));
#36021=CARTESIAN_POINT('Ctrl Pts',(34.9033724169422,4.42080872818289,-54.5443012692132));
#36022=CARTESIAN_POINT('Ctrl Pts',(34.8130378502953,4.41642697910621,-55.3300647584961));
#36023=CARTESIAN_POINT('Ctrl Pts',(34.6117438977039,4.34012314350154,-57.0146657734164));
#36024=CARTESIAN_POINT('Ctrl Pts',(34.4531051253727,4.30922070393653,-58.6662666751489));
#36025=CARTESIAN_POINT('Ctrl Pts',(34.3894975143158,4.47950355174856,-59.9180228144314));
#36026=CARTESIAN_POINT('Ctrl Pts',(34.3823210415351,4.49747234506587,-60.0477815322125));
#36027=CARTESIAN_POINT('Ctrl Pts',(34.3693125647404,4.53678421981033,-60.3200171731233));
#36028=CARTESIAN_POINT('Ctrl Pts',(34.35020497003,4.60894769444198,-60.7904494162606));
#36029=CARTESIAN_POINT('Ctrl Pts',(34.3249474995229,4.77107317620435,-61.7371283591797));
#36030=CARTESIAN_POINT('Ctrl Pts',(34.3191689863112,4.99662311074608,-62.8169964039174));
#36031=CARTESIAN_POINT('Ctrl Pts',(34.3234893783647,5.26791092913627,-63.8949689569154));
#36032=CARTESIAN_POINT('Ctrl Pts',(34.327336292537,5.43868107676422,-64.4990442638172));
#36033=CARTESIAN_POINT('Ctrl Pts',(34.3295138860271,5.56055800279895,-64.9006753433086));
#36034=CARTESIAN_POINT('Ctrl Pts',(34.330800849446,5.64397173868575,-65.1680715349568));
#36035=CARTESIAN_POINT('Ctrl Pts',(34.3317418024156,5.73071023424241,-65.4350013761785));
#36036=CARTESIAN_POINT('Ctrl Pts',(34.3321037329367,5.80955416821317,-65.6680022388863));
#36037=CARTESIAN_POINT('Ctrl Pts',(34.3321557140039,5.85546437902845,-65.8009841429503));
#36038=CARTESIAN_POINT('Ctrl Pts',(34.3320677894955,5.92519716045461,-66.0003057198109));
#36039=CARTESIAN_POINT('Ctrl Pts',(34.331624201174,5.98511440238383,-66.1660442121481));
#36040=CARTESIAN_POINT('Ctrl Pts',(34.3302806170565,6.08691727314271,-66.4403221129988));
#36041=CARTESIAN_POINT('Ctrl Pts',(34.3289626032204,6.20369935850024,-66.7407215332001));
#36042=CARTESIAN_POINT('Ctrl Pts',(34.3270621904633,6.44695750743629,-67.3177229835005));
#36043=CARTESIAN_POINT('Ctrl Pts',(34.3252412284561,6.90584758899664,-68.3028276387302));
#36044=CARTESIAN_POINT('Ctrl Pts',(34.3259284736756,7.90462355977505,-70.1596836659473));
#36045=CARTESIAN_POINT('Ctrl Pts',(34.3296133593729,8.77639942584956,-71.6192787849307));
#36046=CARTESIAN_POINT('Ctrl Pts',(34.3304097572867,9.33027438548443,-72.6734212274245));
#36047=CARTESIAN_POINT('Ctrl Pts',(34.3303710936354,9.46590328165915,-72.9310976231889));
#36048=CARTESIAN_POINT('Ctrl Pts',(34.3304069107005,9.73071077115545,-73.4328814476757));
#36049=CARTESIAN_POINT('Ctrl Pts',(34.3303857676624,10.0652916277749,-74.0647109462501));
#36050=CARTESIAN_POINT('Ctrl Pts',(34.3303712375336,10.466065257165,-74.8187519248144));
#36051=CARTESIAN_POINT('Ctrl Pts',(34.3303065315425,11.2694354886003,-76.3264752362663));
#36052=CARTESIAN_POINT('Ctrl Pts',(34.3302458442975,11.9390055802922,-77.5787656056257));
#36053=CARTESIAN_POINT('Ctrl Pts',(34.3302832165028,12.906702086019,-79.3988760800469));
#36054=CARTESIAN_POINT('Ctrl Pts',(34.330266902442,13.3440986555018,-80.2215709003871));
#36055=CARTESIAN_POINT('Ctrl Pts',(34.3302669024419,13.7806202428913,-81.0425486024853));
#36056=CARTESIAN_POINT('Ctrl Pts',(36.7112167699881,0.0846744253985972,
24.8306211802992));
#36057=CARTESIAN_POINT('Ctrl Pts',(36.7113270504777,0.0846781747077857,
24.7817414397337));
#36058=CARTESIAN_POINT('Ctrl Pts',(36.7114427105277,0.0846821056520928,
24.7328627397048));
#36059=CARTESIAN_POINT('Ctrl Pts',(36.7128085688682,0.0847285604531195,
24.1822497915495));
#36060=CARTESIAN_POINT('Ctrl Pts',(36.7138443146183,0.0847695523576969,
23.1781129933839));
#36061=CARTESIAN_POINT('Ctrl Pts',(36.7162470894082,0.0848677714251754,
21.1695036373261));
#36062=CARTESIAN_POINT('Ctrl Pts',(36.7253377401005,0.0851771162506037,
19.6653426120806));
#36063=CARTESIAN_POINT('Ctrl Pts',(36.7446729845777,0.0858063686810513,
18.4142886437229));
#36064=CARTESIAN_POINT('Ctrl Pts',(36.7539402129429,0.0861094140584334,
17.911453453911));
#36065=CARTESIAN_POINT('Ctrl Pts',(36.7772006719368,0.0868724352925051,
16.9074529235366));
#36066=CARTESIAN_POINT('Ctrl Pts',(36.8270936504073,0.0885071349433262,
15.1536543898094));
#36067=CARTESIAN_POINT('Ctrl Pts',(36.8745711220849,0.0900371434759867,
13.6519851701514));
#36068=CARTESIAN_POINT('Ctrl Pts',(36.9044813039543,0.0909542099707382,
12.3975863726652));
#36069=CARTESIAN_POINT('Ctrl Pts',(36.9167250679747,0.0913242311819742,
11.8966642822298));
#36070=CARTESIAN_POINT('Ctrl Pts',(36.9417383482741,0.092063240256459,10.8948719891067));
#36071=CARTESIAN_POINT('Ctrl Pts',(36.9851411517665,0.0933105117943699,
9.14139175481678));
#36072=CARTESIAN_POINT('Ctrl Pts',(37.0157109083655,0.0941508000170405,
7.63616346562538));
#36073=CARTESIAN_POINT('Ctrl Pts',(37.0293146481114,0.0945177922996605,
6.50517590311963));
#36074=CARTESIAN_POINT('Ctrl Pts',(37.0321450823204,0.0945919285604579,
6.2549752058218));
#36075=CARTESIAN_POINT('Ctrl Pts',(37.0371210043897,0.0947136005399027,
5.75388196216641));
#36076=CARTESIAN_POINT('Ctrl Pts',(37.0440927319416,0.0948615796641339,
4.87551145389234));
#36077=CARTESIAN_POINT('Ctrl Pts',(37.0515786051953,0.0949413242790322,
3.11521835137205));
#36078=CARTESIAN_POINT('Ctrl Pts',(37.0486124688515,0.0947750805650604,
1.60844265176952));
#36079=CARTESIAN_POINT('Ctrl Pts',(37.0436621926746,0.0946871777363435,
0.548832801105595));
#36080=CARTESIAN_POINT('Ctrl Pts',(37.0430108702942,0.0946759195152151,
0.422629163366355));
#36081=CARTESIAN_POINT('Ctrl Pts',(37.0414755532143,0.09464995393213,0.170430001263052));
#36082=CARTESIAN_POINT('Ctrl Pts',(37.0382084476048,0.0945961612704619,
-0.2704136055817));
#36083=CARTESIAN_POINT('Ctrl Pts',(37.032064141019,0.0944958624299077,-0.898867967521424));
#36084=CARTESIAN_POINT('Ctrl Pts',(37.0228917013655,0.0943506252441615,
-1.65140654519409));
#36085=CARTESIAN_POINT('Ctrl Pts',(37.0090325596193,0.0941270031994452,
-2.65320477270874));
#36086=CARTESIAN_POINT('Ctrl Pts',(36.9900665385056,0.0938128390382973,
-3.9037394793735));
#36087=CARTESIAN_POINT('Ctrl Pts',(36.9762063761215,0.0935646684807531,
-4.90469914381444));
#36088=CARTESIAN_POINT('Ctrl Pts',(36.9688985723988,0.0934289358944953,
-5.53140686327081));
#36089=CARTESIAN_POINT('Ctrl Pts',(36.965848701232,0.0934287654566223,-5.78303194814696));
#36090=CARTESIAN_POINT('Ctrl Pts',(36.9593500591013,0.0936049220407772,
-6.28587223138632));
#36091=CARTESIAN_POINT('Ctrl Pts',(36.9471928322836,0.0942670374755707,
-7.16602446820794));
#36092=CARTESIAN_POINT('Ctrl Pts',(36.9290905609926,0.0955974956355437,
-8.4219871970132));
#36093=CARTESIAN_POINT('Ctrl Pts',(36.9140217710994,0.0958307885018514,
-9.6737200225743));
#36094=CARTESIAN_POINT('Ctrl Pts',(36.9071799781076,0.0945953441252705,
-10.5462556420091));
#36095=CARTESIAN_POINT('Ctrl Pts',(36.9046304334507,0.0933734981130456,
-11.0435563604861));
#36096=CARTESIAN_POINT('Ctrl Pts',(36.9038594745276,0.0925705463853636,
-11.2918147610355));
#36097=CARTESIAN_POINT('Ctrl Pts',(36.9034865913886,0.0918882736245058,
-11.4784038866097));
#36098=CARTESIAN_POINT('Ctrl Pts',(36.9030853075895,0.0911945798563351,
-11.5969569379139));
#36099=CARTESIAN_POINT('Ctrl Pts',(36.9017538475644,0.0887426520100996,
-11.8388538451608));
#36100=CARTESIAN_POINT('Ctrl Pts',(36.898216268949,0.0819592352586638,-12.2623810155641));
#36101=CARTESIAN_POINT('Ctrl Pts',(36.8848261987535,0.0544563126445047,
-13.3650612644444));
#36102=CARTESIAN_POINT('Ctrl Pts',(36.8682840211302,0.00873084552395717,
-14.6279437361951));
#36103=CARTESIAN_POINT('Ctrl Pts',(36.883730091319,-0.00140900409272758,
-15.9393810040082));
#36104=CARTESIAN_POINT('Ctrl Pts',(36.9023667045802,0.00738003706140011,
-16.6075952081114));
#36105=CARTESIAN_POINT('Ctrl Pts',(36.9255929932009,0.0257459947431755,
-17.1501335700735));
#36106=CARTESIAN_POINT('Ctrl Pts',(36.9402796510903,0.0393172250515568,
-17.4241536848916));
#36107=CARTESIAN_POINT('Ctrl Pts',(36.9525070144203,0.0512901224359853,
-17.629627336922));
#36108=CARTESIAN_POINT('Ctrl Pts',(36.9612358256281,0.058874478576913,-17.7579791358429));
#36109=CARTESIAN_POINT('Ctrl Pts',(36.9810617739,0.0755937029143875,-18.0191630350841));
#36110=CARTESIAN_POINT('Ctrl Pts',(37.0042360390654,0.0940605022323197,
-18.278869703191));
#36111=CARTESIAN_POINT('Ctrl Pts',(37.0303076881267,0.114621356572637,-18.5395580253906));
#36112=CARTESIAN_POINT('Ctrl Pts',(37.0477123473,0.128337099242465,-18.7023527010502));
#36113=CARTESIAN_POINT('Ctrl Pts',(37.062242949944,0.139859105139886,-18.8326902634384));
#36114=CARTESIAN_POINT('Ctrl Pts',(37.0771577820906,0.151749504377015,-18.9630256422138));
#36115=CARTESIAN_POINT('Ctrl Pts',(37.1196737131603,0.185994854980597,-19.3215789081379));
#36116=CARTESIAN_POINT('Ctrl Pts',(37.1965049267673,0.250784832961701,-19.9087167246095));
#36117=CARTESIAN_POINT('Ctrl Pts',(37.3427176726399,0.392278988510994,-20.9537561882706));
#36118=CARTESIAN_POINT('Ctrl Pts',(37.5211894329389,0.619264465501433,-22.2612597859818));
#36119=CARTESIAN_POINT('Ctrl Pts',(37.6153479218006,0.84303517672332,-23.3094150400843));
#36120=CARTESIAN_POINT('Ctrl Pts',(37.6485511709952,0.98968170088537,-23.9656518899643));
#36121=CARTESIAN_POINT('Ctrl Pts',(37.6593603790078,1.05359960825901,-24.2446617278323));
#36122=CARTESIAN_POINT('Ctrl Pts',(37.6762771025471,1.18842239777695,-24.7838187391321));
#36123=CARTESIAN_POINT('Ctrl Pts',(37.6936520642177,1.44399158749902,-25.7160586081786));
#36124=CARTESIAN_POINT('Ctrl Pts',(37.6938852682224,1.8373117640372,-26.9982673915027));
#36125=CARTESIAN_POINT('Ctrl Pts',(37.6822568333526,2.28941532283948,-28.4718897646818));
#36126=CARTESIAN_POINT('Ctrl Pts',(37.679725915953,2.54033364704782,-29.4065852634538));
#36127=CARTESIAN_POINT('Ctrl Pts',(37.6816143028183,2.65819974592193,-29.9180122945906));
#36128=CARTESIAN_POINT('Ctrl Pts',(37.6810258951326,2.68551429704461,-30.0403811154778));
#36129=CARTESIAN_POINT('Ctrl Pts',(37.6799948340348,2.73816216919017,-30.2806536350076));
#36130=CARTESIAN_POINT('Ctrl Pts',(37.6770312359342,2.82771432743439,-30.7046151956739));
#36131=CARTESIAN_POINT('Ctrl Pts',(37.6682215238293,2.99534732000716,-31.5545149542589));
#36132=CARTESIAN_POINT('Ctrl Pts',(37.6532531101359,3.16522337037743,-32.5346457195609));
#36133=CARTESIAN_POINT('Ctrl Pts',(37.6374410450317,3.32069212311533,-33.5200421450193));
#36134=CARTESIAN_POINT('Ctrl Pts',(37.6259610794996,3.43210328958448,-34.2616953089193));
#36135=CARTESIAN_POINT('Ctrl Pts',(37.6157002543297,3.54025712278262,-35.0053877406598));
#36136=CARTESIAN_POINT('Ctrl Pts',(37.6101924543024,3.61153831044084,-35.5023857947915));
#36137=CARTESIAN_POINT('Ctrl Pts',(37.606760023377,3.66533539524376,-35.8763439464447));
#36138=CARTESIAN_POINT('Ctrl Pts',(37.6049850863926,3.70058659582321,-36.1227070445535));
#36139=CARTESIAN_POINT('Ctrl Pts',(37.601894064277,3.76970638580753,-36.6174113547226));
#36140=CARTESIAN_POINT('Ctrl Pts',(37.5979645128747,3.88624829952936,-37.4812630811199));
#36141=CARTESIAN_POINT('Ctrl Pts',(37.5931988424177,4.10248825673543,-39.208965058032));
#36142=CARTESIAN_POINT('Ctrl Pts',(37.5861294903716,4.25827904016071,-40.6945331880147));
#36143=CARTESIAN_POINT('Ctrl Pts',(37.5712416805247,4.36067583335185,-41.8161547039106));
#36144=CARTESIAN_POINT('Ctrl Pts',(37.5682415240926,4.38222806105262,-42.058508857134));
#36145=CARTESIAN_POINT('Ctrl Pts',(37.5636532761775,4.41297535307706,-42.4262547841356));
#36146=CARTESIAN_POINT('Ctrl Pts',(37.5590376997491,4.44202384408049,-42.7944249851715));
#36147=CARTESIAN_POINT('Ctrl Pts',(37.5526298265626,4.47881865486102,-43.2876809894668));
#36148=CARTESIAN_POINT('Ctrl Pts',(37.5439336707566,4.52147717949122,-43.9073297117841));
#36149=CARTESIAN_POINT('Ctrl Pts',(37.5314839039231,4.568582473753,-44.6559153643209));
#36150=CARTESIAN_POINT('Ctrl Pts',(37.5186404667206,4.60545971778606,-45.2834087418635));
#36151=CARTESIAN_POINT('Ctrl Pts',(37.506365694386,4.63423104404996,-45.7874623348475));
#36152=CARTESIAN_POINT('Ctrl Pts',(37.4960182599751,4.65559735298739,-46.1664926271542));
#36153=CARTESIAN_POINT('Ctrl Pts',(37.4843850602633,4.67692906601873,-46.5464584886975));
#36154=CARTESIAN_POINT('Ctrl Pts',(37.4669493900572,4.70558812969249,-47.0543505925715));
#36155=CARTESIAN_POINT('Ctrl Pts',(37.4514713193433,4.72756749779263,-47.4364875093737));
#36156=CARTESIAN_POINT('Ctrl Pts',(37.4339738194798,4.75041997909752,-47.8208376258834));
#36157=CARTESIAN_POINT('Ctrl Pts',(37.4208222272838,4.76784326333416,-48.0905868022626));
#36158=CARTESIAN_POINT('Ctrl Pts',(37.3910858757268,4.8058890086723,-48.6171456385995));
#36159=CARTESIAN_POINT('Ctrl Pts',(37.330309388502,4.88002773191839,-49.5284249880321));
#36160=CARTESIAN_POINT('Ctrl Pts',(37.2245928522151,4.99256283022992,-50.7853111888859));
#36161=CARTESIAN_POINT('Ctrl Pts',(37.086863900826,5.09644701465494,-52.2179456501514));
#36162=CARTESIAN_POINT('Ctrl Pts',(37.0032964705299,5.11897727890018,-53.1156669284226));
#36163=CARTESIAN_POINT('Ctrl Pts',(36.9591174381978,5.11110123786269,-53.6589488128304));
#36164=CARTESIAN_POINT('Ctrl Pts',(36.9409989107881,5.10299449829485,-53.8508893329867));
#36165=CARTESIAN_POINT('Ctrl Pts',(36.9045711625135,5.07293272516291,-54.268007339853));
#36166=CARTESIAN_POINT('Ctrl Pts',(36.8418253338402,4.98485325407387,-55.0312941587319));
#36167=CARTESIAN_POINT('Ctrl Pts',(36.7330788072467,4.71052689193802,-56.7257680108773));
#36168=CARTESIAN_POINT('Ctrl Pts',(36.6713543917833,4.46372288982941,-58.4421745126765));
#36169=CARTESIAN_POINT('Ctrl Pts',(36.6472973413736,4.55545974642122,-59.7852181242117));
#36170=CARTESIAN_POINT('Ctrl Pts',(36.6446924290674,4.56604719088446,-59.9247926927141));
#36171=CARTESIAN_POINT('Ctrl Pts',(36.6405006918235,4.59158900718835,-60.2162269454623));
#36172=CARTESIAN_POINT('Ctrl Pts',(36.6357573764282,4.64490957412634,-60.7173312098255));
#36173=CARTESIAN_POINT('Ctrl Pts',(36.6354347937168,4.78613690861304,-61.715152217054));
#36174=CARTESIAN_POINT('Ctrl Pts',(36.6504647026249,5.0177553381898,-62.8302318735079));
#36175=CARTESIAN_POINT('Ctrl Pts',(36.6701612909345,5.30491322392381,-63.9216539281145));
#36176=CARTESIAN_POINT('Ctrl Pts',(36.6811085561042,5.48450406800392,-64.5254323194787));
#36177=CARTESIAN_POINT('Ctrl Pts',(36.6875824323416,5.61060406842826,-64.9237425967269));
#36178=CARTESIAN_POINT('Ctrl Pts',(36.6916331850297,5.69628909573889,-65.1880995201401));
#36179=CARTESIAN_POINT('Ctrl Pts',(36.6952034565167,5.78432060322668,-65.4508024646126));
#36180=CARTESIAN_POINT('Ctrl Pts',(36.6977886480399,5.86316279414461,-65.6790619012919));
#36181=CARTESIAN_POINT('Ctrl Pts',(36.6990931550773,5.90870770418195,-65.8090432858565));
#36182=CARTESIAN_POINT('Ctrl Pts',(36.7008684362681,5.97751322044775,-66.0035864232181));
#36183=CARTESIAN_POINT('Ctrl Pts',(36.7019491948177,6.03580673631429,-66.1647301238399));
#36184=CARTESIAN_POINT('Ctrl Pts',(36.7031125057773,6.1336845974579,-66.4308883263072));
#36185=CARTESIAN_POINT('Ctrl Pts',(36.7038419183543,6.25108170444066,-66.7354276678796));
#36186=CARTESIAN_POINT('Ctrl Pts',(36.7049756302362,6.49357344121451,-67.31321041894));
#36187=CARTESIAN_POINT('Ctrl Pts',(36.7057176274359,6.95359681117788,-68.3024739392939));
#36188=CARTESIAN_POINT('Ctrl Pts',(36.7042062532507,7.95644289331439,-70.1615195305834));
#36189=CARTESIAN_POINT('Ctrl Pts',(36.7020394211586,8.83232363000405,-71.6214457270801));
#36190=CARTESIAN_POINT('Ctrl Pts',(36.7036824066944,9.38521971322024,-72.67303574198));
#36191=CARTESIAN_POINT('Ctrl Pts',(36.7036499997214,9.52096894610462,-72.9307872481302));
#36192=CARTESIAN_POINT('Ctrl Pts',(36.703772184435,9.78578067051566,-73.4323584766922));
#36193=CARTESIAN_POINT('Ctrl Pts',(36.7037713350486,10.1204017792823,-74.06414271824));
#36194=CARTESIAN_POINT('Ctrl Pts',(36.7037513271413,10.5211079906384,-74.8180546299337));
#36195=CARTESIAN_POINT('Ctrl Pts',(36.7035899613343,11.3242967756186,-76.3256604793899));
#36196=CARTESIAN_POINT('Ctrl Pts',(36.7033688472319,11.9937053006823,-77.578181963688));
#36197=CARTESIAN_POINT('Ctrl Pts',(36.703426617587,12.9615751163495,-79.3986755482907));
#36198=CARTESIAN_POINT('Ctrl Pts',(36.7033971809566,13.398941260589,-80.2213447601627));
#36199=CARTESIAN_POINT('Ctrl Pts',(36.7033971809565,13.8354628479784,-81.042322462261));
#36200=CARTESIAN_POINT('Ctrl Pts',(39.0888044266541,0.18001366521702,24.8306577616938));
#36201=CARTESIAN_POINT('Ctrl Pts',(39.088921603972,0.180018450330286,24.7817791815388));
#36202=CARTESIAN_POINT('Ctrl Pts',(39.0890444976507,0.180023467314007,24.7329016553144));
#36203=CARTESIAN_POINT('Ctrl Pts',(39.0904957807811,0.180082827660729,24.1823025865289));
#36204=CARTESIAN_POINT('Ctrl Pts',(39.091591381236,0.180114768840105,23.178184197145));
#36205=CARTESIAN_POINT('Ctrl Pts',(39.0941300425472,0.180178317661714,21.16959986221));
#36206=CARTESIAN_POINT('Ctrl Pts',(39.1037889658438,0.180575048338146,19.6654506295828));
#36207=CARTESIAN_POINT('Ctrl Pts',(39.1243579241454,0.1814843255736,18.4144015139445));
#36208=CARTESIAN_POINT('Ctrl Pts',(39.134218049248,0.181913975656292,17.9116384281828));
#36209=CARTESIAN_POINT('Ctrl Pts',(39.1589697243433,0.182982309247605,16.9076900689006));
#36210=CARTESIAN_POINT('Ctrl Pts',(39.2120662004859,0.185276856583134,15.1538859509933));
#36211=CARTESIAN_POINT('Ctrl Pts',(39.262582590445,0.187550367290034,13.6519990340237));
#36212=CARTESIAN_POINT('Ctrl Pts',(39.2943933523544,0.189141556091282,12.3973040853036));
#36213=CARTESIAN_POINT('Ctrl Pts',(39.3074164756704,0.189810834674528,11.8962594688207));
#36214=CARTESIAN_POINT('Ctrl Pts',(39.3340217961813,0.191236665964346,10.8942909995908));
#36215=CARTESIAN_POINT('Ctrl Pts',(39.3801836202682,0.193830901914628,9.14064171979857));
#36216=CARTESIAN_POINT('Ctrl Pts',(39.4126587791981,0.195783190608379,7.63555136734775));
#36217=CARTESIAN_POINT('Ctrl Pts',(39.4270720822274,0.196665431889854,6.50476503310077));
#36218=CARTESIAN_POINT('Ctrl Pts',(39.4300578896244,0.196857006372044,6.25445539718606));
#36219=CARTESIAN_POINT('Ctrl Pts',(39.4352574173322,0.197223852164122,5.75326871972413));
#36220=CARTESIAN_POINT('Ctrl Pts',(39.4424195833984,0.197815265041436,4.87478653411295));
#36221=CARTESIAN_POINT('Ctrl Pts',(39.4497248967473,0.198717316245392,3.11464776031493));
#36222=CARTESIAN_POINT('Ctrl Pts',(39.446414113801,0.198780500191082,1.60867348764858));
#36223=CARTESIAN_POINT('Ctrl Pts',(39.4418832112372,0.198236634498449,0.549912702370506));
#36224=CARTESIAN_POINT('Ctrl Pts',(39.4412881183038,0.198163774332367,0.4238385234358));
#36225=CARTESIAN_POINT('Ctrl Pts',(39.4398848802454,0.197990314496298,0.171867601864431));
#36226=CARTESIAN_POINT('Ctrl Pts',(39.4368979648691,0.197616824096262,-0.268602924693885));
#36227=CARTESIAN_POINT('Ctrl Pts',(39.431265864748,0.196911581478575,-0.896604365271294));
#36228=CARTESIAN_POINT('Ctrl Pts',(39.422825193491,0.195856232866555,-1.64880397032074));
#36229=CARTESIAN_POINT('Ctrl Pts',(39.4099826406263,0.194288855819704,-2.65032760331192));
#36230=CARTESIAN_POINT('Ctrl Pts',(39.3922023559894,0.192200604920921,-3.90095888032641));
#36231=CARTESIAN_POINT('Ctrl Pts',(39.3787476751708,0.190823568782034,-4.90238727422552));
#36232=CARTESIAN_POINT('Ctrl Pts',(39.3714100758577,0.1901561159036,-5.52939102985477));
#36233=CARTESIAN_POINT('Ctrl Pts',(39.3680558466428,0.189642076445195,-5.77731798908185));
#36234=CARTESIAN_POINT('Ctrl Pts',(39.359981910118,0.187821838661392,-6.27623871359611));
#36235=CARTESIAN_POINT('Ctrl Pts',(39.3430914959754,0.183047680568109,-7.15137509663719));
#36236=CARTESIAN_POINT('Ctrl Pts',(39.3157222785391,0.174582961782399,-8.40956360796454));
#36237=CARTESIAN_POINT('Ctrl Pts',(39.2965463492739,0.171255686152978,-9.67486595032553));
#36238=CARTESIAN_POINT('Ctrl Pts',(39.2939982741584,0.175420179906363,-10.563406034056));
#36239=CARTESIAN_POINT('Ctrl Pts',(39.296588702353,0.180221793186859,-11.0716016735842));
#36240=CARTESIAN_POINT('Ctrl Pts',(39.2993871951102,0.183532771774048,-11.325997245483));
#36241=CARTESIAN_POINT('Ctrl Pts',(39.302121938711,0.18640067801295,-11.5172370581218));
#36242=CARTESIAN_POINT('Ctrl Pts',(39.3040112231602,0.187809692523296,-11.6321437067357));
#36243=CARTESIAN_POINT('Ctrl Pts',(39.3079962810501,0.189421600017977,-11.8713598072385));
#36244=CARTESIAN_POINT('Ctrl Pts',(39.3155858132922,0.189066006906126,-12.2901555340803));
#36245=CARTESIAN_POINT('Ctrl Pts',(39.3387577077408,0.176925528543926,-13.3922563216631));
#36246=CARTESIAN_POINT('Ctrl Pts',(39.379396702992,0.152137055996183,-14.684633422449));
#36247=CARTESIAN_POINT('Ctrl Pts',(39.4445092732875,0.211426194910618,-16.0553377348217));
#36248=CARTESIAN_POINT('Ctrl Pts',(39.4835009488612,0.272356020893033,-16.7595291340688));
#36249=CARTESIAN_POINT('Ctrl Pts',(39.5186398233208,0.345587774340604,-17.3338818764406));
#36250=CARTESIAN_POINT('Ctrl Pts',(39.5374228354569,0.391497344347628,-17.6244377267164));
#36251=CARTESIAN_POINT('Ctrl Pts',(39.5518867733331,0.42961675462403,-17.8427244563372));
#36252=CARTESIAN_POINT('Ctrl Pts',(39.5621568573946,0.456200774441884,-17.9895396184138));
#36253=CARTESIAN_POINT('Ctrl Pts',(39.5849235986912,0.514329621361456,-18.2788108673388));
#36254=CARTESIAN_POINT('Ctrl Pts',(39.6107424637159,0.57959390861214,-18.5649718760519));
#36255=CARTESIAN_POINT('Ctrl Pts',(39.6389477430903,0.651132193211088,-18.8469173134216));
#36256=CARTESIAN_POINT('Ctrl Pts',(39.6574199768407,0.698304460318049,-19.0216247414068));
#36257=CARTESIAN_POINT('Ctrl Pts',(39.6726260334296,0.737409770914219,-19.1604034417413));
#36258=CARTESIAN_POINT('Ctrl Pts',(39.6880870527025,0.777395307511695,-19.2985535780004));
#36259=CARTESIAN_POINT('Ctrl Pts',(39.7315368481313,0.890845964556177,-19.6759094763723));
#36260=CARTESIAN_POINT('Ctrl Pts',(39.806426112475,1.09399290202479,-20.2792595435641));
#36261=CARTESIAN_POINT('Ctrl Pts',(39.9378740920715,1.48636765147355,-21.3147777341605));
#36262=CARTESIAN_POINT('Ctrl Pts',(40.0769022433718,1.99948303982382,-22.5469752458342));
#36263=CARTESIAN_POINT('Ctrl Pts',(40.1320094904387,2.35308133618794,-23.4873105317402));
#36264=CARTESIAN_POINT('Ctrl Pts',(40.142345779399,2.53113905762304,-24.0635136067293));
#36265=CARTESIAN_POINT('Ctrl Pts',(40.1400310526758,2.60755111479133,-24.3237713721114));
#36266=CARTESIAN_POINT('Ctrl Pts',(40.1308750507945,2.75349251735673,-24.8250400766174));
#36267=CARTESIAN_POINT('Ctrl Pts',(40.09763032855,3.00245212058905,-25.7090011208127));
#36268=CARTESIAN_POINT('Ctrl Pts',(40.0180962966849,3.33162945615507,-26.9560340181101));
#36269=CARTESIAN_POINT('Ctrl Pts',(39.902796621017,3.67815510636774,-28.4274121422462));
#36270=CARTESIAN_POINT('Ctrl Pts',(39.8343343846314,3.86829718954062,-29.379789457373));
#36271=CARTESIAN_POINT('Ctrl Pts',(39.804782197237,3.96216256771703,-29.9060565264981));
#36272=CARTESIAN_POINT('Ctrl Pts',(39.7980373400526,3.9828073368703,-30.0247988928929));
#36273=CARTESIAN_POINT('Ctrl Pts',(39.7841979689039,4.0223365292869,-30.2618473420464));
#36274=CARTESIAN_POINT('Ctrl Pts',(39.7589815634636,4.08744330929229,-30.678515203839));
#36275=CARTESIAN_POINT('Ctrl Pts',(39.7051855743335,4.20250038485936,-31.516812460355));
#36276=CARTESIAN_POINT('Ctrl Pts',(39.6381570765487,4.30598886780511,-32.4869174834327));
#36277=CARTESIAN_POINT('Ctrl Pts',(39.5706475585584,4.394788911564,-33.4685874803531));
#36278=CARTESIAN_POINT('Ctrl Pts',(39.5211677313474,4.45745183458457,-34.2107164143837));
#36279=CARTESIAN_POINT('Ctrl Pts',(39.4742297070753,4.51953514291641,-34.9585969492648));
#36280=CARTESIAN_POINT('Ctrl Pts',(39.4456483829112,4.56282399841279,-35.4611444533383));
#36281=CARTESIAN_POINT('Ctrl Pts',(39.4255847884175,4.59689962044293,-35.8402485675263));
#36282=CARTESIAN_POINT('Ctrl Pts',(39.4128475749602,4.61846189298307,-36.0852973690997));
#36283=CARTESIAN_POINT('Ctrl Pts',(39.3882931019907,4.66081433303966,-36.5800450924851));
#36284=CARTESIAN_POINT('Ctrl Pts',(39.3481419729083,4.73145168651063,-37.442542601468));
#36285=CARTESIAN_POINT('Ctrl Pts',(39.2768214004295,4.86023949916803,-39.1681386386344));
#36286=CARTESIAN_POINT('Ctrl Pts',(39.2248526929345,4.95191552713248,-40.6505048686668));
#36287=CARTESIAN_POINT('Ctrl Pts',(39.1845302849585,5.01293498501988,-41.7695811407451));
#36288=CARTESIAN_POINT('Ctrl Pts',(39.1757514004488,5.02577818599023,-42.0138900949182));
#36289=CARTESIAN_POINT('Ctrl Pts',(39.1628491891999,5.0440109556031,-42.3827068030056));
#36290=CARTESIAN_POINT('Ctrl Pts',(39.1502379767333,5.06115492093622,-42.751832091601));
#36291=CARTESIAN_POINT('Ctrl Pts',(39.1338144037273,5.08275736157524,-43.2453271230115));
#36292=CARTESIAN_POINT('Ctrl Pts',(39.1140240080415,5.10757619139148,-43.8638896754156));
#36293=CARTESIAN_POINT('Ctrl Pts',(39.091489653487,5.13464443295976,-44.6086804678692));
#36294=CARTESIAN_POINT('Ctrl Pts',(39.0737405500269,5.15559279761439,-45.2309635386264));
#36295=CARTESIAN_POINT('Ctrl Pts',(39.0600981040902,5.17176317841913,-45.7295320218957));
#36296=CARTESIAN_POINT('Ctrl Pts',(39.0501791060971,5.18371745533596,-46.1037852207575));
#36297=CARTESIAN_POINT('Ctrl Pts',(39.0405715239866,5.19559935655028,-46.4782873467315));
#36298=CARTESIAN_POINT('Ctrl Pts',(39.0281533890905,5.21149689504948,-46.9779392016722));
#36299=CARTESIAN_POINT('Ctrl Pts',(39.0193798005833,5.22362506194546,-47.3527953477327));
#36300=CARTESIAN_POINT('Ctrl Pts',(39.0108595472227,5.2361784215474,-47.728985458393));
#36301=CARTESIAN_POINT('Ctrl Pts',(39.005096807157,5.24605595530727,-47.9922131094468));
#36302=CARTESIAN_POINT('Ctrl Pts',(38.9937112535453,5.2687691243098,-48.5072542803165));
#36303=CARTESIAN_POINT('Ctrl Pts',(38.974450496436,5.31479689353639,-49.4003997772548));
#36304=CARTESIAN_POINT('Ctrl Pts',(38.9507961094573,5.38469715282765,-50.6399290110756));
#36305=CARTESIAN_POINT('Ctrl Pts',(38.9332314534559,5.4365038769883,-52.0730062175913));
#36306=CARTESIAN_POINT('Ctrl Pts',(38.9309692503806,5.42542938037497,-52.9896159479058));
#36307=CARTESIAN_POINT('Ctrl Pts',(38.9329698345153,5.39801919326263,-53.5501379417846));
#36308=CARTESIAN_POINT('Ctrl Pts',(38.9340646511458,5.384840725695,-53.7411566584974));
#36309=CARTESIAN_POINT('Ctrl Pts',(38.9385147088793,5.34116348643744,-54.1628515294699));
#36310=CARTESIAN_POINT('Ctrl Pts',(38.9513538843665,5.2250017558252,-54.9345356672974));
#36311=CARTESIAN_POINT('Ctrl Pts',(38.9924301618096,4.87821670055742,-56.6482573136251));
#36312=CARTESIAN_POINT('Ctrl Pts',(39.034695446014,4.56049109913903,-58.3762550348018));
#36313=CARTESIAN_POINT('Ctrl Pts',(39.0475405283856,4.62352423934888,-59.7440668955185));
#36314=CARTESIAN_POINT('Ctrl Pts',(39.0491105869675,4.63145905356436,-59.8881929790463));
#36315=CARTESIAN_POINT('Ctrl Pts',(39.0520556446838,4.65242359175444,-60.1874268764735));
#36316=CARTESIAN_POINT('Ctrl Pts',(39.0568083712244,4.70044200077084,-60.701577007053));
#36317=CARTESIAN_POINT('Ctrl Pts',(39.0647851026013,4.83986722574065,-61.7205682736498));
#36318=CARTESIAN_POINT('Ctrl Pts',(39.0709887180427,5.08325331232971,-62.8490477340757));
#36319=CARTESIAN_POINT('Ctrl Pts',(39.0752427482449,5.38432421645409,-63.9439111987074));
#36320=CARTESIAN_POINT('Ctrl Pts',(39.077120582972,5.57085697178719,-64.5463222893431));
#36321=CARTESIAN_POINT('Ctrl Pts',(39.0782501814497,5.70052797189769,-64.9424009107793));
#36322=CARTESIAN_POINT('Ctrl Pts',(39.0789768145255,5.78828008713039,-65.2049220123974));
#36323=CARTESIAN_POINT('Ctrl Pts',(39.0796760255791,5.87783519500164,-65.465282468161));
#36324=CARTESIAN_POINT('Ctrl Pts',(39.0802782205174,5.95744149860314,-65.6910332366747));
#36325=CARTESIAN_POINT('Ctrl Pts',(39.0806225187686,6.00324452874798,-65.8194497916867));
#36326=CARTESIAN_POINT('Ctrl Pts',(39.0811395675323,6.0722540117692,-66.0115179492368));
#36327=CARTESIAN_POINT('Ctrl Pts',(39.0815785188012,6.13030929947426,-66.1703178692351));
#36328=CARTESIAN_POINT('Ctrl Pts',(39.0823113015601,6.22722406914699,-66.4323128067553));
#36329=CARTESIAN_POINT('Ctrl Pts',(39.0823264257121,6.34542292308159,-66.7374653354443));
#36330=CARTESIAN_POINT('Ctrl Pts',(39.0823439741756,6.58825383385029,-67.3138435469778));
#36331=CARTESIAN_POINT('Ctrl Pts',(39.0814243175378,7.04892946372,-68.3023886475656));
#36332=CARTESIAN_POINT('Ctrl Pts',(39.0780104825526,8.05142233211918,-70.1599124261361));
#36333=CARTESIAN_POINT('Ctrl Pts',(39.0759796367523,8.92684404100238,-71.620429840862));
#36334=CARTESIAN_POINT('Ctrl Pts',(39.0778501765501,9.48039133128234,-72.6727733170531));
#36335=CARTESIAN_POINT('Ctrl Pts',(39.0777036163807,9.61612898152865,-72.930414174574));
#36336=CARTESIAN_POINT('Ctrl Pts',(39.0777332821649,9.88098261723943,-73.4319298126859));
#36337=CARTESIAN_POINT('Ctrl Pts',(39.0776408633731,10.2155893430233,-74.0636143082731));
#36338=CARTESIAN_POINT('Ctrl Pts',(39.0776063699703,10.6162577801302,-74.8174541772381));
#36339=CARTESIAN_POINT('Ctrl Pts',(39.0775123909014,11.4193164891573,-76.3249523442607));
#36340=CARTESIAN_POINT('Ctrl Pts',(39.0775007402611,12.088608941729,-77.5775747026988));
#36341=CARTESIAN_POINT('Ctrl Pts',(39.0775902789745,13.0565767107738,-79.3982809975936));
#36342=CARTESIAN_POINT('Ctrl Pts',(39.077555137614,13.4939144140808,-80.220915032169));
#36343=CARTESIAN_POINT('Ctrl Pts',(39.077555137614,13.9304360014702,-81.0418927342675));
#36344=CARTESIAN_POINT('Ctrl Pts',(40.9894004876467,0.280289965204604,24.8306664866128));
#36345=CARTESIAN_POINT('Ctrl Pts',(40.9895240781924,0.280296218581876,24.781788183931));
#36346=CARTESIAN_POINT('Ctrl Pts',(40.9896536969077,0.280302775699746,24.7329109288453));
#36347=CARTESIAN_POINT('Ctrl Pts',(40.9911843863448,0.280380328702297,24.1823154886843));
#36348=CARTESIAN_POINT('Ctrl Pts',(40.9923576072282,0.28042149746924,23.1782063197446));
#36349=CARTESIAN_POINT('Ctrl Pts',(40.9950876108615,0.280503393819463,21.1696270948689));
#36350=CARTESIAN_POINT('Ctrl Pts',(41.0052748446288,0.281021429451735,19.6654825420095));
#36351=CARTESIAN_POINT('Ctrl Pts',(41.0268800436286,0.282211470259995,18.4144326432552));
#36352=CARTESIAN_POINT('Ctrl Pts',(41.0372448640096,0.282775963518614,17.9116781675146));
#36353=CARTESIAN_POINT('Ctrl Pts',(41.0632779338851,0.284183692506976,16.907738953426));
#36354=CARTESIAN_POINT('Ctrl Pts',(41.1191186246586,0.287208855599439,15.1539438974559));
#36355=CARTESIAN_POINT('Ctrl Pts',(41.1721339589163,0.290184770111345,13.6520495013715));
#36356=CARTESIAN_POINT('Ctrl Pts',(41.2053038114973,0.292227955892151,12.3973231743278));
#36357=CARTESIAN_POINT('Ctrl Pts',(41.2188587008223,0.293083716779208,11.8962631232141));
#36358=CARTESIAN_POINT('Ctrl Pts',(41.2464748712986,0.294894702945755,10.8942726028637));
#36359=CARTESIAN_POINT('Ctrl Pts',(41.2942318035546,0.298165354622819,9.14059418922836));
#36360=CARTESIAN_POINT('Ctrl Pts',(41.3276780750111,0.300596870688662,7.6355550985603));
#36361=CARTESIAN_POINT('Ctrl Pts',(41.3424933819775,0.301687677932141,6.50481724059173));
#36362=CARTESIAN_POINT('Ctrl Pts',(41.3455455913616,0.301921698056121,6.25451349465145));
#36363=CARTESIAN_POINT('Ctrl Pts',(41.3508035537116,0.302358173568668,5.75333848629102));
#36364=CARTESIAN_POINT('Ctrl Pts',(41.3579025293381,0.303033911829633,4.87488551207728));
#36365=CARTESIAN_POINT('Ctrl Pts',(41.3646402494083,0.303988962607526,3.11477685097418));
#36366=CARTESIAN_POINT('Ctrl Pts',(41.3608998764056,0.303976963099249,1.60893402861812));
#36367=CARTESIAN_POINT('Ctrl Pts',(41.3568438589094,0.303443240710702,0.550188033900891));
#36368=CARTESIAN_POINT('Ctrl Pts',(41.3563108048481,0.303372710104812,0.424096199846747));
#36369=CARTESIAN_POINT('Ctrl Pts',(41.3550557054703,0.303205889073847,0.172103952862311));
#36370=CARTESIAN_POINT('Ctrl Pts',(41.3523853952267,0.30284952374001,-0.268403745043762));
#36371=CARTESIAN_POINT('Ctrl Pts',(41.3473498002463,0.302175450216627,-0.896402017998833));
#36372=CARTESIAN_POINT('Ctrl Pts',(41.3397676155733,0.301166611708825,-1.64861694312906));
#36373=CARTESIAN_POINT('Ctrl Pts',(41.32817131415,0.299636955694652,-2.65004641299644));
#36374=CARTESIAN_POINT('Ctrl Pts',(41.3119240978266,0.297526861549583,-3.90045072486229));
#36375=CARTESIAN_POINT('Ctrl Pts',(41.2993231966601,0.295985803859787,-4.90158298379786));
#36376=CARTESIAN_POINT('Ctrl Pts',(41.2922670659562,0.295180386852342,-5.52813800082197));
#36377=CARTESIAN_POINT('Ctrl Pts',(41.2888008321068,0.294128291656232,-5.76976692890284));
#36378=CARTESIAN_POINT('Ctrl Pts',(41.279775715755,0.289610906860302,-6.26180359560708));
#36379=CARTESIAN_POINT('Ctrl Pts',(41.2597292666415,0.276788673760391,-7.12814793049486));
#36380=CARTESIAN_POINT('Ctrl Pts',(41.2260339563164,0.252707693024928,-8.38969666255411));
#36381=CARTESIAN_POINT('Ctrl Pts',(41.2044754185102,0.243431514589407,-9.67758594137821));
#36382=CARTESIAN_POINT('Ctrl Pts',(41.2056667875271,0.257236423541392,-10.5928325387983));
#36383=CARTESIAN_POINT('Ctrl Pts',(41.2124055691996,0.272908132480897,-11.1192902137075));
#36384=CARTESIAN_POINT('Ctrl Pts',(41.2180245806747,0.283699034777166,-11.3838816397246));
#36385=CARTESIAN_POINT('Ctrl Pts',(41.2231896003388,0.293053885000704,-11.5830954853462));
#36386=CARTESIAN_POINT('Ctrl Pts',(41.2270321549076,0.298372571821632,-11.7004341390505));
#36387=CARTESIAN_POINT('Ctrl Pts',(41.2359213994023,0.308805474889505,-11.946101479798));
#36388=CARTESIAN_POINT('Ctrl Pts',(41.2545818424021,0.325521986599661,-12.3752423953399));
#36389=CARTESIAN_POINT('Ctrl Pts',(41.3164031698591,0.366888900265877,-13.503692810886));
#36390=CARTESIAN_POINT('Ctrl Pts',(41.4164791591404,0.432260449691268,-14.8218440732556));
#36391=CARTESIAN_POINT('Ctrl Pts',(41.5126853503333,0.611890804668134,-16.2117251793627));
#36392=CARTESIAN_POINT('Ctrl Pts',(41.5560798164476,0.739109737741911,-16.9227612255263));
#36393=CARTESIAN_POINT('Ctrl Pts',(41.5858226355929,0.867870462690142,-17.5004550174555));
#36394=CARTESIAN_POINT('Ctrl Pts',(41.5986631614551,0.941986198987689,-17.791774374434));
#36395=CARTESIAN_POINT('Ctrl Pts',(41.6073391088081,1.00132103356657,-18.01063350892));
#36396=CARTESIAN_POINT('Ctrl Pts',(41.612336789908,1.04566843983575,-18.168467840582));
#36397=CARTESIAN_POINT('Ctrl Pts',(41.6233445207234,1.13909153802182,-18.4708337039972));
#36398=CARTESIAN_POINT('Ctrl Pts',(41.6347930089352,1.24221991447412,-18.7692102602174));
#36399=CARTESIAN_POINT('Ctrl Pts',(41.6467691662253,1.35210739165747,-19.0592219699898));
#36400=CARTESIAN_POINT('Ctrl Pts',(41.6543765632466,1.42350899292141,-19.2381761479961));
#36401=CARTESIAN_POINT('Ctrl Pts',(41.6605374423642,1.48197440697328,-19.3796471871768));
#36402=CARTESIAN_POINT('Ctrl Pts',(41.6667347584479,1.54130043502988,-19.5201450978797));
#36403=CARTESIAN_POINT('Ctrl Pts',(41.683917789257,1.70774630290237,-19.9024388048089));
#36404=CARTESIAN_POINT('Ctrl Pts',(41.7125416786971,1.99501903901531,-20.5067211987056));
#36405=CARTESIAN_POINT('Ctrl Pts',(41.7625655220588,2.5198132595399,-21.5289948136643));
#36406=CARTESIAN_POINT('Ctrl Pts',(41.8200577472395,3.15307170736816,-22.7212180677817));
#36407=CARTESIAN_POINT('Ctrl Pts',(41.8488304236762,3.53774225526409,-23.5902816645653));
#36408=CARTESIAN_POINT('Ctrl Pts',(41.8532019455559,3.70939876819118,-24.1019133916231));
#36409=CARTESIAN_POINT('Ctrl Pts',(41.847559820479,3.78269989350591,-24.3424841016166));
#36410=CARTESIAN_POINT('Ctrl Pts',(41.8332034174373,3.91366476460714,-24.8058945510647));
#36411=CARTESIAN_POINT('Ctrl Pts',(41.7916431387842,4.11813149520393,-25.6354534315072));
#36412=CARTESIAN_POINT('Ctrl Pts',(41.6981196178867,4.34114005251492,-26.831589099475));
#36413=CARTESIAN_POINT('Ctrl Pts',(41.5529595890076,4.53989978629295,-28.2865892807906));
#36414=CARTESIAN_POINT('Ctrl Pts',(41.4586652482338,4.65218169883083,-29.2630855169144));
#36415=CARTESIAN_POINT('Ctrl Pts',(41.415417858304,4.71536033758119,-29.813734772255));
#36416=CARTESIAN_POINT('Ctrl Pts',(41.4062626735763,4.72786753785767,-29.928444759334));
#36417=CARTESIAN_POINT('Ctrl Pts',(41.3873736554326,4.75186071062575,-30.1629289810428));
#36418=CARTESIAN_POINT('Ctrl Pts',(41.3537867479734,4.78945139312945,-30.5728749307636));
#36419=CARTESIAN_POINT('Ctrl Pts',(41.2843093467636,4.85022130294728,-31.401795513503));
#36420=CARTESIAN_POINT('Ctrl Pts',(41.2025017262904,4.89369214843913,-32.3654256174241));
#36421=CARTESIAN_POINT('Ctrl Pts',(41.1231231912229,4.92654223259855,-33.3475404655346));
#36422=CARTESIAN_POINT('Ctrl Pts',(41.0660176057825,4.94955818888471,-34.0930821250591));
#36423=CARTESIAN_POINT('Ctrl Pts',(41.0124746989083,4.97473940354442,-34.8476683038026));
#36424=CARTESIAN_POINT('Ctrl Pts',(40.9798803467751,4.99552224079456,-35.3568512303255));
#36425=CARTESIAN_POINT('Ctrl Pts',(40.9567923276298,5.01363279690724,-35.7416656893073));
#36426=CARTESIAN_POINT('Ctrl Pts',(40.9418575375759,5.02486297072264,-35.9871898225954));
#36427=CARTESIAN_POINT('Ctrl Pts',(40.9134419266958,5.04715573300395,-36.4848538030037));
#36428=CARTESIAN_POINT('Ctrl Pts',(40.8675702390212,5.08425686877861,-37.3516034800416));
#36429=CARTESIAN_POINT('Ctrl Pts',(40.7892286304169,5.15295731690531,-39.0869665669963));
#36430=CARTESIAN_POINT('Ctrl Pts',(40.7388485386345,5.20226763694573,-40.5777014848992));
#36431=CARTESIAN_POINT('Ctrl Pts',(40.7030370031305,5.23646785505578,-41.7033865298728));
#36432=CARTESIAN_POINT('Ctrl Pts',(40.6951763053688,5.24370191326017,-41.9494781443332));
#36433=CARTESIAN_POINT('Ctrl Pts',(40.6835691587561,5.25381676112557,-42.3207839283218));
#36434=CARTESIAN_POINT('Ctrl Pts',(40.6722320093476,5.2632399079877,-42.6924276736823));
#36435=CARTESIAN_POINT('Ctrl Pts',(40.6575726542033,5.27498381439645,-43.1892030370711));
#36436=CARTESIAN_POINT('Ctrl Pts',(40.6403107816893,5.28830990789018,-43.8117997930508));
#36437=CARTESIAN_POINT('Ctrl Pts',(40.6219085941156,5.3027190798521,-44.561273695052));
#36438=CARTESIAN_POINT('Ctrl Pts',(40.6090109207754,5.31389855681178,-45.1873168583986));
#36439=CARTESIAN_POINT('Ctrl Pts',(40.6005058493631,5.32270348051234,-45.6888589250754));
#36440=CARTESIAN_POINT('Ctrl Pts',(40.5950885572115,5.32928921826061,-46.0652901742846));
#36441=CARTESIAN_POINT('Ctrl Pts',(40.5907117320026,5.33593953036712,-46.441917636326));
#36442=CARTESIAN_POINT('Ctrl Pts',(40.5863809911267,5.34499956462259,-46.9443480187945));
#36443=CARTESIAN_POINT('Ctrl Pts',(40.5848842655861,5.35211785123058,-47.3211462433141));
#36444=CARTESIAN_POINT('Ctrl Pts',(40.5847633692936,5.35964313775713,-47.6992573476703));
#36445=CARTESIAN_POINT('Ctrl Pts',(40.5851228662576,5.36600919820418,-47.9640771570023));
#36446=CARTESIAN_POINT('Ctrl Pts',(40.5875219759791,5.38199478861863,-48.4820864135602));
#36447=CARTESIAN_POINT('Ctrl Pts',(40.5958135821412,5.41659412432496,-49.3803699663312));
#36448=CARTESIAN_POINT('Ctrl Pts',(40.6177810554637,5.47173761809535,-50.6267686734295));
#36449=CARTESIAN_POINT('Ctrl Pts',(40.6554784269053,5.50882248832631,-52.0671302450754));
#36450=CARTESIAN_POINT('Ctrl Pts',(40.6851890519631,5.49197283852475,-52.9879476265502));
#36451=CARTESIAN_POINT('Ctrl Pts',(40.7043047716274,5.4623346564178,-53.5512015026042));
#36452=CARTESIAN_POINT('Ctrl Pts',(40.7126861506626,5.44807663353492,-53.7455801974626));
#36453=CARTESIAN_POINT('Ctrl Pts',(40.7316675370788,5.40330909356921,-54.1715151734727));
#36454=CARTESIAN_POINT('Ctrl Pts',(40.7700244549047,5.28798694743009,-54.9488391356619));
#36455=CARTESIAN_POINT('Ctrl Pts',(40.8592954416422,4.95345830992145,-56.6665193418863));
#36456=CARTESIAN_POINT('Ctrl Pts',(40.9364237216775,4.65839267261391,-58.3911774895459));
#36457=CARTESIAN_POINT('Ctrl Pts',(40.9617107797564,4.72643201987558,-59.7487986227702));
#36458=CARTESIAN_POINT('Ctrl Pts',(40.9646667376791,4.73489817031782,-59.8925588835541));
#36459=CARTESIAN_POINT('Ctrl Pts',(40.9699463811896,4.75676105502465,-60.1906378709165));
#36460=CARTESIAN_POINT('Ctrl Pts',(40.9776820611458,4.80591692343881,-60.7031777052071));
#36461=CARTESIAN_POINT('Ctrl Pts',(40.9876798094656,4.94608479796233,-61.719426669608));
#36462=CARTESIAN_POINT('Ctrl Pts',(40.9894597138152,5.18797722463457,-62.8463779555874));
#36463=CARTESIAN_POINT('Ctrl Pts',(40.9871287060037,5.4870542555106,-63.9408714139306));
#36464=CARTESIAN_POINT('Ctrl Pts',(40.9852447349333,5.67254707948159,-64.5434760398196));
#36465=CARTESIAN_POINT('Ctrl Pts',(40.9841506366498,5.80167198872239,-64.939834443487));
#36466=CARTESIAN_POINT('Ctrl Pts',(40.9834901228094,5.88909927246302,-65.2025816691557));
#36467=CARTESIAN_POINT('Ctrl Pts',(40.9829679493291,5.97841710390143,-65.4632274230487));
#36468=CARTESIAN_POINT('Ctrl Pts',(40.9827042111471,6.05788935343768,-65.6892791115769));
#36469=CARTESIAN_POINT('Ctrl Pts',(40.9826178379952,6.10364136767694,-65.8178824506503));
#36470=CARTESIAN_POINT('Ctrl Pts',(40.9825568597767,6.17259966365106,-66.0102450339768));
#36471=CARTESIAN_POINT('Ctrl Pts',(40.9826595793067,6.23067616599025,-66.1693213756176));
#36472=CARTESIAN_POINT('Ctrl Pts',(40.9830722826943,6.32770140186445,-66.4318038468455));
#36473=CARTESIAN_POINT('Ctrl Pts',(40.9826301895095,6.4457659668906,-66.7368360495315));
#36474=CARTESIAN_POINT('Ctrl Pts',(40.9819298733969,6.68848664498193,-67.3133239784796));
#36475=CARTESIAN_POINT('Ctrl Pts',(40.9799735479708,7.14895751891722,-68.3018674424394));
#36476=CARTESIAN_POINT('Ctrl Pts',(40.9755106159698,8.15122815727162,-70.1595000872727));
#36477=CARTESIAN_POINT('Ctrl Pts',(40.9737637925337,9.02664471902918,-71.6199599132457));
#36478=CARTESIAN_POINT('Ctrl Pts',(40.9759071636186,9.58020392439139,-72.6723061261848));
#36479=CARTESIAN_POINT('Ctrl Pts',(40.9756944292259,9.715932120259,-72.9299622522639));
#36480=CARTESIAN_POINT('Ctrl Pts',(40.9756840265696,9.9807790550013,-73.431497908536));
#36481=CARTESIAN_POINT('Ctrl Pts',(40.975534467898,10.3153885484625,-74.0632025611493));
#36482=CARTESIAN_POINT('Ctrl Pts',(40.9754859360213,10.7160678877822,-74.8170603952781));
#36483=CARTESIAN_POINT('Ctrl Pts',(40.9754043570265,11.519160529892,-76.3245809572268));
#36484=CARTESIAN_POINT('Ctrl Pts',(40.9754628439931,12.1885065742482,-77.577179230038));
#36485=CARTESIAN_POINT('Ctrl Pts',(40.9755662823054,13.1564677204213,-79.3978374532215));
#36486=CARTESIAN_POINT('Ctrl Pts',(40.9755178661405,13.5938174653931,-80.2204797593586));
#36487=CARTESIAN_POINT('Ctrl Pts',(40.9755178661405,14.0303390527825,-81.041457461457));
#36488=CARTESIAN_POINT('Ctrl Pts',(42.8889150787531,0.396068481711534,24.8306496888204));
#36489=CARTESIAN_POINT('Ctrl Pts',(42.8890452628421,0.396076880893202,24.7817708717695));
#36490=CARTESIAN_POINT('Ctrl Pts',(42.8891817953486,0.396085686243203,24.7328930807602));
#36491=CARTESIAN_POINT('Ctrl Pts',(42.890794111377,0.396189858653643,24.1822919985291));
#36492=CARTESIAN_POINT('Ctrl Pts',(42.8920520234772,0.396260174705627,23.1781818084037));
#36493=CARTESIAN_POINT('Ctrl Pts',(42.8949939595196,0.396414545731705,21.1695904333064));
#36494=CARTESIAN_POINT('Ctrl Pts',(42.9057228555591,0.397109674005268,19.6654453673117));
#36495=CARTESIAN_POINT('Ctrl Pts',(42.9283668323194,0.3986324421576,18.4143920639703));
#36496=CARTESIAN_POINT('Ctrl Pts',(42.9392378465306,0.399361893759621,17.9115963066885));
#36497=CARTESIAN_POINT('Ctrl Pts',(42.966554492716,0.401193810292415,16.9076316288254));
#36498=CARTESIAN_POINT('Ctrl Pts',(43.0251424311424,0.405129815060431,15.1538532275295));
#36499=CARTESIAN_POINT('Ctrl Pts',(43.0806374138684,0.408896580224321,13.6521151629944));
#36500=CARTESIAN_POINT('Ctrl Pts',(43.1151397951303,0.411298181410661,12.3975676992226));
#36501=CARTESIAN_POINT('Ctrl Pts',(43.1292134522289,0.412285537605512,11.8965778965405));
#36502=CARTESIAN_POINT('Ctrl Pts',(43.1578019090676,0.414315817551931,10.8946903077876));
#36503=CARTESIAN_POINT('Ctrl Pts',(43.2070698183594,0.417865337697373,9.14110268879431));
#36504=CARTESIAN_POINT('Ctrl Pts',(43.2413981262261,0.420381972370076,7.63604493878829));
#36505=CARTESIAN_POINT('Ctrl Pts',(43.2566055344275,0.421494236844582,6.5052257455832));
#36506=CARTESIAN_POINT('Ctrl Pts',(43.2597261675554,0.421724236178688,6.25499255122132));
#36507=CARTESIAN_POINT('Ctrl Pts',(43.265054561117,0.422124291502451,5.75388353416307));
#36508=CARTESIAN_POINT('Ctrl Pts',(43.2721266717543,0.422675761799587,4.87553172663561));
#36509=CARTESIAN_POINT('Ctrl Pts',(43.2784257741905,0.423242384308679,3.1153638161988));
#36510=CARTESIAN_POINT('Ctrl Pts',(43.2743206313889,0.423040356686762,1.60922688217153));
#36511=CARTESIAN_POINT('Ctrl Pts',(43.270646295444,0.422730846980912,0.550031961270142));
#36512=CARTESIAN_POINT('Ctrl Pts',(43.2701630446794,0.422689748586847,0.42386146716886));
#36513=CARTESIAN_POINT('Ctrl Pts',(43.2690200093843,0.422593013249137,0.171737673254688));
#36514=CARTESIAN_POINT('Ctrl Pts',(43.2665787031098,0.422386510342781,-0.26898297337776));
#36515=CARTESIAN_POINT('Ctrl Pts',(43.2619499985229,0.421999139749318,-0.897171771739731));
#36516=CARTESIAN_POINT('Ctrl Pts',(43.2549683112281,0.421409828411748,-1.64956913593561));
#36517=CARTESIAN_POINT('Ctrl Pts',(43.2442689204981,0.420519244475927,-2.65104599767104));
#36518=CARTESIAN_POINT('Ctrl Pts',(43.2292768897199,0.419285597860539,-3.90125975062038));
#36519=CARTESIAN_POINT('Ctrl Pts',(43.2175584682409,0.418332876173394,-4.90192971557075));
#36520=CARTESIAN_POINT('Ctrl Pts',(43.2109670967596,0.417750167584731,-5.52777393061073));
#36521=CARTESIAN_POINT('Ctrl Pts',(43.2075257487689,0.416170506748705,-5.76115476093335));
#36522=CARTESIAN_POINT('Ctrl Pts',(43.1980260184467,0.408531449786692,-6.24416404317574));
#36523=CARTESIAN_POINT('Ctrl Pts',(43.1761122863911,0.38592218775056,-7.09904072274838));
#36524=CARTESIAN_POINT('Ctrl Pts',(43.1386060796012,0.342232708468757,-8.36514300158209));
#36525=CARTESIAN_POINT('Ctrl Pts',(43.1163909787538,0.325771628148733,-9.68282259533749));
#36526=CARTESIAN_POINT('Ctrl Pts',(43.1211014388009,0.353483267386871,-10.6331225806478));
#36527=CARTESIAN_POINT('Ctrl Pts',(43.1312843977344,0.384576771432351,-11.1834256559264));
#36528=CARTESIAN_POINT('Ctrl Pts',(43.1391397568144,0.405937922333632,-11.4612218857337));
#36529=CARTESIAN_POINT('Ctrl Pts',(43.146200478672,0.424447290733482,-11.6708379761057));
#36530=CARTESIAN_POINT('Ctrl Pts',(43.1516607467815,0.435567740941252,-11.7951244626329));
#36531=CARTESIAN_POINT('Ctrl Pts',(43.1648288797801,0.459308919272857,-12.0539241755026));
#36532=CARTESIAN_POINT('Ctrl Pts',(43.1935227276973,0.502779393692827,-12.5042829261807));
#36533=CARTESIAN_POINT('Ctrl Pts',(43.2918119782271,0.629153848729037,-13.677793750993));
#36534=CARTESIAN_POINT('Ctrl Pts',(43.4467454125466,0.841220065238567,-15.019462467646));
#36535=CARTESIAN_POINT('Ctrl Pts',(43.5583435321655,1.17535730430707,-16.3968673604407));
#36536=CARTESIAN_POINT('Ctrl Pts',(43.5968235463072,1.37363963190595,-17.0927392942544));
#36537=CARTESIAN_POINT('Ctrl Pts',(43.6139629424047,1.55240211508456,-17.6539070332424));
#36538=CARTESIAN_POINT('Ctrl Pts',(43.6175553061863,1.64850035004579,-17.9356752158864));
#36539=CARTESIAN_POINT('Ctrl Pts',(43.6181384922512,1.72310238210498,-18.1473365030579));
#36540=CARTESIAN_POINT('Ctrl Pts',(43.6154303426995,1.7814430065369,-18.3099346755337));
#36541=CARTESIAN_POINT('Ctrl Pts',(43.6102846417711,1.90052004612951,-18.6147396344814));
#36542=CARTESIAN_POINT('Ctrl Pts',(43.602870007724,2.02979070845934,-18.9160782312125));
#36543=CARTESIAN_POINT('Ctrl Pts',(43.5946110817454,2.16471521744707,-19.2068265076608));
#36544=CARTESIAN_POINT('Ctrl Pts',(43.5889845057232,2.25153983815122,-19.3861334620883));
#36545=CARTESIAN_POINT('Ctrl Pts',(43.5843255425046,2.32208625553214,-19.5276182811613));
#36546=CARTESIAN_POINT('Ctrl Pts',(43.5795540667035,2.39335083839521,-19.6680602821549));
#36547=CARTESIAN_POINT('Ctrl Pts',(43.5660313407155,2.59193642338233,-20.0497805933487));
#36548=CARTESIAN_POINT('Ctrl Pts',(43.5425809194297,2.92788658122492,-20.65185956446));
#36549=CARTESIAN_POINT('Ctrl Pts',(43.502823575907,3.52399087311658,-21.6676436722937));
#36550=CARTESIAN_POINT('Ctrl Pts',(43.4667434267997,4.21004027159046,-22.8464385926046));
#36551=CARTESIAN_POINT('Ctrl Pts',(43.4612201547408,4.57433453371028,-23.6690393021299));
#36552=CARTESIAN_POINT('Ctrl Pts',(43.4555230860129,4.71666048256263,-24.1239260645268));
#36553=CARTESIAN_POINT('Ctrl Pts',(43.4463563974337,4.77865788443132,-24.3434559879189));
#36554=CARTESIAN_POINT('Ctrl Pts',(43.4252682870347,4.88049123337781,-24.7666198887204));
#36555=CARTESIAN_POINT('Ctrl Pts',(43.3726379146404,5.02212856520801,-25.533140126944));
#36556=CARTESIAN_POINT('Ctrl Pts',(43.2648052510907,5.13260362804228,-26.6650982276858));
#36557=CARTESIAN_POINT('Ctrl Pts',(43.1114452747013,5.19718538092319,-28.101595939478));
#36558=CARTESIAN_POINT('Ctrl Pts',(43.0185651733528,5.23924054246157,-29.1106253705117));
#36559=CARTESIAN_POINT('Ctrl Pts',(42.975411723984,5.27407710578951,-29.6911791890907));
#36560=CARTESIAN_POINT('Ctrl Pts',(42.9662152538132,5.27991788449142,-29.8027208427268));
#36561=CARTESIAN_POINT('Ctrl Pts',(42.9477927089147,5.29101628404784,-30.0366498359351));
#36562=CARTESIAN_POINT('Ctrl Pts',(42.91614290608,5.30639565662637,-30.443409397974));
#36563=CARTESIAN_POINT('Ctrl Pts',(42.8549443949215,5.3243938549592,-31.27046673341));
#36564=CARTESIAN_POINT('Ctrl Pts',(42.7909610327225,5.32097155220782,-32.2357129529905));
#36565=CARTESIAN_POINT('Ctrl Pts',(42.7334821383245,5.30738667036426,-33.2239095611256));
#36566=CARTESIAN_POINT('Ctrl Pts',(42.6935684398686,5.29586561496228,-33.9755125717022));
#36567=CARTESIAN_POINT('Ctrl Pts',(42.6568047178287,5.28701745361284,-34.7375684502777));
#36568=CARTESIAN_POINT('Ctrl Pts',(42.6342992001023,5.28573624978323,-35.2525662574588));
#36569=CARTESIAN_POINT('Ctrl Pts',(42.6180899591343,5.28762621774343,-35.6420378218769));
#36570=CARTESIAN_POINT('Ctrl Pts',(42.6076098316725,5.28875574807696,-35.8892618882715));
#36571=CARTESIAN_POINT('Ctrl Pts',(42.5880999328398,5.29084322749353,-36.3910947456908));
#36572=CARTESIAN_POINT('Ctrl Pts',(42.5575445668297,5.29403896822109,-37.2645761631907));
#36573=CARTESIAN_POINT('Ctrl Pts',(42.508580153775,5.29886526853191,-39.0133351135283));
#36574=CARTESIAN_POINT('Ctrl Pts',(42.4806557469868,5.30255980347641,-40.5146273530696));
#36575=CARTESIAN_POINT('Ctrl Pts',(42.4598279127556,5.3071617097167,-41.6480996481441));
#36576=CARTESIAN_POINT('Ctrl Pts',(42.4551630127186,5.30797458086478,-41.8956086156392));
#36577=CARTESIAN_POINT('Ctrl Pts',(42.4481045054802,5.3088012311728,-42.2692958029665));
#36578=CARTESIAN_POINT('Ctrl Pts',(42.4410806477194,5.3093045717839,-42.6433529512525));
#36579=CARTESIAN_POINT('Ctrl Pts',(42.4319011994612,5.3096803572806,-43.1434933004772));
#36580=CARTESIAN_POINT('Ctrl Pts',(42.4210267262244,5.30981707015305,-43.7704913693995));
#36581=CARTESIAN_POINT('Ctrl Pts',(42.4097481310677,5.31019237418895,-44.5255742396024));
#36582=CARTESIAN_POINT('Ctrl Pts',(42.4024993086791,5.3113033018907,-45.1565472183013));
#36583=CARTESIAN_POINT('Ctrl Pts',(42.398397320432,5.31304412980648,-45.6621764086441));
#36584=CARTESIAN_POINT('Ctrl Pts',(42.3962707885433,5.31487412266376,-46.0417486495161));
#36585=CARTESIAN_POINT('Ctrl Pts',(42.3951961796171,5.31732308733461,-46.421590372106));
#36586=CARTESIAN_POINT('Ctrl Pts',(42.3953084294671,5.32155303507846,-46.9283993184451));
#36587=CARTESIAN_POINT('Ctrl Pts',(42.3972711090846,5.32593157343998,-47.3085963361452));
#36588=CARTESIAN_POINT('Ctrl Pts',(42.4007224973633,5.33136402272493,-47.6901959858782));
#36589=CARTESIAN_POINT('Ctrl Pts',(42.4035392670192,5.33661313230962,-47.9583036263036));
#36590=CARTESIAN_POINT('Ctrl Pts',(42.4110068955218,5.35158369677478,-48.4818228843904));
#36591=CARTESIAN_POINT('Ctrl Pts',(42.4285681184022,5.38732529484062,-49.3888607634442));
#36592=CARTESIAN_POINT('Ctrl Pts',(42.4645238996338,5.45068060622925,-50.6443525671912));
#36593=CARTESIAN_POINT('Ctrl Pts',(42.5191045186815,5.50423224997189,-52.090968173697));
#36594=CARTESIAN_POINT('Ctrl Pts',(42.5587493674228,5.49944433627563,-53.0127660531225));
#36595=CARTESIAN_POINT('Ctrl Pts',(42.5830810557466,5.47708645406835,-53.5757228925217));
#36596=CARTESIAN_POINT('Ctrl Pts',(42.5934813918469,5.46548208533803,-53.7741404072612));
#36597=CARTESIAN_POINT('Ctrl Pts',(42.6163375594127,5.42734228091482,-54.2046414224714));
#36598=CARTESIAN_POINT('Ctrl Pts',(42.6609056441398,5.32617334286943,-54.9886206253845));
#36599=CARTESIAN_POINT('Ctrl Pts',(42.7600999447217,5.02873100100508,-56.7100594745335));
#36600=CARTESIAN_POINT('Ctrl Pts',(42.8416784052924,4.77265331680418,-58.4251679895872));
#36601=CARTESIAN_POINT('Ctrl Pts',(42.8685582931606,4.85151949519224,-59.7649378323137));
#36602=CARTESIAN_POINT('Ctrl Pts',(42.8717147900666,4.86106114166371,-59.9071771526114));
#36603=CARTESIAN_POINT('Ctrl Pts',(42.8772755002816,4.88475916132963,-60.2020395748597));
#36604=CARTESIAN_POINT('Ctrl Pts',(42.8852597130217,4.93611278948848,-60.7095740147467));
#36605=CARTESIAN_POINT('Ctrl Pts',(42.8948598975998,5.07736527871554,-61.717531467479));
#36606=CARTESIAN_POINT('Ctrl Pts',(42.8947058818154,5.31520926574883,-62.8393075875396));
#36607=CARTESIAN_POINT('Ctrl Pts',(42.8899738228548,5.60917737087592,-63.9323206739159));
#36608=CARTESIAN_POINT('Ctrl Pts',(42.8867547638397,5.79206068141782,-64.5353857364383));
#36609=CARTESIAN_POINT('Ctrl Pts',(42.8848516505248,5.91982637407483,-64.9325557510509));
#36610=CARTESIAN_POINT('Ctrl Pts',(42.8836781105316,6.00646819476968,-65.1959777609207));
#36611=CARTESIAN_POINT('Ctrl Pts',(42.8826910715564,6.09519584324768,-65.4574935630298));
#36612=CARTESIAN_POINT('Ctrl Pts',(42.882073521951,6.17437856538853,-65.6844780375945));
#36613=CARTESIAN_POINT('Ctrl Pts',(42.8818020470254,6.22003480886732,-65.8136632008719));
#36614=CARTESIAN_POINT('Ctrl Pts',(42.8814811499691,6.28892209624111,-66.0069454600372));
#36615=CARTESIAN_POINT('Ctrl Pts',(42.8814074477665,6.34709559252622,-66.1668929685478));
#36616=CARTESIAN_POINT('Ctrl Pts',(42.8815860469944,6.44451339963721,-66.4309135780944));
#36617=CARTESIAN_POINT('Ctrl Pts',(42.8808197276845,6.56224929149011,-66.7356096804903));
#36618=CARTESIAN_POINT('Ctrl Pts',(42.879603870637,6.80478971247199,-67.3124902879198));
#36619=CARTESIAN_POINT('Ctrl Pts',(42.8769176292393,7.26483872667389,-68.3011132441212));
#36620=CARTESIAN_POINT('Ctrl Pts',(42.8717509539682,8.26681183148849,-70.1591713034738));
#36621=CARTESIAN_POINT('Ctrl Pts',(42.8704039331454,9.14211299084993,-71.6194799934297));
#36622=CARTESIAN_POINT('Ctrl Pts',(42.8729303366428,9.69553181558638,-72.6717208012155));
#36623=CARTESIAN_POINT('Ctrl Pts',(42.872671040637,9.83124888405079,-72.9294152719817));
#36624=CARTESIAN_POINT('Ctrl Pts',(42.8726498197238,10.0960764052722,-73.4309878818336));
#36625=CARTESIAN_POINT('Ctrl Pts',(42.8724667652836,10.4306786414141,-74.0627388472059));
#36626=CARTESIAN_POINT('Ctrl Pts',(42.8724079265588,10.8313728766808,-74.8166344421457));
#36627=CARTESIAN_POINT('Ctrl Pts',(42.8723174539684,11.6345214397113,-76.3242063248351));
#36628=CARTESIAN_POINT('Ctrl Pts',(42.8724082948828,12.3039114944934,-77.5767660843792));
#36629=CARTESIAN_POINT('Ctrl Pts',(42.8725371303758,13.2718187211776,-79.3973294406647));
#36630=CARTESIAN_POINT('Ctrl Pts',(42.8724803799683,13.7091749119834,-80.2199918930716));
#36631=CARTESIAN_POINT('Ctrl Pts',(42.8724803799683,14.1456964993729,-81.0409695951699));
#36632=CARTESIAN_POINT('Ctrl Pts',(45.2615410902239,0.56892790035043,24.8305651889563));
#36633=CARTESIAN_POINT('Ctrl Pts',(45.2616788469112,0.568940634819196,24.7816836995172));
#36634=CARTESIAN_POINT('Ctrl Pts',(45.2618233193469,0.568953982664532,24.7328031712021));
#36635=CARTESIAN_POINT('Ctrl Pts',(45.2635294287772,0.569111836537056,24.182171251646));
#36636=CARTESIAN_POINT('Ctrl Pts',(45.2648761502202,0.569267594765854,23.1780307587285));
#36637=CARTESIAN_POINT('Ctrl Pts',(45.2680349536899,0.569648776159213,21.1693813670506));
#36638=CARTESIAN_POINT('Ctrl Pts',(45.2793879851866,0.570699976742199,19.6652259238777));
#36639=CARTESIAN_POINT('Ctrl Pts',(45.3032710496568,0.572756846002772,18.4141660720332));
#36640=CARTESIAN_POINT('Ctrl Pts',(45.3147346667214,0.573760233722913,17.9112035852143));
#36641=CARTESIAN_POINT('Ctrl Pts',(45.3435348065703,0.576309580397626,16.9071247576477));
#36642=CARTESIAN_POINT('Ctrl Pts',(45.4052930371425,0.581772246147764,15.153373130955));
#36643=CARTESIAN_POINT('Ctrl Pts',(45.4637836385732,0.586721616865389,13.6522000105154));
#36644=CARTESIAN_POINT('Ctrl Pts',(45.5001423649963,0.589381953653535,12.3983644658879));
#36645=CARTESIAN_POINT('Ctrl Pts',(45.5149663851462,0.590419644498185,11.8976615784835));
#36646=CARTESIAN_POINT('Ctrl Pts',(45.5450643958688,0.592375084156006,10.8961995239767));
#36647=CARTESIAN_POINT('Ctrl Pts',(45.5969137919438,0.595425285874441,9.14302073301941));
#36648=CARTESIAN_POINT('Ctrl Pts',(45.6330865439585,0.597206501163487,7.63778973696807));
#36649=CARTESIAN_POINT('Ctrl Pts',(45.649195554732,0.597936850330345,6.50655828026605));
#36650=CARTESIAN_POINT('Ctrl Pts',(45.6525038017218,0.598065911712743,6.2565298469245));
#36651=CARTESIAN_POINT('Ctrl Pts',(45.6581651586369,0.598202757340735,5.75558965548895));
#36652=CARTESIAN_POINT('Ctrl Pts',(45.6657159692505,0.598166373938152,4.87748020571371));
#36653=CARTESIAN_POINT('Ctrl Pts',(45.6725898914032,0.597314518635698,3.11704906257916));
#36654=CARTESIAN_POINT('Ctrl Pts',(45.6685138556414,0.596363463605718,1.60983243588655));
#36655=CARTESIAN_POINT('Ctrl Pts',(45.6648670787423,0.596698777805479,0.549183894455631));
#36656=CARTESIAN_POINT('Ctrl Pts',(45.6643767377126,0.596741852454767,0.422844585317528));
#36657=CARTESIAN_POINT('Ctrl Pts',(45.6631854073049,0.596842810294774,0.170395884188534));
#36658=CARTESIAN_POINT('Ctrl Pts',(45.6605762007441,0.597055391369542,-0.270858389192889));
#36659=CARTESIAN_POINT('Ctrl Pts',(45.6555185595092,0.59745299864442,-0.899651604736923));
#36660=CARTESIAN_POINT('Ctrl Pts',(45.6478526863677,0.598043494116904,-1.65265951815702));
#36661=CARTESIAN_POINT('Ctrl Pts',(45.6362144182659,0.598938873236841,-2.6545822356401));
#36662=CARTESIAN_POINT('Ctrl Pts',(45.6203390738768,0.6001363991942,-3.90474838480635));
#36663=CARTESIAN_POINT('Ctrl Pts',(45.6091854285172,0.601113517590204,-4.90501214468221));
#36664=CARTESIAN_POINT('Ctrl Pts',(45.6036109599966,0.601735734372738,-5.52991954576289));
#36665=CARTESIAN_POINT('Ctrl Pts',(45.6006260701382,0.599705001594043,-5.74990053211739));
#36666=CARTESIAN_POINT('Ctrl Pts',(45.5922312328804,0.588079076490982,-6.21835663472809));
#36667=CARTESIAN_POINT('Ctrl Pts',(45.5727483109654,0.551780036098233,-7.05491709802254));
#36668=CARTESIAN_POINT('Ctrl Pts',(45.5400013997707,0.478460081274117,-8.32900326154292));
#36669=CARTESIAN_POINT('Ctrl Pts',(45.5231832958852,0.451664466589343,-9.69595582677582));
#36670=CARTESIAN_POINT('Ctrl Pts',(45.5312025389088,0.50586094227689,-10.7037582186805));
#36671=CARTESIAN_POINT('Ctrl Pts',(45.5428511712477,0.565867706345419,-11.2928440346444));
#36672=CARTESIAN_POINT('Ctrl Pts',(45.5512011633854,0.606996131319551,-11.5918108244126));
#36673=CARTESIAN_POINT('Ctrl Pts',(45.5584957597952,0.642668846885867,-11.818204255642));
#36674=CARTESIAN_POINT('Ctrl Pts',(45.5644217032906,0.665914835001241,-11.9616068001552));
#36675=CARTESIAN_POINT('Ctrl Pts',(45.5792940450002,0.717572370742471,-12.2518202910108));
#36676=CARTESIAN_POINT('Ctrl Pts',(45.6125620818531,0.818496227435111,-12.7533551123664));
#36677=CARTESIAN_POINT('Ctrl Pts',(45.7296217181159,1.13198913807883,-14.026065678441));
#36678=CARTESIAN_POINT('Ctrl Pts',(45.8978143670819,1.62983274007774,-15.3630201137124));
#36679=CARTESIAN_POINT('Ctrl Pts',(45.9897284041635,2.17415695503713,-16.6449752515272));
#36680=CARTESIAN_POINT('Ctrl Pts',(46.0127724924086,2.44677387787828,-17.2789861198244));
#36681=CARTESIAN_POINT('Ctrl Pts',(46.014009774241,2.65995813440371,-17.7842112606934));
#36682=CARTESIAN_POINT('Ctrl Pts',(46.0086679235749,2.76381305873585,-18.0365081413938));
#36683=CARTESIAN_POINT('Ctrl Pts',(46.0020636910816,2.8403821505569,-18.2259250589348));
#36684=CARTESIAN_POINT('Ctrl Pts',(45.9916808054812,2.90249286496111,-18.3814549615846));
#36685=CARTESIAN_POINT('Ctrl Pts',(45.9710975209746,3.02404152226732,-18.6701480431207));
#36686=CARTESIAN_POINT('Ctrl Pts',(45.9455719114267,3.15243902328813,-18.9599438001704));
#36687=CARTESIAN_POINT('Ctrl Pts',(45.9176508537205,3.28290315146194,-19.2408978583454));
#36688=CARTESIAN_POINT('Ctrl Pts',(45.8989712480038,3.36582133959271,-19.4152139613651));
#36689=CARTESIAN_POINT('Ctrl Pts',(45.8835049784142,3.43255754172811,-19.5531457520749));
#36690=CARTESIAN_POINT('Ctrl Pts',(45.8676702465408,3.49960402086995,-19.6903699423378));
#36691=CARTESIAN_POINT('Ctrl Pts',(45.8227735189325,3.68494200445599,-20.064432073456));
#36692=CARTESIAN_POINT('Ctrl Pts',(45.7430985862396,3.99096854553774,-20.6596128083382));
#36693=CARTESIAN_POINT('Ctrl Pts',(45.5942885703309,4.51601048935695,-21.6699979055485));
#36694=CARTESIAN_POINT('Ctrl Pts',(45.4103878731843,5.08412976379374,-22.8411424812185));
#36695=CARTESIAN_POINT('Ctrl Pts',(45.2950650565968,5.35245248641301,-23.6349743610973));
#36696=CARTESIAN_POINT('Ctrl Pts',(45.2467980468575,5.45398333321623,-24.067533279953));
#36697=CARTESIAN_POINT('Ctrl Pts',(45.2273091162407,5.4958660759811,-24.2646722831934));
#36698=CARTESIAN_POINT('Ctrl Pts',(45.1894254535133,5.56227267487467,-24.6530195142001));
#36699=CARTESIAN_POINT('Ctrl Pts',(45.1258434031292,5.64619968427566,-25.3631834960375));
#36700=CARTESIAN_POINT('Ctrl Pts',(45.0483411872772,5.68371483506249,-26.4538242396258));
#36701=CARTESIAN_POINT('Ctrl Pts',(44.982611553414,5.65173052539128,-27.9001654232592));
#36702=CARTESIAN_POINT('Ctrl Pts',(44.9520931849871,5.6297158664385,-28.9494453654781));
#36703=CARTESIAN_POINT('Ctrl Pts',(44.9367550156712,5.63646385005425,-29.5611765185561));
#36704=CARTESIAN_POINT('Ctrl Pts',(44.9335181167507,5.63743428480618,-29.6742737992605));
#36705=CARTESIAN_POINT('Ctrl Pts',(44.9278510404227,5.638342727517,-29.9142297946347));
#36706=CARTESIAN_POINT('Ctrl Pts',(44.9198833000213,5.63695948677616,-30.329708561198));
#36707=CARTESIAN_POINT('Ctrl Pts',(44.9110674004613,5.62363210600333,-31.1738918958072));
#36708=CARTESIAN_POINT('Ctrl Pts',(44.9137412486688,5.58921702124126,-32.1537082145959));
#36709=CARTESIAN_POINT('Ctrl Pts',(44.9223411691491,5.54719748444965,-33.1515379207248));
#36710=CARTESIAN_POINT('Ctrl Pts',(44.9300993735876,5.51501168648089,-33.9075980489476));
#36711=CARTESIAN_POINT('Ctrl Pts',(44.9374788571034,5.48537115623183,-34.6713843255509));
#36712=CARTESIAN_POINT('Ctrl Pts',(44.9410536800944,5.46948092009931,-35.1856280500676));
#36713=CARTESIAN_POINT('Ctrl Pts',(44.9428188911152,5.45985012926995,-35.5739257705073));
#36714=CARTESIAN_POINT('Ctrl Pts',(44.9441592845655,5.45370335423039,-35.8236345693171));
#36715=CARTESIAN_POINT('Ctrl Pts',(44.9474689312597,5.44146970474214,-36.3284493873013));
#36716=CARTESIAN_POINT('Ctrl Pts',(44.954638159495,5.42069090277913,-37.207808874577));
#36717=CARTESIAN_POINT('Ctrl Pts',(44.9728639366942,5.38219060707259,-38.9666289774347));
#36718=CARTESIAN_POINT('Ctrl Pts',(44.9889923982044,5.35602496485368,-40.475866881289));
#36719=CARTESIAN_POINT('Ctrl Pts',(44.9953942460701,5.34195475745522,-41.6149580555204));
#36720=CARTESIAN_POINT('Ctrl Pts',(44.9966432669531,5.33880182227349,-41.8633103712195));
#36721=CARTESIAN_POINT('Ctrl Pts',(44.9980723578167,5.33383563704676,-42.2386233094709));
#36722=CARTESIAN_POINT('Ctrl Pts',(44.9991320563092,5.32880239446087,-42.6143713442757));
#36723=CARTESIAN_POINT('Ctrl Pts',(45.0001409655838,5.32214823876549,-43.1169950546398));
#36724=CARTESIAN_POINT('Ctrl Pts',(45.0008272884051,5.31428038683488,-43.7474178397165));
#36725=CARTESIAN_POINT('Ctrl Pts',(45.0012877427439,5.30658866273375,-44.5071452285576));
#36726=CARTESIAN_POINT('Ctrl Pts',(45.0018337011019,5.30251079913816,-45.1424179587062));
#36727=CARTESIAN_POINT('Ctrl Pts',(45.0026765863635,5.30120986027071,-45.6517210663674));
#36728=CARTESIAN_POINT('Ctrl Pts',(45.0035676018574,5.30133307305741,-46.0341809638089));
#36729=CARTESIAN_POINT('Ctrl Pts',(45.004789315115,5.30269163793039,-46.4170408268167));
#36730=CARTESIAN_POINT('Ctrl Pts',(45.0069605613675,5.30633439736445,-46.9280475789432));
#36731=CARTESIAN_POINT('Ctrl Pts',(45.0092740957863,5.31131329393198,-47.3116113548291));
#36732=CARTESIAN_POINT('Ctrl Pts',(45.0122199512957,5.31809960954172,-47.6967565980147));
#36733=CARTESIAN_POINT('Ctrl Pts',(45.0142487771965,5.32470451541727,-47.9686651663915));
#36734=CARTESIAN_POINT('Ctrl Pts',(45.0186202635373,5.34374882326917,-48.4982678866572));
#36735=CARTESIAN_POINT('Ctrl Pts',(45.0270592218719,5.38976720160193,-49.4147628842762));
#36736=CARTESIAN_POINT('Ctrl Pts',(45.0415152459114,5.4742819482128,-50.6789358291947));
#36737=CARTESIAN_POINT('Ctrl Pts',(45.0627150222664,5.55587055132917,-52.1287938500016));
#36738=CARTESIAN_POINT('Ctrl Pts',(45.0793287693003,5.56822594841936,-53.047487561374));
#36739=CARTESIAN_POINT('Ctrl Pts',(45.0903572481794,5.55517123050684,-53.6069076033485));
#36740=CARTESIAN_POINT('Ctrl Pts',(45.095008174112,5.54684870326733,-53.8080284349928));
#36741=CARTESIAN_POINT('Ctrl Pts',(45.1052426506285,5.5163187230399,-54.2407753067327));
#36742=CARTESIAN_POINT('Ctrl Pts',(45.1254358798707,5.4302233943472,-55.0281454420526));
#36743=CARTESIAN_POINT('Ctrl Pts',(45.1724795764375,5.16831036533154,-56.7499014534075));
#36744=CARTESIAN_POINT('Ctrl Pts',(45.2150148067347,4.94543213105456,-58.4564161559867));
#36745=CARTESIAN_POINT('Ctrl Pts',(45.2290442284572,5.03430264673683,-59.7812190912645));
#36746=CARTESIAN_POINT('Ctrl Pts',(45.2307700751369,5.04477387261886,-59.9217891402866));
#36747=CARTESIAN_POINT('Ctrl Pts',(45.2338887977571,5.07006301467846,-60.2134201034817));
#36748=CARTESIAN_POINT('Ctrl Pts',(45.238675751841,5.12325407856103,-60.7157796244941));
#36749=CARTESIAN_POINT('Ctrl Pts',(45.2456923316338,5.2651167467366,-61.7152143196181));
#36750=CARTESIAN_POINT('Ctrl Pts',(45.2490891950485,5.49881026242882,-62.8315081546936));
#36751=CARTESIAN_POINT('Ctrl Pts',(45.2501264528762,5.78767847262183,-63.9229172106332));
#36752=CARTESIAN_POINT('Ctrl Pts',(45.2502297313784,5.9679585610093,-64.5264409767567));
#36753=CARTESIAN_POINT('Ctrl Pts',(45.2502672432246,6.09437230432477,-64.9244570077799));
#36754=CARTESIAN_POINT('Ctrl Pts',(45.2502950068668,6.18022801163112,-65.1885868554451));
#36755=CARTESIAN_POINT('Ctrl Pts',(45.2503397288732,6.26837601445132,-65.4510184228235));
#36756=CARTESIAN_POINT('Ctrl Pts',(45.2504264703855,6.34726911685607,-65.6789906388552));
#36757=CARTESIAN_POINT('Ctrl Pts',(45.2504933615793,6.39282929282686,-65.8087930688745));
#36758=CARTESIAN_POINT('Ctrl Pts',(45.2506122890501,6.46164378698788,-66.0030523889319));
#36759=CARTESIAN_POINT('Ctrl Pts',(45.25075612524,6.51991763400415,-66.1639269551648));
#36760=CARTESIAN_POINT('Ctrl Pts',(45.2510572428287,6.61772521636265,-66.42959067944));
#36761=CARTESIAN_POINT('Ctrl Pts',(45.250305373501,6.73510925409277,-66.7339934534138));
#36762=CARTESIAN_POINT('Ctrl Pts',(45.2491046658658,6.97745770150096,-67.3113721716749));
#36763=CARTESIAN_POINT('Ctrl Pts',(45.2462900770827,7.43712178562395,-68.3002013325194));
#36764=CARTESIAN_POINT('Ctrl Pts',(45.2406999811744,8.43899343028371,-70.1588236954198));
#36765=CARTESIAN_POINT('Ctrl Pts',(45.2394106211059,9.31441939926999,-71.6189314434897));
#36766=CARTESIAN_POINT('Ctrl Pts',(45.2425965754305,9.86769517696103,-72.6709296364789));
#36767=CARTESIAN_POINT('Ctrl Pts',(45.2423191993804,10.0034062223631,-72.9286676159832));
#36768=CARTESIAN_POINT('Ctrl Pts',(45.2423416503406,10.2682178791503,-73.4302683407546));
#36769=CARTESIAN_POINT('Ctrl Pts',(45.2421536257646,10.6028211926649,-74.0620633849328));
#36770=CARTESIAN_POINT('Ctrl Pts',(45.242085184474,11.0035312252382,-74.8159927127367));
#36771=CARTESIAN_POINT('Ctrl Pts',(45.2419319021468,11.806733918079,-76.3236140381719));
#36772=CARTESIAN_POINT('Ctrl Pts',(45.241945137619,12.4761804875285,-77.5761354704948));
#36773=CARTESIAN_POINT('Ctrl Pts',(45.242101587135,13.4440512328765,-79.3966068480627));
#36774=CARTESIAN_POINT('Ctrl Pts',(45.2420325945625,13.8814194541,-80.219286814076));
#36775=CARTESIAN_POINT('Ctrl Pts',(45.2420325945625,14.3179410414895,-81.0402645161742));
#36776=CARTESIAN_POINT('Ctrl Pts',(48.1081629096089,0.821649737971831,24.8305516722305));
#36777=CARTESIAN_POINT('Ctrl Pts',(48.1083051106799,0.821665512614002,24.7816697400132));
#36778=CARTESIAN_POINT('Ctrl Pts',(48.1084542508962,0.821682047191606,24.7327887495063));
#36779=CARTESIAN_POINT('Ctrl Pts',(48.1102154710524,0.821877593257419,24.1821520591425));
#36780=CARTESIAN_POINT('Ctrl Pts',(48.1115212775643,0.822067622638418,23.1779988161717));
#36781=CARTESIAN_POINT('Ctrl Pts',(48.1145315886128,0.82253067075772,21.1693455405452));
#36782=CARTESIAN_POINT('Ctrl Pts',(48.1262541377065,0.823833454224577,19.6652159354718));
#36783=CARTESIAN_POINT('Ctrl Pts',(48.1513361492619,0.826397238176174,18.4141809690976));
#36784=CARTESIAN_POINT('Ctrl Pts',(48.1633375349177,0.827634154049395,17.9112422895808));
#36785=CARTESIAN_POINT('Ctrl Pts',(48.1934232679837,0.830752491267504,16.9071764083677));
#36786=CARTESIAN_POINT('Ctrl Pts',(48.2579574400696,0.837426380535316,15.1533897846288));
#36787=CARTESIAN_POINT('Ctrl Pts',(48.3196288164366,0.843613101712407,13.6521589092755));
#36788=CARTESIAN_POINT('Ctrl Pts',(48.3589766451503,0.84720841794872,12.3982627094592));
#36789=CARTESIAN_POINT('Ctrl Pts',(48.3751362078385,0.848644122282542,11.8975361584115));
#36790=CARTESIAN_POINT('Ctrl Pts',(48.408316262668,0.85146656541503,10.8960642754308));
#36791=CARTESIAN_POINT('Ctrl Pts',(48.4662441063241,0.856136247284531,9.14292354130284));
#36792=CARTESIAN_POINT('Ctrl Pts',(48.5074331513585,0.859208707164653,7.63783993867673));
#36793=CARTESIAN_POINT('Ctrl Pts',(48.5258835278248,0.860559046852656,6.50665095597728));
#36794=CARTESIAN_POINT('Ctrl Pts',(48.5297150707781,0.860822033143301,6.25656648324836));
#36795=CARTESIAN_POINT('Ctrl Pts',(48.5364301565456,0.861228582180177,5.75556890302458));
#36796=CARTESIAN_POINT('Ctrl Pts',(48.5458033902991,0.861660579302824,4.87740144016084));
#36797=CARTESIAN_POINT('Ctrl Pts',(48.5559513555871,0.861640785299128,3.11699919218724));
#36798=CARTESIAN_POINT('Ctrl Pts',(48.5529452741227,0.861041857828896,1.61024116156234));
#36799=CARTESIAN_POINT('Ctrl Pts',(48.5481105054958,0.861027202313047,0.550173774307906));
#36800=CARTESIAN_POINT('Ctrl Pts',(48.5474362951184,0.860991815439257,0.424583922210125));
#36801=CARTESIAN_POINT('Ctrl Pts',(48.5457145448333,0.860807080018294,0.173133236375915));
#36802=CARTESIAN_POINT('Ctrl Pts',(48.5417872384827,0.860211550198904,-0.266445020311065));
#36803=CARTESIAN_POINT('Ctrl Pts',(48.5339257686467,0.858773503319285,-0.893692784412118));
#36804=CARTESIAN_POINT('Ctrl Pts',(48.522073739976,0.856644410865061,-1.64619413650871));
#36805=CARTESIAN_POINT('Ctrl Pts',(48.5046013324232,0.854081092235267,-2.6492129028255));
#36806=CARTESIAN_POINT('Ctrl Pts',(48.4825692660466,0.85276775254009,-3.90422026265454));
#36807=CARTESIAN_POINT('Ctrl Pts',(48.4707732444907,0.856713137652613,-4.91207054954197));
#36808=CARTESIAN_POINT('Ctrl Pts',(48.4671393010514,0.86149262666492,-5.54219036151472));
#36809=CARTESIAN_POINT('Ctrl Pts',(48.4656067884327,0.860180392622072,-5.74936211818534));
#36810=CARTESIAN_POINT('Ctrl Pts',(48.4623097923741,0.847831923133697,-6.20557559939964));
#36811=CARTESIAN_POINT('Ctrl Pts',(48.4565916177326,0.805002100819759,-7.02772294470306));
#36812=CARTESIAN_POINT('Ctrl Pts',(48.4512469788016,0.714569697331715,-8.31560255293077));
#36813=CARTESIAN_POINT('Ctrl Pts',(48.4548341095276,0.694984707659641,-9.73891151249225));
#36814=CARTESIAN_POINT('Ctrl Pts',(48.4623957231446,0.797083729047604,-10.8079829560626));
#36815=CARTESIAN_POINT('Ctrl Pts',(48.4674917701297,0.901574142012729,-11.4354991653457));
#36816=CARTESIAN_POINT('Ctrl Pts',(48.470106832917,0.971216797118014,-11.75405631707));
#36817=CARTESIAN_POINT('Ctrl Pts',(48.4719992565174,1.03103416280663,-11.9955684581337));
#36818=CARTESIAN_POINT('Ctrl Pts',(48.4735291927885,1.07554025132908,-12.1651232691922));
#36819=CARTESIAN_POINT('Ctrl Pts',(48.4781552422806,1.1730200512042,-12.4927762950991));
#36820=CARTESIAN_POINT('Ctrl Pts',(48.4894872425771,1.36616230530559,-13.0522310028272));
#36821=CARTESIAN_POINT('Ctrl Pts',(48.5307186041763,1.95537885648209,-14.4052094810502));
#36822=CARTESIAN_POINT('Ctrl Pts',(48.5887220196266,2.75812147069433,-15.7094927741229));
#36823=CARTESIAN_POINT('Ctrl Pts',(48.6282107283581,3.45803842130641,-16.886201252276));
#36824=CARTESIAN_POINT('Ctrl Pts',(48.6396659611502,3.76548212629837,-17.4418553275266));
#36825=CARTESIAN_POINT('Ctrl Pts',(48.6402425297031,3.97331324839344,-17.8666263159455));
#36826=CARTESIAN_POINT('Ctrl Pts',(48.6368572480079,4.06259835365295,-18.0714978409077));
#36827=CARTESIAN_POINT('Ctrl Pts',(48.6324201979839,4.12337131538699,-18.2225466256693));
#36828=CARTESIAN_POINT('Ctrl Pts',(48.6234599825036,4.17457310433057,-18.3554234639945));
#36829=CARTESIAN_POINT('Ctrl Pts',(48.6055384286344,4.2684151651007,-18.6015930401312));
#36830=CARTESIAN_POINT('Ctrl Pts',(48.5821426501547,4.36198237974832,-18.8543700374838));
#36831=CARTESIAN_POINT('Ctrl Pts',(48.5554552185872,4.45142617483105,-19.102468133947));
#36832=CARTESIAN_POINT('Ctrl Pts',(48.5371054458672,4.50646811323497,-19.2579465929906));
#36833=CARTESIAN_POINT('Ctrl Pts',(48.5216094979501,4.5496941905776,-19.3817120668446));
#36834=CARTESIAN_POINT('Ctrl Pts',(48.5055367762919,4.59249085270137,-19.5053556776613));
#36835=CARTESIAN_POINT('Ctrl Pts',(48.4591184085395,4.70826835596746,-19.8443953493771));
#36836=CARTESIAN_POINT('Ctrl Pts',(48.3716444075612,4.88748874179812,-20.3934917640079));
#36837=CARTESIAN_POINT('Ctrl Pts',(48.1940359446113,5.177547094172,-21.3481529136738));
#36838=CARTESIAN_POINT('Ctrl Pts',(47.952649797924,5.48916359536832,-22.4914429176204));
#36839=CARTESIAN_POINT('Ctrl Pts',(47.8053384773659,5.67598473315981,-23.3545050106478));
#36840=CARTESIAN_POINT('Ctrl Pts',(47.7514393521066,5.76105663332847,-23.8814135650254));
#36841=CARTESIAN_POINT('Ctrl Pts',(47.7322571534499,5.78789453914611,-24.0780537403835));
#36842=CARTESIAN_POINT('Ctrl Pts',(47.7005023093246,5.83108303792997,-24.4891702584617));
#36843=CARTESIAN_POINT('Ctrl Pts',(47.6618055586385,5.87479485277564,-25.2313840795511));
#36844=CARTESIAN_POINT('Ctrl Pts',(47.6464171221041,5.86067949330697,-26.3718984732227));
#36845=CARTESIAN_POINT('Ctrl Pts',(47.661414214751,5.77854355816339,-27.855477204284));
#36846=CARTESIAN_POINT('Ctrl Pts',(47.6743009899302,5.73560298664759,-28.9198483764603));
#36847=CARTESIAN_POINT('Ctrl Pts',(47.6769703884333,5.73345395831467,-29.5380349652942));
#36848=CARTESIAN_POINT('Ctrl Pts',(47.677730957727,5.73299139472617,-29.6586445118241));
#36849=CARTESIAN_POINT('Ctrl Pts',(47.6798311884685,5.73185060628414,-29.9094857286936));
#36850=CARTESIAN_POINT('Ctrl Pts',(47.6849815494086,5.72942607414121,-30.3441072350726));
#36851=CARTESIAN_POINT('Ctrl Pts',(47.700527716251,5.72310267988212,-31.2186109898455));
#36852=CARTESIAN_POINT('Ctrl Pts',(47.7275269135778,5.71386386515405,-32.2190485708557));
#36853=CARTESIAN_POINT('Ctrl Pts',(47.7580119655262,5.70498183675231,-33.2226063845043));
#36854=CARTESIAN_POINT('Ctrl Pts',(47.781155007125,5.6989158027578,-33.9757793462538));
#36855=CARTESIAN_POINT('Ctrl Pts',(47.8031479086886,5.69373349890801,-34.7293605181625));
#36856=CARTESIAN_POINT('Ctrl Pts',(47.8160572371253,5.69105684482747,-35.2317860159007));
#36857=CARTESIAN_POINT('Ctrl Pts',(47.8247353087206,5.68939382962639,-35.609540706168));
#36858=CARTESIAN_POINT('Ctrl Pts',(47.8306340228238,5.68825044481764,-35.8607462274074));
#36859=CARTESIAN_POINT('Ctrl Pts',(47.8426692085815,5.68610487362212,-36.3636193365152));
#36860=CARTESIAN_POINT('Ctrl Pts',(47.8642093266045,5.6825643968688,-37.2418078118721));
#36861=CARTESIAN_POINT('Ctrl Pts',(47.9074925473444,5.67682038379547,-38.9956446854038));
#36862=CARTESIAN_POINT('Ctrl Pts',(47.9397934253085,5.67429448183844,-40.5002676053438));
#36863=CARTESIAN_POINT('Ctrl Pts',(47.9562383458176,5.67422694979235,-41.6352193462152));
#36864=CARTESIAN_POINT('Ctrl Pts',(47.9596673293312,5.67407137046705,-41.8832711523324));
#36865=CARTESIAN_POINT('Ctrl Pts',(47.9642819516124,5.67346258469438,-42.2577363877267));
#36866=CARTESIAN_POINT('Ctrl Pts',(47.9684051278346,5.6725968579029,-42.6326543517452));
#36867=CARTESIAN_POINT('Ctrl Pts',(47.9733073965259,5.67123657835768,-43.1339856927694));
#36868=CARTESIAN_POINT('Ctrl Pts',(47.9784245457529,5.66942716097581,-43.7625706582561));
#36869=CARTESIAN_POINT('Ctrl Pts',(47.9832885466205,5.66795036229496,-44.519662645377));
#36870=CARTESIAN_POINT('Ctrl Pts',(47.9865607651011,5.66802931005178,-45.1523870811576));
#36871=CARTESIAN_POINT('Ctrl Pts',(47.9888833465312,5.66933836408497,-45.6594096396806));
#36872=CARTESIAN_POINT('Ctrl Pts',(47.9905180716937,5.67104737260073,-46.0400472212068));
#36873=CARTESIAN_POINT('Ctrl Pts',(47.9920879918475,5.67359670763986,-46.4209707502011));
#36874=CARTESIAN_POINT('Ctrl Pts',(47.9941558677818,5.6782725369688,-46.9292389144956));
#36875=CARTESIAN_POINT('Ctrl Pts',(47.9957282263367,5.68336945103735,-47.310588569819));
#36876=CARTESIAN_POINT('Ctrl Pts',(47.997419450837,5.6897951869272,-47.6933797259154));
#36877=CARTESIAN_POINT('Ctrl Pts',(47.9983626666677,5.69589731397596,-47.9631838583766));
#36878=CARTESIAN_POINT('Ctrl Pts',(47.9997584629324,5.71311725397261,-48.4892701742966));
#36879=CARTESIAN_POINT('Ctrl Pts',(48.0011105924857,5.75402758165737,-49.4003616751971));
#36880=CARTESIAN_POINT('Ctrl Pts',(48.001392732923,5.82718212090007,-50.6594925731589));
#36881=CARTESIAN_POINT('Ctrl Pts',(48.0029449168854,5.89268556163609,-52.1071136716778));
#36882=CARTESIAN_POINT('Ctrl Pts',(48.0066715561608,5.89448880236947,-53.0268738746101));
#36883=CARTESIAN_POINT('Ctrl Pts',(48.0103335225241,5.87538737072239,-53.5876646128138));
#36884=CARTESIAN_POINT('Ctrl Pts',(48.011754185608,5.86483201236299,-53.7869517653904));
#36885=CARTESIAN_POINT('Ctrl Pts',(48.0150741130896,5.82900693060963,-54.2179462873563));
#36886=CARTESIAN_POINT('Ctrl Pts',(48.022185167171,5.73211236749528,-55.0027680394616));
#36887=CARTESIAN_POINT('Ctrl Pts',(48.0421436387735,5.44406860609416,-56.7238524205714));
#36888=CARTESIAN_POINT('Ctrl Pts',(48.0651576831185,5.19660981902691,-58.4361828195335));
#36889=CARTESIAN_POINT('Ctrl Pts',(48.0720910374252,5.27841745278614,-59.7710607470195));
#36890=CARTESIAN_POINT('Ctrl Pts',(48.0730274273232,5.28820917419853,-59.9126626681764));
#36891=CARTESIAN_POINT('Ctrl Pts',(48.074762526789,5.31234741047462,-60.2063371455483));
#36892=CARTESIAN_POINT('Ctrl Pts',(48.0776426768627,5.36420511218112,-60.7119239980234));
#36893=CARTESIAN_POINT('Ctrl Pts',(48.082684035864,5.5056353556155,-61.7166202365291));
#36894=CARTESIAN_POINT('Ctrl Pts',(48.0870397172443,5.74237823822888,-62.836120016294));
#36895=CARTESIAN_POINT('Ctrl Pts',(48.0902520185111,6.03501840008531,-63.9282554061026));
#36896=CARTESIAN_POINT('Ctrl Pts',(48.0916806212538,6.21723766416966,-64.5313278074762));
#36897=CARTESIAN_POINT('Ctrl Pts',(48.0924968060045,6.34467449486511,-64.9287081323857));
#36898=CARTESIAN_POINT('Ctrl Pts',(48.0930072141367,6.43113049693596,-65.1923259081768));
#36899=CARTESIAN_POINT('Ctrl Pts',(48.0934638368336,6.51973347346149,-65.4541179476157));
#36900=CARTESIAN_POINT('Ctrl Pts',(48.093826305083,6.59887034019588,-65.6814185423467));
#36901=CARTESIAN_POINT('Ctrl Pts',(48.0940229585271,6.64452074292956,-65.8108056498808));
#36902=CARTESIAN_POINT('Ctrl Pts',(48.0943068714726,6.7134200076301,-66.0044116477408));
#36903=CARTESIAN_POINT('Ctrl Pts',(48.0945234125043,6.77165114316365,-66.1646751482884));
#36904=CARTESIAN_POINT('Ctrl Pts',(48.0948355742627,6.8692273883312,-66.4292657126974));
#36905=CARTESIAN_POINT('Ctrl Pts',(48.0938628546097,6.98678481260344,-66.7337843123861));
#36906=CARTESIAN_POINT('Ctrl Pts',(48.0923533388769,7.22918372170347,-67.3107532529164));
#36907=CARTESIAN_POINT('Ctrl Pts',(48.0889709500158,7.68894236374983,-68.2993244133904));
#36908=CARTESIAN_POINT('Ctrl Pts',(48.0826493213745,8.69064771492824,-70.1574922702234));
#36909=CARTESIAN_POINT('Ctrl Pts',(48.0816614082155,9.56601796591246,-71.6177358852099));
#36910=CARTESIAN_POINT('Ctrl Pts',(48.085543824311,10.1195969025733,-72.6699364937867));
#36911=CARTESIAN_POINT('Ctrl Pts',(48.0852262519432,10.2552982719922,-72.9276374691411));
#36912=CARTESIAN_POINT('Ctrl Pts',(48.0852742552101,10.5201259865344,-73.4292146285592));
#36913=CARTESIAN_POINT('Ctrl Pts',(48.0850639260234,10.8547194339244,-74.0609721479818));
#36914=CARTESIAN_POINT('Ctrl Pts',(48.0849846417621,11.255413651863,-74.8148744822692));
#36915=CARTESIAN_POINT('Ctrl Pts',(48.0847855778271,12.0585639136749,-76.322457536711));
#36916=CARTESIAN_POINT('Ctrl Pts',(48.0847626220492,12.727963631217,-77.5750090039331));
#36917=CARTESIAN_POINT('Ctrl Pts',(48.0849474724551,13.6958717398979,-79.3955503463575));
#36918=CARTESIAN_POINT('Ctrl Pts',(48.0848656797528,14.1332269587404,-80.2182153328694));
#36919=CARTESIAN_POINT('Ctrl Pts',(48.0848656797527,14.5697485461299,-81.0391930349677));
#36920=CARTESIAN_POINT('Ctrl Pts',(50.9533414312497,1.12169071707122,24.8307796472817));
#36921=CARTESIAN_POINT('Ctrl Pts',(50.9534901764155,1.12170400700989,24.7819050388184));
#36922=CARTESIAN_POINT('Ctrl Pts',(50.953646180446,1.12171793023201,24.7330314904674));
#36923=CARTESIAN_POINT('Ctrl Pts',(50.9554886331472,1.12188331301799,24.1824813080586));
#36924=CARTESIAN_POINT('Ctrl Pts',(50.9568037911128,1.12192969540982,23.1784285843174));
#36925=CARTESIAN_POINT('Ctrl Pts',(50.9597987208206,1.12197063286745,21.1699357727456));
#36926=CARTESIAN_POINT('Ctrl Pts',(50.9720658618345,1.12308148654311,19.6658745886222));
#36927=CARTESIAN_POINT('Ctrl Pts',(50.9985674054642,1.1258424345923,18.4148754873179));
#36928=CARTESIAN_POINT('Ctrl Pts',(51.0112520755239,1.12712387007124,17.9124041050695));
#36929=CARTESIAN_POINT('Ctrl Pts',(51.0430661893009,1.13026647803661,16.908669997413));
#36930=CARTESIAN_POINT('Ctrl Pts',(51.1113415352745,1.13702052481593,15.1548258190807));
#36931=CARTESIAN_POINT('Ctrl Pts',(51.1766555159717,1.14402473626949,13.6521353545183));
#36932=CARTESIAN_POINT('Ctrl Pts',(51.2183870703309,1.14951437683359,12.3963078248059));
#36933=CARTESIAN_POINT('Ctrl Pts',(51.235547919752,1.15188249177447,11.8947916948912));
#36934=CARTESIAN_POINT('Ctrl Pts',(51.2708493229605,1.15710724391015,10.8921720267516));
#36935=CARTESIAN_POINT('Ctrl Pts',(51.3325796691209,1.16697185670893,9.13793432471975));
#36936=CARTESIAN_POINT('Ctrl Pts',(51.3764456484271,1.17473756336112,7.63357884883048));
#36937=CARTESIAN_POINT('Ctrl Pts',(51.3958297044449,1.17830805322875,6.50362118199104));
#36938=CARTESIAN_POINT('Ctrl Pts',(51.399831792773,1.17909826536064,6.25298174706968));
#36939=CARTESIAN_POINT('Ctrl Pts',(51.4067582655738,1.18064161126168,5.75153364143083));
#36940=CARTESIAN_POINT('Ctrl Pts',(51.4162015581993,1.18320978341969,4.87277716219866));
#36941=CARTESIAN_POINT('Ctrl Pts',(51.4255816469843,1.18742443036854,3.1132027445773));
#36942=CARTESIAN_POINT('Ctrl Pts',(51.4214908702378,1.18825181340388,1.61014543257973));
#36943=CARTESIAN_POINT('Ctrl Pts',(51.4169517383915,1.18646483593497,0.554414579386592));
#36944=CARTESIAN_POINT('Ctrl Pts',(51.4162990444907,1.18612419515353,0.431150301349283));
#36945=CARTESIAN_POINT('Ctrl Pts',(51.414576836636,1.18498720001586,0.182960482925087));
#36946=CARTESIAN_POINT('Ctrl Pts',(51.4105458029336,1.18190336825363,-0.25122582412197));
#36947=CARTESIAN_POINT('Ctrl Pts',(51.4023164143969,1.17502534226266,-0.873508478834048));
#36948=CARTESIAN_POINT('Ctrl Pts',(51.3899042130627,1.16476018757087,-1.62381014900014));
#36949=CARTESIAN_POINT('Ctrl Pts',(51.3718111002335,1.15118447847443,-2.62905519833519));
#36950=CARTESIAN_POINT('Ctrl Pts',(51.3498278423123,1.13925829229423,-3.8963786857563));
#36951=CARTESIAN_POINT('Ctrl Pts',(51.3406458821957,1.14652303269977,-4.92479211904332));
#36952=CARTESIAN_POINT('Ctrl Pts',(51.3399421908936,1.15995176317395,-5.57074037590767));
#36953=CARTESIAN_POINT('Ctrl Pts',(51.340422865111,1.16145463660532,-5.77681590727876));
#36954=CARTESIAN_POINT('Ctrl Pts',(51.3435729933499,1.15593856293644,-6.23612305337799));
#36955=CARTESIAN_POINT('Ctrl Pts',(51.3542468918493,1.12717613767436,-7.06406249501279));
#36956=CARTESIAN_POINT('Ctrl Pts',(51.3792368604421,1.06537306299732,-8.369130274419));
#36957=CARTESIAN_POINT('Ctrl Pts',(51.4015165176634,1.09673867444157,-9.82000774660129));
#36958=CARTESIAN_POINT('Ctrl Pts',(51.4020940342134,1.25347239491636,-10.9088988545458));
#36959=CARTESIAN_POINT('Ctrl Pts',(51.3955285966775,1.39472579842456,-11.545811398602));
#36960=CARTESIAN_POINT('Ctrl Pts',(51.3895806268922,1.4844434139763,-11.8680296924352));
#36961=CARTESIAN_POINT('Ctrl Pts',(51.383914084086,1.56008462901172,-12.112179992416));
#36962=CARTESIAN_POINT('Ctrl Pts',(51.3787279145381,1.6205720606341,-12.2947773166795));
#36963=CARTESIAN_POINT('Ctrl Pts',(51.368258303711,1.7496111927712,-12.6374803765801));
#36964=CARTESIAN_POINT('Ctrl Pts',(51.3480317930404,2.00341957948846,-13.217974870139));
#36965=CARTESIAN_POINT('Ctrl Pts',(51.2907428732227,2.75321150640632,-14.5831452083601));
#36966=CARTESIAN_POINT('Ctrl Pts',(51.225927360633,3.71750324084946,-15.8769039999603));
#36967=CARTESIAN_POINT('Ctrl Pts',(51.1888189023664,4.47867445749755,-17.016310178288));
#36968=CARTESIAN_POINT('Ctrl Pts',(51.1773022292006,4.78348110038424,-17.5314003101878));
#36969=CARTESIAN_POINT('Ctrl Pts',(51.1707092735231,4.96826566080369,-17.9033559813948));
#36970=CARTESIAN_POINT('Ctrl Pts',(51.167454142606,5.03970800806079,-18.0727299228598));
#36971=CARTESIAN_POINT('Ctrl Pts',(51.164531635878,5.08534082856387,-18.1933732667152));
#36972=CARTESIAN_POINT('Ctrl Pts',(51.158686915049,5.12560921907512,-18.3048956728737));
#36973=CARTESIAN_POINT('Ctrl Pts',(51.1474140167638,5.19548384510815,-18.5104348774773));
#36974=CARTESIAN_POINT('Ctrl Pts',(51.1330526263263,5.26178877509215,-18.7241888721022));
#36975=CARTESIAN_POINT('Ctrl Pts',(51.1169928924075,5.3213202709279,-18.9358738736356));
#36976=CARTESIAN_POINT('Ctrl Pts',(51.106045628326,5.35663218644509,-19.0696324172117));
#36977=CARTESIAN_POINT('Ctrl Pts',(51.0968633257256,5.38353229315555,-19.176746821762));
#36978=CARTESIAN_POINT('Ctrl Pts',(51.0873780885147,5.40965947712826,-19.284228081506));
#36979=CARTESIAN_POINT('Ctrl Pts',(51.0601357208132,5.4782355126452,-19.5808333938109));
#36980=CARTESIAN_POINT('Ctrl Pts',(51.0097682006336,5.57392886357255,-20.0728055332414));
#36981=CARTESIAN_POINT('Ctrl Pts',(50.9108460793228,5.70812600387179,-20.9684285024396));
#36982=CARTESIAN_POINT('Ctrl Pts',(50.7852015582486,5.82953407015952,-22.1344590978249));
#36983=CARTESIAN_POINT('Ctrl Pts',(50.714933507944,5.9081193598174,-23.1223234035987));
#36984=CARTESIAN_POINT('Ctrl Pts',(50.6888867590884,5.95993419098196,-23.7523420878989));
#36985=CARTESIAN_POINT('Ctrl Pts',(50.6801530113606,5.97429674512249,-23.9610482578587));
#36986=CARTESIAN_POINT('Ctrl Pts',(50.6669866029258,5.99623030389602,-24.4094074853637));
#36987=CARTESIAN_POINT('Ctrl Pts',(50.6546421899526,6.01225316678561,-25.2004327933986));
#36988=CARTESIAN_POINT('Ctrl Pts',(50.6606348920818,5.9876694949273,-26.3899162922315));
#36989=CARTESIAN_POINT('Ctrl Pts',(50.684070508213,5.92753779169261,-27.8927229744253));
#36990=CARTESIAN_POINT('Ctrl Pts',(50.6946061788475,5.90351872157916,-28.9465159456603));
#36991=CARTESIAN_POINT('Ctrl Pts',(50.6942533930777,5.90583493545004,-29.5519213155557));
#36992=CARTESIAN_POINT('Ctrl Pts',(50.6941500063852,5.90638391616636,-29.6768765989556));
#36993=CARTESIAN_POINT('Ctrl Pts',(50.6938822422483,5.90784051357585,-29.9320358454859));
#36994=CARTESIAN_POINT('Ctrl Pts',(50.6932605144441,5.9112054457662,-30.3754974172379));
#36995=CARTESIAN_POINT('Ctrl Pts',(50.6915185025583,5.92079918480938,-31.263020330328));
#36996=CARTESIAN_POINT('Ctrl Pts',(50.6889589583413,5.93649274814956,-32.2721514614383));
#36997=CARTESIAN_POINT('Ctrl Pts',(50.6869089393234,5.95321919885304,-33.2768405612288));
#36998=CARTESIAN_POINT('Ctrl Pts',(50.6859214788548,5.9654443733994,-34.0274257354587));
#36999=CARTESIAN_POINT('Ctrl Pts',(50.6858143945714,5.97664950657486,-34.7748619142795));
#37000=CARTESIAN_POINT('Ctrl Pts',(50.6865215248918,5.98289729769915,-35.270809249299));
#37001=CARTESIAN_POINT('Ctrl Pts',(50.6874148224352,5.98693541830552,-35.6429107206182));
#37002=CARTESIAN_POINT('Ctrl Pts',(50.6881567784551,5.98963164038767,-35.8943972430752));
#37003=CARTESIAN_POINT('Ctrl Pts',(50.690149158942,5.99481400010558,-36.3955360652468));
#37004=CARTESIAN_POINT('Ctrl Pts',(50.6948421222203,6.00354382030804,-37.2717999859299));
#37005=CARTESIAN_POINT('Ctrl Pts',(50.7075036636841,6.0193133879144,-39.0208470267752));
#37006=CARTESIAN_POINT('Ctrl Pts',(50.7193810329234,6.03097958496215,-40.5211261071569));
#37007=CARTESIAN_POINT('Ctrl Pts',(50.7239599109397,6.03914737439431,-41.6524715377103));
#37008=CARTESIAN_POINT('Ctrl Pts',(50.7248327254382,6.04072159743099,-41.9001262239914));
#37009=CARTESIAN_POINT('Ctrl Pts',(50.7258014357219,6.0426204028929,-42.2737142037943));
#37010=CARTESIAN_POINT('Ctrl Pts',(50.7264855424824,6.04412897403735,-42.6477530920575));
#37011=CARTESIAN_POINT('Ctrl Pts',(50.7270960595622,6.04576002792844,-43.1477711460489));
#37012=CARTESIAN_POINT('Ctrl Pts',(50.7274392596561,6.04731681597243,-43.7745513505533));
#37013=CARTESIAN_POINT('Ctrl Pts',(50.7276394978465,6.04918560965412,-44.5291835300691));
#37014=CARTESIAN_POINT('Ctrl Pts',(50.728013587656,6.05138931244001,-45.1596246848687));
#37015=CARTESIAN_POINT('Ctrl Pts',(50.7286772908058,6.05392767731241,-45.6647115464628));
#37016=CARTESIAN_POINT('Ctrl Pts',(50.7294097819383,6.05631812303614,-46.043824985108));
#37017=CARTESIAN_POINT('Ctrl Pts',(50.7304347944595,6.05929220166793,-46.4231538169804));
#37018=CARTESIAN_POINT('Ctrl Pts',(50.7322745208644,6.06417377448445,-46.9292097864943));
#37019=CARTESIAN_POINT('Ctrl Pts',(50.7342515600158,6.06899420874078,-47.3087654766622));
#37020=CARTESIAN_POINT('Ctrl Pts',(50.7367700662269,6.07482707758255,-47.6896844161141));
#37021=CARTESIAN_POINT('Ctrl Pts',(50.738506910136,6.08033525938134,-47.9575409942805));
#37022=CARTESIAN_POINT('Ctrl Pts',(50.7422933318491,6.09579700941191,-48.480488180462));
#37023=CARTESIAN_POINT('Ctrl Pts',(50.7497115606343,6.13228903674023,-49.3866831394771));
#37024=CARTESIAN_POINT('Ctrl Pts',(50.7626532705558,6.19631660090494,-50.6412054007193));
#37025=CARTESIAN_POINT('Ctrl Pts',(50.7817833437615,6.24948190302374,-52.0869414693963));
#37026=CARTESIAN_POINT('Ctrl Pts',(50.7964412108546,6.24364500559531,-53.0081849703579));
#37027=CARTESIAN_POINT('Ctrl Pts',(50.8059668372468,6.22038505455988,-53.5707667642567));
#37028=CARTESIAN_POINT('Ctrl Pts',(50.8098281664221,6.20841891443272,-53.7685903339318));
#37029=CARTESIAN_POINT('Ctrl Pts',(50.8183559178301,6.16924089319675,-54.1983830974968));
#37030=CARTESIAN_POINT('Ctrl Pts',(50.8352660608715,6.06557535448727,-54.9814807034273));
#37031=CARTESIAN_POINT('Ctrl Pts',(50.8757576452758,5.76089558294737,-56.7027655854137));
#37032=CARTESIAN_POINT('Ctrl Pts',(50.915202696598,5.496656556801,-58.4195020054296));
#37033=CARTESIAN_POINT('Ctrl Pts',(50.9266780699831,5.57317759167755,-59.76186377409));
#37034=CARTESIAN_POINT('Ctrl Pts',(50.9281192046078,5.58249120781337,-59.9043259989871));
#37035=CARTESIAN_POINT('Ctrl Pts',(50.9306575721336,5.60579772893743,-60.199648203657));
#37036=CARTESIAN_POINT('Ctrl Pts',(50.9344446796052,5.65668455670657,-60.7078780096647));
#37037=CARTESIAN_POINT('Ctrl Pts',(50.9395237932056,5.79772681030116,-61.7169001722879));
#37038=CARTESIAN_POINT('Ctrl Pts',(50.9409631986153,6.03650867779907,-62.8391384168951));
#37039=CARTESIAN_POINT('Ctrl Pts',(50.9403903714156,6.33165112392542,-63.9320017694799));
#37040=CARTESIAN_POINT('Ctrl Pts',(50.9397196268296,6.5151344126419,-64.5347751251295));
#37041=CARTESIAN_POINT('Ctrl Pts',(50.9392943502438,6.6432146121098,-64.9316744184796));
#37042=CARTESIAN_POINT('Ctrl Pts',(50.9390280538705,6.73003968502427,-65.1948956591214));
#37043=CARTESIAN_POINT('Ctrl Pts',(50.9387979083557,6.81890600506985,-65.4561826512923));
#37044=CARTESIAN_POINT('Ctrl Pts',(50.9386625642652,6.89816091629947,-65.6829423491466));
#37045=CARTESIAN_POINT('Ctrl Pts',(50.9386075263059,6.94384315526671,-65.8119923850296));
#37046=CARTESIAN_POINT('Ctrl Pts',(50.9385481095695,7.01275348645454,-66.0050655467178));
#37047=CARTESIAN_POINT('Ctrl Pts',(50.9385539169166,7.0709119129086,-66.1648250278806));
#37048=CARTESIAN_POINT('Ctrl Pts',(50.9386299432502,7.16825163935389,-66.4285222831356));
#37049=CARTESIAN_POINT('Ctrl Pts',(50.9371771379859,7.28589407409485,-66.7331431981932));
#37050=CARTESIAN_POINT('Ctrl Pts',(50.9349480821807,7.52824350147715,-67.3097807941499));
#37051=CARTESIAN_POINT('Ctrl Pts',(50.9304839220131,7.98795765327312,-68.2981545765869));
#37052=CARTESIAN_POINT('Ctrl Pts',(50.9230499483198,8.98941130983985,-70.1559656124676));
#37053=CARTESIAN_POINT('Ctrl Pts',(50.9225279560043,9.86477423134398,-71.6163124623247));
#37054=CARTESIAN_POINT('Ctrl Pts',(50.9269691274999,10.4186322923642,-72.6686895067181));
#37055=CARTESIAN_POINT('Ctrl Pts',(50.9265826329875,10.5543189518767,-72.9263627876053));
#37056=CARTESIAN_POINT('Ctrl Pts',(50.9266146411925,10.8191562096941,-73.4279248486359));
#37057=CARTESIAN_POINT('Ctrl Pts',(50.9263539659393,11.1537373969705,-74.0596550678505));
#37058=CARTESIAN_POINT('Ctrl Pts',(50.9262608462098,11.5544189999126,-74.8135377130594));
#37059=CARTESIAN_POINT('Ctrl Pts',(50.9260519983092,12.3575313978324,-76.3210909010518));
#37060=CARTESIAN_POINT('Ctrl Pts',(50.9260725792638,13.0269046053434,-77.5736611529628));
#37061=CARTESIAN_POINT('Ctrl Pts',(50.9262854692743,13.994843499425,-79.3942538055335));
#37062=CARTESIAN_POINT('Ctrl Pts',(50.9261906789385,14.432188480403,-80.2169075971474));
#37063=CARTESIAN_POINT('Ctrl Pts',(50.9261906789385,14.8687100677924,-81.0378852992458));
#37064=CARTESIAN_POINT('Ctrl Pts',(53.7933900457244,1.46776045816492,24.8308352754981));
#37065=CARTESIAN_POINT('Ctrl Pts',(53.7935558023369,1.46777693452164,24.7819623622908));
#37066=CARTESIAN_POINT('Ctrl Pts',(53.7937296500648,1.46779420749623,24.7330905217149));
#37067=CARTESIAN_POINT('Ctrl Pts',(53.7957820873193,1.46799885980126,24.1825607194227));
#37068=CARTESIAN_POINT('Ctrl Pts',(53.7974363241905,1.46805440166394,23.1785629963308));
#37069=CARTESIAN_POINT('Ctrl Pts',(53.8013468051514,1.4681064766261,21.1700925605004));
#37070=CARTESIAN_POINT('Ctrl Pts',(53.8149997112356,1.46947818305774,19.6659951252516));
#37071=CARTESIAN_POINT('Ctrl Pts',(53.8435465187149,1.47289619177137,18.4149454367022));
#37072=CARTESIAN_POINT('Ctrl Pts',(53.8572984478431,1.47451272292775,17.9124536811641));
#37073=CARTESIAN_POINT('Ctrl Pts',(53.8919413262604,1.47854467572399,16.9087243235041));
#37074=CARTESIAN_POINT('Ctrl Pts',(53.9662447392349,1.48724046780434,15.1549864169005));
#37075=CARTESIAN_POINT('Ctrl Pts',(54.0360578275002,1.49594448733498,13.6523890810428));
#37076=CARTESIAN_POINT('Ctrl Pts',(54.0783673965234,1.50212089892775,12.3965824151409));
#37077=CARTESIAN_POINT('Ctrl Pts',(54.0955109057738,1.50473227021855,11.8950679843877));
#37078=CARTESIAN_POINT('Ctrl Pts',(54.1299634716596,1.51033595700616,10.8924051910278));
#37079=CARTESIAN_POINT('Ctrl Pts',(54.1885336362757,1.52060807428504,9.1380099688249));
#37080=CARTESIAN_POINT('Ctrl Pts',(54.2284304999388,1.52838448388396,7.63358890128757));
#37081=CARTESIAN_POINT('Ctrl Pts',(54.2458099332916,1.53186915181062,6.50371998506009));
#37082=CARTESIAN_POINT('Ctrl Pts',(54.2492828248338,1.53260753050727,6.25318156712738));
#37083=CARTESIAN_POINT('Ctrl Pts',(54.2548893624485,1.53398291082753,5.75186684899312));
#37084=CARTESIAN_POINT('Ctrl Pts',(54.2614845506833,1.53611513211491,4.87329950549318));
#37085=CARTESIAN_POINT('Ctrl Pts',(54.2643379182555,1.53918683799225,3.11387145753909));
#37086=CARTESIAN_POINT('Ctrl Pts',(54.2573995536075,1.53965892925061,1.61025082422581));
#37087=CARTESIAN_POINT('Ctrl Pts',(54.2557401466238,1.53831993636108,0.554383333976408));
#37088=CARTESIAN_POINT('Ctrl Pts',(54.2554784051493,1.53796706602685,0.433343468268538));
#37089=CARTESIAN_POINT('Ctrl Pts',(54.2547074092181,1.53651660057094,0.187972714035989));
#37090=CARTESIAN_POINT('Ctrl Pts',(54.2527674583444,1.53221613334056,-0.241464717897606));
#37091=CARTESIAN_POINT('Ctrl Pts',(54.2485951736577,1.52207359627305,-0.859839813592334));
#37092=CARTESIAN_POINT('Ctrl Pts',(54.2423914644405,1.50688462047672,-1.60938817970641));
#37093=CARTESIAN_POINT('Ctrl Pts',(54.2337678506486,1.48744069579046,-2.61947890070179));
#37094=CARTESIAN_POINT('Ctrl Pts',(54.2247779796255,1.47379799843202,-3.9037136735069));
#37095=CARTESIAN_POINT('Ctrl Pts',(54.2236670013246,1.49465488165937,-4.95631565149324));
#37096=CARTESIAN_POINT('Ctrl Pts',(54.2262007246916,1.52391615578665,-5.62052064335219));
#37097=CARTESIAN_POINT('Ctrl Pts',(54.2284408836682,1.5312744986544,-5.83574805618841));
#37098=CARTESIAN_POINT('Ctrl Pts',(54.2358852067293,1.54106875243503,-6.30994821019978));
#37099=CARTESIAN_POINT('Ctrl Pts',(54.2557903425437,1.54633990549292,-7.15921814904195));
#37100=CARTESIAN_POINT('Ctrl Pts',(54.2949916301286,1.55411524466244,-8.48036615512007));
#37101=CARTESIAN_POINT('Ctrl Pts',(54.32054106886,1.6685408684751,-9.92444849402792));
#37102=CARTESIAN_POINT('Ctrl Pts',(54.3125401600623,1.87358765716265,-10.9933226813509));
#37103=CARTESIAN_POINT('Ctrl Pts',(54.2978284242317,2.03650352741588,-11.6154425790896));
#37104=CARTESIAN_POINT('Ctrl Pts',(54.2867299786695,2.1346535662497,-11.9293507756478));
#37105=CARTESIAN_POINT('Ctrl Pts',(54.2767660804809,2.21568134921396,-12.1672221744866));
#37106=CARTESIAN_POINT('Ctrl Pts',(54.2674574226275,2.2821125766626,-12.3507234833108));
#37107=CARTESIAN_POINT('Ctrl Pts',(54.2483381988399,2.42123276556235,-12.6917517760357));
#37108=CARTESIAN_POINT('Ctrl Pts',(54.2107430146763,2.69229588585007,-13.2699573998623));
#37109=CARTESIAN_POINT('Ctrl Pts',(54.1030026490132,3.48048290088805,-14.6261114160487));
#37110=CARTESIAN_POINT('Ctrl Pts',(53.9770524318318,4.47675841913185,-15.9131448940457));
#37111=CARTESIAN_POINT('Ctrl Pts',(53.8895858536794,5.23570734582795,-17.0367054326486));
#37112=CARTESIAN_POINT('Ctrl Pts',(53.8577495999718,5.52846547248409,-17.537705551924));
#37113=CARTESIAN_POINT('Ctrl Pts',(53.8401597088712,5.69780007321343,-17.8913214151969));
#37114=CARTESIAN_POINT('Ctrl Pts',(53.8336891383102,5.7603034739084,-18.0485034836148));
#37115=CARTESIAN_POINT('Ctrl Pts',(53.8294760043339,5.79918675991689,-18.158710746978));
#37116=CARTESIAN_POINT('Ctrl Pts',(53.8242922855261,5.83336507551644,-18.2601454739158));
#37117=CARTESIAN_POINT('Ctrl Pts',(53.8149854102744,5.89151040863206,-18.4477890497773));
#37118=CARTESIAN_POINT('Ctrl Pts',(53.804751226398,5.94525410329329,-18.643782080729));
#37119=CARTESIAN_POINT('Ctrl Pts',(53.7944218852403,5.99197085515748,-18.8393751415726));
#37120=CARTESIAN_POINT('Ctrl Pts',(53.7877788512421,6.01906761193404,-18.9636069738138));
#37121=CARTESIAN_POINT('Ctrl Pts',(53.782421418259,6.0393069256326,-19.0635424337132));
#37122=CARTESIAN_POINT('Ctrl Pts',(53.7770185795907,6.05869657425846,-19.1641225276032));
#37123=CARTESIAN_POINT('Ctrl Pts',(53.7620375678208,6.1084862383097,-19.4429606103963));
#37124=CARTESIAN_POINT('Ctrl Pts',(53.7369858902576,6.17161183200816,-19.913031472546));
#37125=CARTESIAN_POINT('Ctrl Pts',(53.6934032828376,6.24247369029086,-20.7923851127138));
#37126=CARTESIAN_POINT('Ctrl Pts',(53.6443264410865,6.27322765229458,-21.9784206991347));
#37127=CARTESIAN_POINT('Ctrl Pts',(53.6158452945417,6.29562851322709,-23.0213542879479));
#37128=CARTESIAN_POINT('Ctrl Pts',(53.6028045669425,6.3324843283351,-23.6991333497469));
#37129=CARTESIAN_POINT('Ctrl Pts',(53.5989325122426,6.3427047066574,-23.9180599088565));
#37130=CARTESIAN_POINT('Ctrl Pts',(53.593912842268,6.35920858361621,-24.3890009403331));
#37131=CARTESIAN_POINT('Ctrl Pts',(53.5922803110389,6.37398863179943,-25.2107803923371));
#37132=CARTESIAN_POINT('Ctrl Pts',(53.6044873488314,6.36525379676015,-26.4264350231629));
#37133=CARTESIAN_POINT('Ctrl Pts',(53.6246410636365,6.33362942494894,-27.9280681877689));
#37134=CARTESIAN_POINT('Ctrl Pts',(53.6299854794189,6.31962103324006,-28.9596498518069));
#37135=CARTESIAN_POINT('Ctrl Pts',(53.6275904114776,6.31989336884689,-29.5468372150394));
#37136=CARTESIAN_POINT('Ctrl Pts',(53.6269860187601,6.31996858519039,-29.6714025389371));
#37137=CARTESIAN_POINT('Ctrl Pts',(53.6254590818797,6.32014848759483,-29.9238618153255));
#37138=CARTESIAN_POINT('Ctrl Pts',(53.6220079088107,6.3205644028427,-30.3639320559427));
#37139=CARTESIAN_POINT('Ctrl Pts',(53.6124311150174,6.3217368740878,-31.2451434211193));
#37140=CARTESIAN_POINT('Ctrl Pts',(53.5972125571305,6.32385099937355,-32.2504375748529));
#37141=CARTESIAN_POINT('Ctrl Pts',(53.5815818658841,6.32639839639458,-33.2541968516878));
#37142=CARTESIAN_POINT('Ctrl Pts',(53.5705914377351,6.32840811557273,-34.0057485724029));
#37143=CARTESIAN_POINT('Ctrl Pts',(53.5611950937924,6.33045238168674,-34.7557043762172));
#37144=CARTESIAN_POINT('Ctrl Pts',(53.5566338912338,6.33171857726557,-35.2544416320367));
#37145=CARTESIAN_POINT('Ctrl Pts',(53.5540894921551,6.33258439456126,-35.62899651519));
#37146=CARTESIAN_POINT('Ctrl Pts',(53.5525471172708,6.33314112082372,-35.8803061566907));
#37147=CARTESIAN_POINT('Ctrl Pts',(53.5500721543656,6.33421910065837,-36.3821494728191));
#37148=CARTESIAN_POINT('Ctrl Pts',(53.5470779574238,6.33608019574568,-37.2591841034828));
#37149=CARTESIAN_POINT('Ctrl Pts',(53.5455939632914,6.33963405453553,-39.010344004449));
#37150=CARTESIAN_POINT('Ctrl Pts',(53.5473413277377,6.34321066214864,-40.5124796418315));
#37151=CARTESIAN_POINT('Ctrl Pts',(53.5461525409861,6.34663038394612,-41.6452339196233));
#37152=CARTESIAN_POINT('Ctrl Pts',(53.5458092971824,6.34719150048698,-41.8930044393535));
#37153=CARTESIAN_POINT('Ctrl Pts',(53.5450391848878,6.34762365510011,-42.2669036709439));
#37154=CARTESIAN_POINT('Ctrl Pts',(53.5440878423451,6.3477365541993,-42.641256929972));
#37155=CARTESIAN_POINT('Ctrl Pts',(53.5426497076838,6.34760526561751,-43.1417682640508));
#37156=CARTESIAN_POINT('Ctrl Pts',(53.5406937376445,6.34716654364843,-43.7692597722806));
#37157=CARTESIAN_POINT('Ctrl Pts',(53.5385753322947,6.3470316395596,-44.5249255638812));
#37158=CARTESIAN_POINT('Ctrl Pts',(53.5374029285173,6.3479421810165,-45.1563791848156));
#37159=CARTESIAN_POINT('Ctrl Pts',(53.537080678892,6.3497072495962,-45.6623565642534));
#37160=CARTESIAN_POINT('Ctrl Pts',(53.5371991985082,6.35165485412208,-46.0421851773418));
#37161=CARTESIAN_POINT('Ctrl Pts',(53.537740460393,6.35433187328488,-46.4222756890038));
#37162=CARTESIAN_POINT('Ctrl Pts',(53.5391068127767,6.35902267550402,-46.9294038353548));
#37163=CARTESIAN_POINT('Ctrl Pts',(53.5409466755713,6.36394510200445,-47.309844093545));
#37164=CARTESIAN_POINT('Ctrl Pts',(53.5434576323681,6.37006087923182,-47.6916881569233));
#37165=CARTESIAN_POINT('Ctrl Pts',(53.5452697516784,6.37585970371762,-47.9603598894965));
#37166=CARTESIAN_POINT('Ctrl Pts',(53.5495080101578,6.39220030227994,-48.4846658279806));
#37167=CARTESIAN_POINT('Ctrl Pts',(53.5584241102997,6.43094312194704,-49.392940886843));
#37168=CARTESIAN_POINT('Ctrl Pts',(53.5752247654874,6.49972793378469,-50.6493978653959));
#37169=CARTESIAN_POINT('Ctrl Pts',(53.6002412032182,6.55964718560622,-52.0960064010703));
#37170=CARTESIAN_POINT('Ctrl Pts',(53.6188318440274,6.55826208339829,-53.016900991182));
#37171=CARTESIAN_POINT('Ctrl Pts',(53.6304012698521,6.53753738298099,-53.5790092140046));
#37172=CARTESIAN_POINT('Ctrl Pts',(53.6351414755496,6.5264928871424,-53.7776482020704));
#37173=CARTESIAN_POINT('Ctrl Pts',(53.6455211434246,6.48948253197531,-54.2082493994463));
#37174=CARTESIAN_POINT('Ctrl Pts',(53.6659362726158,6.3902315350268,-54.9924992521234));
#37175=CARTESIAN_POINT('Ctrl Pts',(53.7135446693902,6.09630159129917,-56.7140924202626));
#37176=CARTESIAN_POINT('Ctrl Pts',(53.7588224207161,5.84296406092708,-58.4280717306404));
#37177=CARTESIAN_POINT('Ctrl Pts',(53.7715265525107,5.92253095411376,-59.7656862880565));
#37178=CARTESIAN_POINT('Ctrl Pts',(53.7731098754717,5.93214130941908,-59.9076934093206));
#37179=CARTESIAN_POINT('Ctrl Pts',(53.7758477299353,5.95594634872873,-60.2020912589034));
#37180=CARTESIAN_POINT('Ctrl Pts',(53.7798031476919,6.00740754199605,-60.7088605570528));
#37181=CARTESIAN_POINT('Ctrl Pts',(53.7845465584611,6.14860899244848,-61.7154641107162));
#37182=CARTESIAN_POINT('Ctrl Pts',(53.7844974228809,6.38599143747069,-62.8361597252832));
#37183=CARTESIAN_POINT('Ctrl Pts',(53.782103117691,6.67941249081592,-63.9285556400314));
#37184=CARTESIAN_POINT('Ctrl Pts',(53.7804151278263,6.86200279820823,-64.5314370204442));
#37185=CARTESIAN_POINT('Ctrl Pts',(53.7793721012228,6.98960307318282,-64.9285492426614));
#37186=CARTESIAN_POINT('Ctrl Pts',(53.7787120750193,7.07614332109049,-65.1919500989433));
#37187=CARTESIAN_POINT('Ctrl Pts',(53.7781246786664,7.16478566240634,-65.4534694683211));
#37188=CARTESIAN_POINT('Ctrl Pts',(53.7777139998342,7.24391099674154,-65.6804796823406));
#37189=CARTESIAN_POINT('Ctrl Pts',(53.7775140585173,7.28954006843651,-65.8096859661748));
#37190=CARTESIAN_POINT('Ctrl Pts',(53.7772499665168,7.35839217565976,-66.0030060923424));
#37191=CARTESIAN_POINT('Ctrl Pts',(53.7771150576058,7.41654978603355,-66.1629991209093));
#37192=CARTESIAN_POINT('Ctrl Pts',(53.7769979165408,7.51395562087826,-66.427107494371));
#37193=CARTESIAN_POINT('Ctrl Pts',(53.7751874557642,7.63141908140791,-66.7316106167228));
#37194=CARTESIAN_POINT('Ctrl Pts',(53.7723977403619,7.87358550472339,-67.3083260406967));
#37195=CARTESIAN_POINT('Ctrl Pts',(53.7670738293403,8.33298337809634,-68.2966866318741));
#37196=CARTESIAN_POINT('Ctrl Pts',(53.7586764378322,9.33414718261013,-70.1546037975584));
#37197=CARTESIAN_POINT('Ctrl Pts',(53.7585265782219,10.2095682818923,-71.614903576176));
#37198=CARTESIAN_POINT('Ctrl Pts',(53.7635280769974,10.7635283311995,-72.6672679359216));
#37199=CARTESIAN_POINT('Ctrl Pts',(53.7630829827452,10.8991987161,-72.9249502223087));
#37200=CARTESIAN_POINT('Ctrl Pts',(53.7631089119421,11.1640305013954,-73.4265223596093));
#37201=CARTESIAN_POINT('Ctrl Pts',(53.7628077454296,11.4986013205934,-74.058263832652));
#37202=CARTESIAN_POINT('Ctrl Pts',(53.7627016274684,11.8992841241948,-74.8121559447717));
#37203=CARTESIAN_POINT('Ctrl Pts',(53.762474296671,12.7024066212994,-76.3197212892488));
#37204=CARTESIAN_POINT('Ctrl Pts',(53.7625230103868,13.3717985159555,-77.5722797674868));
#37205=CARTESIAN_POINT('Ctrl Pts',(53.7627689020525,14.339732295039,-79.3928477645874));
#37206=CARTESIAN_POINT('Ctrl Pts',(53.7626628569048,14.7770769853391,-80.2155062080978));
#37207=CARTESIAN_POINT('Ctrl Pts',(53.7626628569049,15.2135985727285,-81.0364839101962));
#37208=CARTESIAN_POINT('Ctrl Pts',(56.6218989148777,1.85136045892844,24.8303065944882));
#37209=CARTESIAN_POINT('Ctrl Pts',(56.6220771833207,1.8513933644215,24.7814170542443));
#37210=CARTESIAN_POINT('Ctrl Pts',(56.622264131534,1.85142783688204,24.7325282854523));
#37211=CARTESIAN_POINT('Ctrl Pts',(56.6244717180094,1.85183601777454,24.1818031689162));
#37212=CARTESIAN_POINT('Ctrl Pts',(56.6263912820124,1.85233537909756,23.1775913604908));
#37213=CARTESIAN_POINT('Ctrl Pts',(56.6310067747904,1.85360135311401,21.1687553754193));
#37214=CARTESIAN_POINT('Ctrl Pts',(56.6456881661146,1.85632073692509,19.6645212396936));
#37215=CARTESIAN_POINT('Ctrl Pts',(56.6756903415303,1.86116033574717,18.4133891312005));
#37216=CARTESIAN_POINT('Ctrl Pts',(56.6901384311248,1.86357764549357,17.9098148785836));
#37217=CARTESIAN_POINT('Ctrl Pts',(56.7265093495165,1.86981416184756,16.9053229544563));
#37218=CARTESIAN_POINT('Ctrl Pts',(56.8044375131954,1.88316195303333,15.151722306397));
#37219=CARTESIAN_POINT('Ctrl Pts',(56.8773956848199,1.89449466324763,13.6525968306754));
#37220=CARTESIAN_POINT('Ctrl Pts',(56.921265128377,1.89914134215809,12.4013060922215));
#37221=CARTESIAN_POINT('Ctrl Pts',(56.9389620475575,1.90076308177012,11.901612767735));
#37222=CARTESIAN_POINT('Ctrl Pts',(56.9743051959492,1.90317797601583,10.9016108579509));
#37223=CARTESIAN_POINT('Ctrl Pts',(57.034010618561,1.90550671368578,9.14974706828727));
#37224=CARTESIAN_POINT('Ctrl Pts',(57.0746529435287,1.90518299224461,7.64372762768176));
#37225=CARTESIAN_POINT('Ctrl Pts',(57.0928779107252,1.90472166370263,6.51106889119965));
#37226=CARTESIAN_POINT('Ctrl Pts',(57.0965545657406,1.90452184313184,6.26176998816713));
#37227=CARTESIAN_POINT('Ctrl Pts',(57.1025967913818,1.90372493647001,5.76145095156286));
#37228=CARTESIAN_POINT('Ctrl Pts',(57.1100127971147,1.90147511564108,4.8841688074548));
#37229=CARTESIAN_POINT('Ctrl Pts',(57.1144126516609,1.89495506678394,3.12306096709394));
#37230=CARTESIAN_POINT('Ctrl Pts',(57.1081276593196,1.89054359979989,1.6115137914328));
#37231=CARTESIAN_POINT('Ctrl Pts',(57.1069369197323,1.89320424839432,0.546521002695334));
#37232=CARTESIAN_POINT('Ctrl Pts',(57.106704640349,1.89326396927256,0.42677368248937));
#37233=CARTESIAN_POINT('Ctrl Pts',(57.105906670196,1.89255411914581,0.182312017995565));
#37234=CARTESIAN_POINT('Ctrl Pts',(57.1037086906732,1.8893227496753,-0.245594539443753));
#37235=CARTESIAN_POINT('Ctrl Pts',(57.0986874322489,1.88041914765443,-0.864388880861254));
#37236=CARTESIAN_POINT('Ctrl Pts',(57.0909501720941,1.86725111695377,-1.61725535047182));
#37237=CARTESIAN_POINT('Ctrl Pts',(57.0799735255966,1.85266345272848,-2.63578860558777));
#37238=CARTESIAN_POINT('Ctrl Pts',(57.0681913152057,1.85142399966878,-3.93733882694326));
#37239=CARTESIAN_POINT('Ctrl Pts',(57.0686411870943,1.89755313172173,-5.01284603289817));
#37240=CARTESIAN_POINT('Ctrl Pts',(57.0741424054941,1.95119902184825,-5.69407227824501));
#37241=CARTESIAN_POINT('Ctrl Pts',(57.0782656048781,1.96836152596059,-5.92460398166542));
#37242=CARTESIAN_POINT('Ctrl Pts',(57.0907803209698,2.00331382182396,-6.42029618339497));
#37243=CARTESIAN_POINT('Ctrl Pts',(57.1223303131829,2.06396544800755,-7.29947588536513));
#37244=CARTESIAN_POINT('Ctrl Pts',(57.1805869280693,2.17680119997923,-8.63277978217996));
#37245=CARTESIAN_POINT('Ctrl Pts',(57.21879850434,2.39766107156909,-10.0481344865149));
#37246=CARTESIAN_POINT('Ctrl Pts',(57.2134878411633,2.65103974697223,-11.075163438603));
#37247=CARTESIAN_POINT('Ctrl Pts',(57.1983971901738,2.82981595871338,-11.6693844706438));
#37248=CARTESIAN_POINT('Ctrl Pts',(57.1864490593766,2.93141090109854,-11.9683787979901));
#37249=CARTESIAN_POINT('Ctrl Pts',(57.1755589950791,3.01318387312317,-12.1949656678289));
#37250=CARTESIAN_POINT('Ctrl Pts',(57.1646377021369,3.08088821895302,-12.3737291910729));
#37251=CARTESIAN_POINT('Ctrl Pts',(57.1424372935763,3.2203090751832,-12.7050339750465));
#37252=CARTESIAN_POINT('Ctrl Pts',(57.098431329832,3.48882736888547,-13.269798702969));
#37253=CARTESIAN_POINT('Ctrl Pts',(56.9714234943707,4.25784184103255,-14.6037208208315));
#37254=CARTESIAN_POINT('Ctrl Pts',(56.8215683084829,5.2117799632523,-15.8851297462418));
#37255=CARTESIAN_POINT('Ctrl Pts',(56.7124614258119,5.92576148056642,-16.9995115321707));
#37256=CARTESIAN_POINT('Ctrl Pts',(56.6705073804071,6.19760185968837,-17.49547298161));
#37257=CARTESIAN_POINT('Ctrl Pts',(56.6457536157039,6.35282413332364,-17.8450721535257));
#37258=CARTESIAN_POINT('Ctrl Pts',(56.6361291491391,6.40947553960446,-18.0007085032136));
#37259=CARTESIAN_POINT('Ctrl Pts',(56.6298206485322,6.44444041539305,-18.1099263859984));
#37260=CARTESIAN_POINT('Ctrl Pts',(56.6238465273791,6.47373614314704,-18.2061673528554));
#37261=CARTESIAN_POINT('Ctrl Pts',(56.6127753835527,6.52318789052139,-18.3863934508124));
#37262=CARTESIAN_POINT('Ctrl Pts',(56.6011197707429,6.56743761917295,-18.5745295664154));
#37263=CARTESIAN_POINT('Ctrl Pts',(56.5895622316385,6.60461514285489,-18.7635135846173));
#37264=CARTESIAN_POINT('Ctrl Pts',(56.5822709951931,6.62557263625537,-18.8838298576913));
#37265=CARTESIAN_POINT('Ctrl Pts',(56.5764559941441,6.64085081833095,-18.9808893137307));
#37266=CARTESIAN_POINT('Ctrl Pts',(56.5706422249478,6.65522596905915,-19.0787275580226));
#37267=CARTESIAN_POINT('Ctrl Pts',(56.5546912627251,6.69105086626354,-19.3506474291268));
#37268=CARTESIAN_POINT('Ctrl Pts',(56.5290686917994,6.73030576444265,-19.8129382656079));
#37269=CARTESIAN_POINT('Ctrl Pts',(56.4869033379652,6.75686122587932,-20.6889248100617));
#37270=CARTESIAN_POINT('Ctrl Pts',(56.4439828569392,6.73207638738493,-21.8901143268291));
#37271=CARTESIAN_POINT('Ctrl Pts',(56.4207878995836,6.72020579063288,-22.9645713483529));
#37272=CARTESIAN_POINT('Ctrl Pts',(56.4083502797615,6.74481557433032,-23.6666501706463));
#37273=CARTESIAN_POINT('Ctrl Pts',(56.4043291434562,6.75174230324922,-23.8933215011308));
#37274=CARTESIAN_POINT('Ctrl Pts',(56.398492185458,6.76332242913761,-24.3786922422349));
#37275=CARTESIAN_POINT('Ctrl Pts',(56.393815893827,6.77508570849919,-25.2203653565117));
#37276=CARTESIAN_POINT('Ctrl Pts',(56.3990629133695,6.77425355762422,-26.4506819756972));
#37277=CARTESIAN_POINT('Ctrl Pts',(56.4127399329853,6.7597315130406,-27.9490222417778));
#37278=CARTESIAN_POINT('Ctrl Pts',(56.4185729457465,6.75181328125929,-28.9647360897816));
#37279=CARTESIAN_POINT('Ctrl Pts',(56.4185239529943,6.7508906297659,-29.5391863786918));
#37280=CARTESIAN_POINT('Ctrl Pts',(56.418485093439,6.75065094731659,-29.6630149700534));
#37281=CARTESIAN_POINT('Ctrl Pts',(56.4183300862443,6.7500433467653,-29.9129783838157));
#37282=CARTESIAN_POINT('Ctrl Pts',(56.4178646736266,6.74866256221038,-30.3496161755409));
#37283=CARTESIAN_POINT('Ctrl Pts',(56.416282878756,6.74477104644997,-31.224923737901));
#37284=CARTESIAN_POINT('Ctrl Pts',(56.4135778544298,6.7384067889161,-32.2268641469045));
#37285=CARTESIAN_POINT('Ctrl Pts',(56.4111284320163,6.73150120937088,-33.2301868337395));
#37286=CARTESIAN_POINT('Ctrl Pts',(56.4097169184839,6.72641635934727,-33.9829585725888));
#37287=CARTESIAN_POINT('Ctrl Pts',(56.4090485548286,6.7218060372717,-34.735601000675));
#37288=CARTESIAN_POINT('Ctrl Pts',(56.4092942227924,6.7193015658958,-35.2371596816712));
#37289=CARTESIAN_POINT('Ctrl Pts',(56.4098113412844,6.71772837300494,-35.6141701797015));
#37290=CARTESIAN_POINT('Ctrl Pts',(56.4102730457911,6.71669168677539,-35.8653728421837));
#37291=CARTESIAN_POINT('Ctrl Pts',(56.4116026068534,6.71465379461935,-36.3679915774757));
#37292=CARTESIAN_POINT('Ctrl Pts',(56.4148812401533,6.71123663261034,-37.2458884360711));
#37293=CARTESIAN_POINT('Ctrl Pts',(56.4240612418311,6.70516318867893,-38.9991861724131));
#37294=CARTESIAN_POINT('Ctrl Pts',(56.4327316323619,6.7020467448753,-40.5031852469808));
#37295=CARTESIAN_POINT('Ctrl Pts',(56.4358176766823,6.70148464569061,-41.6375067241571));
#37296=CARTESIAN_POINT('Ctrl Pts',(56.4363859507804,6.70120093233901,-41.8854524324178));
#37297=CARTESIAN_POINT('Ctrl Pts',(56.4369600134697,6.70040278697019,-42.2597348467726));
#37298=CARTESIAN_POINT('Ctrl Pts',(56.4373019861491,6.69934223132865,-42.6344724404243));
#37299=CARTESIAN_POINT('Ctrl Pts',(56.4375131769031,6.69772413167307,-43.1355563860534));
#37300=CARTESIAN_POINT('Ctrl Pts',(56.43743857815,6.69559543263226,-43.7638356220231));
#37301=CARTESIAN_POINT('Ctrl Pts',(56.4371890772263,6.69375779937644,-44.520576384667));
#37302=CARTESIAN_POINT('Ctrl Pts',(56.4371652256954,6.69356873094274,-45.1530289938705));
#37303=CARTESIAN_POINT('Ctrl Pts',(56.4374532086234,6.69467889993727,-45.6598650883663));
#37304=CARTESIAN_POINT('Ctrl Pts',(56.4378670016389,6.69625334352035,-46.0403702892188));
#37305=CARTESIAN_POINT('Ctrl Pts',(56.438526314343,6.69868310825844,-46.4211700949389));
#37306=CARTESIAN_POINT('Ctrl Pts',(56.4397997988323,6.70322061635112,-46.9292871803912));
#37307=CARTESIAN_POINT('Ctrl Pts',(56.441257007958,6.70824138694336,-47.3105245310882));
#37308=CARTESIAN_POINT('Ctrl Pts',(56.4431613354401,6.71460849120052,-47.6932076238684));
#37309=CARTESIAN_POINT('Ctrl Pts',(56.444461059475,6.72066563953415,-47.9626999638013));
#37310=CARTESIAN_POINT('Ctrl Pts',(56.4473157330693,6.73779781636137,-48.4883604358934));
#37311=CARTESIAN_POINT('Ctrl Pts',(56.4529620758537,6.77856952444017,-49.3987669008521));
#37312=CARTESIAN_POINT('Ctrl Pts',(56.463100633075,6.85159433777694,-50.6573233141209));
#37313=CARTESIAN_POINT('Ctrl Pts',(56.4786218386434,6.91724554550676,-52.1049716210228));
#37314=CARTESIAN_POINT('Ctrl Pts',(56.4907106899684,6.91939000975858,-53.0254174522498));
#37315=CARTESIAN_POINT('Ctrl Pts',(56.4985114506127,6.90058592503779,-53.5868928127147));
#37316=CARTESIAN_POINT('Ctrl Pts',(56.5016375151978,6.8901798231696,-53.7863301337798));
#37317=CARTESIAN_POINT('Ctrl Pts',(56.5085164008023,6.85469462748162,-54.2176593433617));
#37318=CARTESIAN_POINT('Ctrl Pts',(56.5222326673793,6.75852920726253,-55.0029169699139));
#37319=CARTESIAN_POINT('Ctrl Pts',(56.5557322438817,6.47228382886766,-56.7244744790596));
#37320=CARTESIAN_POINT('Ctrl Pts',(56.590501809989,6.22669399758466,-58.4359143044246));
#37321=CARTESIAN_POINT('Ctrl Pts',(56.5992930633333,6.30844846728972,-59.7694961384221));
#37322=CARTESIAN_POINT('Ctrl Pts',(56.6004541754483,6.3182623376236,-59.9110802125503));
#37323=CARTESIAN_POINT('Ctrl Pts',(56.602439888185,6.34240962308779,-60.204643689476));
#37324=CARTESIAN_POINT('Ctrl Pts',(56.6053447885661,6.39424928086466,-60.7100838593593));
#37325=CARTESIAN_POINT('Ctrl Pts',(56.6089205249707,6.53549360265129,-61.7144870525455));
#37326=CARTESIAN_POINT('Ctrl Pts',(56.6091551083785,6.771803729698,-62.8337353857643));
#37327=CARTESIAN_POINT('Ctrl Pts',(56.6076504370481,7.06395119048437,-63.9256406327616));
#37328=CARTESIAN_POINT('Ctrl Pts',(56.6065119391543,7.24589488847553,-64.5285845829376));
#37329=CARTESIAN_POINT('Ctrl Pts',(56.6057784652313,7.37315606264269,-64.9258734582198));
#37330=CARTESIAN_POINT('Ctrl Pts',(56.6053061446002,7.45949804394918,-65.1894282456331));
#37331=CARTESIAN_POINT('Ctrl Pts',(56.6048672956263,7.54799056003658,-65.451153705338));
#37332=CARTESIAN_POINT('Ctrl Pts',(56.60454321205,7.62703670738344,-65.6783915114089));
#37333=CARTESIAN_POINT('Ctrl Pts',(56.6043781250423,7.67263691564513,-65.807741257995));
#37334=CARTESIAN_POINT('Ctrl Pts',(56.6041508853138,7.74146255176413,-66.0012895834968));
#37335=CARTESIAN_POINT('Ctrl Pts',(56.6040117583367,7.79963582982472,-66.1615014626742));
#37336=CARTESIAN_POINT('Ctrl Pts',(56.6038316081065,7.89711952784231,-66.4259998336907));
#37337=CARTESIAN_POINT('Ctrl Pts',(56.6018530730065,8.0144401400366,-66.7303939337344));
#37338=CARTESIAN_POINT('Ctrl Pts',(56.5988000638691,8.25647394535926,-67.3071847283582));
#37339=CARTESIAN_POINT('Ctrl Pts',(56.5930354521079,8.71563413707656,-68.2955326482492));
#37340=CARTESIAN_POINT('Ctrl Pts',(56.5840964631355,9.71659621429294,-70.1535453043583));
#37341=CARTESIAN_POINT('Ctrl Pts',(56.5841638540735,10.5920784606575,-71.6137990424342));
#37342=CARTESIAN_POINT('Ctrl Pts',(56.5896072067733,11.1461190268922,-72.6661379485151));
#37343=CARTESIAN_POINT('Ctrl Pts',(56.5891309607652,11.2817778639891,-72.9238278802343));
#37344=CARTESIAN_POINT('Ctrl Pts',(56.5891672866806,11.5466066329308,-73.4254071841434));
#37345=CARTESIAN_POINT('Ctrl Pts',(56.588845595627,11.8811706681873,-74.0571574235573));
#37346=CARTESIAN_POINT('Ctrl Pts',(56.5887302787201,12.2818548355253,-74.8110572860588));
#37347=CARTESIAN_POINT('Ctrl Pts',(56.5884745468439,13.0849849212197,-76.3186335874071));
#37348=CARTESIAN_POINT('Ctrl Pts',(56.5885067406493,13.7543899062702,-77.5711825092658));
#37349=CARTESIAN_POINT('Ctrl Pts',(56.5887723366122,14.7223194411704,-79.3917286253267));
#37350=CARTESIAN_POINT('Ctrl Pts',(56.5886561011866,15.1596642818603,-80.2143906195593));
#37351=CARTESIAN_POINT('Ctrl Pts',(56.5886561011865,15.5961858692498,-81.0353683216575));
#37352=CARTESIAN_POINT('Ctrl Pts',(59.4327147758635,2.25264759904533,24.8301370357426));
#37353=CARTESIAN_POINT('Ctrl Pts',(59.4328805699872,2.25268328427295,24.7812421415735));
#37354=CARTESIAN_POINT('Ctrl Pts',(59.4330544581857,2.25272065661361,24.7323479892438));
#37355=CARTESIAN_POINT('Ctrl Pts',(59.4351081479366,2.25316352958089,24.1815581347574));
#37356=CARTESIAN_POINT('Ctrl Pts',(59.4365154515769,2.25375717421373,23.1771805010386));
#37357=CARTESIAN_POINT('Ctrl Pts',(59.4396802483187,2.25527681160943,21.168266890462));
#37358=CARTESIAN_POINT('Ctrl Pts',(59.4533544085439,2.25822384829969,19.664119974994));
#37359=CARTESIAN_POINT('Ctrl Pts',(59.4831900958584,2.26322002674582,18.4131232939436));
#37360=CARTESIAN_POINT('Ctrl Pts',(59.4973611339143,2.26566136680147,17.909530731663));
#37361=CARTESIAN_POINT('Ctrl Pts',(59.5326905890348,2.27186275277079,16.9049746402285));
#37362=CARTESIAN_POINT('Ctrl Pts',(59.6084537998042,2.28507927696242,15.1511100840618));
#37363=CARTESIAN_POINT('Ctrl Pts',(59.682155229076,2.29664260171308,13.6519166082037));
#37364=CARTESIAN_POINT('Ctrl Pts',(59.7316197253229,2.30214680015721,12.4008547144836));
#37365=CARTESIAN_POINT('Ctrl Pts',(59.7521786564858,2.30418787278943,11.9013037511421));
#37366=CARTESIAN_POINT('Ctrl Pts',(59.7951798385236,2.30767854931378,10.9015996797567));
#37367=CARTESIAN_POINT('Ctrl Pts',(59.871920487792,2.31235844347836,9.15030235439126));
#37368=CARTESIAN_POINT('Ctrl Pts',(59.9284261569215,2.31424867536969,7.64436614155757));
#37369=CARTESIAN_POINT('Ctrl Pts',(59.9544677432662,2.31510430612518,6.51125887373394));
#37370=CARTESIAN_POINT('Ctrl Pts',(59.9599887072642,2.31520084670204,6.26176258734173));
#37371=CARTESIAN_POINT('Ctrl Pts',(59.9701234406006,2.31513483587211,5.76118080724149));
#37372=CARTESIAN_POINT('Ctrl Pts',(59.9854549317823,2.31445343676422,4.88349131580663));
#37373=CARTESIAN_POINT('Ctrl Pts',(60.0066557259146,2.3116903349232,3.122050961627));
#37374=CARTESIAN_POINT('Ctrl Pts',(60.0081729114145,2.31041786813838,1.61015526670906));
#37375=CARTESIAN_POINT('Ctrl Pts',(60.0000133827516,2.31151798348453,0.547318300038715));
#37376=CARTESIAN_POINT('Ctrl Pts',(59.9987799969336,2.31117336970775,0.43263093270387));
#37377=CARTESIAN_POINT('Ctrl Pts',(59.9952905821698,2.30883587110844,0.194803767687823));
#37378=CARTESIAN_POINT('Ctrl Pts',(59.9867407237385,2.30078952656156,-0.221872168562404));
#37379=CARTESIAN_POINT('Ctrl Pts',(59.9687552635737,2.28042457466313,-0.830809221312308));
#37380=CARTESIAN_POINT('Ctrl Pts',(59.9419828448459,2.24998125672055,-1.58053884969406));
#37381=CARTESIAN_POINT('Ctrl Pts',(59.9045114164938,2.21332006777769,-2.60837725670198));
#37382=CARTESIAN_POINT('Ctrl Pts',(59.8638467657641,2.19824901379055,-3.94728156666758));
#37383=CARTESIAN_POINT('Ctrl Pts',(59.8547531658741,2.27161453180319,-5.07662983961258));
#37384=CARTESIAN_POINT('Ctrl Pts',(59.8612777254522,2.36142900914507,-5.79808115446848));
#37385=CARTESIAN_POINT('Ctrl Pts',(59.8667790865954,2.39532201728264,-6.05855832069619));
#37386=CARTESIAN_POINT('Ctrl Pts',(59.8857622841587,2.47308322652155,-6.59755779715002));
#37387=CARTESIAN_POINT('Ctrl Pts',(59.9369986063271,2.63002365791845,-7.53693807282327));
#37388=CARTESIAN_POINT('Ctrl Pts',(60.0379370888202,2.92928801589726,-8.89353364220382));
#37389=CARTESIAN_POINT('Ctrl Pts',(60.1099184078909,3.33173088950953,-10.2468366988312));
#37390=CARTESIAN_POINT('Ctrl Pts',(60.1185581245289,3.65744077076127,-11.1940983723255));
#37391=CARTESIAN_POINT('Ctrl Pts',(60.1089394250062,3.85489440144113,-11.7360559881447));
#37392=CARTESIAN_POINT('Ctrl Pts',(60.0988057825633,3.95716232528036,-12.0071578997948));
#37393=CARTESIAN_POINT('Ctrl Pts',(60.088867015177,4.03585186488094,-12.2124631115407));
#37394=CARTESIAN_POINT('Ctrl Pts',(60.0770799382493,4.10162443878164,-12.3804759509473));
#37395=CARTESIAN_POINT('Ctrl Pts',(60.0533423220747,4.23335080955239,-12.6916421900252));
#37396=CARTESIAN_POINT('Ctrl Pts',(60.0048222621594,4.48160461407792,-13.2286596866252));
#37397=CARTESIAN_POINT('Ctrl Pts',(59.8591649769858,5.17318220046663,-14.520766291152));
#37398=CARTESIAN_POINT('Ctrl Pts',(59.6737288778186,6.00238966144673,-15.7920829004921));
#37399=CARTESIAN_POINT('Ctrl Pts',(59.5263120296862,6.61088078796949,-16.8978546252372));
#37400=CARTESIAN_POINT('Ctrl Pts',(59.4651538261524,6.84135783860763,-17.3942967990539));
#37401=CARTESIAN_POINT('Ctrl Pts',(59.4267168765041,6.97398996864091,-17.749743920164));
#37402=CARTESIAN_POINT('Ctrl Pts',(59.4113161943744,7.02320296959488,-17.9115274404766));
#37403=CARTESIAN_POINT('Ctrl Pts',(59.4013852878992,7.05389951784351,-18.0266279574196));
#37404=CARTESIAN_POINT('Ctrl Pts',(59.3940826480698,7.07707674929802,-18.1188405616837));
#37405=CARTESIAN_POINT('Ctrl Pts',(59.3803725278826,7.11649992658285,-18.2961177733231));
#37406=CARTESIAN_POINT('Ctrl Pts',(59.3671207098108,7.15031966048852,-18.480276260381));
#37407=CARTESIAN_POINT('Ctrl Pts',(59.3546789178648,7.17768441585883,-18.6669679798643));
#37408=CARTESIAN_POINT('Ctrl Pts',(59.3471904049831,7.19249453279696,-18.7859681713174));
#37409=CARTESIAN_POINT('Ctrl Pts',(59.3414003725508,7.20291843621819,-18.8822443641514));
#37410=CARTESIAN_POINT('Ctrl Pts',(59.3357390090068,7.21244523533041,-18.9794037813503));
#37411=CARTESIAN_POINT('Ctrl Pts',(59.3207106649973,7.23499990532823,-19.2499932907629));
#37412=CARTESIAN_POINT('Ctrl Pts',(59.2992033293261,7.2525723692102,-19.7128140108013));
#37413=CARTESIAN_POINT('Ctrl Pts',(59.2695633569605,7.23976893671297,-20.595989007654));
#37414=CARTESIAN_POINT('Ctrl Pts',(59.2466259148726,7.16407388584051,-21.8137241348146));
#37415=CARTESIAN_POINT('Ctrl Pts',(59.2333573088729,7.11836760292419,-22.9079330706097));
#37416=CARTESIAN_POINT('Ctrl Pts',(59.2225729318419,7.12836870657141,-23.6256260071911));
#37417=CARTESIAN_POINT('Ctrl Pts',(59.218879188711,7.13116315677762,-23.8586364848611));
#37418=CARTESIAN_POINT('Ctrl Pts',(59.2130886994703,7.13583646035015,-24.3552912337382));
#37419=CARTESIAN_POINT('Ctrl Pts',(59.2069711153891,7.14052696112994,-25.213894792417));
#37420=CARTESIAN_POINT('Ctrl Pts',(59.2071940926013,7.13992372229919,-26.4598845391602));
#37421=CARTESIAN_POINT('Ctrl Pts',(59.2142118004288,7.13359020698822,-27.9631595869271));
#37422=CARTESIAN_POINT('Ctrl Pts',(59.2183316401815,7.13037250268532,-28.9727155137208));
#37423=CARTESIAN_POINT('Ctrl Pts',(59.2191463856912,7.13007778108586,-29.5412674506224));
#37424=CARTESIAN_POINT('Ctrl Pts',(59.2193436844314,7.1300024132007,-29.6660369532951));
#37425=CARTESIAN_POINT('Ctrl Pts',(59.2197848025345,7.12980927296514,-29.9165584568622));
#37426=CARTESIAN_POINT('Ctrl Pts',(59.2206776267452,7.129379567084,-30.3546893553598));
#37427=CARTESIAN_POINT('Ctrl Pts',(59.2229317471094,7.12818122773045,-31.2319841001822));
#37428=CARTESIAN_POINT('Ctrl Pts',(59.2264614389033,7.12633563783124,-32.2353584891699));
#37429=CARTESIAN_POINT('Ctrl Pts',(59.2307545410767,7.12444933988321,-33.2388608029659));
#37430=CARTESIAN_POINT('Ctrl Pts',(59.2343020974957,7.1231198708239,-33.9912364403544));
#37431=CARTESIAN_POINT('Ctrl Pts',(59.2381004226901,7.1220247993843,-34.7429205634483));
#37432=CARTESIAN_POINT('Ctrl Pts',(59.2407678765008,7.1215048376743,-35.2434588351024));
#37433=CARTESIAN_POINT('Ctrl Pts',(59.2428133314656,7.12121201221069,-35.6195715682491));
#37434=CARTESIAN_POINT('Ctrl Pts',(59.2442723839178,7.12101105794536,-35.8708228135));
#37435=CARTESIAN_POINT('Ctrl Pts',(59.2475011339763,7.12060361293872,-36.3731615660546));
#37436=CARTESIAN_POINT('Ctrl Pts',(59.2538137491707,7.11994127909612,-37.2507475076407));
#37437=CARTESIAN_POINT('Ctrl Pts',(59.2681942977094,7.11886970086017,-39.0032177529718));
#37438=CARTESIAN_POINT('Ctrl Pts',(59.2799886515837,7.11921953999885,-40.5065411340942));
#37439=CARTESIAN_POINT('Ctrl Pts',(59.2851996153717,7.12074410872078,-41.6403275585497));
#37440=CARTESIAN_POINT('Ctrl Pts',(59.2862494874205,7.12090603734663,-41.8882328760425));
#37441=CARTESIAN_POINT('Ctrl Pts',(59.2875421020988,7.12075925363304,-42.2623994447051));
#37442=CARTESIAN_POINT('Ctrl Pts',(59.2885945057288,7.12032313164209,-42.6370193484372));
#37443=CARTESIAN_POINT('Ctrl Pts',(59.2897262224044,7.11949943860257,-43.1379169156182));
#37444=CARTESIAN_POINT('Ctrl Pts',(59.2907301525556,7.11827942067128,-43.7659238140434));
#37445=CARTESIAN_POINT('Ctrl Pts',(59.2915831244807,7.11736409262801,-44.5222645555723));
#37446=CARTESIAN_POINT('Ctrl Pts',(59.2922548730296,7.11777499065889,-45.1543232707919));
#37447=CARTESIAN_POINT('Ctrl Pts',(59.292926826433,7.1192442939905,-45.6608028819353));
#37448=CARTESIAN_POINT('Ctrl Pts',(59.2935333732457,7.12102430836641,-46.0410215359872));
#37449=CARTESIAN_POINT('Ctrl Pts',(59.2942811015061,7.12359120049604,-46.4215152867929));
#37450=CARTESIAN_POINT('Ctrl Pts',(59.2955170927399,7.12821485543452,-46.929197281356));
#37451=CARTESIAN_POINT('Ctrl Pts',(59.2967687246829,7.13318361907883,-47.310081014493));
#37452=CARTESIAN_POINT('Ctrl Pts',(59.2983163931068,7.13941329099905,-47.69238596202));
#37453=CARTESIAN_POINT('Ctrl Pts',(59.2993206163489,7.14533248224309,-47.9615277700545));
#37454=CARTESIAN_POINT('Ctrl Pts',(59.301396120705,7.16205185116678,-48.4866123228665));
#37455=CARTESIAN_POINT('Ctrl Pts',(59.3052220622473,7.20177535478386,-49.3961426670782));
#37456=CARTESIAN_POINT('Ctrl Pts',(59.3117584695497,7.27260781155126,-50.6539242057696));
#37457=CARTESIAN_POINT('Ctrl Pts',(59.3220001282436,7.33517126435499,-52.1013146689092));
#37458=CARTESIAN_POINT('Ctrl Pts',(59.3304026861646,7.33526075828364,-53.0220323256413));
#37459=CARTESIAN_POINT('Ctrl Pts',(59.335943439786,7.31525779761466,-53.5837977277501));
#37460=CARTESIAN_POINT('Ctrl Pts',(59.3380744041258,7.30439822250382,-53.7829956038034));
#37461=CARTESIAN_POINT('Ctrl Pts',(59.3427825664043,7.26785423620579,-54.2141155699194));
#37462=CARTESIAN_POINT('Ctrl Pts',(59.352318123001,7.16956134865011,-54.9990500754213));
#37463=CARTESIAN_POINT('Ctrl Pts',(59.3767789545431,6.87830922953412,-56.7205007536377));
#37464=CARTESIAN_POINT('Ctrl Pts',(59.4048060029405,6.62818987442243,-58.4327422573043));
#37465=CARTESIAN_POINT('Ctrl Pts',(59.411130482769,6.70855050145335,-59.767853832079));
#37466=CARTESIAN_POINT('Ctrl Pts',(59.4120059030465,6.71822542519762,-59.9096031455069));
#37467=CARTESIAN_POINT('Ctrl Pts',(59.4134825887939,6.74213391775351,-60.2034888696665));
#37468=CARTESIAN_POINT('Ctrl Pts',(59.4156518251278,6.7936798491486,-60.7094410989841));
#37469=CARTESIAN_POINT('Ctrl Pts',(59.4183146497419,6.93474877284089,-61.7146766129639));
#37470=CARTESIAN_POINT('Ctrl Pts',(59.4184992485081,7.1715190036146,-62.8344221591378));
#37471=CARTESIAN_POINT('Ctrl Pts',(59.4173589498161,7.46427912981003,-63.9264212002982));
#37472=CARTESIAN_POINT('Ctrl Pts',(59.4164757584546,7.6465429618124,-64.5292803407694));
#37473=CARTESIAN_POINT('Ctrl Pts',(59.4158918488738,7.77397289223777,-64.9264596667921));
#37474=CARTESIAN_POINT('Ctrl Pts',(59.4155105646797,7.86041369573992,-65.1899275045537));
#37475=CARTESIAN_POINT('Ctrl Pts',(59.4151469227141,7.94898045296805,-65.451546102566));
#37476=CARTESIAN_POINT('Ctrl Pts',(59.4148663751997,8.02806526429127,-65.6786728946603));
#37477=CARTESIAN_POINT('Ctrl Pts',(59.4147189579701,8.0736791676609,-65.8079543090621));
#37478=CARTESIAN_POINT('Ctrl Pts',(59.4145103915492,8.14251666840732,-66.0013954283672));
#37479=CARTESIAN_POINT('Ctrl Pts',(59.4143701375348,8.20068035980342,-66.1615077310751));
#37480=CARTESIAN_POINT('Ctrl Pts',(59.4141584642359,8.29812025686491,-66.4258317734694));
#37481=CARTESIAN_POINT('Ctrl Pts',(59.4121076614625,8.41545533517109,-66.7302379496878));
#37482=CARTESIAN_POINT('Ctrl Pts',(59.4089539368078,8.65747797861771,-67.3069545825026));
#37483=CARTESIAN_POINT('Ctrl Pts',(59.4030514710827,9.11662614725699,-68.2952495881172));
#37484=CARTESIAN_POINT('Ctrl Pts',(59.3940392140636,10.1175425980928,-70.1531805878224));
#37485=CARTESIAN_POINT('Ctrl Pts',(59.3942963770557,10.9930399610668,-71.6134582690787));
#37486=CARTESIAN_POINT('Ctrl Pts',(59.3998653033869,11.5471474796941,-72.6658362501666));
#37487=CARTESIAN_POINT('Ctrl Pts',(59.3993829957394,11.6828034066944,-72.9235196368838));
#37488=CARTESIAN_POINT('Ctrl Pts',(59.3994250933298,11.9476351383384,-73.4250951811133));
#37489=CARTESIAN_POINT('Ctrl Pts',(59.3991008911446,12.2821967199485,-74.0568391088504));
#37490=CARTESIAN_POINT('Ctrl Pts',(59.3989841193555,12.6828780415212,-74.8107346122541));
#37491=CARTESIAN_POINT('Ctrl Pts',(59.3987200829908,13.4859987647365,-76.3183047595498));
#37492=CARTESIAN_POINT('Ctrl Pts',(59.3987454302011,14.1553957607975,-77.570859071339));
#37493=CARTESIAN_POINT('Ctrl Pts',(59.3990166195318,15.1233319175322,-79.3914167710635));
#37494=CARTESIAN_POINT('Ctrl Pts',(59.3988987558118,15.5606742957496,-80.2140763701825));
#37495=CARTESIAN_POINT('Ctrl Pts',(59.3988987558118,15.997195883139,-81.0350540722808));
#37496=CARTESIAN_POINT('Ctrl Pts',(62.2324107530731,2.65110775638153,24.8313041334545));
#37497=CARTESIAN_POINT('Ctrl Pts',(62.2325712481792,2.65111389896304,24.7824463733246));
#37498=CARTESIAN_POINT('Ctrl Pts',(62.2327396152326,2.6511203034555,24.7335900578008));
#37499=CARTESIAN_POINT('Ctrl Pts',(62.2347278245421,2.65119902107034,24.1832355424136));
#37500=CARTESIAN_POINT('Ctrl Pts',(62.2357081947501,2.65089165244121,23.1793104561523));
#37501=CARTESIAN_POINT('Ctrl Pts',(62.2376372653672,2.64989331869101,21.1712236096822));
#37502=CARTESIAN_POINT('Ctrl Pts',(62.2508916536482,2.65046341990255,19.6674110821095));
#37503=CARTESIAN_POINT('Ctrl Pts',(62.2817148825578,2.65350817891073,18.4166244925075));
#37504=CARTESIAN_POINT('Ctrl Pts',(62.2963483870087,2.65475016941358,17.9154921162311));
#37505=CARTESIAN_POINT('Ctrl Pts',(62.3328691172103,2.6574719171568,16.9126541421275));
#37506=CARTESIAN_POINT('Ctrl Pts',(62.4114002121739,2.6633388598978,15.1583819672954));
#37507=CARTESIAN_POINT('Ctrl Pts',(62.4886606605266,2.67186677246271,13.6513017842059));
#37508=CARTESIAN_POINT('Ctrl Pts',(62.5416548070192,2.68272815015991,12.3900241288783));
#37509=CARTESIAN_POINT('Ctrl Pts',(62.5639056817367,2.68778557754191,11.8862883820249));
#37510=CARTESIAN_POINT('Ctrl Pts',(62.6111306817512,2.70009765356894,10.8805255622894));
#37511=CARTESIAN_POINT('Ctrl Pts',(62.6965531064208,2.72558859986316,9.12351798064619));
#37512=CARTESIAN_POINT('Ctrl Pts',(62.759762075258,2.74792577759869,7.62112627372732));
#37513=CARTESIAN_POINT('Ctrl Pts',(62.7870471025404,2.75842639956328,6.4944158415301));
#37514=CARTESIAN_POINT('Ctrl Pts',(62.7926887078876,2.76085425419954,6.24239056560327));
#37515=CARTESIAN_POINT('Ctrl Pts',(62.8024671671064,2.7658357454544,5.73982521057602));
#37516=CARTESIAN_POINT('Ctrl Pts',(62.8158643319916,2.77467446058688,4.85939786465086));
#37517=CARTESIAN_POINT('Ctrl Pts',(62.8293418335807,2.79097470902073,3.10187281411723));
#37518=CARTESIAN_POINT('Ctrl Pts',(62.8245351274415,2.79542965430205,1.60675084670123));
#37519=CARTESIAN_POINT('Ctrl Pts',(62.8215962252372,2.79042733884296,0.562689137332636));
#37520=CARTESIAN_POINT('Ctrl Pts',(62.8210154022939,2.78909900073173,0.458689070067316));
#37521=CARTESIAN_POINT('Ctrl Pts',(62.8190965256766,2.78354103411644,0.235639881228226));
#37522=CARTESIAN_POINT('Ctrl Pts',(62.8139101492631,2.76682592587925,-0.156856461533343));
#37523=CARTESIAN_POINT('Ctrl Pts',(62.8023761501897,2.72650026401499,-0.744804542152578));
#37524=CARTESIAN_POINT('Ctrl Pts',(62.7849294582608,2.66393931300271,-1.48602674337414));
#37525=CARTESIAN_POINT('Ctrl Pts',(62.7601020876933,2.58128900315883,-2.52537635631036));
#37526=CARTESIAN_POINT('Ctrl Pts',(62.7319170070745,2.51604925639296,-3.91937869392183));
#37527=CARTESIAN_POINT('Ctrl Pts',(62.7291057998474,2.61099085146794,-5.14442267966518));
#37528=CARTESIAN_POINT('Ctrl Pts',(62.7362630542708,2.75759085859505,-5.93636508459741));
#37529=CARTESIAN_POINT('Ctrl Pts',(62.741770321279,2.82176513592095,-6.24514557083446));
#37530=CARTESIAN_POINT('Ctrl Pts',(62.7599115715833,2.97658271776053,-6.85273437634613));
#37531=CARTESIAN_POINT('Ctrl Pts',(62.8061174584549,3.30597913808947,-7.8806370854957));
#37532=CARTESIAN_POINT('Ctrl Pts',(62.8863958085257,3.89707212753794,-9.25228156988392));
#37533=CARTESIAN_POINT('Ctrl Pts',(62.9397736056384,4.52674995443731,-10.5119043306548));
#37534=CARTESIAN_POINT('Ctrl Pts',(62.9483073836637,4.92853685878937,-11.3479068954967));
#37535=CARTESIAN_POINT('Ctrl Pts',(62.9426225817136,5.13846212177897,-11.8136574168422));
#37536=CARTESIAN_POINT('Ctrl Pts',(62.935877313132,5.23527026475624,-12.0423083109252));
#37537=CARTESIAN_POINT('Ctrl Pts',(62.9289467471649,5.30491005784014,-12.2140196746635));
#37538=CARTESIAN_POINT('Ctrl Pts',(62.9178468592772,5.36388030319758,-12.36298456468));
#37539=CARTESIAN_POINT('Ctrl Pts',(62.8961604147852,5.47660367245371,-12.638969827769));
#37540=CARTESIAN_POINT('Ctrl Pts',(62.8501167546216,5.68011606065942,-13.1247631815501));
#37541=CARTESIAN_POINT('Ctrl Pts',(62.7055471700459,6.20985984960202,-14.3304179005817));
#37542=CARTESIAN_POINT('Ctrl Pts',(62.4912338497451,6.78245990414777,-15.5747418743489));
#37543=CARTESIAN_POINT('Ctrl Pts',(62.2993029893369,7.20735187064418,-16.6805280552391));
#37544=CARTESIAN_POINT('Ctrl Pts',(62.2163632975749,7.37607495476045,-17.1955964358133));
#37545=CARTESIAN_POINT('Ctrl Pts',(62.1634721816956,7.48085730828298,-17.5834240481002));
#37546=CARTESIAN_POINT('Ctrl Pts',(62.1425670082912,7.52293760023202,-17.7693118352408));
#37547=CARTESIAN_POINT('Ctrl Pts',(62.1294390175357,7.55035896134082,-17.9052542089931));
#37548=CARTESIAN_POINT('Ctrl Pts',(62.1211563672464,7.56761908025001,-17.998106111389));
#37549=CARTESIAN_POINT('Ctrl Pts',(62.1060386122447,7.59818832727529,-18.1847977995392));
#37550=CARTESIAN_POINT('Ctrl Pts',(62.0930891012341,7.62317609429139,-18.3759276979325));
#37551=CARTESIAN_POINT('Ctrl Pts',(62.0822144223327,7.6428536058607,-18.5711944201463));
#37552=CARTESIAN_POINT('Ctrl Pts',(62.0762525917653,7.65302519565803,-18.6951977645338));
#37553=CARTESIAN_POINT('Ctrl Pts',(62.0719662087674,7.65992486605567,-18.7955588852272));
#37554=CARTESIAN_POINT('Ctrl Pts',(62.0679951985242,7.66601390368074,-18.8967266479224));
#37555=CARTESIAN_POINT('Ctrl Pts',(62.0583389004949,7.67951185973049,-19.1781893365365));
#37556=CARTESIAN_POINT('Ctrl Pts',(62.0491579848126,7.6843381603447,-19.6572844659895));
#37557=CARTESIAN_POINT('Ctrl Pts',(62.0471164144703,7.6543263621362,-20.5627064856723));
#37558=CARTESIAN_POINT('Ctrl Pts',(62.0621269100584,7.56710224252032,-21.7946524647982));
#37559=CARTESIAN_POINT('Ctrl Pts',(62.0706822093106,7.51375182233016,-22.8859597117177));
#37560=CARTESIAN_POINT('Ctrl Pts',(62.0668999269535,7.51427019692833,-23.5975676711049));
#37561=CARTESIAN_POINT('Ctrl Pts',(62.0655820576767,7.51436969700696,-23.8360686960198));
#37562=CARTESIAN_POINT('Ctrl Pts',(62.0635918991896,7.51431755456326,-24.3384860432659));
#37563=CARTESIAN_POINT('Ctrl Pts',(62.0616150444944,7.51362663741968,-25.2077384672639));
#37564=CARTESIAN_POINT('Ctrl Pts',(62.0621011031445,7.5115907307205,-26.4627170410167));
#37565=CARTESIAN_POINT('Ctrl Pts',(62.0648413323574,7.50921458405261,-27.970321999584));
#37566=CARTESIAN_POINT('Ctrl Pts',(62.0659292167856,7.50884682134933,-28.977749244481));
#37567=CARTESIAN_POINT('Ctrl Pts',(62.0657024475546,7.5092866457995,-29.5438704056461));
#37568=CARTESIAN_POINT('Ctrl Pts',(62.0656416363747,7.50939383567201,-29.6694876250792));
#37569=CARTESIAN_POINT('Ctrl Pts',(62.065487129712,7.50965895993831,-29.9208561665864));
#37570=CARTESIAN_POINT('Ctrl Pts',(62.0651364468902,7.51024656387718,-30.3607234336883));
#37571=CARTESIAN_POINT('Ctrl Pts',(62.0641874801837,7.51185658664952,-31.2405845311435));
#37572=CARTESIAN_POINT('Ctrl Pts',(62.0628511063028,7.51444177549677,-32.2457033193181));
#37573=CARTESIAN_POINT('Ctrl Pts',(62.0619103176685,7.51726239035914,-33.2494543277796));
#37574=CARTESIAN_POINT('Ctrl Pts',(62.0615653654591,7.51937480913954,-34.001324586973));
#37575=CARTESIAN_POINT('Ctrl Pts',(62.0617406922815,7.52137880169214,-34.7518222937873));
#37576=CARTESIAN_POINT('Ctrl Pts',(62.0623142980273,7.52256208676719,-35.2510989017198));
#37577=CARTESIAN_POINT('Ctrl Pts',(62.0629588222116,7.52336429710618,-35.6261040174291));
#37578=CARTESIAN_POINT('Ctrl Pts',(62.063482259618,7.52388694043014,-35.8774098318808));
#37579=CARTESIAN_POINT('Ctrl Pts',(62.0648533349532,7.5248751427224,-36.379401153661));
#37580=CARTESIAN_POINT('Ctrl Pts',(62.0679875202739,7.5264987578139,-37.2566176006549));
#37581=CARTESIAN_POINT('Ctrl Pts',(62.0763297936556,7.52948981660232,-39.0081166132972));
#37582=CARTESIAN_POINT('Ctrl Pts',(62.0839656121537,7.53241511387234,-40.5106520379719));
#37583=CARTESIAN_POINT('Ctrl Pts',(62.0869051196726,7.53551992569335,-41.6437574713479));
#37584=CARTESIAN_POINT('Ctrl Pts',(62.0874696162204,7.53602680982341,-41.8915847922602));
#37585=CARTESIAN_POINT('Ctrl Pts',(62.0880919637729,7.53638204364662,-42.2655810687143));
#37586=CARTESIAN_POINT('Ctrl Pts',(62.0885286959401,7.53642856982292,-42.6400285125531));
#37587=CARTESIAN_POINT('Ctrl Pts',(62.0889117416412,7.536217481607,-43.1406690708058));
#37588=CARTESIAN_POINT('Ctrl Pts',(62.089110888396,7.53569612756946,-43.7683203882214));
#37589=CARTESIAN_POINT('Ctrl Pts',(62.0891971286507,7.53548224296686,-44.5241748107218));
#37590=CARTESIAN_POINT('Ctrl Pts',(62.0893868535754,7.53633812587254,-45.1557822312303));
#37591=CARTESIAN_POINT('Ctrl Pts',(62.0897605897562,7.53806579301751,-45.6618675530432));
#37592=CARTESIAN_POINT('Ctrl Pts',(62.090186372261,7.53998630844427,-46.0417760871001));
#37593=CARTESIAN_POINT('Ctrl Pts',(62.0907946046371,7.54263675345113,-46.4219447920921));
#37594=CARTESIAN_POINT('Ctrl Pts',(62.0918987822575,7.54728997860321,-46.9291720506793));
#37595=CARTESIAN_POINT('Ctrl Pts',(62.0931073870063,7.55218477568363,-47.3096935045049));
#37596=CARTESIAN_POINT('Ctrl Pts',(62.0946500272994,7.55826552660255,-47.6916137330119));
#37597=CARTESIAN_POINT('Ctrl Pts',(62.0956899306758,7.56404442827066,-47.9603806883333));
#37598=CARTESIAN_POINT('Ctrl Pts',(62.0979567486044,7.58036458850267,-48.4848483930344));
#37599=CARTESIAN_POINT('Ctrl Pts',(62.1023967485155,7.61910468697639,-49.3934153829413));
#37600=CARTESIAN_POINT('Ctrl Pts',(62.1103353217924,7.68794869441984,-50.6502655802821));
#37601=CARTESIAN_POINT('Ctrl Pts',(62.1224233583074,7.74777139027884,-52.0972078070305));
#37602=CARTESIAN_POINT('Ctrl Pts',(62.1317299659118,7.74613906151579,-53.0181400026945));
#37603=CARTESIAN_POINT('Ctrl Pts',(62.1376265100412,7.72516009843336,-53.5801983221761));
#37604=CARTESIAN_POINT('Ctrl Pts',(62.1399009906046,7.71395919386377,-53.7790356598082));
#37605=CARTESIAN_POINT('Ctrl Pts',(62.144891893323,7.67660866103408,-54.2098301643304));
#37606=CARTESIAN_POINT('Ctrl Pts',(62.1548861078054,7.57668998629144,-54.9943176964645));
#37607=CARTESIAN_POINT('Ctrl Pts',(62.1799950971101,7.28140426678334,-56.7158154644147));
#37608=CARTESIAN_POINT('Ctrl Pts',(62.2081833873139,7.02729986390898,-58.4291811313585));
#37609=CARTESIAN_POINT('Ctrl Pts',(62.214434191419,7.10645430029738,-59.7660691188329));
#37610=CARTESIAN_POINT('Ctrl Pts',(62.2152921603056,7.11601138045444,-59.9080078322041));
#37611=CARTESIAN_POINT('Ctrl Pts',(62.2167187516735,7.13971652526845,-60.2022648135528));
#37612=CARTESIAN_POINT('Ctrl Pts',(62.2187556195035,7.19101526209245,-60.7088079055096));
#37613=CARTESIAN_POINT('Ctrl Pts',(62.2210058151301,7.33194406379086,-61.7150167266094));
#37614=CARTESIAN_POINT('Ctrl Pts',(62.220494103909,7.56912255440908,-62.8353925702497));
#37615=CARTESIAN_POINT('Ctrl Pts',(62.2186541786765,7.86241183339184,-63.9275931935359));
#37616=CARTESIAN_POINT('Ctrl Pts',(62.21741273019,8.04494685543862,-64.5304140788372));
#37617=CARTESIAN_POINT('Ctrl Pts',(62.2166188453856,8.17251642994582,-64.9275069514343));
#37618=CARTESIAN_POINT('Ctrl Pts',(62.2161062636506,8.25903749032414,-65.1909009442395));
#37619=CARTESIAN_POINT('Ctrl Pts',(62.2156253772436,8.34766269691667,-65.4524219022825));
#37620=CARTESIAN_POINT('Ctrl Pts',(62.215257134898,8.42677423198685,-65.6794420084634));
#37621=CARTESIAN_POINT('Ctrl Pts',(62.2150641387944,8.47239575868788,-65.8086563808691));
#37622=CARTESIAN_POINT('Ctrl Pts',(62.2147919316114,8.54123677518438,-66.00199105567));
#37623=CARTESIAN_POINT('Ctrl Pts',(62.214608655405,8.59938592525983,-66.1620016010331));
#37624=CARTESIAN_POINT('Ctrl Pts',(62.2143413509797,8.69677672156467,-66.4261446314036));
#37625=CARTESIAN_POINT('Ctrl Pts',(62.2122609913914,8.81415479402535,-66.7305926507935));
#37626=CARTESIAN_POINT('Ctrl Pts',(62.2090683229704,9.0562048004226,-67.3072649369297));
#37627=CARTESIAN_POINT('Ctrl Pts',(62.2031701902083,9.51541638792159,-68.2955523830468));
#37628=CARTESIAN_POINT('Ctrl Pts',(62.1943317515038,10.5163927506456,-70.1534306834209));
#37629=CARTESIAN_POINT('Ctrl Pts',(62.1947391875034,11.3919020579306,-71.6137286933384));
#37630=CARTESIAN_POINT('Ctrl Pts',(62.2001943443147,11.9460014704505,-72.6661252618744));
#37631=CARTESIAN_POINT('Ctrl Pts',(62.1997185000816,12.0816602390721,-72.9238044443063));
#37632=CARTESIAN_POINT('Ctrl Pts',(62.1997564287731,12.3464935835405,-73.4253766509266));
#37633=CARTESIAN_POINT('Ctrl Pts',(62.1994358797236,12.6810568195398,-74.0571159606845));
#37634=CARTESIAN_POINT('Ctrl Pts',(62.1993211872213,13.0817369941327,-74.8110076497966));
#37635=CARTESIAN_POINT('Ctrl Pts',(62.1990653816072,13.8848530540247,-76.3185722749635));
#37636=CARTESIAN_POINT('Ctrl Pts',(62.19909669396,14.5542450034784,-77.5711307503444));
#37637=CARTESIAN_POINT('Ctrl Pts',(62.1993620993693,15.522185035061,-79.3916988003171));
#37638=CARTESIAN_POINT('Ctrl Pts',(62.1992463983474,15.9595269771664,-80.2143564816684));
#37639=CARTESIAN_POINT('Ctrl Pts',(62.1992463983475,16.3960485645559,-81.0353341837667));
#37640=CARTESIAN_POINT('Ctrl Pts',(65.0350887199224,3.04279907572872,24.8318421095528));
#37641=CARTESIAN_POINT('Ctrl Pts',(65.0353017889815,3.04279961695075,24.7830009397453));
#37642=CARTESIAN_POINT('Ctrl Pts',(65.0355252186173,3.04280017067125,24.7341613775858));
#37643=CARTESIAN_POINT('Ctrl Pts',(65.0381641497023,3.04280943774363,24.1840053062511));
#37644=CARTESIAN_POINT('Ctrl Pts',(65.0404998815081,3.04221679745299,23.1805170310154));
#37645=CARTESIAN_POINT('Ctrl Pts',(65.0461349316008,3.04039477281519,21.1726957556785));
#37646=CARTESIAN_POINT('Ctrl Pts',(65.0636872999614,3.04049794599169,19.6686880458142));
#37647=CARTESIAN_POINT('Ctrl Pts',(65.0993507487901,3.04372919187809,18.4175941768535));
#37648=CARTESIAN_POINT('Ctrl Pts',(65.1167602515594,3.0451355595967,17.9167397691228));
#37649=CARTESIAN_POINT('Ctrl Pts',(65.1610398139268,3.0484776471246,16.9142213017312));
#37650=CARTESIAN_POINT('Ctrl Pts',(65.2560876381536,3.05589826579763,15.1605998381288));
#37651=CARTESIAN_POINT('Ctrl Pts',(65.342626033825,3.06567363951754,13.6528125363831));
#37652=CARTESIAN_POINT('Ctrl Pts',(65.3898843591986,3.07637763944379,12.3899226094541));
#37653=CARTESIAN_POINT('Ctrl Pts',(65.4085180142653,3.08135168757766,11.8852522165172));
#37654=CARTESIAN_POINT('Ctrl Pts',(65.4441920740314,3.0933433491944,10.8780226376535));
#37655=CARTESIAN_POINT('Ctrl Pts',(65.5009220975331,3.11769180542614,9.11918017470684));
#37656=CARTESIAN_POINT('Ctrl Pts',(65.5344794590062,3.13759875586273,7.6178743897185));
#37657=CARTESIAN_POINT('Ctrl Pts',(65.5471867022137,3.14577990885582,6.49413363918257));
#37658=CARTESIAN_POINT('Ctrl Pts',(65.5490108295873,3.14719859434244,6.24591338779225));
#37659=CARTESIAN_POINT('Ctrl Pts',(65.5493695640765,3.14901745638244,5.74792996731733));
#37660=CARTESIAN_POINT('Ctrl Pts',(65.5427279547781,3.15004309780587,4.87350841866235));
#37661=CARTESIAN_POINT('Ctrl Pts',(65.5123377950902,3.14737548357901,3.11538246504764));
#37662=CARTESIAN_POINT('Ctrl Pts',(65.4950425644462,3.15244240092772,1.59718349180721));
#37663=CARTESIAN_POINT('Ctrl Pts',(65.5195985678633,3.16718619113657,0.529987804286143));
#37664=CARTESIAN_POINT('Ctrl Pts',(65.5229281006724,3.16804817025962,0.428403986222372));
#37665=CARTESIAN_POINT('Ctrl Pts',(65.5308547631716,3.16716048655649,0.206936702530311));
#37666=CARTESIAN_POINT('Ctrl Pts',(65.547966618142,3.15892053708572,-0.18214975514755));
#37667=CARTESIAN_POINT('Ctrl Pts',(65.5803545845031,3.13129166108476,-0.769062301553117));
#37668=CARTESIAN_POINT('Ctrl Pts',(65.6288087636496,3.08514444170353,-1.51529637587801));
#37669=CARTESIAN_POINT('Ctrl Pts',(65.700942704077,3.02972102648233,-2.57286733842955));
#37670=CARTESIAN_POINT('Ctrl Pts',(65.7958646181749,3.02141719199554,-4.01463727808764));
#37671=CARTESIAN_POINT('Ctrl Pts',(65.833958114971,3.21412823865908,-5.28558652813274));
#37672=CARTESIAN_POINT('Ctrl Pts',(65.8290085163487,3.43645951471753,-6.09719268068851));
#37673=CARTESIAN_POINT('Ctrl Pts',(65.8247241295313,3.54288014629557,-6.43980697173696));
#37674=CARTESIAN_POINT('Ctrl Pts',(65.8126064943145,3.78785542812985,-7.07974279986513));
#37675=CARTESIAN_POINT('Ctrl Pts',(65.7825329713037,4.28934782841537,-8.13424384932138));
#37676=CARTESIAN_POINT('Ctrl Pts',(65.7262757152049,5.10673810755621,-9.47955367822884));
#37677=CARTESIAN_POINT('Ctrl Pts',(65.6775989537901,5.87382979784091,-10.6881579950518));
#37678=CARTESIAN_POINT('Ctrl Pts',(65.6530739245746,6.29691093481057,-11.4492871912878));
#37679=CARTESIAN_POINT('Ctrl Pts',(65.6402509604291,6.49393833534442,-11.8545350240845));
#37680=CARTESIAN_POINT('Ctrl Pts',(65.6338047380311,6.5756459006392,-12.0455006429786));
#37681=CARTESIAN_POINT('Ctrl Pts',(65.6284680607276,6.63059158179909,-12.1853986619525));
#37682=CARTESIAN_POINT('Ctrl Pts',(65.6190373441314,6.67765228874231,-12.311998747581));
#37683=CARTESIAN_POINT('Ctrl Pts',(65.6011805048907,6.76260522595195,-12.5468430177704));
#37684=CARTESIAN_POINT('Ctrl Pts',(65.5631589210313,6.90664693731635,-12.9664952301201));
#37685=CARTESIAN_POINT('Ctrl Pts',(65.4439643271269,7.2355614364749,-14.034879865786));
#37686=CARTESIAN_POINT('Ctrl Pts',(65.2467846105436,7.50697175850343,-15.2036231533799));
#37687=CARTESIAN_POINT('Ctrl Pts',(65.0613357293355,7.72730564767796,-16.3447594771015));
#37688=CARTESIAN_POINT('Ctrl Pts',(64.9821707265439,7.82439690662045,-16.9129922839534));
#37689=CARTESIAN_POINT('Ctrl Pts',(64.9317938132122,7.89318054939857,-17.3665581781212));
#37690=CARTESIAN_POINT('Ctrl Pts',(64.9118997134959,7.92425307371857,-17.593609467152));
#37691=CARTESIAN_POINT('Ctrl Pts',(64.8993078170653,7.94604297832826,-17.7629114259997));
#37692=CARTESIAN_POINT('Ctrl Pts',(64.8917354443301,7.9577231709319,-17.862764794746));
#37693=CARTESIAN_POINT('Ctrl Pts',(64.8782668624603,7.97935239629412,-18.071834896486));
#37694=CARTESIAN_POINT('Ctrl Pts',(64.8675100284545,7.99635574954936,-18.2813015057794));
#37695=CARTESIAN_POINT('Ctrl Pts',(64.8591513260664,8.00965782593826,-18.4954392521802));
#37696=CARTESIAN_POINT('Ctrl Pts',(64.8548934131429,8.01635413238409,-18.6303138116814));
#37697=CARTESIAN_POINT('Ctrl Pts',(64.8520291464493,8.02082955198509,-18.7391604425263));
#37698=CARTESIAN_POINT('Ctrl Pts',(64.8495178118383,8.02471289520919,-18.8485275415764));
#37699=CARTESIAN_POINT('Ctrl Pts',(64.8440168783019,8.03305322470471,-19.151562519944));
#37700=CARTESIAN_POINT('Ctrl Pts',(64.8422051716334,8.03446836901049,-19.6600026041905));
#37701=CARTESIAN_POINT('Ctrl Pts',(64.8535522086806,8.01105171857207,-20.5996300476593));
#37702=CARTESIAN_POINT('Ctrl Pts',(64.8837721490584,7.95109059523506,-21.8412831543704));
#37703=CARTESIAN_POINT('Ctrl Pts',(64.9003529795289,7.91660579442229,-22.9055204389761));
#37704=CARTESIAN_POINT('Ctrl Pts',(64.900277402366,7.91617325660034,-23.5899675786111));
#37705=CARTESIAN_POINT('Ctrl Pts',(64.9003030466406,7.91601809697143,-23.8329269136991));
#37706=CARTESIAN_POINT('Ctrl Pts',(64.9005401853198,7.91574867606951,-24.3354244521531));
#37707=CARTESIAN_POINT('Ctrl Pts',(64.9013716578895,7.91538329393073,-25.2086195369282));
#37708=CARTESIAN_POINT('Ctrl Pts',(64.9032688859418,7.91511031742878,-26.4649259761897));
#37709=CARTESIAN_POINT('Ctrl Pts',(64.9051772354161,7.91503595164712,-27.9727274470494));
#37710=CARTESIAN_POINT('Ctrl Pts',(64.9052137834096,7.91514938428072,-28.9779253703462));
#37711=CARTESIAN_POINT('Ctrl Pts',(64.9046311313933,7.91523345071605,-29.5423469924773));
#37712=CARTESIAN_POINT('Ctrl Pts',(64.9044796832551,7.91525415166103,-29.6678552241075));
#37713=CARTESIAN_POINT('Ctrl Pts',(64.9040899436161,7.91530319787013,-29.918872357726));
#37714=CARTESIAN_POINT('Ctrl Pts',(64.9031960134775,7.915411596412,-30.3582566268718));
#37715=CARTESIAN_POINT('Ctrl Pts',(64.9006918760774,7.91570657713133,-31.2372869259982));
#37716=CARTESIAN_POINT('Ctrl Pts',(64.89677233778,7.91620876660362,-32.2419466203269));
#37717=CARTESIAN_POINT('Ctrl Pts',(64.8929724427649,7.9168128149532,-33.2456438209988));
#37718=CARTESIAN_POINT('Ctrl Pts',(64.8904741843251,7.91729973895228,-33.99768199076));
#37719=CARTESIAN_POINT('Ctrl Pts',(64.8886108925044,7.91781497916351,-34.7485909478118));
#37720=CARTESIAN_POINT('Ctrl Pts',(64.8879880285033,7.91816196656921,-35.2482953845696));
#37721=CARTESIAN_POINT('Ctrl Pts',(64.8878265442141,7.9184188811029,-35.6236680650367));
#37722=CARTESIAN_POINT('Ctrl Pts',(64.8878043645194,7.9185774585649,-35.8749590326448));
#37723=CARTESIAN_POINT('Ctrl Pts',(64.8880697266912,7.91885465191016,-36.377066978034));
#37724=CARTESIAN_POINT('Ctrl Pts',(64.8892403338603,7.91926838647898,-37.2544411099771));
#37725=CARTESIAN_POINT('Ctrl Pts',(64.8936821150121,7.92003795010626,-39.0063008097556));
#37726=CARTESIAN_POINT('Ctrl Pts',(64.8984206741914,7.92142088740016,-40.5092037903869));
#37727=CARTESIAN_POINT('Ctrl Pts',(64.8998416479655,7.92364914218204,-41.6425587006194));
#37728=CARTESIAN_POINT('Ctrl Pts',(64.900086735534,7.92397092305037,-41.8904039225992));
#37729=CARTESIAN_POINT('Ctrl Pts',(64.9002731327335,7.92406146234017,-42.2644517559109));
#37730=CARTESIAN_POINT('Ctrl Pts',(64.9003142004051,7.92385916136743,-42.6389503791446));
#37731=CARTESIAN_POINT('Ctrl Pts',(64.9002194850142,7.92333674755533,-43.139672374497));
#37732=CARTESIAN_POINT('Ctrl Pts',(64.8999069802989,7.92246723541446,-43.7674412347485));
#37733=CARTESIAN_POINT('Ctrl Pts',(64.8994925944636,7.92190539145051,-44.5234677640342));
#37734=CARTESIAN_POINT('Ctrl Pts',(64.899339922121,7.92253352259311,-45.155245631552));
#37735=CARTESIAN_POINT('Ctrl Pts',(64.8994703796176,7.92412104846715,-45.661477068022));
#37736=CARTESIAN_POINT('Ctrl Pts',(64.8997271906668,7.92595720904262,-46.0415036119417));
#37737=CARTESIAN_POINT('Ctrl Pts',(64.900176872622,7.92854497560912,-46.4217982374827));
#37738=CARTESIAN_POINT('Ctrl Pts',(64.9010781824461,7.93314457097787,-46.9292021071505));
#37739=CARTESIAN_POINT('Ctrl Pts',(64.9021442437456,7.93803373319031,-47.3098718598978));
#37740=CARTESIAN_POINT('Ctrl Pts',(64.9035395227039,7.94413377331177,-47.6919455868718));
#37741=CARTESIAN_POINT('Ctrl Pts',(64.9044953458893,7.94994285497855,-47.9608592494408));
#37742=CARTESIAN_POINT('Ctrl Pts',(64.9066406887799,7.96637203100846,-48.4855644513516));
#37743=CARTESIAN_POINT('Ctrl Pts',(64.9109756826221,8.0054171998626,-49.3944919298558));
#37744=CARTESIAN_POINT('Ctrl Pts',(64.9189764880102,8.07493592398898,-50.6516573118312));
#37745=CARTESIAN_POINT('Ctrl Pts',(64.9311717897488,8.13568908426217,-52.0986939738742));
#37746=CARTESIAN_POINT('Ctrl Pts',(64.9403930891791,8.13463902398254,-53.0195112352081));
#37747=CARTESIAN_POINT('Ctrl Pts',(64.9461217879297,8.11397309546367,-53.5814465389996));
#37748=CARTESIAN_POINT('Ctrl Pts',(64.9483334556686,8.10288366697726,-53.7803766739668));
#37749=CARTESIAN_POINT('Ctrl Pts',(64.9531665353562,8.06579808845442,-54.2112509890253));
#37750=CARTESIAN_POINT('Ctrl Pts',(64.9628117033353,7.96641817521339,-54.9958646771246));
#37751=CARTESIAN_POINT('Ctrl Pts',(64.9868737195004,7.6724124170175,-56.7174073592783));
#37752=CARTESIAN_POINT('Ctrl Pts',(65.013938987719,7.4195820506246,-58.4304576933914));
#37753=CARTESIAN_POINT('Ctrl Pts',(65.0196793288631,7.49908996597736,-59.7667411537284));
#37754=CARTESIAN_POINT('Ctrl Pts',(65.020474205641,7.50867707433676,-59.9086143602503));
#37755=CARTESIAN_POINT('Ctrl Pts',(65.0217742074001,7.53243121116188,-60.2027437125628));
#37756=CARTESIAN_POINT('Ctrl Pts',(65.0235878298676,7.58377523464587,-60.7090835159779));
#37757=CARTESIAN_POINT('Ctrl Pts',(65.0253881213518,7.72466418199519,-61.7149614631889));
#37758=CARTESIAN_POINT('Ctrl Pts',(65.0243773613579,7.9615923705701,-62.8351390984063));
#37759=CARTESIAN_POINT('Ctrl Pts',(65.0220949239444,8.25460244180564,-63.9273035771588));
#37760=CARTESIAN_POINT('Ctrl Pts',(65.0206320327183,8.43699654685904,-64.5301596479062));
#37761=CARTESIAN_POINT('Ctrl Pts',(65.0197044168754,8.56449069371539,-64.9272970447687));
#37762=CARTESIAN_POINT('Ctrl Pts',(65.0191063773078,8.6509669508869,-65.1907263261488));
#37763=CARTESIAN_POINT('Ctrl Pts',(65.0185462704627,8.73955686405517,-65.4522904566082));
#37764=CARTESIAN_POINT('Ctrl Pts',(65.0181139983008,8.81864751039845,-65.6793553095181));
#37765=CARTESIAN_POINT('Ctrl Pts',(65.0178860252226,8.86426023414526,-65.8085971865833));
#37766=CARTESIAN_POINT('Ctrl Pts',(65.0175629808496,8.93309127293903,-66.0019749788851));
#37767=CARTESIAN_POINT('Ctrl Pts',(65.0173408944881,8.99123922852743,-66.1620255738922));
#37768=CARTESIAN_POINT('Ctrl Pts',(65.0170143927561,9.08863824119291,-66.4262385596083));
#37769=CARTESIAN_POINT('Ctrl Pts',(65.0149031169624,9.20600366322717,-66.7306827345292));
#37770=CARTESIAN_POINT('Ctrl Pts',(65.0116617417207,9.44804792453631,-67.3073858132993));
#37771=CARTESIAN_POINT('Ctrl Pts',(65.0057438245385,9.90725669751229,-68.2956962623178));
#37772=CARTESIAN_POINT('Ctrl Pts',(64.9970188351687,10.9082654800716,-70.1536086093708));
#37773=CARTESIAN_POINT('Ctrl Pts',(64.9975705399216,11.7837966760876,-71.6138987652382));
#37774=CARTESIAN_POINT('Ctrl Pts',(65.0029598100462,12.3378648994254,-72.6662797523441));
#37775=CARTESIAN_POINT('Ctrl Pts',(65.002487371209,12.4735251591182,-72.9239616170365));
#37776=CARTESIAN_POINT('Ctrl Pts',(65.0025224625631,12.7383572372994,-73.4255353796307));
#37777=CARTESIAN_POINT('Ctrl Pts',(65.0022038072545,13.0729215944058,-74.057277410925));
#37778=CARTESIAN_POINT('Ctrl Pts',(65.0020901349283,13.4736029531655,-74.8111709208594));
#37779=CARTESIAN_POINT('Ctrl Pts',(65.0018390996726,14.2767229057767,-76.3187381401072));
#37780=CARTESIAN_POINT('Ctrl Pts',(65.001875261823,14.9461178731812,-77.5712949614773));
#37781=CARTESIAN_POINT('Ctrl Pts',(65.0021384204276,15.9140549467347,-79.3918586961565));
#37782=CARTESIAN_POINT('Ctrl Pts',(65.002024063166,16.3513978914706,-80.2145175100176));
#37783=CARTESIAN_POINT('Ctrl Pts',(65.002024063166,16.7879194788601,-81.035495212116));
#37784=CARTESIAN_POINT('Ctrl Pts',(67.8429974293793,3.43540891085927,24.8291469487336));
#37785=CARTESIAN_POINT('Ctrl Pts',(67.8432546799249,3.43547993540378,24.7802220571657));
#37786=CARTESIAN_POINT('Ctrl Pts',(67.8435244457074,3.43555420488368,24.7312971430194));
#37787=CARTESIAN_POINT('Ctrl Pts',(67.8467070822611,3.43643846206893,24.1801612308648));
#37788=CARTESIAN_POINT('Ctrl Pts',(67.850423105421,3.4379671540823,23.1756927981266));
#37789=CARTESIAN_POINT('Ctrl Pts',(67.8599412644937,3.44198240237162,21.1660007123087));
#37790=CARTESIAN_POINT('Ctrl Pts',(67.8810365616718,3.44791094163207,19.6612635405338));
#37791=CARTESIAN_POINT('Ctrl Pts',(67.9194095919738,3.45624901551685,18.409658962508));
#37792=CARTESIAN_POINT('Ctrl Pts',(67.9382116424961,3.4607672753705,17.9030503904782));
#37793=CARTESIAN_POINT('Ctrl Pts',(67.9860593898693,3.47303081770967,16.8965427733973));
#37794=CARTESIAN_POINT('Ctrl Pts',(68.0882530593835,3.4993540656767,15.1438909478789));
#37795=CARTESIAN_POINT('Ctrl Pts',(68.1787020133392,3.51729805224381,13.654927397164));
#37796=CARTESIAN_POINT('Ctrl Pts',(68.2236660773134,3.51554802305279,12.4161247663745));
#37797=CARTESIAN_POINT('Ctrl Pts',(68.2402940648383,3.51324781151146,11.9218520300229));
#37798=CARTESIAN_POINT('Ctrl Pts',(68.2689151422823,3.50367772430015,10.9290931776768));
#37799=CARTESIAN_POINT('Ctrl Pts',(68.3084504452622,3.47762893596726,9.1831112953065));
#37800=CARTESIAN_POINT('Ctrl Pts',(68.330124390067,3.4515286669216,7.67044414590866));
#37801=CARTESIAN_POINT('Ctrl Pts',(68.3456639197554,3.44053297281301,6.52969946796556));
#37802=CARTESIAN_POINT('Ctrl Pts',(68.3481632218097,3.43698454189682,6.29585970801378));
#37803=CARTESIAN_POINT('Ctrl Pts',(68.3499188822826,3.42562590693248,5.8110691096698));
#37804=CARTESIAN_POINT('Ctrl Pts',(68.3461702772678,3.39691663158025,4.95317353448009));
#37805=CARTESIAN_POINT('Ctrl Pts',(68.3238717322638,3.32643314269278,3.17678659116776));
#37806=CARTESIAN_POINT('Ctrl Pts',(68.3243578395531,3.30825769820171,1.56727520685246));
#37807=CARTESIAN_POINT('Ctrl Pts',(68.3814824067012,3.39780401006464,0.387492102800521));
#37808=CARTESIAN_POINT('Ctrl Pts',(68.389250840906,3.40656484668491,0.26586218911445));
#37809=CARTESIAN_POINT('Ctrl Pts',(68.4077484859294,3.42556880479836,0.0101695747041382));
#37810=CARTESIAN_POINT('Ctrl Pts',(68.4474826307831,3.46000134869164,-0.435804959134103));
#37811=CARTESIAN_POINT('Ctrl Pts',(68.5214044436428,3.51863205261851,-1.08807597925497));
#37812=CARTESIAN_POINT('Ctrl Pts',(68.624423997359,3.6148516485158,-1.88624930375177));
#37813=CARTESIAN_POINT('Ctrl Pts',(68.7620990810596,3.78900640467524,-2.97208615448307));
#37814=CARTESIAN_POINT('Ctrl Pts',(68.8980905600522,4.10565556291278,-4.35854980325192));
#37815=CARTESIAN_POINT('Ctrl Pts',(68.9128946603297,4.46292612828363,-5.48743278551075));
#37816=CARTESIAN_POINT('Ctrl Pts',(68.8835321215552,4.7191174855521,-6.20457561297709));
#37817=CARTESIAN_POINT('Ctrl Pts',(68.8610375207658,4.84466562132032,-6.53581971169089));
#37818=CARTESIAN_POINT('Ctrl Pts',(68.8102656905332,5.11135281124297,-7.1438921545796));
#37819=CARTESIAN_POINT('Ctrl Pts',(68.7008946900405,5.63082823153305,-8.16490344646017));
#37820=CARTESIAN_POINT('Ctrl Pts',(68.5263288525118,6.43604086948472,-9.48848256415375));
#37821=CARTESIAN_POINT('Ctrl Pts',(68.3742468746776,7.15026545438326,-10.683440426365));
#37822=CARTESIAN_POINT('Ctrl Pts',(68.2960339802855,7.50953919485437,-11.4168810335362));
#37823=CARTESIAN_POINT('Ctrl Pts',(68.2603517774568,7.66556351915815,-11.7970269947054));
#37824=CARTESIAN_POINT('Ctrl Pts',(68.2455245078802,7.72624147090396,-11.9718237923998));
#37825=CARTESIAN_POINT('Ctrl Pts',(68.2353382633363,7.76560838945387,-12.0977864186943));
#37826=CARTESIAN_POINT('Ctrl Pts',(68.2257645812627,7.79765679592859,-12.2057340926592));
#37827=CARTESIAN_POINT('Ctrl Pts',(68.2071433316097,7.85343174661,-12.4091862488));
#37828=CARTESIAN_POINT('Ctrl Pts',(68.1716312700611,7.94179601760658,-12.7737396653198));
#37829=CARTESIAN_POINT('Ctrl Pts',(68.070486285267,8.11552251078656,-13.7174857085627));
#37830=CARTESIAN_POINT('Ctrl Pts',(67.9379271384842,8.19411424588751,-14.8288877330147));
#37831=CARTESIAN_POINT('Ctrl Pts',(67.8270359888485,8.24471186271882,-16.0333728136624));
#37832=CARTESIAN_POINT('Ctrl Pts',(67.7795558283908,8.2697989416524,-16.6593623509797));
#37833=CARTESIAN_POINT('Ctrl Pts',(67.7480027142475,8.29425523150742,-17.1744641828378));
#37834=CARTESIAN_POINT('Ctrl Pts',(67.7345704814989,8.30877875862203,-17.4370146473669));
#37835=CARTESIAN_POINT('Ctrl Pts',(67.7255160094835,8.3207465314588,-17.6343120719918));
#37836=CARTESIAN_POINT('Ctrl Pts',(67.7200766017121,8.32681894664132,-17.7435082074001));
#37837=CARTESIAN_POINT('Ctrl Pts',(67.7104052476175,8.33825756147983,-17.9755239104982));
#37838=CARTESIAN_POINT('Ctrl Pts',(67.702668557414,8.34716469625958,-18.2044901227104));
#37839=CARTESIAN_POINT('Ctrl Pts',(67.6966250109244,8.35418836361364,-18.437558078899));
#37840=CARTESIAN_POINT('Ctrl Pts',(67.6935261925001,8.35773483471823,-18.5833576386051));
#37841=CARTESIAN_POINT('Ctrl Pts',(67.6914266176471,8.36012556721365,-18.700617985052));
#37842=CARTESIAN_POINT('Ctrl Pts',(67.6895735618216,8.36221490888489,-18.8180965572433));
#37843=CARTESIAN_POINT('Ctrl Pts',(67.6854569006598,8.36677787513441,-19.1423230547089));
#37844=CARTESIAN_POINT('Ctrl Pts',(67.683716101415,8.36815072888433,-19.6791104208062));
#37845=CARTESIAN_POINT('Ctrl Pts',(67.6906761505665,8.35815154914856,-20.6510943341447));
#37846=CARTESIAN_POINT('Ctrl Pts',(67.7103986169785,8.33193530589776,-21.8996246348123));
#37847=CARTESIAN_POINT('Ctrl Pts',(67.7210587015029,8.31777296136097,-22.9339488548299));
#37848=CARTESIAN_POINT('Ctrl Pts',(67.7207969392067,8.3181111672581,-23.5892647051119));
#37849=CARTESIAN_POINT('Ctrl Pts',(67.7207306160019,8.31824392125545,-23.8355536683885));
#37850=CARTESIAN_POINT('Ctrl Pts',(67.7207252873965,8.31853514921489,-24.3362841907622));
#37851=CARTESIAN_POINT('Ctrl Pts',(67.7210028303336,8.31908037425217,-25.2105431345649));
#37852=CARTESIAN_POINT('Ctrl Pts',(67.7219597458375,8.31988698628591,-26.4655163566117));
#37853=CARTESIAN_POINT('Ctrl Pts',(67.7232034214329,8.3205421062546,-27.9726789655983));
#37854=CARTESIAN_POINT('Ctrl Pts',(67.7235294458012,8.32054619474664,-28.9767651545849));
#37855=CARTESIAN_POINT('Ctrl Pts',(67.7234122675956,8.32035226803725,-29.5405232802499));
#37856=CARTESIAN_POINT('Ctrl Pts',(67.7233746171398,8.32030086018687,-29.665766997083));
#37857=CARTESIAN_POINT('Ctrl Pts',(67.7232565399633,8.32017038515015,-29.9163489293805));
#37858=CARTESIAN_POINT('Ctrl Pts',(67.7229457623811,8.3198743612853,-30.3550172917412));
#37859=CARTESIAN_POINT('Ctrl Pts',(67.721980878253,8.31904185460349,-31.2329279534054));
#37860=CARTESIAN_POINT('Ctrl Pts',(67.7204180440811,8.31770949448862,-32.236944381495));
#37861=CARTESIAN_POINT('Ctrl Pts',(67.7190520692494,8.31630697009927,-33.240595565807));
#37862=CARTESIAN_POINT('Ctrl Pts',(67.7182903018882,8.31530078369864,-33.9928807647374));
#37863=CARTESIAN_POINT('Ctrl Pts',(67.7179528068233,8.31443177002382,-34.7443577769532));
#37864=CARTESIAN_POINT('Ctrl Pts',(67.7181208176444,8.31399598397217,-35.2446452982413));
#37865=CARTESIAN_POINT('Ctrl Pts',(67.7184362791062,8.3137414196746,-35.6205207851054));
#37866=CARTESIAN_POINT('Ctrl Pts',(67.7187154377707,8.31356151267366,-35.8717925217382));
#37867=CARTESIAN_POINT('Ctrl Pts',(67.7195144026143,8.31317245546242,-36.3740602203172));
#37868=CARTESIAN_POINT('Ctrl Pts',(67.7214612042378,8.31246119216897,-37.2516305553014));
#37869=CARTESIAN_POINT('Ctrl Pts',(67.7269127321384,8.31113260339281,-39.0039479458648));
#37870=CARTESIAN_POINT('Ctrl Pts',(67.7320337192982,8.31109429173692,-40.507281071242));
#37871=CARTESIAN_POINT('Ctrl Pts',(67.733889374357,8.31249478383146,-41.6409678438519));
#37872=CARTESIAN_POINT('Ctrl Pts',(67.7342365493349,8.31263805274339,-41.8888468551525));
#37873=CARTESIAN_POINT('Ctrl Pts',(67.7345947148907,8.31247397045901,-42.2629720819454));
#37874=CARTESIAN_POINT('Ctrl Pts',(67.7348187479955,8.31203100483415,-42.6375477798209));
#37875=CARTESIAN_POINT('Ctrl Pts',(67.7349753077395,8.31120760165609,-43.1383858366007));
#37876=CARTESIAN_POINT('Ctrl Pts',(67.7349742950132,8.31000056685548,-43.7663153738706));
#37877=CARTESIAN_POINT('Ctrl Pts',(67.7348795055068,8.3091021318316,-44.5225634357967));
#37878=CARTESIAN_POINT('Ctrl Pts',(67.7349061582348,8.30951233118236,-45.1545493559836));
#37879=CARTESIAN_POINT('Ctrl Pts',(67.7351015739539,8.31096392461986,-45.6609591786128));
#37880=CARTESIAN_POINT('Ctrl Pts',(67.735362038661,8.31271925403025,-46.0411268459948));
#37881=CARTESIAN_POINT('Ctrl Pts',(67.7357638526901,8.31524787949285,-46.4215697992487));
#37882=CARTESIAN_POINT('Ctrl Pts',(67.7365243631353,8.31979852684157,-46.9291808229217));
#37883=CARTESIAN_POINT('Ctrl Pts',(67.737388241482,8.32468631346973,-47.3100182253739));
#37884=CARTESIAN_POINT('Ctrl Pts',(67.7385041109757,8.33080992955567,-47.6922682683125));
#37885=CARTESIAN_POINT('Ctrl Pts',(67.739248602412,8.33665209329345,-47.9613502341259));
#37886=CARTESIAN_POINT('Ctrl Pts',(67.7408867984485,8.35319737208983,-48.4863342036919));
#37887=CARTESIAN_POINT('Ctrl Pts',(67.7441288417548,8.39256514828176,-49.3956985438844));
#37888=CARTESIAN_POINT('Ctrl Pts',(67.7500732418108,8.46277674166923,-50.6532915323841));
#37889=CARTESIAN_POINT('Ctrl Pts',(67.7593067036381,8.52446860885247,-52.1005370157973));
#37890=CARTESIAN_POINT('Ctrl Pts',(67.7663929158143,8.52396027275911,-53.0212614429966));
#37891=CARTESIAN_POINT('Ctrl Pts',(67.7707931388197,8.50357810494722,-53.5830672845635));
#37892=CARTESIAN_POINT('Ctrl Pts',(67.7724365295146,8.4925742604724,-53.7821583853968));
#37893=CARTESIAN_POINT('Ctrl Pts',(67.7760235766481,8.45570310541286,-54.2131780875111));
#37894=CARTESIAN_POINT('Ctrl Pts',(67.7832529202123,8.35676358196918,-54.9979917213648));
#37895=CARTESIAN_POINT('Ctrl Pts',(67.8019920467125,8.06391172112489,-56.7195171344691));
#37896=CARTESIAN_POINT('Ctrl Pts',(67.8248577335212,7.81231208452433,-58.4320647827162));
#37897=CARTESIAN_POINT('Ctrl Pts',(67.8290183714227,7.89213801775489,-59.7675459959514));
#37898=CARTESIAN_POINT('Ctrl Pts',(67.8296331107842,7.9017520647363,-59.9093334780841));
#37899=CARTESIAN_POINT('Ctrl Pts',(67.8306053782331,7.92554871689266,-60.2032949580968));
#37900=CARTESIAN_POINT('Ctrl Pts',(67.8319311069114,7.97692662403817,-60.7093677144899));
#37901=CARTESIAN_POINT('Ctrl Pts',(67.8330622134766,8.11775522230267,-61.7148065060258));
#37902=CARTESIAN_POINT('Ctrl Pts',(67.8318330009838,8.35441804035953,-62.8347017929115));
#37903=CARTESIAN_POINT('Ctrl Pts',(67.8295738539522,8.64714263134489,-63.9267787167824));
#37904=CARTESIAN_POINT('Ctrl Pts',(67.8281598888321,8.82939594565336,-64.529654252364));
#37905=CARTESIAN_POINT('Ctrl Pts',(67.8272568146161,8.95681579596969,-64.9268321940373));
#37906=CARTESIAN_POINT('Ctrl Pts',(67.8266716120575,9.04324849122267,-65.190295819569));
#37907=CARTESIAN_POINT('Ctrl Pts',(67.8261164977612,9.13180453280574,-65.4519050623698));
#37908=CARTESIAN_POINT('Ctrl Pts',(67.825678111527,9.21087621799224,-65.6790189570298));
#37909=CARTESIAN_POINT('Ctrl Pts',(67.8254430601022,9.25648137965921,-65.8082915981344));
#37910=CARTESIAN_POINT('Ctrl Pts',(67.8251055458828,9.32530445335825,-66.0017181851269));
#37911=CARTESIAN_POINT('Ctrl Pts',(67.8248627228961,9.38345311529571,-66.1618153350162));
#37912=CARTESIAN_POINT('Ctrl Pts',(67.8244873775853,9.48086370737567,-66.4261110285533));
#37913=CARTESIAN_POINT('Ctrl Pts',(67.8223242435178,9.59820079307097,-66.7305374425062));
#37914=CARTESIAN_POINT('Ctrl Pts',(67.8190037054621,9.84021958890711,-67.3072623116103));
#37915=CARTESIAN_POINT('Ctrl Pts',(67.8129957587451,10.2993885429522,-68.2955785243475));
#37916=CARTESIAN_POINT('Ctrl Pts',(67.8042632784492,11.3003828720975,-70.1535166719588));
#37917=CARTESIAN_POINT('Ctrl Pts',(67.8049703733839,12.1759401810533,-71.6137975769271));
#37918=CARTESIAN_POINT('Ctrl Pts',(67.8104034129806,12.7300087363492,-72.6661690355186));
#37919=CARTESIAN_POINT('Ctrl Pts',(67.8099283136533,12.8656678936038,-72.9238529497301));
#37920=CARTESIAN_POINT('Ctrl Pts',(67.8099648416568,13.130499120933,-73.4254282690125));
#37921=CARTESIAN_POINT('Ctrl Pts',(67.8096445242436,13.465062786893,-74.0571725299553));
#37922=CARTESIAN_POINT('Ctrl Pts',(67.8095299586602,13.8657447063598,-74.8110678320985));
#37923=CARTESIAN_POINT('Ctrl Pts',(67.8092757135153,14.6688669633785,-76.3186376482257));
#37924=CARTESIAN_POINT('Ctrl Pts',(67.8093094569773,15.338264183902,-77.5711925878768));
#37925=CARTESIAN_POINT('Ctrl Pts',(67.809574689212,16.3061992093518,-79.3917515508846));
#37926=CARTESIAN_POINT('Ctrl Pts',(67.8094593526752,16.7435423574498,-80.2144112969835));
#37927=CARTESIAN_POINT('Ctrl Pts',(67.809459352675,17.1800639448392,-81.0353889990819));
#37928=CARTESIAN_POINT('Ctrl Pts',(70.6494615867083,3.83081038259429,24.8276527484924));
#37929=CARTESIAN_POINT('Ctrl Pts',(70.6496322197946,3.83090610428414,24.7786798140215));
#37930=CARTESIAN_POINT('Ctrl Pts',(70.6498112335071,3.83100625888237,24.729706115986));
#37931=CARTESIAN_POINT('Ctrl Pts',(70.6519243534644,3.83219418091214,24.1780051253099));
#37932=CARTESIAN_POINT('Ctrl Pts',(70.6530393935946,3.83471357029684,23.1723497522651));
#37933=CARTESIAN_POINT('Ctrl Pts',(70.6553276454399,3.84151431914779,21.1618905015551));
#37934=CARTESIAN_POINT('Ctrl Pts',(70.6694173401099,3.84933576491011,19.6579544827044));
#37935=CARTESIAN_POINT('Ctrl Pts',(70.7017957450429,3.85799813994687,18.4074358300531));
#37936=CARTESIAN_POINT('Ctrl Pts',(70.716679458464,3.86261409154474,17.8992953377625));
#37937=CARTESIAN_POINT('Ctrl Pts',(70.7528580384059,3.8748631628684,16.8915796329347));
#37938=CARTESIAN_POINT('Ctrl Pts',(70.8302073256714,3.90047804800543,15.1380162766548));
#37939=CARTESIAN_POINT('Ctrl Pts',(70.9112737776838,3.91699285560921,13.6541782529586));
#37940=CARTESIAN_POINT('Ctrl Pts',(70.9763136585358,3.91434581461649,12.4237737939805));
#37941=CARTESIAN_POINT('Ctrl Pts',(71.0030615265596,3.91054675463754,11.9395225358356));
#37942=CARTESIAN_POINT('Ctrl Pts',(71.059252040738,3.89423065634749,10.9566776530166));
#37943=CARTESIAN_POINT('Ctrl Pts',(71.1632501986744,3.85093053759193,9.21600588337804));
#37944=CARTESIAN_POINT('Ctrl Pts',(71.258082759856,3.81527809606321,7.6801825507519));
#37945=CARTESIAN_POINT('Ctrl Pts',(71.3272876674223,3.82214129678024,6.50824099154105));
#37946=CARTESIAN_POINT('Ctrl Pts',(71.3427511315147,3.82225228568385,6.28252554743425));
#37947=CARTESIAN_POINT('Ctrl Pts',(71.3749157017795,3.81715545366023,5.80195360798077));
#37948=CARTESIAN_POINT('Ctrl Pts',(71.4340146686344,3.79815526889341,4.94708066621355));
#37949=CARTESIAN_POINT('Ctrl Pts',(71.5592359131306,3.74889711351366,3.13847167959589));
#37950=CARTESIAN_POINT('Ctrl Pts',(71.6637014711367,3.81595624082737,1.43529850844767));
#37951=CARTESIAN_POINT('Ctrl Pts',(71.695580427591,4.05978180199612,0.177804686666928));
#37952=CARTESIAN_POINT('Ctrl Pts',(71.6999732590441,4.08946439535741,0.0303564999101921));
#37953=CARTESIAN_POINT('Ctrl Pts',(71.7086632146237,4.15430759573429,-0.263208884210683));
#37954=CARTESIAN_POINT('Ctrl Pts',(71.7241800042281,4.28010993359288,-0.770233236761601));
#37955=CARTESIAN_POINT('Ctrl Pts',(71.7446746252156,4.49143771191879,-1.47731006830424));
#37956=CARTESIAN_POINT('Ctrl Pts',(71.762159457237,4.78057345871927,-2.29732944268844));
#37957=CARTESIAN_POINT('Ctrl Pts',(71.7719393440816,5.19615493718386,-3.35702174402344));
#37958=CARTESIAN_POINT('Ctrl Pts',(71.7559918046913,5.73883808961284,-4.62551787475727));
#37959=CARTESIAN_POINT('Ctrl Pts',(71.7136458140211,6.14233610559966,-5.60372928407037));
#37960=CARTESIAN_POINT('Ctrl Pts',(71.6746492911468,6.36893997037483,-6.21041150356981));
#37961=CARTESIAN_POINT('Ctrl Pts',(71.6454197256439,6.47958282642054,-6.50916156374574));
#37962=CARTESIAN_POINT('Ctrl Pts',(71.5852832929708,6.69926928674286,-7.06348594446982));
#37963=CARTESIAN_POINT('Ctrl Pts',(71.4592658050832,7.10401302870599,-8.02462303818132));
#37964=CARTESIAN_POINT('Ctrl Pts',(71.2502834631539,7.68573829926759,-9.31372015535913));
#37965=CARTESIAN_POINT('Ctrl Pts',(71.0413556697638,8.17269220545024,-10.4897481554329));
#37966=CARTESIAN_POINT('Ctrl Pts',(70.9194458564485,8.41683332486132,-11.2238938763871));
#37967=CARTESIAN_POINT('Ctrl Pts',(70.8610035588855,8.52564254806769,-11.615056859852));
#37968=CARTESIAN_POINT('Ctrl Pts',(70.8363802328729,8.56936123861665,-11.8004058535334));
#37969=CARTESIAN_POINT('Ctrl Pts',(70.8199004857342,8.59828419220826,-11.9363044116113));
#37970=CARTESIAN_POINT('Ctrl Pts',(70.8088851203888,8.61784702361031,-12.0351348832902));
#37971=CARTESIAN_POINT('Ctrl Pts',(70.7877298701005,8.65261401658615,-12.2300774357788));
#37972=CARTESIAN_POINT('Ctrl Pts',(70.7529125032501,8.70419637134419,-12.5775034833244));
#37973=CARTESIAN_POINT('Ctrl Pts',(70.6746241477646,8.79351350793665,-13.4950523222552));
#37974=CARTESIAN_POINT('Ctrl Pts',(70.6249320620081,8.77854019843266,-14.6202130090127));
#37975=CARTESIAN_POINT('Ctrl Pts',(70.5942999785663,8.73282150953588,-15.8659952169765));
#37976=CARTESIAN_POINT('Ctrl Pts',(70.5806966383333,8.71427565623005,-16.5189882853968));
#37977=CARTESIAN_POINT('Ctrl Pts',(70.5696178200984,8.70844385895726,-17.0599653686636));
#37978=CARTESIAN_POINT('Ctrl Pts',(70.5636838942566,8.71000547360416,-17.336837376577));
#37979=CARTESIAN_POINT('Ctrl Pts',(70.5590254237539,8.71329389796812,-17.5453587994702));
#37980=CARTESIAN_POINT('Ctrl Pts',(70.5561572316978,8.71502260422576,-17.6621814337956));
#37981=CARTESIAN_POINT('Ctrl Pts',(70.5510255856973,8.71822746059492,-17.9085181649483));
#37982=CARTESIAN_POINT('Ctrl Pts',(70.5468012755684,8.72073272086908,-18.150816531429));
#37983=CARTESIAN_POINT('Ctrl Pts',(70.5433888034654,8.72269270957472,-18.3960889291585));
#37984=CARTESIAN_POINT('Ctrl Pts',(70.5415763630612,8.72368369038835,-18.5490734867898));
#37985=CARTESIAN_POINT('Ctrl Pts',(70.5403073344523,8.72435033031262,-18.671805298334));
#37986=CARTESIAN_POINT('Ctrl Pts',(70.5391551996401,8.72493311342539,-18.7945736263313));
#37987=CARTESIAN_POINT('Ctrl Pts',(70.5364509944023,8.72620928357726,-19.1326061682313));
#37988=CARTESIAN_POINT('Ctrl Pts',(70.5343972821601,8.72661516653376,-19.687874997866));
#37989=CARTESIAN_POINT('Ctrl Pts',(70.5355551407817,8.72397510411148,-20.6811247268949));
#37990=CARTESIAN_POINT('Ctrl Pts',(70.5423870553301,8.71703505613488,-21.9344602149432));
#37991=CARTESIAN_POINT('Ctrl Pts',(70.5458672100272,8.71341297499298,-22.9497504021268));
#37992=CARTESIAN_POINT('Ctrl Pts',(70.5450425115542,8.71353162267228,-23.5865416628728));
#37993=CARTESIAN_POINT('Ctrl Pts',(70.5447524535521,8.71358037896091,-23.8349082908723));
#37994=CARTESIAN_POINT('Ctrl Pts',(70.5442983469629,8.7136916662106,-24.3345141000982));
#37995=CARTESIAN_POINT('Ctrl Pts',(70.5438078693597,8.7139106295647,-25.2095714068707));
#37996=CARTESIAN_POINT('Ctrl Pts',(70.5437941381743,8.71424852180923,-26.4642469765464));
#37997=CARTESIAN_POINT('Ctrl Pts',(70.5443287824551,8.71451471806677,-27.9721250967088));
#37998=CARTESIAN_POINT('Ctrl Pts',(70.5446736941038,8.71452884238773,-28.9765652628975));
#37999=CARTESIAN_POINT('Ctrl Pts',(70.5447699397357,8.71445478785512,-29.5405978731148));
#38000=CARTESIAN_POINT('Ctrl Pts',(70.5447892237904,8.71443464959818,-29.6659103240058));
#38001=CARTESIAN_POINT('Ctrl Pts',(70.5448181933689,8.71438230721395,-29.9166154371908));
#38002=CARTESIAN_POINT('Ctrl Pts',(70.54484704347,8.71426257513622,-30.3554914438346));
#38003=CARTESIAN_POINT('Ctrl Pts',(70.5448484874897,8.71392245129362,-31.2337460927015));
#38004=CARTESIAN_POINT('Ctrl Pts',(70.5448503146429,8.71338620005043,-32.2380110739719));
#38005=CARTESIAN_POINT('Ctrl Pts',(70.5451209127849,8.71284402078748,-33.2417255403863));
#38006=CARTESIAN_POINT('Ctrl Pts',(70.545524545668,8.71247043219124,-33.9939571890433));
#38007=CARTESIAN_POINT('Ctrl Pts',(70.5461899905228,8.71217492752451,-34.745310445793));
#38008=CARTESIAN_POINT('Ctrl Pts',(70.5468533445406,8.71205173577247,-35.2454547113171));
#38009=CARTESIAN_POINT('Ctrl Pts',(70.5474518280046,8.7119952320563,-35.6211998712757));
#38010=CARTESIAN_POINT('Ctrl Pts',(70.5479053429065,8.71194401385795,-35.8724813300518));
#38011=CARTESIAN_POINT('Ctrl Pts',(70.5489976699394,8.71180045174142,-36.3747090579339));
#38012=CARTESIAN_POINT('Ctrl Pts',(70.5513235945551,8.71148120053779,-37.25224972174));
#38013=CARTESIAN_POINT('Ctrl Pts',(70.5571200607568,8.71082727063191,-39.0044553013496));
#38014=CARTESIAN_POINT('Ctrl Pts',(70.5622026385591,8.71119028705882,-40.507733876685));
#38015=CARTESIAN_POINT('Ctrl Pts',(70.5642533127471,8.71286542617711,-41.6413563416797));
#38016=CARTESIAN_POINT('Ctrl Pts',(70.5646535512609,8.71307078591043,-41.8892293291521));
#38017=CARTESIAN_POINT('Ctrl Pts',(70.5651134875453,8.7129994767808,-42.2633385288916));
#38018=CARTESIAN_POINT('Ctrl Pts',(70.5654559292171,8.71264828930115,-42.6378971883292));
#38019=CARTESIAN_POINT('Ctrl Pts',(70.5657845586926,8.7119437590644,-43.1387086748049));
#38020=CARTESIAN_POINT('Ctrl Pts',(70.5660106650976,8.71087613352797,-43.7665989444598));
#38021=CARTESIAN_POINT('Ctrl Pts',(70.5661608227567,8.71012005394437,-44.5227896309756));
#38022=CARTESIAN_POINT('Ctrl Pts',(70.566329581619,8.71061958030634,-45.1547199927119));
#38023=CARTESIAN_POINT('Ctrl Pts',(70.5665777677508,8.71212136138571,-45.6610764214851));
#38024=CARTESIAN_POINT('Ctrl Pts',(70.5668416372251,8.71390179747749,-46.0412015657389));
#38025=CARTESIAN_POINT('Ctrl Pts',(70.5672048319196,8.71644188043345,-46.4215992068969));
#38026=CARTESIAN_POINT('Ctrl Pts',(70.5678496720794,8.72098788065634,-46.9291451205241));
#38027=CARTESIAN_POINT('Ctrl Pts',(70.5685468480872,8.72584790750339,-47.3099316252934));
#38028=CARTESIAN_POINT('Ctrl Pts',(70.5694292279528,8.73192477619373,-47.6921253853199));
#38029=CARTESIAN_POINT('Ctrl Pts',(70.5700003368078,8.73772742858547,-47.9611518169856));
#38030=CARTESIAN_POINT('Ctrl Pts',(70.5712314195025,8.75416940983707,-48.48604651909));
#38031=CARTESIAN_POINT('Ctrl Pts',(70.5736110193162,8.79329630484929,-49.3952769089704));
#38032=CARTESIAN_POINT('Ctrl Pts',(70.5779524846989,8.86303714057703,-50.6527605487821));
#38033=CARTESIAN_POINT('Ctrl Pts',(70.5848185478071,8.92405103147752,-52.0999818910618));
#38034=CARTESIAN_POINT('Ctrl Pts',(70.5901264532065,8.92307445153632,-53.020761634185));
#38035=CARTESIAN_POINT('Ctrl Pts',(70.5933774910263,8.90240281065996,-53.5826199270936));
#38036=CARTESIAN_POINT('Ctrl Pts',(70.5945212135569,8.89128249120398,-53.7816814909825));
#38037=CARTESIAN_POINT('Ctrl Pts',(70.5970060354552,8.85414562790396,-54.2126775327943));
#38038=CARTESIAN_POINT('Ctrl Pts',(70.602081823671,8.75468006093425,-54.9974504674917));
#38039=CARTESIAN_POINT('Ctrl Pts',(70.6160221912734,8.46061464007003,-56.7189531513493));
#38040=CARTESIAN_POINT('Ctrl Pts',(70.6351103426861,8.20797913919722,-58.4315994063654));
#38041=CARTESIAN_POINT('Ctrl Pts',(70.6378365999834,8.28745204929791,-59.7672968589652));
#38042=CARTESIAN_POINT('Ctrl Pts',(70.6382848453043,8.29702790860994,-59.9091084957715));
#38043=CARTESIAN_POINT('Ctrl Pts',(70.6389525410391,8.32075687283495,-60.2031166527417));
#38044=CARTESIAN_POINT('Ctrl Pts',(70.6398172088392,8.37204173475601,-60.709263749262));
#38045=CARTESIAN_POINT('Ctrl Pts',(70.6402867499701,8.51277042585894,-61.7148228641222));
#38046=CARTESIAN_POINT('Ctrl Pts',(70.638773558215,8.74946275086096,-62.8347876548578));
#38047=CARTESIAN_POINT('Ctrl Pts',(70.6364542699192,9.04226090895522,-63.9268738865825));
#38048=CARTESIAN_POINT('Ctrl Pts',(70.6350447518703,9.22455564675501,-64.5297344920004));
#38049=CARTESIAN_POINT('Ctrl Pts',(70.6341417987604,9.35199653545435,-64.9268947241361));
#38050=CARTESIAN_POINT('Ctrl Pts',(70.6335546618577,9.43844104194086,-65.190344545352));
#38051=CARTESIAN_POINT('Ctrl Pts',(70.6329927939914,9.52700508046247,-65.4519370729589));
#38052=CARTESIAN_POINT('Ctrl Pts',(70.6325409742643,9.60607918432695,-65.6790338502266));
#38053=CARTESIAN_POINT('Ctrl Pts',(70.6322956459119,9.65168428141731,-65.8082960098274));
#38054=CARTESIAN_POINT('Ctrl Pts',(70.6319398706883,9.72050573437257,-66.0017062053914));
#38055=CARTESIAN_POINT('Ctrl Pts',(70.6316754937635,9.77864972549694,-66.1617882408552));
#38056=CARTESIAN_POINT('Ctrl Pts',(70.6312532272026,9.87604743186078,-66.4260575880187));
#38057=CARTESIAN_POINT('Ctrl Pts',(70.6290371086404,9.99337943718072,-66.7304845122077));
#38058=CARTESIAN_POINT('Ctrl Pts',(70.6256389157257,10.2353858042967,-67.307196740313));
#38059=CARTESIAN_POINT('Ctrl Pts',(70.6195462770368,10.6945410254072,-68.2955029168157));
#38060=CARTESIAN_POINT('Ctrl Pts',(70.6108239238681,11.6955282837264,-70.1534275139502));
#38061=CARTESIAN_POINT('Ctrl Pts',(70.6116930692152,12.5711084944599,-71.6137122376235));
#38062=CARTESIAN_POINT('Ctrl Pts',(70.6171581906643,13.1251914954288,-72.6660905521361));
#38063=CARTESIAN_POINT('Ctrl Pts',(70.6166812737942,13.2608498799591,-72.9237733872693));
#38064=CARTESIAN_POINT('Ctrl Pts',(70.6167190088863,13.5256816230138,-73.4253481416168));
#38065=CARTESIAN_POINT('Ctrl Pts',(70.6163977241997,13.8602447820587,-74.057091397903));
#38066=CARTESIAN_POINT('Ctrl Pts',(70.6162826798284,14.2609262348746,-74.8109860365976));
#38067=CARTESIAN_POINT('Ctrl Pts',(70.616026343113,15.0640469642179,-76.3185549194688));
#38068=CARTESIAN_POINT('Ctrl Pts',(70.6160585036137,15.7334432769212,-77.5711107183318));
#38069=CARTESIAN_POINT('Ctrl Pts',(70.6163251147076,16.7013796602407,-79.3916714502491));
#38070=CARTESIAN_POINT('Ctrl Pts',(70.61620923224,17.1387224495204,-80.2143308256623));
#38071=CARTESIAN_POINT('Ctrl Pts',(70.6162092322401,17.5752440369097,-81.0353085277609));
#38072=CARTESIAN_POINT('Ctrl Pts',(73.4534500542343,4.22530703961414,24.8335658669903));
#38073=CARTESIAN_POINT('Ctrl Pts',(73.4535261461378,4.22524543761862,24.7847807094142));
#38074=CARTESIAN_POINT('Ctrl Pts',(73.4536061943624,4.22518075424666,24.7359974325107));
#38075=CARTESIAN_POINT('Ctrl Pts',(73.4545512309376,4.22442705508417,24.1865265777239));
#38076=CARTESIAN_POINT('Ctrl Pts',(73.4518393006747,4.22214471221797,23.1833994211906));
#38077=CARTESIAN_POINT('Ctrl Pts',(73.4432871874621,4.21564347341985,21.1771448625688));
#38078=CARTESIAN_POINT('Ctrl Pts',(73.4496477417741,4.21095875268741,19.675290208693));
#38079=CARTESIAN_POINT('Ctrl Pts',(73.4803655216321,4.20940140260513,18.4259537057235));
#38080=CARTESIAN_POINT('Ctrl Pts',(73.4934052258452,4.20716909151018,17.932690249231));
#38081=CARTESIAN_POINT('Ctrl Pts',(73.5231636817857,4.19898855516301,16.9350263109554));
#38082=CARTESIAN_POINT('Ctrl Pts',(73.5876238488452,4.18199957258835,15.1776786176254));
#38083=CARTESIAN_POINT('Ctrl Pts',(73.6730048552458,4.18371618038397,13.6462334631478));
#38084=CARTESIAN_POINT('Ctrl Pts',(73.7707468465167,4.21638754708557,12.3551073610112));
#38085=CARTESIAN_POINT('Ctrl Pts',(73.8141206538761,4.22930990269526,11.8605690057779));
#38086=CARTESIAN_POINT('Ctrl Pts',(73.9145642754093,4.25858474957933,10.8516399198657));
#38087=CARTESIAN_POINT('Ctrl Pts',(74.1168743384341,4.32647233590466,9.07410025684771));
#38088=CARTESIAN_POINT('Ctrl Pts',(74.3029360600045,4.4425032821772,7.50898960266336));
#38089=CARTESIAN_POINT('Ctrl Pts',(74.4141506591024,4.58646542369393,6.31641947569288));
#38090=CARTESIAN_POINT('Ctrl Pts',(74.4407928859277,4.61616562076266,6.06973731158189));
#38091=CARTESIAN_POINT('Ctrl Pts',(74.4971534009537,4.6806267462007,5.56172564630839));
#38092=CARTESIAN_POINT('Ctrl Pts',(74.601678333609,4.8034795552565,4.66722232741208));
#38093=CARTESIAN_POINT('Ctrl Pts',(74.8082987931951,5.10837288549013,2.83336863996513));
#38094=CARTESIAN_POINT('Ctrl Pts',(74.8896403398205,5.4850325276308,1.22545573439517));
#38095=CARTESIAN_POINT('Ctrl Pts',(74.8560557798504,5.79782347580794,0.0737985541994678));
#38096=CARTESIAN_POINT('Ctrl Pts',(74.85013591491,5.83828359682733,-0.0741003001395361));
#38097=CARTESIAN_POINT('Ctrl Pts',(74.8368000379755,5.92109119870578,-0.360513775030337));
#38098=CARTESIAN_POINT('Ctrl Pts',(74.8077813744316,6.07422124244255,-0.857580978294587));
#38099=CARTESIAN_POINT('Ctrl Pts',(74.7543900602967,6.30982836377159,-1.54628365855503));
#38100=CARTESIAN_POINT('Ctrl Pts',(74.6794527915681,6.60760335801143,-2.34684895453022));
#38101=CARTESIAN_POINT('Ctrl Pts',(74.5732518390376,7.00990054092547,-3.38247175253405));
#38102=CARTESIAN_POINT('Ctrl Pts',(74.4409539994718,7.4958887565096,-4.62234763704644));
#38103=CARTESIAN_POINT('Ctrl Pts',(74.3475250999459,7.80738682333361,-5.54684334097161));
#38104=CARTESIAN_POINT('Ctrl Pts',(74.2938139307462,7.96133952783586,-6.0988766407598));
#38105=CARTESIAN_POINT('Ctrl Pts',(74.2647775466287,8.03246032546773,-6.36322088900162));
#38106=CARTESIAN_POINT('Ctrl Pts',(74.2041405975534,8.16462668068318,-6.86450029538272));
#38107=CARTESIAN_POINT('Ctrl Pts',(74.082310243454,8.38762885031026,-7.74660588572107));
#38108=CARTESIAN_POINT('Ctrl Pts',(73.8765336055004,8.67004719556913,-8.96897319517573));
#38109=CARTESIAN_POINT('Ctrl Pts',(73.6612677870246,8.90659584048753,-10.136850718449));
#38110=CARTESIAN_POINT('Ctrl Pts',(73.5369674395633,9.04056470444529,-10.9203298436466));
#38111=CARTESIAN_POINT('Ctrl Pts',(73.4783954127976,9.10574908890705,-11.3597543307435));
#38112=CARTESIAN_POINT('Ctrl Pts',(73.4540520371645,9.1340838595355,-11.576618913669));
#38113=CARTESIAN_POINT('Ctrl Pts',(73.4378760186849,9.15358601547536,-11.738750893759));
#38114=CARTESIAN_POINT('Ctrl Pts',(73.4277279991916,9.16489552177659,-11.8419683144316));
#38115=CARTESIAN_POINT('Ctrl Pts',(73.4094336380798,9.18538844204145,-12.0534225491334));
#38116=CARTESIAN_POINT('Ctrl Pts',(73.3828098713282,9.21382756833954,-12.4260873709192));
#38117=CARTESIAN_POINT('Ctrl Pts',(73.3396199506344,9.25366717695632,-13.4097635557345));
#38118=CARTESIAN_POINT('Ctrl Pts',(73.3513919908944,9.21041740505572,-14.579844251102));
#38119=CARTESIAN_POINT('Ctrl Pts',(73.3724351517644,9.15254998529332,-15.8391607356278));
#38120=CARTESIAN_POINT('Ctrl Pts',(73.3809135708858,9.12816610581944,-16.4913838822319));
#38121=CARTESIAN_POINT('Ctrl Pts',(73.3838015871584,9.11595394197832,-17.0271642040383));
#38122=CARTESIAN_POINT('Ctrl Pts',(73.3834810356021,9.11322709619638,-17.2998548135131));
#38123=CARTESIAN_POINT('Ctrl Pts',(73.3824118783939,9.11277040383227,-17.5049039873859));
#38124=CARTESIAN_POINT('Ctrl Pts',(73.3817303794556,9.11252511086424,-17.6264661651878));
#38125=CARTESIAN_POINT('Ctrl Pts',(73.3804945331111,9.11204419200424,-17.8778405066787));
#38126=CARTESIAN_POINT('Ctrl Pts',(73.3794318496841,9.11163048321859,-18.1262675031507));
#38127=CARTESIAN_POINT('Ctrl Pts',(73.3785303839214,9.11125930326834,-18.376417266739));
#38128=CARTESIAN_POINT('Ctrl Pts',(73.3780294989107,9.11104885276049,-18.5324459754145));
#38129=CARTESIAN_POINT('Ctrl Pts',(73.3776646905098,9.11089109109327,-18.6574341720327));
#38130=CARTESIAN_POINT('Ctrl Pts',(73.3773229575204,9.11074085129781,-18.782403736847));
#38131=CARTESIAN_POINT('Ctrl Pts',(73.3764752540345,9.1103577006343,-19.126171262133));
#38132=CARTESIAN_POINT('Ctrl Pts',(73.375560929654,9.10988412298222,-19.6891487734336));
#38133=CARTESIAN_POINT('Ctrl Pts',(73.37492459789,9.10937069259306,-20.6913692318905));
#38134=CARTESIAN_POINT('Ctrl Pts',(73.3753250105335,9.1091511101525,-21.9470238577363));
#38135=CARTESIAN_POINT('Ctrl Pts',(73.3754902779273,9.10896297491011,-22.9548467423427));
#38136=CARTESIAN_POINT('Ctrl Pts',(73.3750953915219,9.10869646092465,-23.5842032232804));
#38137=CARTESIAN_POINT('Ctrl Pts',(73.3749589661061,9.10859484477579,-23.8334633318891));
#38138=CARTESIAN_POINT('Ctrl Pts',(73.374757891282,9.10840641206924,-24.3327077001457));
#38139=CARTESIAN_POINT('Ctrl Pts',(73.3745720422855,9.10811659521834,-25.2082704533436));
#38140=CARTESIAN_POINT('Ctrl Pts',(73.3746618262452,9.10783137522724,-26.4631295916326));
#38141=CARTESIAN_POINT('Ctrl Pts',(73.3749657200172,9.10770078254226,-27.9717563735793));
#38142=CARTESIAN_POINT('Ctrl Pts',(73.3750395148263,9.10776770662891,-28.9767329786706));
#38143=CARTESIAN_POINT('Ctrl Pts',(73.374971844802,9.10784600977214,-29.5411142749989));
#38144=CARTESIAN_POINT('Ctrl Pts',(73.3749520653695,9.10786501892074,-29.6665536455528));
#38145=CARTESIAN_POINT('Ctrl Pts',(73.3748952785016,9.10791093907323,-29.9174696229282));
#38146=CARTESIAN_POINT('Ctrl Pts',(73.374754720345,9.10801155353313,-30.356701473297));
#38147=CARTESIAN_POINT('Ctrl Pts',(73.374343963929,9.10828383298627,-31.235529090884));
#38148=CARTESIAN_POINT('Ctrl Pts',(73.3737352665426,9.10872849397928,-32.240171135434));
#38149=CARTESIAN_POINT('Ctrl Pts',(73.3733039339751,9.10923386491297,-33.2439532345848));
#38150=CARTESIAN_POINT('Ctrl Pts',(73.3731483647105,9.10962642968375,-33.9960783367514));
#38151=CARTESIAN_POINT('Ctrl Pts',(73.3732390933077,9.11002142319734,-34.7471853776243));
#38152=CARTESIAN_POINT('Ctrl Pts',(73.3735168372938,9.11027405601257,-35.2470629337144));
#38153=CARTESIAN_POINT('Ctrl Pts',(73.3738272805288,9.11045526780762,-35.6225726730903));
#38154=CARTESIAN_POINT('Ctrl Pts',(73.3740783756241,9.11055927079173,-35.8738667644384));
#38155=CARTESIAN_POINT('Ctrl Pts',(73.3747327033794,9.11071066242431,-36.3760208794514));
#38156=CARTESIAN_POINT('Ctrl Pts',(73.3762244220803,9.11086826910444,-37.2534866607658));
#38157=CARTESIAN_POINT('Ctrl Pts',(73.3801775570183,9.11102577369151,-39.005485963845));
#38158=CARTESIAN_POINT('Ctrl Pts',(73.3837917918894,9.11189357371564,-40.5086054277271));
#38159=CARTESIAN_POINT('Ctrl Pts',(73.3851792829503,9.11389947437443,-41.6420873839513));
#38160=CARTESIAN_POINT('Ctrl Pts',(73.3854450145328,9.11417701530638,-41.8899447419186));
#38161=CARTESIAN_POINT('Ctrl Pts',(73.3857372125606,9.1142140555757,-42.2640189060008));
#38162=CARTESIAN_POINT('Ctrl Pts',(73.3859411380443,9.11396919579392,-42.6385418757349));
#38163=CARTESIAN_POINT('Ctrl Pts',(73.3861185940242,9.1134023526539,-43.139299737331));
#38164=CARTESIAN_POINT('Ctrl Pts',(73.3862074374739,9.11249544850946,-43.7671150597367));
#38165=CARTESIAN_POINT('Ctrl Pts',(73.3862410262631,9.11190324748228,-44.5232019152918));
#38166=CARTESIAN_POINT('Ctrl Pts',(73.3863239318621,9.1125059872366,-45.1550349083222));
#38167=CARTESIAN_POINT('Ctrl Pts',(73.3864921887458,9.11406440388159,-45.6613053538075));
#38168=CARTESIAN_POINT('Ctrl Pts',(73.3866864657229,9.1158731191196,-46.0413625920448));
#38169=CARTESIAN_POINT('Ctrl Pts',(73.3869660099852,9.11842584219486,-46.4216887641487));
#38170=CARTESIAN_POINT('Ctrl Pts',(73.38747481916,9.12296591629808,-46.9291343438024));
#38171=CARTESIAN_POINT('Ctrl Pts',(73.3880358469146,9.12779386455806,-47.3098405435582));
#38172=CARTESIAN_POINT('Ctrl Pts',(73.3887503569359,9.13381707555844,-47.691948928767));
#38173=CARTESIAN_POINT('Ctrl Pts',(73.3892102426715,9.13957410884946,-47.9608941784767));
#38174=CARTESIAN_POINT('Ctrl Pts',(73.3902179406663,9.15589543877677,-48.4856545677139));
#38175=CARTESIAN_POINT('Ctrl Pts',(73.3921985051051,9.19474065609386,-49.3946756678471));
#38176=CARTESIAN_POINT('Ctrl Pts',(73.3959021785531,9.26392505198861,-50.6519574390876));
#38177=CARTESIAN_POINT('Ctrl Pts',(73.4017820248472,9.32415959397272,-52.0990825771574));
#38178=CARTESIAN_POINT('Ctrl Pts',(73.4062117762354,9.32265822262322,-53.0199084620258));
#38179=CARTESIAN_POINT('Ctrl Pts',(73.4088249153412,9.3016739371985,-53.5818290458706));
#38180=CARTESIAN_POINT('Ctrl Pts',(73.4096908343255,9.29043617440867,-53.7808133826808));
#38181=CARTESIAN_POINT('Ctrl Pts',(73.4115519159643,9.25302703661083,-54.2117394820634));
#38182=CARTESIAN_POINT('Ctrl Pts',(73.4153808109127,9.15301479350725,-54.9964162298912));
#38183=CARTESIAN_POINT('Ctrl Pts',(73.4264123496012,8.8576334816423,-56.7179266148824));
#38184=CARTESIAN_POINT('Ctrl Pts',(73.4430779286312,8.60377321678145,-58.4308178751789));
#38185=CARTESIAN_POINT('Ctrl Pts',(73.444838502715,8.68284878733253,-59.7669036929714));
#38186=CARTESIAN_POINT('Ctrl Pts',(73.4451721176443,8.69238362667795,-59.9087566277868));
#38187=CARTESIAN_POINT('Ctrl Pts',(73.4456240207106,8.71603985479539,-60.2028457441212));
#38188=CARTESIAN_POINT('Ctrl Pts',(73.446143750728,8.76722709000681,-60.709121606154));
#38189=CARTESIAN_POINT('Ctrl Pts',(73.4460455539418,8.90785948285092,-61.7148923746929));
#38190=CARTESIAN_POINT('Ctrl Pts',(73.4441177941321,9.14460506842151,-62.8349929840275));
#38191=CARTESIAN_POINT('Ctrl Pts',(73.4415270623419,9.43750285592813,-63.9271205232897));
#38192=CARTESIAN_POINT('Ctrl Pts',(73.4400005326718,9.6198518088817,-64.5299709949832));
#38193=CARTESIAN_POINT('Ctrl Pts',(73.4390267578198,9.74731987964292,-64.9271111701042));
#38194=CARTESIAN_POINT('Ctrl Pts',(73.4383938206596,9.83377965730146,-65.1905440689006));
#38195=CARTESIAN_POINT('Ctrl Pts',(73.4377874324485,9.9223538360786,-65.4521145233453));
#38196=CARTESIAN_POINT('Ctrl Pts',(73.4372964622778,10.0014310286135,-65.6791873567961));
#38197=CARTESIAN_POINT('Ctrl Pts',(73.4370285010553,10.0470360365303,-65.8084345186529));
#38198=CARTESIAN_POINT('Ctrl Pts',(73.4366384216936,10.1158554304746,-66.001820943482));
#38199=CARTESIAN_POINT('Ctrl Pts',(73.4363444861434,10.1739933922247,-66.1618803559984));
#38200=CARTESIAN_POINT('Ctrl Pts',(73.4358709744576,10.2713748692444,-66.4261095447157));
#38201=CARTESIAN_POINT('Ctrl Pts',(73.4336107433578,10.3887104406191,-66.73054466064));
#38202=CARTESIAN_POINT('Ctrl Pts',(73.430148174877,10.6307141189376,-67.3072458305105));
#38203=CARTESIAN_POINT('Ctrl Pts',(73.4240012424698,11.0898737170571,-68.2955485558258));
#38204=CARTESIAN_POINT('Ctrl Pts',(73.4153423680144,12.0908750091205,-70.1534602311583));
#38205=CARTESIAN_POINT('Ctrl Pts',(73.4163672214855,12.9664743628694,-71.6137496163334));
#38206=CARTESIAN_POINT('Ctrl Pts',(73.4218150309494,13.5205581904781,-72.6661328912094));
#38207=CARTESIAN_POINT('Ctrl Pts',(73.4213389989221,13.6562169812378,-72.9238146915836));
#38208=CARTESIAN_POINT('Ctrl Pts',(73.4213760062523,13.9210491080679,-73.4253886789845));
#38209=CARTESIAN_POINT('Ctrl Pts',(73.4210551940842,14.2556124364939,-74.0571308278724));
#38210=CARTESIAN_POINT('Ctrl Pts',(73.4209404667533,14.6562935493408,-74.8110245846817));
#38211=CARTESIAN_POINT('Ctrl Pts',(73.4206854856395,15.4594130397602,-76.3185921935163));
#38212=CARTESIAN_POINT('Ctrl Pts',(73.4207187415443,16.1288080248881,-77.5711489603293));
#38213=CARTESIAN_POINT('Ctrl Pts',(73.4209844325267,17.0967453127965,-79.3917120641317));
#38214=CARTESIAN_POINT('Ctrl Pts',(73.4208688751132,17.534087889402,-80.2143709854359));
#38215=CARTESIAN_POINT('Ctrl Pts',(73.4208688751139,17.9706094767917,-81.035348687534));
#38216=CARTESIAN_POINT('Ctrl Pts',(76.2590036766147,4.61859585860129,24.8393189247761));
#38217=CARTESIAN_POINT('Ctrl Pts',(76.2592676270511,4.61842433362789,24.7907142376174));
#38218=CARTESIAN_POINT('Ctrl Pts',(76.259544344814,4.61824484467112,24.7421096031221));
#38219=CARTESIAN_POINT('Ctrl Pts',(76.2628175286996,4.61612267835582,24.1948928050072));
#38220=CARTESIAN_POINT('Ctrl Pts',(76.2639556688969,4.60859814771707,23.1986363586193));
#38221=CARTESIAN_POINT('Ctrl Pts',(76.2656134729886,4.5871973764053,21.1946693826308));
#38222=CARTESIAN_POINT('Ctrl Pts',(76.2875108300358,4.57291605684706,19.6882732104818));
#38223=CARTESIAN_POINT('Ctrl Pts',(76.3407769139473,4.57211738482582,18.4315980169902));
#38224=CARTESIAN_POINT('Ctrl Pts',(76.3647952026638,4.56784493819628,17.9582353768577));
#38225=CARTESIAN_POINT('Ctrl Pts',(76.4225707356139,4.54820045830769,16.9721940721953));
#38226=CARTESIAN_POINT('Ctrl Pts',(76.5461507315241,4.50383685775637,15.2086150331147));
#38227=CARTESIAN_POINT('Ctrl Pts',(76.6816328251804,4.51394742999633,13.604103234509));
#38228=CARTESIAN_POINT('Ctrl Pts',(76.7973134235421,4.64070067877184,12.2178313104145));
#38229=CARTESIAN_POINT('Ctrl Pts',(76.8482846182611,4.6959007062244,11.6963571978168));
#38230=CARTESIAN_POINT('Ctrl Pts',(76.9619010427407,4.83491465463365,10.6384381496348));
#38231=CARTESIAN_POINT('Ctrl Pts',(77.1773114937794,5.14739340279784,8.80323228594006));
#38232=CARTESIAN_POINT('Ctrl Pts',(77.3359786624805,5.52637920512046,7.2324101828848));
#38233=CARTESIAN_POINT('Ctrl Pts',(77.3978386221007,5.84607093393154,6.05183145962771));
#38234=CARTESIAN_POINT('Ctrl Pts',(77.4104440826745,5.92294208370831,5.77136055629867));
#38235=CARTESIAN_POINT('Ctrl Pts',(77.4347134233158,6.08613463998106,5.22885950434643));
#38236=CARTESIAN_POINT('Ctrl Pts',(77.471937172593,6.39735498949603,4.29054285111247));
#38237=CARTESIAN_POINT('Ctrl Pts',(77.5145027935911,7.0818025705993,2.48801682144282));
#38238=CARTESIAN_POINT('Ctrl Pts',(77.4910544212567,7.65143597159282,1.04581588660632));
#38239=CARTESIAN_POINT('Ctrl Pts',(77.4563839266263,7.93937104286881,0.0587093473684586));
#38240=CARTESIAN_POINT('Ctrl Pts',(77.4493287306598,7.97629022026226,-0.0741408717249266));
#38241=CARTESIAN_POINT('Ctrl Pts',(77.4352764439675,8.04762450080056,-0.330701574080755));
#38242=CARTESIAN_POINT('Ctrl Pts',(77.4064449579892,8.17091110776995,-0.78274962825136));
#38243=CARTESIAN_POINT('Ctrl Pts',(77.3563221876615,8.33976514909286,-1.42166202765295));
#38244=CARTESIAN_POINT('Ctrl Pts',(77.2826934866484,8.53037197855714,-2.18023274413119));
#38245=CARTESIAN_POINT('Ctrl Pts',(77.1698662581585,8.76522838164144,-3.17513501720164));
#38246=CARTESIAN_POINT('Ctrl Pts',(77.0078560361427,9.0165802652799,-4.38307638235827));
#38247=CARTESIAN_POINT('Ctrl Pts',(76.8810645642699,9.16472063733229,-5.3041822170234));
#38248=CARTESIAN_POINT('Ctrl Pts',(76.8143606679954,9.23977858033352,-5.86669711176399));
#38249=CARTESIAN_POINT('Ctrl Pts',(76.7876061568717,9.266926356809,-6.09824862163579));
#38250=CARTESIAN_POINT('Ctrl Pts',(76.7305215689549,9.31381517204141,-6.56031303999017));
#38251=CARTESIAN_POINT('Ctrl Pts',(76.623822642093,9.3779155277621,-7.37656498058418));
#38252=CARTESIAN_POINT('Ctrl Pts',(76.4588572052781,9.43436856860635,-8.55885909257655));
#38253=CARTESIAN_POINT('Ctrl Pts',(76.3083552744269,9.47478631504437,-9.77012444616046));
#38254=CARTESIAN_POINT('Ctrl Pts',(76.2268866003434,9.50274871976792,-10.6328070530146));
#38255=CARTESIAN_POINT('Ctrl Pts',(76.1889647647772,9.51944356435535,-11.1295119194356));
#38256=CARTESIAN_POINT('Ctrl Pts',(76.1732048820239,9.5282313628706,-11.3791645664889));
#38257=CARTESIAN_POINT('Ctrl Pts',(76.1626496791194,9.5350723706033,-11.5673286472237));
#38258=CARTESIAN_POINT('Ctrl Pts',(76.1561044817567,9.5389808438474,-11.6835147323112));
#38259=CARTESIAN_POINT('Ctrl Pts',(76.1449164746475,9.54587575628024,-11.9221801824993));
#38260=CARTESIAN_POINT('Ctrl Pts',(76.1301509865121,9.55494466884804,-12.3381363417809));
#38261=CARTESIAN_POINT('Ctrl Pts',(76.1141476656422,9.5648467015866,-13.4170088493667));
#38262=CARTESIAN_POINT('Ctrl Pts',(76.1462414682578,9.54491422434753,-14.6383040341395));
#38263=CARTESIAN_POINT('Ctrl Pts',(76.1814607883465,9.52362279337754,-15.894220196008));
#38264=CARTESIAN_POINT('Ctrl Pts',(76.1958833316405,9.51493334637066,-16.5310026710859));
#38265=CARTESIAN_POINT('Ctrl Pts',(76.2032117585579,9.51049495165966,-17.046382647654));
#38266=CARTESIAN_POINT('Ctrl Pts',(76.2050790182465,9.5093235528455,-17.3060970096061));
#38267=CARTESIAN_POINT('Ctrl Pts',(76.2056606273789,9.50892263229608,-17.5007250548875));
#38268=CARTESIAN_POINT('Ctrl Pts',(76.2060184706633,9.50867014132164,-17.6246100787378));
#38269=CARTESIAN_POINT('Ctrl Pts',(76.2066327169784,9.50821630284198,-17.8752336778117));
#38270=CARTESIAN_POINT('Ctrl Pts',(76.2070999316946,9.50783368567201,-18.1248775363383));
#38271=CARTESIAN_POINT('Ctrl Pts',(76.2074393459038,9.50751639611427,-18.3751636995251));
#38272=CARTESIAN_POINT('Ctrl Pts',(76.2076003451942,9.50734337631093,-18.5315010636906));
#38273=CARTESIAN_POINT('Ctrl Pts',(76.2077008744814,9.50721940852223,-18.6566402448602));
#38274=CARTESIAN_POINT('Ctrl Pts',(76.2077830451556,9.50710470991487,-18.781780794401));
#38275=CARTESIAN_POINT('Ctrl Pts',(76.2079349339152,9.50682601690064,-19.1259787582423));
#38276=CARTESIAN_POINT('Ctrl Pts',(76.2078128004655,9.50655792868122,-19.6895414673316));
#38277=CARTESIAN_POINT('Ctrl Pts',(76.2068697612793,9.50646427618187,-20.6924456477076));
#38278=CARTESIAN_POINT('Ctrl Pts',(76.2049543558568,9.50677808697286,-21.9482349694304));
#38279=CARTESIAN_POINT('Ctrl Pts',(76.203958537714,9.50690801497891,-22.9554528492817));
#38280=CARTESIAN_POINT('Ctrl Pts',(76.2039285981864,9.50677138616243,-23.5842091939704));
#38281=CARTESIAN_POINT('Ctrl Pts',(76.2039311347776,9.50671986233443,-23.8335357791018));
#38282=CARTESIAN_POINT('Ctrl Pts',(76.2039825343625,9.50662769705605,-24.3327384697341));
#38283=CARTESIAN_POINT('Ctrl Pts',(76.2041753964794,9.50649314315013,-25.2083158964201));
#38284=CARTESIAN_POINT('Ctrl Pts',(76.2046272231609,9.50637007241075,-26.4631392982103));
#38285=CARTESIAN_POINT('Ctrl Pts',(76.2050840179851,9.5063208851935,-27.9716989624441));
#38286=CARTESIAN_POINT('Ctrl Pts',(76.2050838163052,9.50634879469455,-28.9766009445786));
#38287=CARTESIAN_POINT('Ctrl Pts',(76.2049320907037,9.50638032028333,-29.5409277274078));
#38288=CARTESIAN_POINT('Ctrl Pts',(76.2048918219022,9.50638821118415,-29.666345751297));
#38289=CARTESIAN_POINT('Ctrl Pts',(76.2047860045326,9.50640681192304,-29.9172262835149));
#38290=CARTESIAN_POINT('Ctrl Pts',(76.2045395599007,9.50644670041097,-30.3563998095175));
#38291=CARTESIAN_POINT('Ctrl Pts',(76.2038416766349,9.50655408259969,-31.2351348597051));
#38292=CARTESIAN_POINT('Ctrl Pts',(76.2027578708194,9.50673109815979,-32.2397225010295));
#38293=CARTESIAN_POINT('Ctrl Pts',(76.2017524308679,9.50694563130845,-33.2434991114049));
#38294=CARTESIAN_POINT('Ctrl Pts',(76.2011285677281,9.50712068230683,-33.9956434809428));
#38295=CARTESIAN_POINT('Ctrl Pts',(76.2007252022021,9.5073048364333,-34.7467978244661));
#38296=CARTESIAN_POINT('Ctrl Pts',(76.2006640374012,9.50743052225041,-35.2467244669251));
#38297=CARTESIAN_POINT('Ctrl Pts',(76.2007189105449,9.50752525625275,-35.622276173328));
#38298=CARTESIAN_POINT('Ctrl Pts',(76.2007883358698,9.50757016226445,-35.8735687461266));
#38299=CARTESIAN_POINT('Ctrl Pts',(76.2010434311644,9.50760144195324,-36.3757362086335));
#38300=CARTESIAN_POINT('Ctrl Pts',(76.2017574405851,9.50753650552576,-37.2532213547367));
#38301=CARTESIAN_POINT('Ctrl Pts',(76.2039545767969,9.5072513251119,-39.0052620549296));
#38302=CARTESIAN_POINT('Ctrl Pts',(76.206126750897,9.50776410084192,-40.5084303125359));
#38303=CARTESIAN_POINT('Ctrl Pts',(76.2068674914565,9.50959494160429,-41.6419434750376));
#38304=CARTESIAN_POINT('Ctrl Pts',(76.2070026761808,9.50983789499437,-41.8898027095891));
#38305=CARTESIAN_POINT('Ctrl Pts',(76.2071320080402,9.50982784025946,-42.2638829212183));
#38306=CARTESIAN_POINT('Ctrl Pts',(76.2072014362706,9.50954136566926,-42.6384117975113));
#38307=CARTESIAN_POINT('Ctrl Pts',(76.2072316055659,9.50892484198801,-43.1391793194606));
#38308=CARTESIAN_POINT('Ctrl Pts',(76.2071851505408,9.50796609456154,-43.76700866489));
#38309=CARTESIAN_POINT('Ctrl Pts',(76.2070991026037,9.50732373313355,-44.5231165146298));
#38310=CARTESIAN_POINT('Ctrl Pts',(76.2070884073366,9.50789121619783,-45.1549708306134));
#38311=CARTESIAN_POINT('Ctrl Pts',(76.2071669746945,9.50942463486588,-45.6612586675138));
#38312=CARTESIAN_POINT('Ctrl Pts',(76.2072824929622,9.5112151213506,-46.0413301443371));
#38313=CARTESIAN_POINT('Ctrl Pts',(76.2074673026926,9.5137497869097,-46.4216716023164));
#38314=CARTESIAN_POINT('Ctrl Pts',(76.2078223026706,9.5182653104936,-46.9291383597721));
#38315=CARTESIAN_POINT('Ctrl Pts',(76.2082312789042,9.52307370849484,-47.3098632961747));
#38316=CARTESIAN_POINT('Ctrl Pts',(76.2087589593374,9.5290754095034,-47.6919903466628));
#38317=CARTESIAN_POINT('Ctrl Pts',(76.2090927997495,9.53481972517867,-47.9609551129328));
#38318=CARTESIAN_POINT('Ctrl Pts',(76.2098414512392,9.55111981400484,-48.4857460181741));
#38319=CARTESIAN_POINT('Ctrl Pts',(76.2113469227438,9.58993601670354,-49.3948129839473));
#38320=CARTESIAN_POINT('Ctrl Pts',(76.2142833548468,9.65909393983966,-50.65213186042));
#38321=CARTESIAN_POINT('Ctrl Pts',(76.2190264986818,9.71927591471838,-52.0992608602766));
#38322=CARTESIAN_POINT('Ctrl Pts',(76.2225088710447,9.7177154226995,-53.020066261725));
#38323=CARTESIAN_POINT('Ctrl Pts',(76.2244549931009,9.6966778945239,-53.581967440294));
#38324=CARTESIAN_POINT('Ctrl Pts',(76.225035007649,9.68541465582122,-53.7809575537511));
#38325=CARTESIAN_POINT('Ctrl Pts',(76.2262568620834,9.64795036230627,-54.2118872595482));
#38326=CARTESIAN_POINT('Ctrl Pts',(76.2288167885687,9.54783156701677,-54.9965732007058));
#38327=CARTESIAN_POINT('Ctrl Pts',(76.236898472628,9.25220174007932,-56.7180959689487));
#38328=CARTESIAN_POINT('Ctrl Pts',(76.2510991373395,8.9981673470454,-58.4309626675799));
#38329=CARTESIAN_POINT('Ctrl Pts',(76.2518790547583,9.07715845498505,-59.766985659836));
#38330=CARTESIAN_POINT('Ctrl Pts',(76.2520969510277,9.08668144561503,-59.9088314444499));
#38331=CARTESIAN_POINT('Ctrl Pts',(76.2523314530188,9.11031499731494,-60.2029068149855));
#38332=CARTESIAN_POINT('Ctrl Pts',(76.2525057894986,9.16146302212859,-60.7091605105868));
#38333=CARTESIAN_POINT('Ctrl Pts',(76.2518458409884,9.30202082941623,-61.7148952460834));
#38334=CARTESIAN_POINT('Ctrl Pts',(76.249520620965,9.53869253043827,-62.8349750285185));
#38335=CARTESIAN_POINT('Ctrl Pts',(76.2466748244391,9.83153217266925,-63.9271011416989));
#38336=CARTESIAN_POINT('Ctrl Pts',(76.245038643789,10.0138542845839,-64.5299573523145));
#38337=CARTESIAN_POINT('Ctrl Pts',(76.2439976050462,10.1413071595377,-64.9271036563846));
#38338=CARTESIAN_POINT('Ctrl Pts',(76.2433208040966,10.2277574522173,-65.190541278871));
#38339=CARTESIAN_POINT('Ctrl Pts',(76.2426712695385,10.3163232784996,-65.4521172547543));
#38340=CARTESIAN_POINT('Ctrl Pts',(76.2421416178469,10.3953940026921,-65.6791956689038));
#38341=CARTESIAN_POINT('Ctrl Pts',(76.2418510869757,10.4409955708514,-65.808446214391));
#38342=CARTESIAN_POINT('Ctrl Pts',(76.2414265822491,10.5098100504663,-66.0018379033021));
#38343=CARTESIAN_POINT('Ctrl Pts',(76.2411025706284,10.5679444806704,-66.1619021108702));
#38344=CARTESIAN_POINT('Ctrl Pts',(76.2405762973677,10.6653207116708,-66.4261395776643));
#38345=CARTESIAN_POINT('Ctrl Pts',(76.2382736295417,10.782650343015,-66.7305752420116));
#38346=CARTESIAN_POINT('Ctrl Pts',(76.2347476360257,11.0246466535472,-67.3072811653499));
#38347=CARTESIAN_POINT('Ctrl Pts',(76.2285480902281,11.4838012691017,-68.2955882384519));
#38348=CARTESIAN_POINT('Ctrl Pts',(76.2199518240085,12.4848160711236,-70.1535050170501));
#38349=CARTESIAN_POINT('Ctrl Pts',(76.2211301356414,13.3604371029294,-71.6137934767777));
#38350=CARTESIAN_POINT('Ctrl Pts',(76.2265603989672,13.9145144198684,-72.6661742339041));
#38351=CARTESIAN_POINT('Ctrl Pts',(76.2260852072361,14.0501736049526,-72.923856427483));
#38352=CARTESIAN_POINT('Ctrl Pts',(76.2261213973963,14.3150055295701,-73.4254306080582));
#38353=CARTESIAN_POINT('Ctrl Pts',(76.2258010288081,14.6495691638506,-74.0571731429503));
#38354=CARTESIAN_POINT('Ctrl Pts',(76.2256865732654,15.0502504868885,-74.8110671308814));
#38355=CARTESIAN_POINT('Ctrl Pts',(76.2254329300688,15.8533706308797,-76.3186350674606));
#38356=CARTESIAN_POINT('Ctrl Pts',(76.2254675779746,16.5227661783838,-77.571191652404));
#38357=CARTESIAN_POINT('Ctrl Pts',(76.2257326223979,17.4907030767103,-79.3917542575282));
#38358=CARTESIAN_POINT('Ctrl Pts',(76.2256174138935,17.9280458738864,-80.2144133394732));
#38359=CARTESIAN_POINT('Ctrl Pts',(76.2256174138933,18.3645674612764,-81.0353910415709));
#38360=CARTESIAN_POINT('Ctrl Pts',(78.1311761235466,4.88238476433655,24.8296314603199));
#38361=CARTESIAN_POINT('Ctrl Pts',(78.1317586768894,4.88248888926511,24.7807222995813));
#38362=CARTESIAN_POINT('Ctrl Pts',(78.1323693534611,4.882597812653,24.7317992420864));
#38363=CARTESIAN_POINT('Ctrl Pts',(78.1395699941658,4.88389574527485,24.1812167300954));
#38364=CARTESIAN_POINT('Ctrl Pts',(78.1492419926987,4.88177196689673,23.1890789328558));
#38365=CARTESIAN_POINT('Ctrl Pts',(78.1745360446089,4.87447704577674,21.1752495305265));
#38366=CARTESIAN_POINT('Ctrl Pts',(78.2220498596193,4.88324512237042,19.6543634732364));
#38367=CARTESIAN_POINT('Ctrl Pts',(78.301833748746,4.91934107595181,18.3802225175682));
#38368=CARTESIAN_POINT('Ctrl Pts',(78.3395068064966,4.93035400094775,17.9047187002429));
#38369=CARTESIAN_POINT('Ctrl Pts',(78.4321782336654,4.94791260069687,16.9119065524815));
#38370=CARTESIAN_POINT('Ctrl Pts',(78.6275650402547,4.98365588797779,15.1385193904962));
#38371=CARTESIAN_POINT('Ctrl Pts',(78.8098035271563,5.08984219840305,13.5202512022143));
#38372=CARTESIAN_POINT('Ctrl Pts',(78.9141079171548,5.30595926923579,12.1229955240602));
#38373=CARTESIAN_POINT('Ctrl Pts',(78.9585931964819,5.39913427657366,11.5903098623216));
#38374=CARTESIAN_POINT('Ctrl Pts',(79.0492236844176,5.62075197894407,10.5216533462124));
#38375=CARTESIAN_POINT('Ctrl Pts',(79.2018289295449,6.08316796559141,8.68166927386263));
#38376=CARTESIAN_POINT('Ctrl Pts',(79.2830187397639,6.5635051146988,7.13011330676721));
#38377=CARTESIAN_POINT('Ctrl Pts',(79.2878543220827,6.92316409732294,5.96944852000437));
#38378=CARTESIAN_POINT('Ctrl Pts',(79.2829833844745,7.01389849089022,5.68124415713134));
#38379=CARTESIAN_POINT('Ctrl Pts',(79.271246982088,7.20055849904512,5.13353023311153));
#38380=CARTESIAN_POINT('Ctrl Pts',(79.2395720183877,7.54899306029872,4.18865645472214));
#38381=CARTESIAN_POINT('Ctrl Pts',(79.1505282295557,8.27794976463893,2.39178159898726));
#38382=CARTESIAN_POINT('Ctrl Pts',(79.0707071874785,8.82468205108704,0.980148004169901));
#38383=CARTESIAN_POINT('Ctrl Pts',(79.0228181033673,9.05591605411342,0.0730197621118544));
#38384=CARTESIAN_POINT('Ctrl Pts',(79.0149188641117,9.08588408324921,-0.0495289334430407));
#38385=CARTESIAN_POINT('Ctrl Pts',(78.9990824940997,9.14173887775737,-0.286403972854207));
#38386=CARTESIAN_POINT('Ctrl Pts',(78.9680075267001,9.23421719715553,-0.704916603339056));
#38387=CARTESIAN_POINT('Ctrl Pts',(78.9167265681545,9.34909292918604,-1.29979766176164));
#38388=CARTESIAN_POINT('Ctrl Pts',(78.8452750379769,9.46363926693925,-2.01421891223975));
#38389=CARTESIAN_POINT('Ctrl Pts',(78.7408109727822,9.5901340366282,-2.96551438085703));
#38390=CARTESIAN_POINT('Ctrl Pts',(78.5987776215388,9.70979928799303,-4.1543523026218));
#38391=CARTESIAN_POINT('Ctrl Pts',(78.4950284590842,9.78175363508764,-5.10676467868206));
#38392=CARTESIAN_POINT('Ctrl Pts',(78.4416364854941,9.82093138357967,-5.70314228973472));
#38393=CARTESIAN_POINT('Ctrl Pts',(78.4207377850043,9.83260536946596,-5.92375439756827));
#38394=CARTESIAN_POINT('Ctrl Pts',(78.3787158818719,9.84940713990351,-6.38078537880414));
#38395=CARTESIAN_POINT('Ctrl Pts',(78.3063526725102,9.86034267366957,-7.18824108477744));
#38396=CARTESIAN_POINT('Ctrl Pts',(78.2100666718561,9.83680804858785,-8.38360326993399));
#38397=CARTESIAN_POINT('Ctrl Pts',(78.1312684243954,9.79254145045081,-9.62622229216998));
#38398=CARTESIAN_POINT('Ctrl Pts',(78.0885073456006,9.77017076955802,-10.5210983738634));
#38399=CARTESIAN_POINT('Ctrl Pts',(78.0681938151062,9.76286330053317,-11.0392012330339));
#38400=CARTESIAN_POINT('Ctrl Pts',(78.0594902883523,9.76154296606314,-11.3006543404583));
#38401=CARTESIAN_POINT('Ctrl Pts',(78.053513304347,9.76161940798103,-11.4981603609995));
#38402=CARTESIAN_POINT('Ctrl Pts',(78.0498055521674,9.76166010227368,-11.6217338577917));
#38403=CARTESIAN_POINT('Ctrl Pts',(78.0435526389846,9.76183362725649,-11.8737777491659));
#38404=CARTESIAN_POINT('Ctrl Pts',(78.0355232386197,9.76230013096662,-12.3116981948741));
#38405=CARTESIAN_POINT('Ctrl Pts',(78.0282957738844,9.76406912607226,-13.4375530291881));
#38406=CARTESIAN_POINT('Ctrl Pts',(78.0502925386483,9.76693574462966,-14.6828678286821));
#38407=CARTESIAN_POINT('Ctrl Pts',(78.0734323284533,9.76987699356143,-15.933933680242));
#38408=CARTESIAN_POINT('Ctrl Pts',(78.0829751157319,9.77115884436228,-16.561181415999));
#38409=CARTESIAN_POINT('Ctrl Pts',(78.0879251613887,9.77194777263734,-17.064707833481));
#38410=CARTESIAN_POINT('Ctrl Pts',(78.0892795292674,9.77223839921884,-17.3170551029141));
#38411=CARTESIAN_POINT('Ctrl Pts',(78.0897794549923,9.77240971775399,-17.5057890593336));
#38412=CARTESIAN_POINT('Ctrl Pts',(78.0900864923832,9.77251557331494,-17.6302578920605));
#38413=CARTESIAN_POINT('Ctrl Pts',(78.0906091998735,9.77270182264529,-17.879482666526));
#38414=CARTESIAN_POINT('Ctrl Pts',(78.0910077930249,9.77285050784834,-18.1287582169543));
#38415=CARTESIAN_POINT('Ctrl Pts',(78.0912880502502,9.77296669339788,-18.3782285630347));
#38416=CARTESIAN_POINT('Ctrl Pts',(78.0914191479227,9.77302624074914,-18.5341964086388));
#38417=CARTESIAN_POINT('Ctrl Pts',(78.0914982961441,9.77306666014432,-18.6590126540799));
#38418=CARTESIAN_POINT('Ctrl Pts',(78.0915611860204,9.77310237578932,-18.7838528243454));
#38419=CARTESIAN_POINT('Ctrl Pts',(78.0916718013574,9.77318167950402,-19.1272582336073));
#38420=CARTESIAN_POINT('Ctrl Pts',(78.0915282776836,9.77321629682544,-19.6897562128712));
#38421=CARTESIAN_POINT('Ctrl Pts',(78.09065113725,9.77308984641989,-20.6914136827282));
#38422=CARTESIAN_POINT('Ctrl Pts',(78.0889245135217,9.77273623121217,-21.946838300024));
#38423=CARTESIAN_POINT('Ctrl Pts',(78.0880606587,9.77256333897646,-22.9550490867659));
#38424=CARTESIAN_POINT('Ctrl Pts',(78.08803696042,9.77258874259918,-23.5847732614642));
#38425=CARTESIAN_POINT('Ctrl Pts',(78.0880381835476,9.77260043014001,-23.8339776845296));
#38426=CARTESIAN_POINT('Ctrl Pts',(78.0880823882946,9.77262844554538,-24.3332132054465));
#38427=CARTESIAN_POINT('Ctrl Pts',(78.0882514781816,9.772687450661,-25.2086880038889));
#38428=CARTESIAN_POINT('Ctrl Pts',(78.0886614183903,9.77278519551231,-26.4634120692526));
#38429=CARTESIAN_POINT('Ctrl Pts',(78.0891046021519,9.77287286052947,-27.9717324597234));
#38430=CARTESIAN_POINT('Ctrl Pts',(78.0891672773944,9.77287455436938,-28.9764534780923));
#38431=CARTESIAN_POINT('Ctrl Pts',(78.0890753000005,9.77284962231787,-29.5406571996044));
#38432=CARTESIAN_POINT('Ctrl Pts',(78.0890494952249,9.77284294733562,-29.6660260402146));
#38433=CARTESIAN_POINT('Ctrl Pts',(78.0889791775516,9.77282553595872,-29.916825989271));
#38434=CARTESIAN_POINT('Ctrl Pts',(78.0888106525499,9.77278499385702,-30.3558649020516));
#38435=CARTESIAN_POINT('Ctrl Pts',(78.0883206261467,9.77266964692748,-31.2343866557592));
#38436=CARTESIAN_POINT('Ctrl Pts',(78.0875455572616,9.77248571113029,-32.2388424815497));
#38437=CARTESIAN_POINT('Ctrl Pts',(78.0868239127496,9.77230330533085,-33.2426017642358));
#38438=CARTESIAN_POINT('Ctrl Pts',(78.0863765096049,9.77218063491253,-33.994789260345));
#38439=CARTESIAN_POINT('Ctrl Pts',(78.0860914339031,9.7720852698536,-34.7460434515072));
#38440=CARTESIAN_POINT('Ctrl Pts',(78.0860541719157,9.77204885607964,-35.2460753752379));
#38441=CARTESIAN_POINT('Ctrl Pts',(78.0861004458006,9.7720352564668,-35.6217189501983));
#38442=CARTESIAN_POINT('Ctrl Pts',(78.0861554677218,9.77200747680218,-35.8730072441829));
#38443=CARTESIAN_POINT('Ctrl Pts',(78.0863508169533,9.77189287874838,-36.3752036603097));
#38444=CARTESIAN_POINT('Ctrl Pts',(78.0868897252747,9.77157429449981,-37.2527215600665));
#38445=CARTESIAN_POINT('Ctrl Pts',(78.0885304025336,9.77079517197216,-39.0048450922735));
#38446=CARTESIAN_POINT('Ctrl Pts',(78.0901443779921,9.77095535125212,-40.5080843724291));
#38447=CARTESIAN_POINT('Ctrl Pts',(78.0906943772335,9.77259474850997,-41.6416550706781));
#38448=CARTESIAN_POINT('Ctrl Pts',(78.090794629494,9.77279711194888,-41.8895200839283));
#38449=CARTESIAN_POINT('Ctrl Pts',(78.0908902742295,9.77273077332194,-42.2636138715192));
#38450=CARTESIAN_POINT('Ctrl Pts',(78.0909412497351,9.77239247733141,-42.6381564279869));
#38451=CARTESIAN_POINT('Ctrl Pts',(78.0909626971188,9.77171259311439,-43.1389447144232));
#38452=CARTESIAN_POINT('Ctrl Pts',(78.090926616524,9.77068487605055,-43.7668031830724));
#38453=CARTESIAN_POINT('Ctrl Pts',(78.0908600921664,9.7699747402942,-44.522951737293));
#38454=CARTESIAN_POINT('Ctrl Pts',(78.0908490780117,9.77049711716599,-45.1548446218977));
#38455=CARTESIAN_POINT('Ctrl Pts',(78.0909037548587,9.77200020186817,-45.6611662031078));
#38456=CARTESIAN_POINT('Ctrl Pts',(78.0909862434953,9.77377082767171,-46.0412644505658));
#38457=CARTESIAN_POINT('Ctrl Pts',(78.09111952065,9.7762883158246,-46.4216341543253));
#38458=CARTESIAN_POINT('Ctrl Pts',(78.0913765780375,9.78078426265377,-46.9291405658452));
#38459=CARTESIAN_POINT('Ctrl Pts',(78.091674312547,9.78558158784181,-47.3098975341711));
#38460=CARTESIAN_POINT('Ctrl Pts',(78.0920582451879,9.79157417936065,-47.6920584907085));
#38461=CARTESIAN_POINT('Ctrl Pts',(78.092290121104,9.79731540407121,-47.9610555008819));
#38462=CARTESIAN_POINT('Ctrl Pts',(78.0928133460247,9.81361748257627,-48.4858996199633));
#38463=CARTESIAN_POINT('Ctrl Pts',(78.0938693960702,9.85245632736365,-49.3950492918544));
#38464=CARTESIAN_POINT('Ctrl Pts',(78.0960164804529,9.92168060508791,-50.6524468435612));
#38465=CARTESIAN_POINT('Ctrl Pts',(78.0996044526606,9.98194540832576,-52.0996111866457));
#38466=CARTESIAN_POINT('Ctrl Pts',(78.1021962417671,9.98041336536394,-53.0203964617832));
#38467=CARTESIAN_POINT('Ctrl Pts',(78.1035520022358,9.95937927344506,-53.5822721134691));
#38468=CARTESIAN_POINT('Ctrl Pts',(78.1038786353797,9.94811087479182,-53.7812906420223));
#38469=CARTESIAN_POINT('Ctrl Pts',(78.1045393796479,9.91063979260362,-54.2122457592885));
#38470=CARTESIAN_POINT('Ctrl Pts',(78.1059983986141,9.8105113177491,-54.9969674004099));
#38471=CARTESIAN_POINT('Ctrl Pts',(78.1115855487694,9.51488504017041,-56.7184898330074));
#38472=CARTESIAN_POINT('Ctrl Pts',(78.1237628749783,9.26090774064384,-58.4312662472414));
#38473=CARTESIAN_POINT('Ctrl Pts',(78.1237572022669,9.33988962176433,-59.7671397048542));
#38474=CARTESIAN_POINT('Ctrl Pts',(78.1238834968223,9.34940945215823,-59.9089694517362));
#38475=CARTESIAN_POINT('Ctrl Pts',(78.123948344431,9.37303563774044,-60.2030134627939));
#38476=CARTESIAN_POINT('Ctrl Pts',(78.123860278138,9.42416576273053,-60.7092172719043));
#38477=CARTESIAN_POINT('Ctrl Pts',(78.1228007482891,9.56467332005635,-61.7148702192895));
#38478=CARTESIAN_POINT('Ctrl Pts',(78.1202486506339,9.80126886303687,-62.8348983695161));
#38479=CARTESIAN_POINT('Ctrl Pts',(78.1172932387441,10.0940390606951,-63.9270100415927));
#38480=CARTESIAN_POINT('Ctrl Pts',(78.1156185224597,10.2763282371946,-64.529871145115));
#38481=CARTESIAN_POINT('Ctrl Pts',(78.1145527478538,10.4037632125647,-64.9270258697791));
#38482=CARTESIAN_POINT('Ctrl Pts',(78.113859133745,10.4902027451492,-65.1904704743225));
#38483=CARTESIAN_POINT('Ctrl Pts',(78.113191450897,10.5787596618105,-65.4520554270822));
#38484=CARTESIAN_POINT('Ctrl Pts',(78.112643225262,10.6578244912705,-65.6791434672428));
#38485=CARTESIAN_POINT('Ctrl Pts',(78.1123410970943,10.7034232613404,-65.8084000171421));
#38486=CARTESIAN_POINT('Ctrl Pts',(78.1118981045971,10.7722341252842,-66.0018011992152));
#38487=CARTESIAN_POINT('Ctrl Pts',(78.1115561931355,10.8303667975822,-66.1618743965424));
#38488=CARTESIAN_POINT('Ctrl Pts',(78.1109957852442,10.9277418190334,-66.4261277666418));
#38489=CARTESIAN_POINT('Ctrl Pts',(78.1086625472797,11.0450636807174,-66.7305607189423));
#38490=CARTESIAN_POINT('Ctrl Pts',(78.105090688148,11.2870515878708,-67.3072716108154));
#38491=CARTESIAN_POINT('Ctrl Pts',(78.098847683009,11.7461962687019,-68.2955809242267));
#38492=CARTESIAN_POINT('Ctrl Pts',(78.0902779682787,12.747213949018,-70.1535034158577));
#38493=CARTESIAN_POINT('Ctrl Pts',(78.0915595497525,13.6228501821446,-71.6137900374506));
#38494=CARTESIAN_POINT('Ctrl Pts',(78.0969916965239,14.1769255672346,-72.6661684683484));
#38495=CARTESIAN_POINT('Ctrl Pts',(78.0965163028863,14.3125846847232,-72.9238511157893));
#38496=CARTESIAN_POINT('Ctrl Pts',(78.096552461901,14.5774164020563,-73.4254256093465));
#38497=CARTESIAN_POINT('Ctrl Pts',(78.0962319470329,14.9119800013117,-74.0571686214722));
#38498=CARTESIAN_POINT('Ctrl Pts',(78.0961174294113,15.3126614747988,-74.8110629716249));
#38499=CARTESIAN_POINT('Ctrl Pts',(78.0958636910111,16.1157821891972,-76.3186314299804));
#38500=CARTESIAN_POINT('Ctrl Pts',(78.0958984464845,16.7851782478249,-77.5711876351949));
#38501=CARTESIAN_POINT('Ctrl Pts',(78.0961636612281,17.7531146699538,-79.3917492952804));
#38502=CARTESIAN_POINT('Ctrl Pts',(78.0960484086298,18.1904575551487,-80.2144085738345));
#38503=CARTESIAN_POINT('Ctrl Pts',(78.0960484086287,18.6269791425379,-81.035386275933));
#38504=CARTESIAN_POINT('Ctrl Pts',(79.0674174572816,5.01522268798702,24.8190563697355));
#38505=CARTESIAN_POINT('Ctrl Pts',(79.0681671244069,5.01561130574058,24.7698112483116));
#38506=CARTESIAN_POINT('Ctrl Pts',(79.0689526523201,5.01601890898661,24.7205402199319));
#38507=CARTESIAN_POINT('Ctrl Pts',(79.0782204295203,5.02082369775688,24.1661600490855));
#38508=CARTESIAN_POINT('Ctrl Pts',(79.0927100922061,5.02499971059091,23.1752017953721));
#38509=CARTESIAN_POINT('Ctrl Pts',(79.13103764065,5.03563871650282,21.1518987462585));
#38510=CARTESIAN_POINT('Ctrl Pts',(79.1918013249263,5.06857469890096,19.6199983452087));
#38511=CARTESIAN_POINT('Ctrl Pts',(79.2833409011377,5.13810232036442,18.3332047185655));
#38512=CARTESIAN_POINT('Ctrl Pts',(79.3271982411792,5.16402176082393,17.84951198812));
#38513=CARTESIAN_POINT('Ctrl Pts',(79.4350318672687,5.21929330547081,16.8471016897774));
#38514=CARTESIAN_POINT('Ctrl Pts',(79.6597738786907,5.3369308565268,15.0668569726542));
#38515=CARTESIAN_POINT('Ctrl Pts',(79.8528846773185,5.52342816880157,13.4624411336813));
#38516=CARTESIAN_POINT('Ctrl Pts',(79.9478662062515,5.77956862039127,12.0840553932277));
#38517=CARTESIAN_POINT('Ctrl Pts',(79.9872497031577,5.88971864287113,11.549661093268));
#38518=CARTESIAN_POINT('Ctrl Pts',(80.0644577893544,6.14288461106471,10.4849494612428));
#38519=CARTESIAN_POINT('Ctrl Pts',(80.1868739514183,6.65297453317945,8.65255246253285));
#38520=CARTESIAN_POINT('Ctrl Pts',(80.2380434661674,7.1519521376352,7.11347354620467));
#38521=CARTESIAN_POINT('Ctrl Pts',(80.220439279543,7.50474250480026,5.96584701383932));
#38522=CARTESIAN_POINT('Ctrl Pts',(80.2096598301317,7.59336202603015,5.67864593662744));
#38523=CARTESIAN_POINT('Ctrl Pts',(80.1847388141545,7.77373997953912,5.13331455420261));
#38524=CARTESIAN_POINT('Ctrl Pts',(80.1261981063281,8.10627260965177,4.19103989716421));
#38525=CARTESIAN_POINT('Ctrl Pts',(79.9741025993112,8.78915160892049,2.3987733150821));
#38526=CARTESIAN_POINT('Ctrl Pts',(79.8394769089903,9.27574069900803,0.998413564670721));
#38527=CARTESIAN_POINT('Ctrl Pts',(79.776274034096,9.47255577832048,0.106471274813789));
#38528=CARTESIAN_POINT('Ctrl Pts',(79.767194457764,9.49782300197105,-0.0121282343591863));
#38529=CARTESIAN_POINT('Ctrl Pts',(79.7492041230658,9.54449995459902,-0.242617772173818));
#38530=CARTESIAN_POINT('Ctrl Pts',(79.7157700463245,9.62061451730498,-0.650089440549976));
#38531=CARTESIAN_POINT('Ctrl Pts',(79.6641794164148,9.71223552902357,-1.23187976654897));
#38532=CARTESIAN_POINT('Ctrl Pts',(79.5969640703358,9.79990367294021,-1.93470248939131));
#38533=CARTESIAN_POINT('Ctrl Pts',(79.5029917261061,9.89209665672663,-2.87653843532152));
#38534=CARTESIAN_POINT('Ctrl Pts',(79.3825599458077,9.97162214304041,-4.06583657236809));
#38535=CARTESIAN_POINT('Ctrl Pts',(79.2987270860321,10.0151794261321,-5.0329814941378));
#38536=CARTESIAN_POINT('Ctrl Pts',(79.2557147461728,10.0403137244337,-5.64265294304191));
#38537=CARTESIAN_POINT('Ctrl Pts',(79.2392553093125,10.0469381856339,-5.86265292508084));
#38538=CARTESIAN_POINT('Ctrl Pts',(79.2076266893868,10.0536784745051,-6.32229191317324));
#38539=CARTESIAN_POINT('Ctrl Pts',(79.1564991190038,10.0477999042845,-7.13344037568369));
#38540=CARTESIAN_POINT('Ctrl Pts',(79.095707653065,10.0015426863692,-8.3366524324552));
#38541=CARTESIAN_POINT('Ctrl Pts',(79.0509098119789,9.93743938884988,-9.58843116417154));
#38542=CARTESIAN_POINT('Ctrl Pts',(79.0268821972649,9.90337508252064,-10.4912278027067));
#38543=CARTESIAN_POINT('Ctrl Pts',(79.0150755982232,9.89016064836555,-11.0141123219708));
#38544=CARTESIAN_POINT('Ctrl Pts',(79.0097798694179,9.88618613227508,-11.2780557604261));
#38545=CARTESIAN_POINT('Ctrl Pts',(79.0060078185597,9.88439984881659,-11.4774995193815));
#38546=CARTESIAN_POINT('Ctrl Pts',(79.0036646128689,9.88335806765953,-11.603394679048));
#38547=CARTESIAN_POINT('Ctrl Pts',(78.9997403997698,9.8816487714516,-11.8592855259742));
#38548=CARTESIAN_POINT('Ctrl Pts',(78.994761626747,9.87966497487754,-12.3037147241161));
#38549=CARTESIAN_POINT('Ctrl Pts',(78.9906389493915,9.87901407437311,-13.4432992897924));
#38550=CARTESIAN_POINT('Ctrl Pts',(79.0055392688548,9.88809053067284,-14.6957989256028));
#38551=CARTESIAN_POINT('Ctrl Pts',(79.0211129616261,9.89743196753811,-15.9454740289875));
#38552=CARTESIAN_POINT('Ctrl Pts',(79.0275063270077,9.90133064832979,-16.5699512103482));
#38553=CARTESIAN_POINT('Ctrl Pts',(79.0308470126228,9.90348293817318,-17.0700172850903));
#38554=CARTESIAN_POINT('Ctrl Pts',(79.0317705160842,9.90415023660917,-17.3202164927592));
#38555=CARTESIAN_POINT('Ctrl Pts',(79.0321228819547,9.90446515454591,-17.5072310492657));
#38556=CARTESIAN_POINT('Ctrl Pts',(79.032337739374,9.90466298605188,-17.6318736294089));
#38557=CARTESIAN_POINT('Ctrl Pts',(79.0326993816342,9.90501330195036,-17.8806948601256));
#38558=CARTESIAN_POINT('Ctrl Pts',(79.0329642770318,9.90529960964907,-18.1298687430497));
#38559=CARTESIAN_POINT('Ctrl Pts',(79.0331427080346,9.90552884765909,-18.3791056551831));
#38560=CARTESIAN_POINT('Ctrl Pts',(79.0332205008359,9.9056495194714,-18.5349686115737));
#38561=CARTESIAN_POINT('Ctrl Pts',(79.033263780692,9.90573338983648,-18.6596927967284));
#38562=CARTESIAN_POINT('Ctrl Pts',(79.0332948783198,9.90580906228168,-18.7844474542172));
#38563=CARTESIAN_POINT('Ctrl Pts',(79.0333320742632,9.90598416472866,-19.1276271552783));
#38564=CARTESIAN_POINT('Ctrl Pts',(79.0331487356763,9.90610415692518,-19.6898219896876));
#38565=CARTESIAN_POINT('Ctrl Pts',(79.0323543044741,9.90598184028357,-20.691124554094));
#38566=CARTESIAN_POINT('Ctrl Pts',(79.0309053714312,9.90546300842679,-21.946441629422));
#38567=CARTESIAN_POINT('Ctrl Pts',(79.0301633435523,9.90521302908391,-22.9549301710126));
#38568=CARTESIAN_POINT('Ctrl Pts',(79.0301115641125,9.90528387188766,-23.5849311300825));
#38569=CARTESIAN_POINT('Ctrl Pts',(79.0301019745384,9.90531313413815,-23.8340998784275));
#38570=CARTESIAN_POINT('Ctrl Pts',(79.0301210191317,9.90537475774982,-24.33334418637));
#38571=CARTESIAN_POINT('Ctrl Pts',(79.0302400236347,9.90548755710516,-25.2087899692583));
#38572=CARTESIAN_POINT('Ctrl Pts',(79.0305714553795,9.90564282039012,-26.4634885417697));
#38573=CARTESIAN_POINT('Ctrl Pts',(79.030959298768,9.9057612371249,-27.9717423758669));
#38574=CARTESIAN_POINT('Ctrl Pts',(79.0310334197768,9.90575228243049,-28.9764101349445));
#38575=CARTESIAN_POINT('Ctrl Pts',(79.0309728668496,9.90571199706992,-29.5405779896386));
#38576=CARTESIAN_POINT('Ctrl Pts',(79.0309554746975,9.90570156829581,-29.6659328551748));
#38577=CARTESIAN_POINT('Ctrl Pts',(79.0309061139083,9.9056748904435,-29.9167097801928));
#38578=CARTESIAN_POINT('Ctrl Pts',(79.0307843866883,9.90561375846606,-30.3557101966999));
#38579=CARTESIAN_POINT('Ctrl Pts',(79.0304226216911,9.90544194556123,-31.2341706187796));
#38580=CARTESIAN_POINT('Ctrl Pts',(79.0298448496468,9.90516647822444,-32.2385881454819));
#38581=CARTESIAN_POINT('Ctrl Pts',(79.0293143868082,9.9048833276159,-33.2423420552038));
#38582=CARTESIAN_POINT('Ctrl Pts',(79.0289931241137,9.90468470258017,-33.9945417556105));
#38583=CARTESIAN_POINT('Ctrl Pts',(79.0288015672039,9.9045163686194,-34.7458244523766));
#38584=CARTESIAN_POINT('Ctrl Pts',(79.0287955792199,9.90443623244035,-35.2458865329308));
#38585=CARTESIAN_POINT('Ctrl Pts',(79.0288500605975,9.90439277023724,-35.621556387038));
#38586=CARTESIAN_POINT('Ctrl Pts',(79.0289061929832,9.90434466294553,-35.8728434775819));
#38587=CARTESIAN_POINT('Ctrl Pts',(79.0290881140862,9.90418857142105,-36.3750481798328));
#38588=CARTESIAN_POINT('Ctrl Pts',(79.0295670331225,9.90379457777519,-37.2525756951283));
#38589=CARTESIAN_POINT('Ctrl Pts',(79.030981405081,9.90286410656558,-39.004723044727));
#38590=CARTESIAN_POINT('Ctrl Pts',(79.0323520207929,9.90290731861339,-40.5079837794954));
#38591=CARTESIAN_POINT('Ctrl Pts',(79.032828231492,9.90448791210333,-41.6415712959431));
#38592=CARTESIAN_POINT('Ctrl Pts',(79.0329157952561,9.90467835555726,-41.889438042092));
#38593=CARTESIAN_POINT('Ctrl Pts',(79.0330014944524,9.90459583103868,-42.2635358201197));
#38594=CARTESIAN_POINT('Ctrl Pts',(79.033049886041,9.90424312054807,-42.6380823835159));
#38595=CARTESIAN_POINT('Ctrl Pts',(79.0330754060422,9.903546008436,-43.1388767358232));
#38596=CARTESIAN_POINT('Ctrl Pts',(79.0330542033092,9.90250021442703,-43.7667436590274));
#38597=CARTESIAN_POINT('Ctrl Pts',(79.0330074024399,9.90177258117173,-44.5229039801225));
#38598=CARTESIAN_POINT('Ctrl Pts',(79.0330028838391,9.90228279501689,-45.1548080060181));
#38599=CARTESIAN_POINT('Ctrl Pts',(79.0330499122594,9.90377720905201,-45.661139141396));
#38600=CARTESIAN_POINT('Ctrl Pts',(79.0331185088012,9.90554159635451,-46.0412449734253));
#38601=CARTESIAN_POINT('Ctrl Pts',(79.0332280130535,9.90805298035099,-46.4216226721918));
#38602=CARTESIAN_POINT('Ctrl Pts',(79.0334379143621,9.91254077080098,-46.9291402370918));
#38603=CARTESIAN_POINT('Ctrl Pts',(79.0336802549664,9.91733169902102,-47.3099063411047));
#38604=CARTESIAN_POINT('Ctrl Pts',(79.0339918692555,9.92331741644185,-47.6920768194761));
#38605=CARTESIAN_POINT('Ctrl Pts',(79.0341721220784,9.92905466802767,-47.9610826352538));
#38606=CARTESIAN_POINT('Ctrl Pts',(79.0345801987364,9.94535040630575,-48.4859414577754));
#38607=CARTESIAN_POINT('Ctrl Pts',(79.0354045483133,9.98418152818373,-49.3951141830985));
#38608=CARTESIAN_POINT('Ctrl Pts',(79.0371404675913,10.0534000779738,-50.6525346834891));
#38609=CARTESIAN_POINT('Ctrl Pts',(79.0401258992488,10.1136512244723,-52.0997107596071));
#38610=CARTESIAN_POINT('Ctrl Pts',(79.0422538093688,10.1120991412615,-53.0204920363285));
#38611=CARTESIAN_POINT('Ctrl Pts',(79.0433031166023,10.0910468013029,-53.5823614482346));
#38612=CARTESIAN_POINT('Ctrl Pts',(79.0434978739722,10.079768538197,-53.7813889810288));
#38613=CARTESIAN_POINT('Ctrl Pts',(79.0438666169688,10.0422768550406,-54.2123523928334));
#38614=CARTESIAN_POINT('Ctrl Pts',(79.0447526255036,9.94210926415323,-54.9970852213269));
#38615=CARTESIAN_POINT('Ctrl Pts',(79.0490442932728,9.64640230422955,-56.7186062684982));
#38616=CARTESIAN_POINT('Ctrl Pts',(79.0601752091258,9.39237855590308,-58.4313538317651));
#38617=CARTESIAN_POINT('Ctrl Pts',(79.059765077974,9.47133310933444,-59.7671833796691));
#38618=CARTESIAN_POINT('Ctrl Pts',(79.059844272936,9.48084906648494,-59.9090085147957));
#38619=CARTESIAN_POINT('Ctrl Pts',(79.0598220382771,9.50446771414443,-60.2030434561234));
#38620=CARTESIAN_POINT('Ctrl Pts',(79.0595996895095,9.55558442298195,-60.7092328461023));
#38621=CARTESIAN_POINT('Ctrl Pts',(79.0583373808453,9.69606534726421,-61.714862060537));
#38622=CARTESIAN_POINT('Ctrl Pts',(79.0556740185159,9.9326329152352,-62.8348748135544));
#38623=CARTESIAN_POINT('Ctrl Pts',(79.0526682675542,10.2253806864803,-63.9269816045994));
#38624=CARTESIAN_POINT('Ctrl Pts',(79.0509770368797,10.4076596115538,-64.5298437088795));
#38625=CARTESIAN_POINT('Ctrl Pts',(79.0499005595451,10.535088907577,-64.9270005875088));
#38626=CARTESIAN_POINT('Ctrl Pts',(79.0491995939402,10.6215249556936,-65.1904470301732));
#38627=CARTESIAN_POINT('Ctrl Pts',(79.0485237590337,10.7100788792758,-65.452034393878));
#38628=CARTESIAN_POINT('Ctrl Pts',(79.0479669167474,10.7891415145841,-65.6791250682007));
#38629=CARTESIAN_POINT('Ctrl Pts',(79.0476593247898,10.834739158003,-65.8083832713257));
#38630=CARTESIAN_POINT('Ctrl Pts',(79.0472075401805,10.9035484565487,-66.001787077094));
#38631=CARTESIAN_POINT('Ctrl Pts',(79.0468569356967,10.9616801042072,-66.1618627777127));
#38632=CARTESIAN_POINT('Ctrl Pts',(79.0462796991508,11.0590537418934,-66.4261205988185));
#38633=CARTESIAN_POINT('Ctrl Pts',(79.0439307937972,11.1763722519809,-66.7305525790236));
#38634=CARTESIAN_POINT('Ctrl Pts',(79.0403355509136,11.4183560689343,-67.3072646265125));
#38635=CARTESIAN_POINT('Ctrl Pts',(79.0340698029988,11.8774960798622,-68.2955742231883));
#38636=CARTESIAN_POINT('Ctrl Pts',(79.0255118814883,12.8785147036822,-70.1534980894638));
#38637=CARTESIAN_POINT('Ctrl Pts',(79.0268453569621,13.7541586521472,-71.6137842112993));
#38638=CARTESIAN_POINT('Ctrl Pts',(79.0322798354967,14.3082341286308,-72.6661621416571));
#38639=CARTESIAN_POINT('Ctrl Pts',(79.0318042672112,14.4438931804177,-72.923844899657));
#38640=CARTESIAN_POINT('Ctrl Pts',(79.0318404699244,14.7087248514462,-73.4254194789814));
#38641=CARTESIAN_POINT('Ctrl Pts',(79.0315198355751,15.043288421734,-74.0571626126466));
#38642=CARTESIAN_POINT('Ctrl Pts',(79.0314052642792,15.4439699314055,-74.8110570612082));
#38643=CARTESIAN_POINT('Ctrl Pts',(79.0311513756816,16.2470907856448,-76.3186256622214));
#38644=CARTESIAN_POINT('Ctrl Pts',(79.031186060788,16.9164870242636,-77.5711817648655));
#38645=CARTESIAN_POINT('Ctrl Pts',(79.0314513893355,17.8844233649719,-79.3917431632681));
#38646=CARTESIAN_POINT('Ctrl Pts',(79.0313360800254,18.3217662758759,-80.2144024928222));
#38647=CARTESIAN_POINT('Ctrl Pts',(79.0313360800244,18.7582878632648,-81.0353801949212));
#38648=CARTESIAN_POINT('',(6.0874749758614E-15,-1.93207323326078,-8.62957429809281));
#38649=CARTESIAN_POINT('',(-11.7470010949101,-1.24897189262896,-5.16040757324739));
#38650=CARTESIAN_POINT('Ctrl Pts',(6.41902973990636E-15,-1.93207323326078,
-8.62957429809281));
#38651=CARTESIAN_POINT('Ctrl Pts',(-0.658062683030888,-1.93165972294369,
-8.58745240866785));
#38652=CARTESIAN_POINT('Ctrl Pts',(-2.46516391286739,-1.98743098295203,
-8.49849688064982));
#38653=CARTESIAN_POINT('Ctrl Pts',(-4.39676963179061,-2.13852225314529,
-8.46329578588585));
#38654=CARTESIAN_POINT('Ctrl Pts',(-6.35409454450772,-2.18205385875907,
-8.11784826271868));
#38655=CARTESIAN_POINT('Ctrl Pts',(-8.15537660210863,-2.1050270665009,-7.52858105609529));
#38656=CARTESIAN_POINT('Ctrl Pts',(-10.2097165609597,-1.7375710793364,-6.40958181990177));
#38657=CARTESIAN_POINT('Ctrl Pts',(-11.2781006865412,-1.40420632664524,
-5.56975094644535));
#38658=CARTESIAN_POINT('Ctrl Pts',(-11.7470010949101,-1.24897189262896,
-5.16040757324739));
#38659=CARTESIAN_POINT('',(-16.6859947282585,-0.000213685071574765,0.653010349651234));
#38660=CARTESIAN_POINT('Ctrl Pts',(-11.7470010949101,-1.24897189262896,
-5.16040757324739));
#38661=CARTESIAN_POINT('Ctrl Pts',(-12.0051227941173,-1.16133413061408,
-4.91749318228553));
#38662=CARTESIAN_POINT('Ctrl Pts',(-12.7010876741305,-0.905923104279308,
-4.23327664549238));
#38663=CARTESIAN_POINT('Ctrl Pts',(-13.4034560583173,-0.630382964431516,
-3.47895409086386));
#38664=CARTESIAN_POINT('Ctrl Pts',(-14.2693062595799,-0.346358717812154,
-2.463047534852));
#38665=CARTESIAN_POINT('Ctrl Pts',(-14.9655514589865,-0.169147364522696,
-1.59527625944176));
#38666=CARTESIAN_POINT('Ctrl Pts',(-15.802459484106,-0.0396258388242596,
-0.512753421506671));
#38667=CARTESIAN_POINT('Ctrl Pts',(-16.3914046039635,-0.0079781652302746,
0.264045566458043));
#38668=CARTESIAN_POINT('Ctrl Pts',(-16.6859947282585,-0.000213685071574765,
0.653010349651234));
#38669=CARTESIAN_POINT('',(-21.1430614769936,0.000756295652328289,6.63001173744468));
#38670=CARTESIAN_POINT('Ctrl Pts',(-16.6863334278776,-0.000204653071346932,
0.653462911021818));
#38671=CARTESIAN_POINT('Ctrl Pts',(-16.8118521335206,0.00314150838095653,
0.821178522657258));
#38672=CARTESIAN_POINT('Ctrl Pts',(-16.937649788032,0.00537544180921331,
0.990238755444057));
#38673=CARTESIAN_POINT('Ctrl Pts',(-17.0633706860534,0.0068090556350368,
1.15985916130958));
#38674=CARTESIAN_POINT('Ctrl Pts',(-17.1804382136137,0.00814399380925252,
1.31780459322238));
#38675=CARTESIAN_POINT('Ctrl Pts',(-17.2974387804625,0.00878473931917982,
1.47623543730744));
#38676=CARTESIAN_POINT('Ctrl Pts',(-17.4141122266992,0.0089781522474648,
1.63455929336058));
#38677=CARTESIAN_POINT('Ctrl Pts',(-17.5138264956263,0.00914345145964242,
1.76986983804117));
#38678=CARTESIAN_POINT('Ctrl Pts',(-17.6133042468771,0.00898183853621348,
1.90510568704074));
#38679=CARTESIAN_POINT('Ctrl Pts',(-17.7124025646993,0.00864633652358228,
2.03992407930371));
#38680=CARTESIAN_POINT('Ctrl Pts',(-17.7724114264697,0.008443173701628,
2.1215631872443));
#38681=CARTESIAN_POINT('Ctrl Pts',(-17.8322823536763,0.00817623153716935,
2.20305085372838));
#38682=CARTESIAN_POINT('Ctrl Pts',(-17.8919878634841,0.00787965725593698,
2.28431647094987));
#38683=CARTESIAN_POINT('Ctrl Pts',(-17.9273873601848,0.00770381786818521,
2.33249899142373));
#38684=CARTESIAN_POINT('Ctrl Pts',(-17.962728014113,0.00751757003612775,
2.38060250534804));
#38685=CARTESIAN_POINT('Ctrl Pts',(-17.9980083677065,0.00732807539521961,
2.42861802646074));
#38686=CARTESIAN_POINT('Ctrl Pts',(-18.001488971058,0.00730938069363454,
2.43335502500778));
#38687=CARTESIAN_POINT('Ctrl Pts',(-18.0049689406119,0.00729065469608626,
2.43809110323027));
#38688=CARTESIAN_POINT('Ctrl Pts',(-18.0084482439713,0.00727190448674141,
2.4428262102729));
#38689=CARTESIAN_POINT('Ctrl Pts',(-18.0356067319927,0.00712554549378024,
2.47978715751235));
#38690=CARTESIAN_POINT('Ctrl Pts',(-18.0627246109005,0.00697771079836186,
2.51668890611163));
#38691=CARTESIAN_POINT('Ctrl Pts',(-18.0898011533159,0.0068289269468095,
2.5535288181166));
#38692=CARTESIAN_POINT('Ctrl Pts',(-18.1068160814727,0.00673543101567395,
2.57667905814547));
#38693=CARTESIAN_POINT('Ctrl Pts',(-18.1238146910947,0.00664156041842843,
2.59980488613449));
#38694=CARTESIAN_POINT('Ctrl Pts',(-18.1407968393983,0.00654744676484664,
2.62290570083462));
#38695=CARTESIAN_POINT('Ctrl Pts',(-18.1552563546868,0.00646731333363974,
2.64257497808765));
#38696=CARTESIAN_POINT('Ctrl Pts',(-18.1697062080985,0.00638699100024018,
2.6622292107353));
#38697=CARTESIAN_POINT('Ctrl Pts',(-18.1841315126729,0.0063066438702019,
2.68184790502516));
#38698=CARTESIAN_POINT('Ctrl Pts',(-18.2628094149958,0.0058684178614192,
2.78885137972402));
#38699=CARTESIAN_POINT('Ctrl Pts',(-18.3408481744454,0.00542899616870739,
2.89492157878975));
#38700=CARTESIAN_POINT('Ctrl Pts',(-18.4185857226721,0.00499942937006533,
3.00047974395752));
#38701=CARTESIAN_POINT('Ctrl Pts',(-18.4582257304868,0.00478038424137877,
3.05430606839922));
#38702=CARTESIAN_POINT('Ctrl Pts',(-18.4977862541486,0.00456389907576071,
3.10799768886104));
#38703=CARTESIAN_POINT('Ctrl Pts',(-18.5373111419189,0.00435140300386188,
3.16160920698918));
#38704=CARTESIAN_POINT('Ctrl Pts',(-18.5752980418245,0.0041471755545533,
3.21313459992012));
#38705=CARTESIAN_POINT('Ctrl Pts',(-18.6132539759574,0.00394662084038625,
3.26458865570651));
#38706=CARTESIAN_POINT('Ctrl Pts',(-18.651225173531,0.00375096160359643,
3.3160297059887));
#38707=CARTESIAN_POINT('Ctrl Pts',(-18.6968885985567,0.00351566560398003,
3.37789171437661));
#38708=CARTESIAN_POINT('Ctrl Pts',(-18.7425740592339,0.00328744702494928,
3.43973487390792));
#38709=CARTESIAN_POINT('Ctrl Pts',(-18.7883405339597,0.00306792151733238,
3.50163208321023));
#38710=CARTESIAN_POINT('Ctrl Pts',(-18.8311081784255,0.00286278033227939,
3.55947350221248));
#38711=CARTESIAN_POINT('Ctrl Pts',(-18.873948318386,0.00266521867923928,
3.61736450244666));
#38712=CARTESIAN_POINT('Ctrl Pts',(-18.9169244512462,0.00247653826503431,
3.67538501492457));
#38713=CARTESIAN_POINT('Ctrl Pts',(-18.9454700021879,0.00235121320628823,
3.713923324083));
#38714=CARTESIAN_POINT('Ctrl Pts',(-18.9740766062369,0.00222980450534266,
3.75252018088541));
#38715=CARTESIAN_POINT('Ctrl Pts',(-19.002750377202,0.00211276369809768,
3.79118206185684));
#38716=CARTESIAN_POINT('Ctrl Pts',(-19.0918166419762,0.0017492123695992,
3.91127332336012));
#38717=CARTESIAN_POINT('Ctrl Pts',(-19.1815578127268,0.00142743926558962,
4.03202941632129));
#38718=CARTESIAN_POINT('Ctrl Pts',(-19.2726875642447,0.00116042555726567,
4.15435173614995));
#38719=CARTESIAN_POINT('Ctrl Pts',(-19.2813816998375,0.00113495140259462,
4.16602176505818));
#38720=CARTESIAN_POINT('Ctrl Pts',(-19.2900885036145,0.00110997811710799,
4.17770607709459));
#38721=CARTESIAN_POINT('Ctrl Pts',(-19.2988086153749,0.0010855186267792,
4.18940547392399));
#38722=CARTESIAN_POINT('Ctrl Pts',(-19.3208152543193,0.0010237910724514,
4.21893082967267));
#38723=CARTESIAN_POINT('Ctrl Pts',(-19.3429066761686,0.000965335607998434,
4.24855229564063));
#38724=CARTESIAN_POINT('Ctrl Pts',(-19.3650764005361,0.000910020328793069,
4.27826132650726));
#38725=CARTESIAN_POINT('Ctrl Pts',(-19.3762575288259,0.00088212249736634,
4.2932448454712));
#38726=CARTESIAN_POINT('Ctrl Pts',(-19.3874585697425,0.000855023480585796,
4.30825063094925));
#38727=CARTESIAN_POINT('Ctrl Pts',(-19.3986786603822,0.000828706764082194,
4.32327754097334));
#38728=CARTESIAN_POINT('Ctrl Pts',(-19.4053571075269,0.00081304246993035,
4.33222189156429));
#38729=CARTESIAN_POINT('Ctrl Pts',(-19.4120423033525,0.000797655341410091,
4.34117372573289));
#38730=CARTESIAN_POINT('Ctrl Pts',(-19.4187340617144,0.000782541935546666,
4.35013279669144));
#38731=CARTESIAN_POINT('Ctrl Pts',(-19.4232484622159,0.00077234611505843,
4.35617677381085));
#38732=CARTESIAN_POINT('Ctrl Pts',(-19.4277598943644,0.000762288330701381,
4.36221607166435));
#38733=CARTESIAN_POINT('Ctrl Pts',(-19.4322675941183,0.000752368019598222,
4.36824967400285));
#38734=CARTESIAN_POINT('Ctrl Pts',(-19.4992389541811,0.000604980934588682,
4.45789152611113));
#38735=CARTESIAN_POINT('Ctrl Pts',(-19.5654385820019,0.00048765834225139,
4.54634670309566));
#38736=CARTESIAN_POINT('Ctrl Pts',(-19.6309044885807,0.000393902767859228,
4.63368322649588));
#38737=CARTESIAN_POINT('Ctrl Pts',(-19.6958323846366,0.00030091769353715,
4.72030200273454));
#38738=CARTESIAN_POINT('Ctrl Pts',(-19.760041586352,0.000231152537014414,
4.80582437353299));
#38739=CARTESIAN_POINT('Ctrl Pts',(-19.8235857619775,0.000179736863706651,
4.89033133041942));
#38740=CARTESIAN_POINT('Ctrl Pts',(-19.8670360901756,0.000144579780342639,
4.94811561946853));
#38741=CARTESIAN_POINT('Ctrl Pts',(-19.9101845732443,0.000118027126229189,
5.00543706756955));
#38742=CARTESIAN_POINT('Ctrl Pts',(-19.9530232955811,9.96610527972666E-5,
5.06228647275008));
#38743=CARTESIAN_POINT('Ctrl Pts',(-19.9690367114538,9.27956853033225E-5,
5.08353718046521));
#38744=CARTESIAN_POINT('Ctrl Pts',(-19.9850067567005,8.70756546104475E-5,
5.10472180088031));
#38745=CARTESIAN_POINT('Ctrl Pts',(-20.0009402615093,8.24965293587667E-5,
5.12584969761139));
#38746=CARTESIAN_POINT('Ctrl Pts',(-20.0882904962193,5.73929711453812E-5,
5.24167648905154));
#38747=CARTESIAN_POINT('Ctrl Pts',(-20.1744301620068,6.74023279539181E-5,
5.35564896659735));
#38748=CARTESIAN_POINT('Ctrl Pts',(-20.2594797574646,9.87670179380714E-5,
5.46798070174529));
#38749=CARTESIAN_POINT('Ctrl Pts',(-20.3187694951726,0.000120631957241371,
5.54628935303708));
#38750=CARTESIAN_POINT('Ctrl Pts',(-20.3775302368743,0.000152856878649054,
5.62380177343142));
#38751=CARTESIAN_POINT('Ctrl Pts',(-20.4358109975843,0.000190598969018732,
5.70060256600532));
#38752=CARTESIAN_POINT('Ctrl Pts',(-20.4813036494772,0.000220059596470905,
5.76055153851536));
#38753=CARTESIAN_POINT('Ctrl Pts',(-20.5265022303766,0.000253020880174828,
5.82006480704543));
#38754=CARTESIAN_POINT('Ctrl Pts',(-20.5714278548838,0.000287990739945883,
5.87918011463099));
#38755=CARTESIAN_POINT('Ctrl Pts',(-20.6679178821708,0.00036309804809229,
6.00614635504664));
#38756=CARTESIAN_POINT('Ctrl Pts',(-20.7631498007969,0.000447248524295111,
6.13127798052428));
#38757=CARTESIAN_POINT('Ctrl Pts',(-20.8573180070559,0.00052811713989227,
6.25493296623428));
#38758=CARTESIAN_POINT('Ctrl Pts',(-20.9389114498876,0.000598186954596536,
6.36207566766404));
#38759=CARTESIAN_POINT('Ctrl Pts',(-21.0197031680878,0.000665846435185652,
6.46810590314616));
#38760=CARTESIAN_POINT('Ctrl Pts',(-21.0998834016831,0.000725144819930417,
6.57334051556745));
#38761=CARTESIAN_POINT('Ctrl Pts',(-21.1142981099604,0.000735805413933246,
6.59225947066038));
#38762=CARTESIAN_POINT('Ctrl Pts',(-21.1286931164174,0.000746200536834672,
6.61115278824243));
#38763=CARTESIAN_POINT('Ctrl Pts',(-21.1430614769885,0.00075629653388815,
6.63001173743882));
#38764=CARTESIAN_POINT('',(-25.4512489408135,0.000583306484460569,12.6480025703979));
#38765=CARTESIAN_POINT('Ctrl Pts',(-21.1430614769933,0.000756296099460927,
6.63001173744467));
#38766=CARTESIAN_POINT('Ctrl Pts',(-21.5124085805419,0.00101581966494258,
7.11527647647093));
#38767=CARTESIAN_POINT('Ctrl Pts',(-21.9044241285154,0.00128152445976316,
7.62953628224353));
#38768=CARTESIAN_POINT('Ctrl Pts',(-22.6640844355056,0.00168268680946039,
8.64319916298904));
#38769=CARTESIAN_POINT('Ctrl Pts',(-23.0167102203234,0.00181865873821434,
9.12236041343943));
#38770=CARTESIAN_POINT('Ctrl Pts',(-23.7317035063752,0.00188587826873779,
10.1199883360218));
#38771=CARTESIAN_POINT('Ctrl Pts',(-24.0922922523239,0.00182192529464304,
10.6334016822487));
#38772=CARTESIAN_POINT('Ctrl Pts',(-24.7917978700544,0.0013940595563037,
11.6565878432607));
#38773=CARTESIAN_POINT('Ctrl Pts',(-25.1830186836289,0.000952760036780517,
12.2452305023429));
#38774=CARTESIAN_POINT('Ctrl Pts',(-25.4512489408144,0.000583307123841907,
12.6480025703979));
#38775=CARTESIAN_POINT('',(-30.3222847657765,-0.00413284663027091,18.6660068644689));
#38776=CARTESIAN_POINT('Ctrl Pts',(-25.4512489408144,0.000583307123841869,
12.6480025703979));
#38777=CARTESIAN_POINT('Ctrl Pts',(-26.2375266602302,-0.000499689987680418,
13.8286704081032));
#38778=CARTESIAN_POINT('Ctrl Pts',(-26.9256080520826,-0.00206137009404955,
14.8637894175972));
#38779=CARTESIAN_POINT('Ctrl Pts',(-28.5066600268001,-0.0048491048562661,
16.9014277594712));
#38780=CARTESIAN_POINT('Ctrl Pts',(-29.3327715286854,-0.00627370115692009,
17.789618484765));
#38781=CARTESIAN_POINT('Ctrl Pts',(-30.3222847382684,-0.00412017247110571,
18.6660068643839));
#38782=CARTESIAN_POINT('',(-44.3052665433893,0.50176463722647,24.6839663391592));
#38783=CARTESIAN_POINT('Ctrl Pts',(-30.3222847657765,-0.00413284663027091,
18.6660068644689));
#38784=CARTESIAN_POINT('Ctrl Pts',(-30.7285587386581,-0.00325138912786291,
19.0258393291216));
#38785=CARTESIAN_POINT('Ctrl Pts',(-31.3846390634535,-0.00108090020159251,
19.5676919050105));
#38786=CARTESIAN_POINT('Ctrl Pts',(-32.4133598840372,0.00689348995379523,
20.3244421620242));
#38787=CARTESIAN_POINT('Ctrl Pts',(-34.9086113550027,0.0335760566375183,
22.0306340145341));
#38788=CARTESIAN_POINT('Ctrl Pts',(-37.6978937468501,0.11693363945437,23.2888479293169));
#38789=CARTESIAN_POINT('Ctrl Pts',(-39.7806058664349,0.216865324193402,
23.8826917702588));
#38790=CARTESIAN_POINT('Ctrl Pts',(-40.597421702395,0.259993271724183,24.084560939485));
#38791=CARTESIAN_POINT('Ctrl Pts',(-41.4486629431555,0.307991395735675,
24.2719159198737));
#38792=CARTESIAN_POINT('Ctrl Pts',(-42.6707056826778,0.383592726711738,
24.4939878032503));
#38793=CARTESIAN_POINT('Ctrl Pts',(-43.7457382365382,0.459542695930701,
24.6297413546134));
#38794=CARTESIAN_POINT('Ctrl Pts',(-44.3052665433893,0.501764637226471,
24.6839663391592));
#38795=CARTESIAN_POINT('',(-49.3675963148847,0.956500242243167,24.6840252060176));
#38796=CARTESIAN_POINT('Ctrl Pts',(-44.3052665433893,0.501764637226471,
24.6839663391592));
#38797=CARTESIAN_POINT('Ctrl Pts',(-45.8824543200059,0.620779044324047,
24.8368171284471));
#38798=CARTESIAN_POINT('Ctrl Pts',(-47.6223636079185,0.774187094160568,
24.8731447167143));
#38799=CARTESIAN_POINT('Ctrl Pts',(-49.3675963149307,0.956500241803143,
24.6840252060176));
#38800=CARTESIAN_POINT('',(-61.5166608776679,2.54670163095537,18.6669577173835));
#38801=CARTESIAN_POINT('Ctrl Pts',(-49.3675963149307,0.956500241803143,
24.6840252060176));
#38802=CARTESIAN_POINT('Ctrl Pts',(-50.8584101085268,1.11223589479094,24.5224746204595));
#38803=CARTESIAN_POINT('Ctrl Pts',(-53.5751452720453,1.43410480188598,23.9491047084121));
#38804=CARTESIAN_POINT('Ctrl Pts',(-56.685826170517,1.86305916206279,22.9608139368193));
#38805=CARTESIAN_POINT('Ctrl Pts',(-58.1934501574325,2.0765014749507,22.2614053479118));
#38806=CARTESIAN_POINT('Ctrl Pts',(-59.4665491367357,2.25831996402558,21.3906391167669));
#38807=CARTESIAN_POINT('Ctrl Pts',(-60.5958520140507,2.41846826761656,20.1757428158229));
#38808=CARTESIAN_POINT('Ctrl Pts',(-61.2120138672132,2.50451285269251,19.2030902538488));
#38809=CARTESIAN_POINT('Ctrl Pts',(-61.5166608776679,2.54670163095537,18.6669577173835));
#38810=CARTESIAN_POINT('',(-64.4551411469067,2.94895124118343,12.643128511615));
#38811=CARTESIAN_POINT('Ctrl Pts',(-61.5166579557216,2.54672260023573,18.6669577083775));
#38812=CARTESIAN_POINT('Ctrl Pts',(-61.9449589659908,2.60609546337214,17.9143482600221));
#38813=CARTESIAN_POINT('Ctrl Pts',(-62.3851009475059,2.66495993045432,17.0249620269639));
#38814=CARTESIAN_POINT('Ctrl Pts',(-63.2835028538324,2.78486870373281,15.1472982754152));
#38815=CARTESIAN_POINT('Ctrl Pts',(-63.5467635706412,2.82032508158459,14.5938134505021));
#38816=CARTESIAN_POINT('Ctrl Pts',(-64.0017146934209,2.88329552572288,13.6289746707392));
#38817=CARTESIAN_POINT('Ctrl Pts',(-64.2299173026253,2.91581081465848,13.1396374113502));
#38818=CARTESIAN_POINT('Ctrl Pts',(-64.4551318427595,2.94901660708818,12.6431286647104));
#38819=CARTESIAN_POINT('',(-66.7632425918307,3.2720446654144,6.633020912074));
#38820=CARTESIAN_POINT('Ctrl Pts',(-64.4551411469067,2.94895124118343,12.643128511615));
#38821=CARTESIAN_POINT('Ctrl Pts',(-64.8619798876637,3.00903884605696,11.7454668071155));
#38822=CARTESIAN_POINT('Ctrl Pts',(-65.505440000895,3.11095649481449,10.2498012385406));
#38823=CARTESIAN_POINT('Ctrl Pts',(-66.2655539657919,3.21663700939875,8.09409501252873));
#38824=CARTESIAN_POINT('Ctrl Pts',(-66.6022993283403,3.25480527973138,7.07959750520892));
#38825=CARTESIAN_POINT('Ctrl Pts',(-66.7631910382533,3.27249821191336,6.63302022230481));
#38826=CARTESIAN_POINT('',(-73.6760374232779,5.16935883999202,0.190989875004182));
#38827=CARTESIAN_POINT('Ctrl Pts',(-66.7632425918307,3.2720446654144,6.633020912074));
#38828=CARTESIAN_POINT('Ctrl Pts',(-66.7778516238031,3.27363852677518,6.59368385722911));
#38829=CARTESIAN_POINT('Ctrl Pts',(-66.7926503366434,3.27521476311706,6.55407752441134));
#38830=CARTESIAN_POINT('Ctrl Pts',(-66.8076622570084,3.27677215677882,6.51414962524557));
#38831=CARTESIAN_POINT('Ctrl Pts',(-66.8227415209764,3.27833653692185,6.47404260918319));
#38832=CARTESIAN_POINT('Ctrl Pts',(-66.8380359055963,3.27988190475181,6.43361142106289));
#38833=CARTESIAN_POINT('Ctrl Pts',(-66.8535704549874,3.28140734584648,6.39274919904974));
#38834=CARTESIAN_POINT('Ctrl Pts',(-66.8691050043786,3.28293278694115,6.35188697703659));
#38835=CARTESIAN_POINT('Ctrl Pts',(-66.8848797161219,3.28443830178511,6.31059393057822));
#38836=CARTESIAN_POINT('Ctrl Pts',(-66.9009208783732,3.28592329229036,6.26870578557491));
#38837=CARTESIAN_POINT('Ctrl Pts',(-66.925751174839,3.28822192588786,6.20386665219223));
#38838=CARTESIAN_POINT('Ctrl Pts',(-66.9512195193938,3.29047109652991,6.13758563776401));
#38839=CARTESIAN_POINT('Ctrl Pts',(-66.9774293209226,3.2926746892832,6.07018552522113));
#38840=CARTESIAN_POINT('Ctrl Pts',(-66.9988272592458,3.29447372396008,6.0151594141083));
#38841=CARTESIAN_POINT('Ctrl Pts',(-67.0207195340082,3.29624244802965,5.95938828124706));
#38842=CARTESIAN_POINT('Ctrl Pts',(-67.0431661797375,3.29798514864501,5.90307322483236));
#38843=CARTESIAN_POINT('Ctrl Pts',(-67.081595026309,3.30096866677845,5.80666137387091));
#38844=CARTESIAN_POINT('Ctrl Pts',(-67.1216471810934,3.30387469587049,5.70866225403845));
#38845=CARTESIAN_POINT('Ctrl Pts',(-67.1636464856163,3.30674464355634,5.60964585544974));
#38846=CARTESIAN_POINT('Ctrl Pts',(-67.2071111346927,3.3097147229529,5.50717480107519));
#38847=CARTESIAN_POINT('Ctrl Pts',(-67.2527690423822,3.31264837414508,5.40305522896293));
#38848=CARTESIAN_POINT('Ctrl Pts',(-67.3008684292325,3.31559000642976,5.29763784637666));
#38849=CARTESIAN_POINT('Ctrl Pts',(-67.3207250789926,3.31680438702429,5.25411887073675));
#38850=CARTESIAN_POINT('Ctrl Pts',(-67.3409981849322,3.31802043944008,5.21037835697596));
#38851=CARTESIAN_POINT('Ctrl Pts',(-67.3617067668992,3.31924268717797,5.16643939842894));
#38852=CARTESIAN_POINT('Ctrl Pts',(-67.4131411385364,3.32227841142426,5.05730721705296));
#38853=CARTESIAN_POINT('Ctrl Pts',(-67.4672594232976,3.32534977695346,4.94695098046708));
#38854=CARTESIAN_POINT('Ctrl Pts',(-67.5243778514364,3.32854526909525,4.83578384025443));
#38855=CARTESIAN_POINT('Ctrl Pts',(-67.5797346638728,3.33164220759477,4.72804525692193));
#38856=CARTESIAN_POINT('Ctrl Pts',(-67.637909632063,3.33485546291609,4.61954493297593));
#38857=CARTESIAN_POINT('Ctrl Pts',(-67.6992220665778,3.33830219654704,4.51065257941795));
#38858=CARTESIAN_POINT('Ctrl Pts',(-67.7594871016904,3.34169004967889,4.40362043230804));
#38859=CARTESIAN_POINT('Ctrl Pts',(-67.8227834984399,3.34530314118978,4.29620941841597));
#38860=CARTESIAN_POINT('Ctrl Pts',(-67.8894425869409,3.34929320208703,4.18876581786222));
#38861=CARTESIAN_POINT('Ctrl Pts',(-67.9544129231919,3.35318217812895,4.08404421105687));
#38862=CARTESIAN_POINT('Ctrl Pts',(-68.022577948134,3.35742904100138,3.97929148951414));
#38863=CARTESIAN_POINT('Ctrl Pts',(-68.0942684114907,3.36221702676486,3.87482570228378));
#38864=CARTESIAN_POINT('Ctrl Pts',(-68.1439301056711,3.3655337787231,3.80245975938383));
#38865=CARTESIAN_POINT('Ctrl Pts',(-68.1952840339283,3.36911107463874,3.73023144553659));
#38866=CARTESIAN_POINT('Ctrl Pts',(-68.2484463317038,3.37302320707464,3.65824640771746));
#38867=CARTESIAN_POINT('Ctrl Pts',(-68.2963237263679,3.37654643154854,3.59341745543768));
#38868=CARTESIAN_POINT('Ctrl Pts',(-68.3456679353863,3.38034131488696,3.52878579007826));
#38869=CARTESIAN_POINT('Ctrl Pts',(-68.396566560834,3.38447437656862,3.46442745789461));
#38870=CARTESIAN_POINT('Ctrl Pts',(-68.4399174001416,3.38799454418091,3.40961285942435));
#38871=CARTESIAN_POINT('Ctrl Pts',(-68.4843962019402,3.39176007652746,3.35499649460645));
#38872=CARTESIAN_POINT('Ctrl Pts',(-68.5300478346321,3.39582059599171,3.30062598661843));
#38873=CARTESIAN_POINT('Ctrl Pts',(-68.605148574348,3.40250048885453,3.21118197053735));
#38874=CARTESIAN_POINT('Ctrl Pts',(-68.6832846494335,3.4099628769802,3.12244281424077));
#38875=CARTESIAN_POINT('Ctrl Pts',(-68.7644215211146,3.41843068019497,3.03458147483682));
#38876=CARTESIAN_POINT('Ctrl Pts',(-68.8437792250609,3.42671280158652,2.94864675716427));
#38877=CARTESIAN_POINT('Ctrl Pts',(-68.9260078649796,3.43595736036824,2.86355140090532));
#38878=CARTESIAN_POINT('Ctrl Pts',(-69.0110358708828,3.44639725953889,2.77947643571424));
#38879=CARTESIAN_POINT('Ctrl Pts',(-69.0953878948292,3.45675416036805,2.69606987570192));
#38880=CARTESIAN_POINT('Ctrl Pts',(-69.1824951022211,3.46828818269589,2.61366721682793));
#38881=CARTESIAN_POINT('Ctrl Pts',(-69.2722450959242,3.4812410257998,2.53246965132781));
#38882=CARTESIAN_POINT('Ctrl Pts',(-69.3615880501007,3.49413512439679,2.45164033787172));
#38883=CARTESIAN_POINT('Ctrl Pts',(-69.4535498120667,3.50843600124425,2.37200498389905));
#38884=CARTESIAN_POINT('Ctrl Pts',(-69.5479765076371,3.52438501326241,2.29379058216315));
#38885=CARTESIAN_POINT('Ctrl Pts',(-69.5835334743656,3.53039071415298,2.26433845675087));
#38886=CARTESIAN_POINT('Ctrl Pts',(-69.6194395246876,3.53663007920999,2.2350881216089));
#38887=CARTESIAN_POINT('Ctrl Pts',(-69.6556849168736,3.54311573774292,2.20605283237209));
#38888=CARTESIAN_POINT('Ctrl Pts',(-69.7514241999826,3.56024708219757,2.12935845527359));
#38889=CARTESIAN_POINT('Ctrl Pts',(-69.8495489942764,3.57910088692489,2.05416051893023));
#38890=CARTESIAN_POINT('Ctrl Pts',(-69.9497187807409,3.59988140484318,1.98056289443286));
#38891=CARTESIAN_POINT('Ctrl Pts',(-70.0493579133009,3.62055183704241,1.90735515662866));
#38892=CARTESIAN_POINT('Ctrl Pts',(-70.1510198437214,3.64312944268963,1.83573095377873));
#38893=CARTESIAN_POINT('Ctrl Pts',(-70.2543363411126,3.66778714917268,1.76581974058179));
#38894=CARTESIAN_POINT('Ctrl Pts',(-70.3568397508631,3.69225080265454,1.69645871970495));
#38895=CARTESIAN_POINT('Ctrl Pts',(-70.4609711070713,3.71876259431705,1.62878411238229));
#38896=CARTESIAN_POINT('Ctrl Pts',(-70.5663476422515,3.74745271803715,1.56294609407678));
#38897=CARTESIAN_POINT('Ctrl Pts',(-70.6704395356238,3.77579308142074,1.49791070484539));
#38898=CARTESIAN_POINT('Ctrl Pts',(-70.7757457442586,3.80625938925171,1.43466779231534));
#38899=CARTESIAN_POINT('Ctrl Pts',(-70.8818848613732,3.83893150095146,1.37338032282391));
#38900=CARTESIAN_POINT('Ctrl Pts',(-70.9359385471963,3.85557049427463,1.34216832755918));
#38901=CARTESIAN_POINT('Ctrl Pts',(-70.9902081180437,3.87278080606398,1.31146374997487));
#38902=CARTESIAN_POINT('Ctrl Pts',(-71.0446427957615,3.89056794250507,1.28128941908642));
#38903=CARTESIAN_POINT('Ctrl Pts',(-71.1348036965975,3.92002901974587,1.23131126234723));
#38904=CARTESIAN_POINT('Ctrl Pts',(-71.225431930372,3.95108245182755,1.18276232504616));
#38905=CARTESIAN_POINT('Ctrl Pts',(-71.316067797823,3.98366316485251,1.13570828437813));
#38906=CARTESIAN_POINT('Ctrl Pts',(-71.4049975632047,4.01563058842073,1.08953997469508));
#38907=CARTESIAN_POINT('Ctrl Pts',(-71.4939342726877,4.049068371674,1.04481112345883));
#38908=CARTESIAN_POINT('Ctrl Pts',(-71.5824508941236,4.08386513405905,1.00158432608665));
#38909=CARTESIAN_POINT('Ctrl Pts',(-71.6050814782526,4.09276144128134,0.990532755673197));
#38910=CARTESIAN_POINT('Ctrl Pts',(-71.6276846575919,4.10174631856564,0.979579355859735));
#38911=CARTESIAN_POINT('Ctrl Pts',(-71.6502534198816,4.11081736792181,0.968725141126268));
#38912=CARTESIAN_POINT('Ctrl Pts',(-71.7413595560693,4.14743560366732,0.924908579410377));
#38913=CARTESIAN_POINT('Ctrl Pts',(-71.8319031202047,4.18546188054524,0.882709644373667));
#38914=CARTESIAN_POINT('Ctrl Pts',(-71.9214481093997,4.22457715179907,0.842184297212655));
#38915=CARTESIAN_POINT('Ctrl Pts',(-72.0174138967299,4.26649717251995,0.79875309149031));
#38916=CARTESIAN_POINT('Ctrl Pts',(-72.1122322699238,4.30966740820752,0.757244478751865));
#38917=CARTESIAN_POINT('Ctrl Pts',(-72.2053958847573,4.35364318548031,0.717705234412282));
#38918=CARTESIAN_POINT('Ctrl Pts',(-72.2985594995909,4.3976189627531,0.678165990072699));
#38919=CARTESIAN_POINT('Ctrl Pts',(-72.390068306429,4.44239909257851,0.640596137078233));
#38920=CARTESIAN_POINT('Ctrl Pts',(-72.479447063832,4.48750315511749,0.605018247143105));
#38921=CARTESIAN_POINT('Ctrl Pts',(-72.5702985368102,4.53335040829074,0.568854131642064));
#38922=CARTESIAN_POINT('Ctrl Pts',(-72.659020807773,4.57956119168153,0.534719321379211));
#38923=CARTESIAN_POINT('Ctrl Pts',(-72.7457116179679,4.62594207736946,0.502385439090387));
#38924=CARTESIAN_POINT('Ctrl Pts',(-72.8366881117079,4.67461586813179,0.468453085326186));
#38925=CARTESIAN_POINT('Ctrl Pts',(-72.9254276354649,4.72347695076411,0.436503801608705));
#38926=CARTESIAN_POINT('Ctrl Pts',(-73.0120512426314,4.7723580160016,0.406259796438403));
#38927=CARTESIAN_POINT('Ctrl Pts',(-73.1013783849707,4.82276466627851,0.375071871539767));
#38928=CARTESIAN_POINT('Ctrl Pts',(-73.1884557723436,4.87319281725982,0.345696966659892));
#38929=CARTESIAN_POINT('Ctrl Pts',(-73.2734196953545,4.92351553196678,0.317821550706115));
#38930=CARTESIAN_POINT('Ctrl Pts',(-73.3629470980995,4.97654111961786,0.288448924038924));
#38931=CARTESIAN_POINT('Ctrl Pts',(-73.450128176113,5.02944981953762,0.260740832188493));
#38932=CARTESIAN_POINT('Ctrl Pts',(-73.5351217584104,5.08215181279788,0.234326404103092));
#38933=CARTESIAN_POINT('Ctrl Pts',(-73.582596736888,5.11158963537376,0.21957206182269));
#38934=CARTESIAN_POINT('Ctrl Pts',(-73.6293891746598,5.14096398116758,0.205221308463415));
#38935=CARTESIAN_POINT('Ctrl Pts',(-73.6755262547354,5.17026613426529,0.191209597395648));
#38936=CARTESIAN_POINT('',(-79.5980561166416,9.79488102647745,-1.92025417899612));
#38937=CARTESIAN_POINT('Ctrl Pts',(-73.6764877119598,5.1685596039116,0.190796321415114));
#38938=CARTESIAN_POINT('Ctrl Pts',(-74.7404219526711,5.85068157891375,-0.142609954538472));
#38939=CARTESIAN_POINT('Ctrl Pts',(-75.9741654535975,6.89428741101915,-0.412567402884934));
#38940=CARTESIAN_POINT('Ctrl Pts',(-77.4581499404949,8.19662250468364,-0.873282366765809));
#38941=CARTESIAN_POINT('Ctrl Pts',(-78.1080385927614,8.74315679055215,-1.12050093759123));
#38942=CARTESIAN_POINT('Ctrl Pts',(-78.8357086373011,9.31133939639374,-1.44888811728152));
#38943=CARTESIAN_POINT('Ctrl Pts',(-79.2776917908501,9.61051959968398,-1.69898330179011));
#38944=CARTESIAN_POINT('Ctrl Pts',(-79.5980561168787,9.79488102596951,-1.92025417907613));
#38945=CARTESIAN_POINT('',(-77.5413434256017,9.45934560247393,-5.67965754882122));
#38946=CARTESIAN_POINT('Ctrl Pts',(-79.5980561168786,9.7948810259695,-1.92025417907612));
#38947=CARTESIAN_POINT('Ctrl Pts',(-79.3926541200977,9.78652201900712,-2.47576181499884));
#38948=CARTESIAN_POINT('Ctrl Pts',(-78.8071962567564,9.7034726253451,-3.78882461998114));
#38949=CARTESIAN_POINT('Ctrl Pts',(-78.0251745283461,9.56134461172776,-5.02766395488251));
#38950=CARTESIAN_POINT('Ctrl Pts',(-77.5413122691002,9.45942207531784,-5.67964638243143));
#38951=CARTESIAN_POINT('',(-70.7282577522101,8.51486331985853,-11.892519184563));
#38952=CARTESIAN_POINT('Ctrl Pts',(-77.5413434256017,9.45934560247393,-5.67965754882122));
#38953=CARTESIAN_POINT('Ctrl Pts',(-77.5142821984464,9.45356384346927,-5.71556759801311));
#38954=CARTESIAN_POINT('Ctrl Pts',(-77.4869693706751,9.44763492792691,-5.75132849528266));
#38955=CARTESIAN_POINT('Ctrl Pts',(-77.459392567839,9.44158248309945,-5.78710530983847));
#38956=CARTESIAN_POINT('Ctrl Pts',(-77.4323651788443,9.43565062139332,-5.82216934136303));
#38957=CARTESIAN_POINT('Ctrl Pts',(-77.4050841899675,9.42960017534997,-5.85724885204878));
#38958=CARTESIAN_POINT('Ctrl Pts',(-77.3775393869878,9.42344934005853,-5.89245008383269));
#38959=CARTESIAN_POINT('Ctrl Pts',(-77.3507057470255,9.41745730955464,-5.926742475781));
#38960=CARTESIAN_POINT('Ctrl Pts',(-77.3236217027424,9.41137006917975,-5.96115047465854));
#38961=CARTESIAN_POINT('Ctrl Pts',(-77.2962797330602,9.40519958906143,-5.99572323319143));
#38962=CARTESIAN_POINT('Ctrl Pts',(-77.2823729183937,9.4020611274068,-6.01330780924863));
#38963=CARTESIAN_POINT('Ctrl Pts',(-77.2683994129127,9.39890104755503,-6.03093420635041));
#38964=CARTESIAN_POINT('Ctrl Pts',(-77.2543584747973,9.39572034184949,-6.04860371317784));
#38965=CARTESIAN_POINT('Ctrl Pts',(-77.2093734063961,9.38552983587676,-6.10521417372642));
#38966=CARTESIAN_POINT('Ctrl Pts',(-77.1636964406147,9.37512650810942,-6.16225985620397));
#38967=CARTESIAN_POINT('Ctrl Pts',(-77.1173124297829,9.36452720094655,-6.21966639031466));
#38968=CARTESIAN_POINT('Ctrl Pts',(-77.0724581614658,9.35427745843977,-6.27517965960673));
#38969=CARTESIAN_POINT('Ctrl Pts',(-77.0269427749634,9.34384437086552,-6.33103023795012));
#38970=CARTESIAN_POINT('Ctrl Pts',(-76.9807507843413,9.33325212543006,-6.38719925161227));
#38971=CARTESIAN_POINT('Ctrl Pts',(-76.9702354818589,9.33084087050855,-6.39998575768921));
#38972=CARTESIAN_POINT('Ctrl Pts',(-76.9596851070482,9.32842140837096,-6.41278897398065));
#38973=CARTESIAN_POINT('Ctrl Pts',(-76.9490994584738,9.32599409895416,-6.42560905396616));
#38974=CARTESIAN_POINT('Ctrl Pts',(-76.8689375031935,9.3076128096497,-6.52269169101637));
#38975=CARTESIAN_POINT('Ctrl Pts',(-76.7867518479299,9.28878025003937,-6.62074657320179));
#38976=CARTESIAN_POINT('Ctrl Pts',(-76.7024649817347,9.26965359217964,-6.71973310414691));
#38977=CARTESIAN_POINT('Ctrl Pts',(-76.625561125183,9.25220231158567,-6.81004902547595));
#38978=CARTESIAN_POINT('Ctrl Pts',(-76.5469082661047,9.23450749951946,-6.90114067648958));
#38979=CARTESIAN_POINT('Ctrl Pts',(-76.4664583841173,9.21669125658552,-6.99293229934345));
#38980=CARTESIAN_POINT('Ctrl Pts',(-76.4055809814877,9.20320948920882,-7.06239213501332));
#38981=CARTESIAN_POINT('Ctrl Pts',(-76.3436746896887,9.18965823967548,-7.13225188856446));
#38982=CARTESIAN_POINT('Ctrl Pts',(-76.2807215287226,9.17608787534858,-7.20245910972558));
#38983=CARTESIAN_POINT('Ctrl Pts',(-76.2175251915839,9.1624650912669,-7.27293752812414));
#38984=CARTESIAN_POINT('Ctrl Pts',(-76.1532738906648,9.14882286470201,-7.34376497718704));
#38985=CARTESIAN_POINT('Ctrl Pts',(-76.087955371975,9.13521006306119,-7.41489463717834));
#38986=CARTESIAN_POINT('Ctrl Pts',(-75.9758314377519,9.11184271018204,-7.53699381331019));
#38987=CARTESIAN_POINT('Ctrl Pts',(-75.8605011879027,9.08860063350606,-7.66039372555022));
#38988=CARTESIAN_POINT('Ctrl Pts',(-75.7413454478133,9.06564256808275,-7.78544462689756));
#38989=CARTESIAN_POINT('Ctrl Pts',(-75.6337419763672,9.04491031015393,-7.89837171779831));
#38990=CARTESIAN_POINT('Ctrl Pts',(-75.523018539085,9.0244100059248,-8.01264591774364));
#38991=CARTESIAN_POINT('Ctrl Pts',(-75.4087158498956,9.00428410594188,-8.12849174972041));
#38992=CARTESIAN_POINT('Ctrl Pts',(-75.3343282518198,8.99118627447822,-8.20388361712937));
#38993=CARTESIAN_POINT('Ctrl Pts',(-75.2584246377425,8.97824756940062,-8.27994043561488));
#38994=CARTESIAN_POINT('Ctrl Pts',(-75.1808786513554,8.96551237918548,-8.35671312887169));
#38995=CARTESIAN_POINT('Ctrl Pts',(-75.0861154632862,8.9499496494856,-8.45053133286425));
#38996=CARTESIAN_POINT('Ctrl Pts',(-74.9888998796607,8.93468501931142,-8.54536890727092));
#38997=CARTESIAN_POINT('Ctrl Pts',(-74.8895954521882,8.91990014338027,-8.64082848977418));
#38998=CARTESIAN_POINT('Ctrl Pts',(-74.8237602476036,8.91009831121166,-8.70411470272186));
#38999=CARTESIAN_POINT('Ctrl Pts',(-74.7570073460718,8.90050666601648,-8.7676736961274));
#39000=CARTESIAN_POINT('Ctrl Pts',(-74.6894475678803,8.89116756387664,-8.83138447768835));
#39001=CARTESIAN_POINT('Ctrl Pts',(-74.5927641137914,8.87780256065818,-8.92255970929652));
#39002=CARTESIAN_POINT('Ctrl Pts',(-74.4944270055992,8.86495684504577,-9.01404623510722));
#39003=CARTESIAN_POINT('Ctrl Pts',(-74.3947926712449,8.85270483437522,-9.10547037505296));
#39004=CARTESIAN_POINT('Ctrl Pts',(-74.29578008106,8.84052927943902,-9.19632400457842));
#39005=CARTESIAN_POINT('Ctrl Pts',(-74.195486619814,8.82894028441388,-9.28711544802413));
#39006=CARTESIAN_POINT('Ctrl Pts',(-74.0942825153974,8.81796417439208,-9.37747159674706));
#39007=CARTESIAN_POINT('Ctrl Pts',(-73.9934637520285,8.80702985660548,-9.46748370870173));
#39008=CARTESIAN_POINT('Ctrl Pts',(-73.891741598813,8.79670387124786,-9.55706325103888));
#39009=CARTESIAN_POINT('Ctrl Pts',(-73.7894983248483,8.78696310332303,-9.64584369468491));
#39010=CARTESIAN_POINT('Ctrl Pts',(-73.7744301881695,8.78552755439393,-9.65892774224506));
#39011=CARTESIAN_POINT('Ctrl Pts',(-73.7593507563086,8.78410462767017,-9.67199444704903));
#39012=CARTESIAN_POINT('Ctrl Pts',(-73.7442612753102,8.78269415742303,-9.68504265207626));
#39013=CARTESIAN_POINT('Ctrl Pts',(-73.6420318120065,8.77313838699025,-9.7734427101798));
#39014=CARTESIAN_POINT('Ctrl Pts',(-73.5393410808177,8.7641587418496,-9.8609932390083));
#39015=CARTESIAN_POINT('Ctrl Pts',(-73.4365784472836,8.75566920417689,-9.94734692942645));
#39016=CARTESIAN_POINT('Ctrl Pts',(-73.3285944434713,8.7467483130233,-10.0380882515845));
#39017=CARTESIAN_POINT('Ctrl Pts',(-73.2205317290125,8.73836812583255,-10.1275072089461));
#39018=CARTESIAN_POINT('Ctrl Pts',(-73.1128365659561,8.73037266133452,-10.2152131863157));
#39019=CARTESIAN_POINT('Ctrl Pts',(-73.071220190016,8.72728299373086,-10.2491051905879));
#39020=CARTESIAN_POINT('Ctrl Pts',(-73.0296585866431,8.72425024662359,-10.2827415972262));
#39021=CARTESIAN_POINT('Ctrl Pts',(-72.9881769722381,8.72126366625822,-10.3161007689154));
#39022=CARTESIAN_POINT('Ctrl Pts',(-72.927197056175,8.71687325323771,-10.3651403137527));
#39023=CARTESIAN_POINT('Ctrl Pts',(-72.8663948120556,8.71257989567172,-10.4135664782779));
#39024=CARTESIAN_POINT('Ctrl Pts',(-72.8057311638433,8.70833772590909,-10.4614014331091));
#39025=CARTESIAN_POINT('Ctrl Pts',(-72.6720088391437,8.69898661005723,-10.5668451634225));
#39026=CARTESIAN_POINT('Ctrl Pts',(-72.5389607681471,8.6898833035686,-10.6694195862342));
#39027=CARTESIAN_POINT('Ctrl Pts',(-72.4061666716076,8.68054726327208,-10.7693713198737));
#39028=CARTESIAN_POINT('Ctrl Pts',(-72.2844782862219,8.67199200592869,-10.8609639840058));
#39029=CARTESIAN_POINT('Ctrl Pts',(-72.1630026242835,8.66324239041884,-10.9503544622541));
#39030=CARTESIAN_POINT('Ctrl Pts',(-72.0414094827878,8.65392446659711,-11.0376910827571));
#39031=CARTESIAN_POINT('Ctrl Pts',(-71.9568362998022,8.6474434556887,-11.0984374036128));
#39032=CARTESIAN_POINT('Ctrl Pts',(-71.8722061531492,8.64068749379229,-11.1581892721519));
#39033=CARTESIAN_POINT('Ctrl Pts',(-71.7874075681809,8.63352479050082,-11.216982677569));
#39034=CARTESIAN_POINT('Ctrl Pts',(-71.6784906925915,8.62432488152153,-11.2924980181338));
#39035=CARTESIAN_POINT('Ctrl Pts',(-71.5692957068855,8.61445495735751,-11.3664337484946));
#39036=CARTESIAN_POINT('Ctrl Pts',(-71.4595925371217,8.60361780995115,-11.4388129550185));
#39037=CARTESIAN_POINT('Ctrl Pts',(-71.3942487439551,8.59716275199647,-11.4819250356525));
#39038=CARTESIAN_POINT('Ctrl Pts',(-71.3287247224875,8.59036411398718,-11.5244841417791));
#39039=CARTESIAN_POINT('Ctrl Pts',(-71.2629723517172,8.58315381021533,-11.5664879117912));
#39040=CARTESIAN_POINT('Ctrl Pts',(-71.1364990449913,8.56928494206896,-11.6472812828309));
#39041=CARTESIAN_POINT('Ctrl Pts',(-71.0091819466483,8.5538952244241,-11.7260192601636));
#39042=CARTESIAN_POINT('Ctrl Pts',(-70.8806724029974,8.53650122260619,-11.8027469173222));
#39043=CARTESIAN_POINT('Ctrl Pts',(-70.8660800072997,8.53452611515439,-11.8114594245991));
#39044=CARTESIAN_POINT('Ctrl Pts',(-70.85147221969,8.53252511247036,-11.8201459985682));
#39045=CARTESIAN_POINT('Ctrl Pts',(-70.8368485139656,8.53049746366489,-11.8288066959609));
#39046=CARTESIAN_POINT('Ctrl Pts',(-70.8017234668938,8.5256272029335,-11.8496090431446));
#39047=CARTESIAN_POINT('Ctrl Pts',(-70.7665066081501,8.52060323625991,-11.8702621150382));
#39048=CARTESIAN_POINT('Ctrl Pts',(-70.7311906833193,8.51541564895962,-11.8907668872392));
#39049=CARTESIAN_POINT('Ctrl Pts',(-70.7302019192612,8.51527040853634,-11.8913409733454));
#39050=CARTESIAN_POINT('Ctrl Pts',(-70.7292130176079,8.51512517529256,-11.8919155266462));
#39051=CARTESIAN_POINT('Ctrl Pts',(-70.7282239782404,8.51497994858646,-11.8924905441709));
#39052=CARTESIAN_POINT('',(-57.8135230789085,6.69056632342548,-18.0349157105246));
#39053=CARTESIAN_POINT('Ctrl Pts',(-70.7282577522101,8.51486331985853,-11.892519184563));
#39054=CARTESIAN_POINT('Ctrl Pts',(-70.1991067619348,8.44172633189886,-12.218539623772));
#39055=CARTESIAN_POINT('Ctrl Pts',(-68.595429397507,8.158930957405,-13.1757731414385));
#39056=CARTESIAN_POINT('Ctrl Pts',(-66.4080850486133,7.61830551402404,-14.5220628619485));
#39057=CARTESIAN_POINT('Ctrl Pts',(-63.7670026279933,7.28205441226018,-15.9847718406443));
#39058=CARTESIAN_POINT('Ctrl Pts',(-61.8892806965024,7.15471518367529,-16.8453028714865));
#39059=CARTESIAN_POINT('Ctrl Pts',(-59.9765401917668,7.00460230079879,-17.5365065043827));
#39060=CARTESIAN_POINT('Ctrl Pts',(-58.5497235666632,6.81245518627654,-17.8884040415039));
#39061=CARTESIAN_POINT('Ctrl Pts',(-57.8135230790975,6.69056632259502,-18.0349157107833));
#39062=CARTESIAN_POINT('',(-44.8643748761871,5.20597739865049,-23.9801519720622));
#39063=CARTESIAN_POINT('Ctrl Pts',(-57.8135230790975,6.69056632259502,-18.0349157107833));
#39064=CARTESIAN_POINT('Ctrl Pts',(-57.1239745403965,6.58412560248485,-18.1969381440623));
#39065=CARTESIAN_POINT('Ctrl Pts',(-55.0066008221098,6.23208146801642,-18.6635552175992));
#39066=CARTESIAN_POINT('Ctrl Pts',(-52.3438248091449,5.73435620824511,-19.2638310488358));
#39067=CARTESIAN_POINT('Ctrl Pts',(-50.0095424054025,5.30085549787886,-20.220604371564));
#39068=CARTESIAN_POINT('Ctrl Pts',(-48.2669654993335,5.10361702097977,-21.2264548583875));
#39069=CARTESIAN_POINT('Ctrl Pts',(-46.9594441235353,5.13430758608674,-22.1958151860038));
#39070=CARTESIAN_POINT('Ctrl Pts',(-45.8504881283735,5.21184561373662,-23.1088853518396));
#39071=CARTESIAN_POINT('Ctrl Pts',(-45.2012130342128,5.23387305606066,-23.6826188427425));
#39072=CARTESIAN_POINT('Ctrl Pts',(-44.8643748763769,5.20597739807172,-23.9801519722228));
#39073=CARTESIAN_POINT('',(-41.4215456143024,4.68791021227308,-29.7512571116587));
#39074=CARTESIAN_POINT('Ctrl Pts',(-44.8643748763769,5.20597739807172,-23.9801519722228));
#39075=CARTESIAN_POINT('Ctrl Pts',(-44.74295142856,5.19893273360771,-24.0982573983942));
#39076=CARTESIAN_POINT('Ctrl Pts',(-44.4866987396665,5.17768472779144,-24.3599634571171));
#39077=CARTESIAN_POINT('Ctrl Pts',(-43.7774989443756,5.08577719072335,-25.1469769549528));
#39078=CARTESIAN_POINT('Ctrl Pts',(-42.7956488003254,4.84372654876611,-26.5306371507459));
#39079=CARTESIAN_POINT('Ctrl Pts',(-41.9333999007591,4.68167633313014,-28.2389876838209));
#39080=CARTESIAN_POINT('Ctrl Pts',(-41.5686373679341,4.67844271843895,-29.2605708183325));
#39081=CARTESIAN_POINT('Ctrl Pts',(-41.4215456143024,4.68791021227308,-29.7512571116587));
#39082=CARTESIAN_POINT('',(-40.1355627918321,4.76730435132371,-35.6660886995316));
#39083=CARTESIAN_POINT('Ctrl Pts',(-41.4215456143025,4.68791021227309,-29.7512571116587));
#39084=CARTESIAN_POINT('Ctrl Pts',(-41.3092811227302,4.69284109397027,-30.1101403746882));
#39085=CARTESIAN_POINT('Ctrl Pts',(-41.1168122255416,4.70227545160565,-30.8154015426932));
#39086=CARTESIAN_POINT('Ctrl Pts',(-40.9411342639833,4.71057860533754,-31.5583878958659));
#39087=CARTESIAN_POINT('Ctrl Pts',(-40.72104027405,4.72052127144792,-32.5727429381947));
#39088=CARTESIAN_POINT('Ctrl Pts',(-40.5142429668683,4.72897579183149,-33.638548551572));
#39089=CARTESIAN_POINT('Ctrl Pts',(-40.3021090297733,4.74530128710119,-34.7695223916763));
#39090=CARTESIAN_POINT('Ctrl Pts',(-40.197670469322,4.75763956421394,-35.3320435682359));
#39091=CARTESIAN_POINT('Ctrl Pts',(-40.1355627919428,4.76730435097372,-35.6660886995623));
#39092=CARTESIAN_POINT('',(-38.8604541099244,4.82976572790842,-41.6539325852781));
#39093=CARTESIAN_POINT('Ctrl Pts',(-40.1355627919428,4.76730435097372,-35.6660886995623));
#39094=CARTESIAN_POINT('Ctrl Pts',(-40.0697893952873,4.77667332555081,-36.0099787209928));
#39095=CARTESIAN_POINT('Ctrl Pts',(-39.9548407119179,4.79179800913514,-36.603881143725));
#39096=CARTESIAN_POINT('Ctrl Pts',(-39.7443037262004,4.81133016772462,-37.6330866698068));
#39097=CARTESIAN_POINT('Ctrl Pts',(-39.5813565519597,4.82173156565819,-38.3962454196463));
#39098=CARTESIAN_POINT('Ctrl Pts',(-39.4305411403599,4.82773783061676,-39.0811836979273));
#39099=CARTESIAN_POINT('Ctrl Pts',(-39.2609912818215,4.83170251246378,-39.8388585382037));
#39100=CARTESIAN_POINT('Ctrl Pts',(-39.0664822089796,4.83206157401462,-40.699884114134));
#39101=CARTESIAN_POINT('Ctrl Pts',(-38.9270116850831,4.83045996119414,-41.3378025229821));
#39102=CARTESIAN_POINT('Ctrl Pts',(-38.8604541099244,4.82976572790842,-41.6539325852781));
#39103=CARTESIAN_POINT('',(-38.0224643186749,4.86842248838796,-47.6590907843941));
#39104=CARTESIAN_POINT('Ctrl Pts',(-38.8604525038006,4.82977022535046,-41.6539322549122));
#39105=CARTESIAN_POINT('Ctrl Pts',(-38.7895469391281,4.82895050845352,-41.9867860224295));
#39106=CARTESIAN_POINT('Ctrl Pts',(-38.7233060696144,4.82752930432473,-42.3153012863669));
#39107=CARTESIAN_POINT('Ctrl Pts',(-38.6000287997093,4.82483865752222,-42.9730936841352));
#39108=CARTESIAN_POINT('Ctrl Pts',(-38.5399565866358,4.8233804990704,-43.3171996550799));
#39109=CARTESIAN_POINT('Ctrl Pts',(-38.4516802292394,4.82286779338988,-43.8813591795731));
#39110=CARTESIAN_POINT('Ctrl Pts',(-38.4197926585925,4.82326787763993,-44.1037768924137));
#39111=CARTESIAN_POINT('Ctrl Pts',(-38.2254488332384,4.82915172129242,-45.5525914827238));
#39112=CARTESIAN_POINT('Ctrl Pts',(-38.1374175968506,4.85081367644718,-46.6695328022788));
#39113=CARTESIAN_POINT('Ctrl Pts',(-38.0216341588543,4.87047774970745,-47.6589526062877));
#39114=CARTESIAN_POINT('',(-36.1829138277439,4.79791400485576,-53.6562428681641));
#39115=CARTESIAN_POINT('Ctrl Pts',(-38.0224643186749,4.86842248838796,-47.6590907843941));
#39116=CARTESIAN_POINT('Ctrl Pts',(-37.9812657358155,4.87623123772776,-48.0222701187376));
#39117=CARTESIAN_POINT('Ctrl Pts',(-37.8390083119489,4.91385101443275,-49.095218604347));
#39118=CARTESIAN_POINT('Ctrl Pts',(-37.4172837879437,4.97200393690399,-51.0816259402684));
#39119=CARTESIAN_POINT('Ctrl Pts',(-36.8018062134426,4.93958207757202,-52.5177243515675));
#39120=CARTESIAN_POINT('Ctrl Pts',(-36.1829138277439,4.79791400485575,-53.6562428681641));
#39121=CARTESIAN_POINT('',(-33.2870419059708,4.35253527752949,-59.9326413363873));
#39122=CARTESIAN_POINT('Ctrl Pts',(-36.1829138277439,4.79791400485575,-53.6562428681641));
#39123=CARTESIAN_POINT('Ctrl Pts',(-35.8221894292354,4.71279832802143,-54.2735126527001));
#39124=CARTESIAN_POINT('Ctrl Pts',(-35.1345762789437,4.46191327643785,-55.4630423598499));
#39125=CARTESIAN_POINT('Ctrl Pts',(-34.1112888063175,4.18758073788383,-57.6561452037581));
#39126=CARTESIAN_POINT('Ctrl Pts',(-33.5340571648804,4.24789457701618,-59.2008344761412));
#39127=CARTESIAN_POINT('Ctrl Pts',(-33.2870419060249,4.35253527707242,-59.9326413364709));
#39128=CARTESIAN_POINT('',(-30.3753540341099,6.01695723880277,-66.3794227429406));
#39129=CARTESIAN_POINT('Ctrl Pts',(-33.2870419060249,4.35253527707242,-59.9326413364709));
#39130=CARTESIAN_POINT('Ctrl Pts',(-33.1236843979303,4.41327697339383,-60.3703598245789));
#39131=CARTESIAN_POINT('Ctrl Pts',(-32.6598069524929,4.6233160195265,-61.6572795724073));
#39132=CARTESIAN_POINT('Ctrl Pts',(-31.725539611122,5.1629429740609,-64.061279077029));
#39133=CARTESIAN_POINT('Ctrl Pts',(-30.929578969617,5.6097190919677,-65.4015789370632));
#39134=CARTESIAN_POINT('Ctrl Pts',(-30.3753540341099,6.01695723880277,-66.3794227429406));
#39135=CARTESIAN_POINT('',(-27.8032099026791,9.23603570625527,-72.5577783044281));
#39136=CARTESIAN_POINT('Ctrl Pts',(-30.3753540341099,6.01695723880277,-66.3794227429406));
#39137=CARTESIAN_POINT('Ctrl Pts',(-30.1088133612586,6.21732189962616,-66.8603832394881));
#39138=CARTESIAN_POINT('Ctrl Pts',(-29.7096580135423,6.55735136704459,-67.5873569901587));
#39139=CARTESIAN_POINT('Ctrl Pts',(-28.7821722057447,7.57574471691707,-69.5467552476757));
#39140=CARTESIAN_POINT('Ctrl Pts',(-28.2846186462697,8.42885715791647,-71.0332031632364));
#39141=CARTESIAN_POINT('Ctrl Pts',(-27.8032099026791,9.23603570625527,-72.5577783044281));
#39142=CARTESIAN_POINT('',(-25.9521939426092,12.4413262855032,-78.5797190178297));
#39143=CARTESIAN_POINT('Ctrl Pts',(-27.8032099155366,9.23604325175907,-72.5577743135822));
#39144=CARTESIAN_POINT('Ctrl Pts',(-27.7898641356696,9.25902028195003,-72.6011740541424));
#39145=CARTESIAN_POINT('Ctrl Pts',(-27.7716651061686,9.29043033079141,-72.6604932145904));
#39146=CARTESIAN_POINT('Ctrl Pts',(-27.7311843931623,9.36074589208966,-72.7932093170237));
#39147=CARTESIAN_POINT('Ctrl Pts',(-27.7131022311491,9.39228751256304,-72.8527202187813));
#39148=CARTESIAN_POINT('Ctrl Pts',(-27.6591706521313,9.48670680637636,-73.0308045499805));
#39149=CARTESIAN_POINT('Ctrl Pts',(-27.6233481930299,9.54988119753572,-73.1498763380756));
#39150=CARTESIAN_POINT('Ctrl Pts',(-27.5171321758154,9.73818724164291,-73.5045914452129));
#39151=CARTESIAN_POINT('Ctrl Pts',(-27.4454683323948,9.86657180310599,-73.7461526383459));
#39152=CARTESIAN_POINT('Ctrl Pts',(-27.2390203345148,10.2379066566848,-74.4442925145932));
#39153=CARTESIAN_POINT('Ctrl Pts',(-27.0994468304465,10.4909718054446,-74.9193670196221));
#39154=CARTESIAN_POINT('Ctrl Pts',(-26.7946207936278,11.0357645089441,-75.9416399738098));
#39155=CARTESIAN_POINT('Ctrl Pts',(-26.6360619980652,11.314717467905,-76.4648390599111));
#39156=CARTESIAN_POINT('Ctrl Pts',(-26.3050671814268,11.8772403762864,-77.5203681238995));
#39157=CARTESIAN_POINT('Ctrl Pts',(-26.1315729170005,12.1624636612076,-78.0558078244091));
#39158=CARTESIAN_POINT('Ctrl Pts',(-25.9521939426143,12.4413262860545,-78.5797190175208));
#39159=CARTESIAN_POINT('',(-25.701333505378,12.8213469096823,-79.2936899992609));
#39160=CARTESIAN_POINT('Ctrl Pts',(-25.9521939426076,12.4413262858927,-78.5797190176306));
#39161=CARTESIAN_POINT('Ctrl Pts',(-25.8694938500183,12.5699781302287,-78.8214229331902));
#39162=CARTESIAN_POINT('Ctrl Pts',(-25.7858492981987,12.6969136284318,-79.0599051073278));
#39163=CARTESIAN_POINT('Ctrl Pts',(-25.7013798878604,12.8212786209475,-79.2935616983239));
#39164=CARTESIAN_POINT('',(-20.8093218985896,12.6047452125772,-78.8857087163453));
#39165=CARTESIAN_POINT('Ctrl Pts',(-25.7013238054811,12.8213611907999,-79.2937168306377));
#39166=CARTESIAN_POINT('Ctrl Pts',(-25.677759723027,12.9497254061923,-79.5350654335173));
#39167=CARTESIAN_POINT('Ctrl Pts',(-25.6134596233024,13.054467242967,-79.731873404679));
#39168=CARTESIAN_POINT('Ctrl Pts',(-25.4062110463656,13.2656356021316,-80.128476351569));
#39169=CARTESIAN_POINT('Ctrl Pts',(-25.2498435162777,13.350811855551,-80.2882896491754));
#39170=CARTESIAN_POINT('Ctrl Pts',(-24.9061202849933,13.4995897428215,-80.5673656272477));
#39171=CARTESIAN_POINT('Ctrl Pts',(-24.6468918170405,13.5747625375941,-80.7082619530755));
#39172=CARTESIAN_POINT('Ctrl Pts',(-23.9892905759402,13.6953664711755,-80.9343907983184));
#39173=CARTESIAN_POINT('Ctrl Pts',(-23.4919735177951,13.7506233016025,-81.038109384192));
#39174=CARTESIAN_POINT('Ctrl Pts',(-22.5135030627148,13.7417998945799,-81.0220713233488));
#39175=CARTESIAN_POINT('Ctrl Pts',(-22.1753683303654,13.7101025139875,-80.9628345173954));
#39176=CARTESIAN_POINT('Ctrl Pts',(-21.6613306788478,13.620361236039,-80.7946514359959));
#39177=CARTESIAN_POINT('Ctrl Pts',(-21.4654769001396,13.5650100503355,-80.6908083589357));
#39178=CARTESIAN_POINT('Ctrl Pts',(-21.1272843829631,13.4213387174777,-80.4210520847113));
#39179=CARTESIAN_POINT('Ctrl Pts',(-21.0209737284345,13.3421252329789,-80.2722205693931));
#39180=CARTESIAN_POINT('Ctrl Pts',(-20.8884830981335,13.209475077092,-80.0229241692315));
#39181=CARTESIAN_POINT('Ctrl Pts',(-20.8159402909792,13.1168800297615,-79.8488783976986));
#39182=CARTESIAN_POINT('Ctrl Pts',(-20.7555355063041,12.8585107795136,-79.3630420047952));
#39183=CARTESIAN_POINT('Ctrl Pts',(-20.7713716558706,12.7296582669527,-79.1206857196503));
#39184=CARTESIAN_POINT('Ctrl Pts',(-20.8093218984874,12.6047452132069,-78.8857087160435));
#39185=CARTESIAN_POINT('',(-21.0431040492689,12.4421761536719,-78.5796470221002));
#39186=CARTESIAN_POINT('Ctrl Pts',(-20.8093218987925,12.6047452131661,-78.8857087159663));
#39187=CARTESIAN_POINT('Ctrl Pts',(-20.8889387478986,12.5521187796536,-78.7866255044787));
#39188=CARTESIAN_POINT('Ctrl Pts',(-20.9668291889875,12.4978886120539,-78.6845286315191));
#39189=CARTESIAN_POINT('Ctrl Pts',(-21.043057427238,12.4422102065963,-78.5797111314019));
#39190=CARTESIAN_POINT('',(-23.6734819284684,9.24326495192996,-72.5612011682817));
#39191=CARTESIAN_POINT('Ctrl Pts',(-21.0431231485117,12.4421622035058,-78.5796207589988));
#39192=CARTESIAN_POINT('Ctrl Pts',(-21.1180479364394,12.3874344879029,-78.4765929841646));
#39193=CARTESIAN_POINT('Ctrl Pts',(-21.1912719403466,12.3312721447608,-78.3708704737982));
#39194=CARTESIAN_POINT('Ctrl Pts',(-21.2629202654535,12.2738551841641,-78.2627919303907));
#39195=CARTESIAN_POINT('Ctrl Pts',(-21.3432015307692,12.2095200271257,-78.1416909527295));
#39196=CARTESIAN_POINT('Ctrl Pts',(-21.4215050496884,12.143609457215,-78.0176315203387));
#39197=CARTESIAN_POINT('Ctrl Pts',(-21.4979790544219,12.0763456889671,-77.8910318283258));
#39198=CARTESIAN_POINT('Ctrl Pts',(-21.565187494861,12.0172315759066,-77.7797709117582));
#39199=CARTESIAN_POINT('Ctrl Pts',(-21.630982480635,11.9570714261746,-77.6665463444693));
#39200=CARTESIAN_POINT('Ctrl Pts',(-21.6954456408304,11.8960034591588,-77.5516183175351));
#39201=CARTESIAN_POINT('Ctrl Pts',(-21.7623500478192,11.8326228227331,-77.4323379182326));
#39202=CARTESIAN_POINT('Ctrl Pts',(-21.82799276352,11.7680944969581,-77.310902619301));
#39203=CARTESIAN_POINT('Ctrl Pts',(-21.8921956945099,11.7028022397038,-77.1880352793384));
#39204=CARTESIAN_POINT('Ctrl Pts',(-21.9142041224075,11.680420396478,-77.1459169998324));
#39205=CARTESIAN_POINT('Ctrl Pts',(-21.9360435805853,11.6579489835836,-77.1036308166521));
#39206=CARTESIAN_POINT('Ctrl Pts',(-21.957707579971,11.6354040017278,-77.0612068658632));
#39207=CARTESIAN_POINT('Ctrl Pts',(-22.0297903066051,11.5603899779938,-76.9200494556811));
#39208=CARTESIAN_POINT('Ctrl Pts',(-22.099927047318,11.4845606008049,-76.7773651932802));
#39209=CARTESIAN_POINT('Ctrl Pts',(-22.1682847108296,11.4079311890524,-76.6331838251872));
#39210=CARTESIAN_POINT('Ctrl Pts',(-22.2206631919412,11.3492145508602,-76.5227060721842));
#39211=CARTESIAN_POINT('Ctrl Pts',(-22.2719983650367,11.2900282995873,-76.411349529747));
#39212=CARTESIAN_POINT('Ctrl Pts',(-22.3223795367015,11.2303864433944,-76.2991408990849));
#39213=CARTESIAN_POINT('Ctrl Pts',(-22.3765225385033,11.166291286005,-76.1785539438521));
#39214=CARTESIAN_POINT('Ctrl Pts',(-22.4294720817398,11.1017772920471,-76.0571848686692));
#39215=CARTESIAN_POINT('Ctrl Pts',(-22.4812879554131,11.0369702725863,-75.9352703929272));
#39216=CARTESIAN_POINT('Ctrl Pts',(-22.5008207932577,11.0125402106655,-75.8893127448791));
#39217=CARTESIAN_POINT('Ctrl Pts',(-22.5201926240654,10.9880687491465,-75.8432780440593));
#39218=CARTESIAN_POINT('Ctrl Pts',(-22.5394068429119,10.9635635598301,-75.7971807191217));
#39219=CARTESIAN_POINT('Ctrl Pts',(-22.5437545941372,10.9580185794316,-75.7867499177145));
#39220=CARTESIAN_POINT('Ctrl Pts',(-22.5480942753898,10.9524718743525,-75.7763159140468));
#39221=CARTESIAN_POINT('Ctrl Pts',(-22.5524259259098,10.9469235374562,-75.7658788827482));
#39222=CARTESIAN_POINT('Ctrl Pts',(-22.5561213420508,10.9421901422692,-75.7569748463429));
#39223=CARTESIAN_POINT('Ctrl Pts',(-22.5598105984477,10.9374559716686,-75.7480693818334));
#39224=CARTESIAN_POINT('Ctrl Pts',(-22.5634994289947,10.9327137217901,-75.7391487499829));
#39225=CARTESIAN_POINT('Ctrl Pts',(-22.5824755837965,10.9083185465013,-75.6932590598033));
#39226=CARTESIAN_POINT('Ctrl Pts',(-22.6014048462052,10.8837550175016,-75.6470534899443));
#39227=CARTESIAN_POINT('Ctrl Pts',(-22.6202838428499,10.8590326983467,-75.6005500503436));
#39228=CARTESIAN_POINT('Ctrl Pts',(-22.6320499157315,10.8436248557345,-75.5715674264319));
#39229=CARTESIAN_POINT('Ctrl Pts',(-22.6437961517736,10.8281557605298,-75.5424699027608));
#39230=CARTESIAN_POINT('Ctrl Pts',(-22.6555194494533,10.8126310685817,-75.5132681220383));
#39231=CARTESIAN_POINT('Ctrl Pts',(-22.6738690250963,10.7883314630426,-75.4675608220178));
#39232=CARTESIAN_POINT('Ctrl Pts',(-22.6921652750908,10.7638918850865,-75.4215910187751));
#39233=CARTESIAN_POINT('Ctrl Pts',(-22.7104142012248,10.7393109564447,-75.3753561336587));
#39234=CARTESIAN_POINT('Ctrl Pts',(-22.7539775345839,10.6806320412672,-75.2649854905671));
#39235=CARTESIAN_POINT('Ctrl Pts',(-22.7972711094583,10.6211470908519,-75.1531032527699));
#39236=CARTESIAN_POINT('Ctrl Pts',(-22.8402166930606,10.5610049408755,-75.0399873237489));
#39237=CARTESIAN_POINT('Ctrl Pts',(-22.867492931559,10.5228065630923,-74.9681434506626));
#39238=CARTESIAN_POINT('Ctrl Pts',(-22.8946288307021,10.484343222191,-74.89580218923));
#39239=CARTESIAN_POINT('Ctrl Pts',(-22.9216048537358,10.4456543240943,-74.8230371235709));
#39240=CARTESIAN_POINT('Ctrl Pts',(-22.9418060954355,10.4166817887221,-74.7685463382969));
#39241=CARTESIAN_POINT('Ctrl Pts',(-22.9619206816493,10.3875785173637,-74.7138099023665));
#39242=CARTESIAN_POINT('Ctrl Pts',(-22.981943766366,10.3583563871592,-74.6588499300766));
#39243=CARTESIAN_POINT('Ctrl Pts',(-23.0439255439702,10.2678988177548,-74.4887204606268));
#39244=CARTESIAN_POINT('Ctrl Pts',(-23.1050288911212,10.1763036291092,-74.3164514897427));
#39245=CARTESIAN_POINT('Ctrl Pts',(-23.1650997057093,10.0839475808336,-74.1427449174312));
#39246=CARTESIAN_POINT('Ctrl Pts',(-23.2188715201287,10.0012759486535,-73.9872531427013));
#39247=CARTESIAN_POINT('Ctrl Pts',(-23.2718178159678,9.91799184453354,-73.8306041553568));
#39248=CARTESIAN_POINT('Ctrl Pts',(-23.3238195434587,9.83438895875108,-73.6733455075521));
#39249=CARTESIAN_POINT('Ctrl Pts',(-23.3543891421507,9.78524238629715,-73.5808998526444));
#39250=CARTESIAN_POINT('Ctrl Pts',(-23.3846322346305,9.73598600952977,-73.4882441891714));
#39251=CARTESIAN_POINT('Ctrl Pts',(-23.4145252260723,9.68668036351007,-73.3954914020482));
#39252=CARTESIAN_POINT('Ctrl Pts',(-23.4370059800081,9.64960049821896,-73.3257375071183));
#39253=CARTESIAN_POINT('Ctrl Pts',(-23.4592874913637,9.61249489713648,-73.2559326884176));
#39254=CARTESIAN_POINT('Ctrl Pts',(-23.4813656216018,9.57537981682306,-73.186107108416));
#39255=CARTESIAN_POINT('Ctrl Pts',(-23.4978643016036,9.54764423293412,-73.1339274225477));
#39256=CARTESIAN_POINT('Ctrl Pts',(-23.5142498889896,9.51990254705391,-73.0817346219641));
#39257=CARTESIAN_POINT('Ctrl Pts',(-23.5305218647511,9.49215930247276,-73.0295370768705));
#39258=CARTESIAN_POINT('Ctrl Pts',(-23.5427177420063,9.47136568708553,-72.9904149160266));
#39259=CARTESIAN_POINT('Ctrl Pts',(-23.5548501855968,9.45057052225198,-72.9512888220383));
#39260=CARTESIAN_POINT('Ctrl Pts',(-23.5669176669966,9.42977789958617,-72.9121664177397));
#39261=CARTESIAN_POINT('Ctrl Pts',(-23.6031521881662,9.36734476203297,-72.7946952122912));
#39262=CARTESIAN_POINT('Ctrl Pts',(-23.6387828450897,9.30496036670618,-72.6773057886921));
#39263=CARTESIAN_POINT('Ctrl Pts',(-23.6734819284684,9.24326495192996,-72.5612011682817));
#39264=CARTESIAN_POINT('',(-24.8514914924163,6.0392731730085,-66.5176718854411));
#39265=CARTESIAN_POINT('Ctrl Pts',(-23.6734819284749,9.24326495191836,-72.5612011682599));
#39266=CARTESIAN_POINT('Ctrl Pts',(-23.7649042668809,9.0816244028814,-72.257009894464));
#39267=CARTESIAN_POINT('Ctrl Pts',(-24.026191926212,8.5949110125477,-71.3440354252429));
#39268=CARTESIAN_POINT('Ctrl Pts',(-24.3676733444401,7.85042242107576,-69.9555629639005));
#39269=CARTESIAN_POINT('Ctrl Pts',(-24.6786062061593,6.94797749971677,-68.2666525661597));
#39270=CARTESIAN_POINT('Ctrl Pts',(-24.8079585801581,6.32785027214234,-67.080190599109));
#39271=CARTESIAN_POINT('Ctrl Pts',(-24.8514914924163,6.0392731730085,-66.5176718854411));
#39272=CARTESIAN_POINT('',(-24.7799130650367,2.95812473554076,-60.3565443657526));
#39273=CARTESIAN_POINT('Ctrl Pts',(-24.8514914924163,6.0392731730085,-66.5176718854411));
#39274=CARTESIAN_POINT('Ctrl Pts',(-24.9519006567039,5.4000946661346,-65.2716949090004));
#39275=CARTESIAN_POINT('Ctrl Pts',(-24.9551931519226,4.48977772329943,-63.5721308413706));
#39276=CARTESIAN_POINT('Ctrl Pts',(-24.9193282160013,4.02246798717194,-62.6314379535427));
#39277=CARTESIAN_POINT('Ctrl Pts',(-24.9088241241943,3.89449030749864,-62.3747837256354));
#39278=CARTESIAN_POINT('Ctrl Pts',(-24.9003852832803,3.80179791434547,-62.1865158010774));
#39279=CARTESIAN_POINT('Ctrl Pts',(-24.8848681816847,3.64819007810987,-61.8717738157264));
#39280=CARTESIAN_POINT('Ctrl Pts',(-24.8483424703915,3.34834435316993,-61.2421934759334));
#39281=CARTESIAN_POINT('Ctrl Pts',(-24.8095511279375,3.11147085333639,-60.7161135136638));
#39282=CARTESIAN_POINT('Ctrl Pts',(-24.7799130650367,2.95812473554075,-60.3565443657526));
#39283=CARTESIAN_POINT('',(-23.8932421744747,0.740634811882228,-53.9986859556407));
#39284=CARTESIAN_POINT('Ctrl Pts',(-24.7799130650367,2.95812473554076,-60.3565443657526));
#39285=CARTESIAN_POINT('Ctrl Pts',(-24.7093254167293,2.61894304809241,-59.562121477931));
#39286=CARTESIAN_POINT('Ctrl Pts',(-24.5694830832048,2.04316650995158,-58.1763047923767));
#39287=CARTESIAN_POINT('Ctrl Pts',(-24.3518230181499,1.42202438632593,-56.4243962709067));
#39288=CARTESIAN_POINT('Ctrl Pts',(-24.1714172775178,1.07110956737089,-55.2893749713734));
#39289=CARTESIAN_POINT('Ctrl Pts',(-24.0036588764749,0.844289079598309,
-54.4481403827476));
#39290=CARTESIAN_POINT('Ctrl Pts',(-23.8932421744747,0.740634811882228,
-53.9986859556407));
#39291=CARTESIAN_POINT('',(-18.0841506639546,0.0170011460072001,-47.6824918097827));
#39292=CARTESIAN_POINT('Ctrl Pts',(-23.8932550579139,0.73992114273642,-53.9988467607157));
#39293=CARTESIAN_POINT('Ctrl Pts',(-23.865369025631,0.713604674760589,-53.8843295077257));
#39294=CARTESIAN_POINT('Ctrl Pts',(-23.8354617846255,0.68786774595474,-53.767717765413));
#39295=CARTESIAN_POINT('Ctrl Pts',(-23.8035406699943,0.662904079149062,
-53.6495820580012));
#39296=CARTESIAN_POINT('Ctrl Pts',(-23.7715750315953,0.637905592866783,
-53.5312815741754));
#39297=CARTESIAN_POINT('Ctrl Pts',(-23.7375902175562,0.613682667000672,
-53.4114530424051));
#39298=CARTESIAN_POINT('Ctrl Pts',(-23.7016079266509,0.590379285496312,
-53.2906700249736));
#39299=CARTESIAN_POINT('Ctrl Pts',(-23.6677194403066,0.568431924558008,
-53.1769153547216));
#39300=CARTESIAN_POINT('Ctrl Pts',(-23.6320595820234,0.547299755878345,
-53.0623142112197));
#39301=CARTESIAN_POINT('Ctrl Pts',(-23.5946537465948,0.527061396986049,
-52.9473439087602));
#39302=CARTESIAN_POINT('Ctrl Pts',(-23.5472816563339,0.501430814132001,
-52.8017413982689));
#39303=CARTESIAN_POINT('Ctrl Pts',(-23.4971096480315,0.477224946459548,
-52.6555051471916));
#39304=CARTESIAN_POINT('Ctrl Pts',(-23.4435698220804,0.454449330017018,
-52.5090750461682));
#39305=CARTESIAN_POINT('Ctrl Pts',(-23.425065721271,0.44657776347449,-52.4584667876851));
#39306=CARTESIAN_POINT('Ctrl Pts',(-23.4061595713412,0.438876645481701,
-52.4078353903899));
#39307=CARTESIAN_POINT('Ctrl Pts',(-23.3868286107285,0.431344925720856,
-52.3571990316685));
#39308=CARTESIAN_POINT('Ctrl Pts',(-23.3310171351507,0.409599684917134,
-52.2110040259085));
#39309=CARTESIAN_POINT('Ctrl Pts',(-23.2716636289628,0.389270140173637,
-52.064768000871));
#39310=CARTESIAN_POINT('Ctrl Pts',(-23.2082281614495,0.370301554837552,
-51.9188967633294));
#39311=CARTESIAN_POINT('Ctrl Pts',(-23.1457449149932,0.351617704320727,
-51.7752151788231));
#39312=CARTESIAN_POINT('Ctrl Pts',(-23.0793024602032,0.334254343966579,
-51.6318879227277));
#39313=CARTESIAN_POINT('Ctrl Pts',(-23.0083890530461,0.318110160841051,
-51.4892953868701));
#39314=CARTESIAN_POINT('Ctrl Pts',(-22.9415774480444,0.302899796125833,
-51.3549507465004));
#39315=CARTESIAN_POINT('Ctrl Pts',(-22.8707983153925,0.288771253646912,
-51.2212586648078));
#39316=CARTESIAN_POINT('Ctrl Pts',(-22.7956110574691,0.275598830743189,
-51.0885250594739));
#39317=CARTESIAN_POINT('Ctrl Pts',(-22.7475861174807,0.267185106969701,
-51.0037430949938));
#39318=CARTESIAN_POINT('Ctrl Pts',(-22.6977624520621,0.259160652050131,
-50.919351922552));
#39319=CARTESIAN_POINT('Ctrl Pts',(-22.6460187082459,0.251484345223507,
-50.8354272526696));
#39320=CARTESIAN_POINT('Ctrl Pts',(-22.6384330035932,0.250358987989642,
-50.8231237795952));
#39321=CARTESIAN_POINT('Ctrl Pts',(-22.6308060202752,0.249241101953243,
-50.8108303258452));
#39322=CARTESIAN_POINT('Ctrl Pts',(-22.6231373508233,0.248130568613676,
-50.7985471282056));
#39323=CARTESIAN_POINT('Ctrl Pts',(-22.6136841630144,0.246761611418079,
-50.7834056000817));
#39324=CARTESIAN_POINT('Ctrl Pts',(-22.60416746881,0.245403845777488,-50.7682798097095));
#39325=CARTESIAN_POINT('Ctrl Pts',(-22.5945866051412,0.244057158520407,
-50.75317136449));
#39326=CARTESIAN_POINT('Ctrl Pts',(-22.520830673283,0.233690016579786,-50.6368627001968));
#39327=CARTESIAN_POINT('Ctrl Pts',(-22.4432747299908,0.223981871840293,
-50.5215841488338));
#39328=CARTESIAN_POINT('Ctrl Pts',(-22.3615976638741,0.214866063520751,
-50.4080728596082));
#39329=CARTESIAN_POINT('Ctrl Pts',(-22.2778491054295,0.205519060229424,
-50.2916826990428));
#39330=CARTESIAN_POINT('Ctrl Pts',(-22.1897679291785,0.196793847772579,
-50.1771509867835));
#39331=CARTESIAN_POINT('Ctrl Pts',(-22.0969687417925,0.188595152285034,
-50.0652405302303));
#39332=CARTESIAN_POINT('Ctrl Pts',(-22.0208828689396,0.181873057835754,
-49.9734853650389));
#39333=CARTESIAN_POINT('Ctrl Pts',(-21.9416245491178,0.175504160748907,
-49.8834916975784));
#39334=CARTESIAN_POINT('Ctrl Pts',(-21.8589623507553,0.169432268974329,
-49.7956624028172));
#39335=CARTESIAN_POINT('Ctrl Pts',(-21.7652606973502,0.162549482043352,
-49.6961035923867));
#39336=CARTESIAN_POINT('Ctrl Pts',(-21.6671931181628,0.156046312566252,
-49.5993256138718));
#39337=CARTESIAN_POINT('Ctrl Pts',(-21.5655469854621,0.149823557003932,
-49.5057302780702));
#39338=CARTESIAN_POINT('Ctrl Pts',(-21.458001267195,0.143239630013606,-49.4067026284412));
#39339=CARTESIAN_POINT('Ctrl Pts',(-21.3464479140259,0.13696833417058,-49.3112370218204));
#39340=CARTESIAN_POINT('Ctrl Pts',(-21.2317882308461,0.130930860823799,
-49.2197844474539));
#39341=CARTESIAN_POINT('Ctrl Pts',(-21.2244571308433,0.130544837422701,
-49.2139371613844));
#39342=CARTESIAN_POINT('Ctrl Pts',(-21.2171133271496,0.130159785938529,
-49.2081062754909));
#39343=CARTESIAN_POINT('Ctrl Pts',(-21.2097570538576,0.129775692478805,
-49.2022919057832));
#39344=CARTESIAN_POINT('Ctrl Pts',(-21.0990434606392,0.123994998183015,
-49.1147843136807));
#39345=CARTESIAN_POINT('Ctrl Pts',(-20.9855047073545,0.118427639898545,
-49.0310147540628));
#39346=CARTESIAN_POINT('Ctrl Pts',(-20.8699414509509,0.113046831612799,
-48.951329823701));
#39347=CARTESIAN_POINT('Ctrl Pts',(-20.7287606166067,0.106473228316489,
-48.8539806722214));
#39348=CARTESIAN_POINT('Ctrl Pts',(-20.584559314947,0.100188172347876,-48.7628237679712));
#39349=CARTESIAN_POINT('Ctrl Pts',(-20.4343295065461,0.0940004548219974,
-48.6755849178391));
#39350=CARTESIAN_POINT('Ctrl Pts',(-20.2980308949655,0.088386540269303,
-48.59643595083));
#39351=CARTESIAN_POINT('Ctrl Pts',(-20.1567727277326,0.0828531018242971,
-48.5205157941745));
#39352=CARTESIAN_POINT('Ctrl Pts',(-20.0083008190481,0.0772774204330494,
-48.4461313374821));
#39353=CARTESIAN_POINT('Ctrl Pts',(-19.9067948782763,0.0734654886671241,
-48.3952768403435));
#39354=CARTESIAN_POINT('Ctrl Pts',(-19.8019169633049,0.0696340466546913,
-48.3451415621776));
#39355=CARTESIAN_POINT('Ctrl Pts',(-19.6929361743208,0.0657592881968911,
-48.2952882858672));
#39356=CARTESIAN_POINT('Ctrl Pts',(-19.5621032696068,0.0611075884906894,
-48.235438756331));
#39357=CARTESIAN_POINT('Ctrl Pts',(-19.4254042690855,0.0563375063641562,
-48.1752852783097));
#39358=CARTESIAN_POINT('Ctrl Pts',(-19.2809513108291,0.0515296105362735,
-48.115343315774));
#39359=CARTESIAN_POINT('Ctrl Pts',(-19.2430868439431,0.0502693496557501,
-48.099631138724));
#39360=CARTESIAN_POINT('Ctrl Pts',(-19.2046894662233,0.0490066581924538,
-48.0839333380788));
#39361=CARTESIAN_POINT('Ctrl Pts',(-19.1657248392323,0.0477433954684069,
-48.068258869099));
#39362=CARTESIAN_POINT('Ctrl Pts',(-19.0876721514813,0.0452128682040143,
-48.0368602769034));
#39363=CARTESIAN_POINT('Ctrl Pts',(-19.0073434524589,0.0426798135396984,
-48.0055549360527));
#39364=CARTESIAN_POINT('Ctrl Pts',(-18.9244607930308,0.0401473901296877,
-47.9742150154492));
#39365=CARTESIAN_POINT('Ctrl Pts',(-18.7868979753429,0.0359442515930639,
-47.922199216076));
#39366=CARTESIAN_POINT('Ctrl Pts',(-18.6422965332993,0.0317435187318599,
-47.8700852781068));
#39367=CARTESIAN_POINT('Ctrl Pts',(-18.4894608715532,0.0275580329317178,
-47.8173980644618));
#39368=CARTESIAN_POINT('Ctrl Pts',(-18.3604557424757,0.0240251589301201,
-47.7729259777816));
#39369=CARTESIAN_POINT('Ctrl Pts',(-18.2255837584678,0.0205033034188778,
-47.728047397392));
#39370=CARTESIAN_POINT('Ctrl Pts',(-18.0841506697213,0.0170011623984622,
-47.6824917993401));
#39371=CARTESIAN_POINT('',(-1.26595091974945E-14,-0.0251265935465125,-45.4192972571095));
#39372=CARTESIAN_POINT('Ctrl Pts',(-18.0841506673754,0.017001162336854,
-47.682491798537));
#39373=CARTESIAN_POINT('Ctrl Pts',(-18.0828067270674,0.0169658686183399,
-47.6820317354795));
#39374=CARTESIAN_POINT('Ctrl Pts',(-18.0814621764952,0.0169305690162963,
-47.6815715039635));
#39375=CARTESIAN_POINT('Ctrl Pts',(-18.0801170157235,0.016895263522413,
-47.6811111034811));
#39376=CARTESIAN_POINT('Ctrl Pts',(-17.9371307597341,0.0131424032754297,
-47.6321720156008));
#39377=CARTESIAN_POINT('Ctrl Pts',(-17.7872420326831,0.00952942749988126,
-47.5826598841899));
#39378=CARTESIAN_POINT('Ctrl Pts',(-17.6305393229821,0.00611053317163838,
-47.5326793306452));
#39379=CARTESIAN_POINT('Ctrl Pts',(-17.4856634580748,0.0029496735172275,
-47.4864709661751));
#39380=CARTESIAN_POINT('Ctrl Pts',(-17.3349630466611,-4.50415560202498E-5,
-47.4398622491996));
#39381=CARTESIAN_POINT('Ctrl Pts',(-17.1785524330135,-0.00283268066233115,
-47.3929444476255));
#39382=CARTESIAN_POINT('Ctrl Pts',(-17.1295044874326,-0.00370684110449546,
-47.3782317518262));
#39383=CARTESIAN_POINT('Ctrl Pts',(-17.0798953942529,-0.00456066835218952,
-47.363488727926));
#39384=CARTESIAN_POINT('Ctrl Pts',(-17.0297297511583,-0.00539300427001911,
-47.3487183767908));
#39385=CARTESIAN_POINT('Ctrl Pts',(-16.8246964071324,-0.00879486670131436,
-47.2883500789106));
#39386=CARTESIAN_POINT('Ctrl Pts',(-16.6103659378757,-0.0118351451518027,
-47.2275230092626));
#39387=CARTESIAN_POINT('Ctrl Pts',(-16.3868922470239,-0.0144668416866325,
-47.1664370632235));
#39388=CARTESIAN_POINT('Ctrl Pts',(-16.2677193435885,-0.0158702593140994,
-47.1338614632913));
#39389=CARTESIAN_POINT('Ctrl Pts',(-16.1459464731934,-0.01715800953983,
-47.1012127290439));
#39390=CARTESIAN_POINT('Ctrl Pts',(-16.0215982073155,-0.0183278502655368,
-47.0685249337755));
#39391=CARTESIAN_POINT('Ctrl Pts',(-15.8252153036707,-0.0201753767822469,
-47.0169011808969));
#39392=CARTESIAN_POINT('Ctrl Pts',(-15.6224066945634,-0.0217256335218394,
-46.9651818010465));
#39393=CARTESIAN_POINT('Ctrl Pts',(-15.4151351031891,-0.0229904625177885,
-46.9138752345334));
#39394=CARTESIAN_POINT('Ctrl Pts',(-15.3369804296771,-0.0234673841092691,
-46.894529370837));
#39395=CARTESIAN_POINT('Ctrl Pts',(-15.2581911495873,-0.0239042040029462,
-46.8752424356118));
#39396=CARTESIAN_POINT('Ctrl Pts',(-15.1788721220257,-0.0243032761764485,
-46.856042448883));
#39397=CARTESIAN_POINT('Ctrl Pts',(-15.1625141020367,-0.024385577117243,
-46.8520828218382));
#39398=CARTESIAN_POINT('Ctrl Pts',(-15.1461335503751,-0.0244662757029685,
-46.8481268939813));
#39399=CARTESIAN_POINT('Ctrl Pts',(-15.1297313855253,-0.0245453974024568,
-46.8441749113411));
#39400=CARTESIAN_POINT('Ctrl Pts',(-14.9052849331823,-0.0256280950168327,
-46.7900961667706));
#39401=CARTESIAN_POINT('Ctrl Pts',(-14.6767937755882,-0.0264119003889579,
-46.7367551086416));
#39402=CARTESIAN_POINT('Ctrl Pts',(-14.4465981274285,-0.0269614391779066,
-46.684780205967));
#39403=CARTESIAN_POINT('Ctrl Pts',(-14.201003504354,-0.0275477394525454,
-46.629328433817));
#39404=CARTESIAN_POINT('Ctrl Pts',(-13.9534691875118,-0.0278679797972098,
-46.5754330516193));
#39405=CARTESIAN_POINT('Ctrl Pts',(-13.706799907371,-0.0280476913177893,
-46.523860833991));
#39406=CARTESIAN_POINT('Ctrl Pts',(-13.6210212488823,-0.0281101855738291,
-46.5059267173433));
#39407=CARTESIAN_POINT('Ctrl Pts',(-13.5353468539472,-0.0281560242974536,
-46.4882734661745));
#39408=CARTESIAN_POINT('Ctrl Pts',(-13.4498935848609,-0.0281913248931165,
-46.4709329195597));
#39409=CARTESIAN_POINT('Ctrl Pts',(-13.3947418774956,-0.0282141079667501,
-46.4597412967852));
#39410=CARTESIAN_POINT('Ctrl Pts',(-13.3396835209908,-0.0282325237416178,
-46.4486794603052));
#39411=CARTESIAN_POINT('Ctrl Pts',(-13.2846698560428,-0.0282483363564616,
-46.4377360407384));
#39412=CARTESIAN_POINT('Ctrl Pts',(-13.2687094122857,-0.0282529238775821,
-46.434561159867));
#39413=CARTESIAN_POINT('Ctrl Pts',(-13.2527527303915,-0.0282572922185099,
-46.4313962462305));
#39414=CARTESIAN_POINT('Ctrl Pts',(-13.2367986226354,-0.0282614841788263,
-46.4282410231313));
#39415=CARTESIAN_POINT('Ctrl Pts',(-13.0892763365774,-0.0283002458305825,
-46.399065732871));
#39416=CARTESIAN_POINT('Ctrl Pts',(-12.9419741004642,-0.0283241198939822,
-46.3707185504486));
#39417=CARTESIAN_POINT('Ctrl Pts',(-12.7939331331414,-0.028343224990845,
-46.3429648529121));
#39418=CARTESIAN_POINT('Ctrl Pts',(-12.5746967900316,-0.0283715180481433,
-46.3018639383091));
#39419=CARTESIAN_POINT('Ctrl Pts',(-12.3538448271959,-0.0283892866023391,
-46.262067827578));
#39420=CARTESIAN_POINT('Ctrl Pts',(-12.1347763626038,-0.0284191143890332,
-46.2243744720574));
#39421=CARTESIAN_POINT('Ctrl Pts',(-11.8709361810454,-0.0284550381751039,
-46.1789776059104));
#39422=CARTESIAN_POINT('Ctrl Pts',(-11.6097640085207,-0.0285093107968806,
-46.1366172767541));
#39423=CARTESIAN_POINT('Ctrl Pts',(-11.3508600261442,-0.0286135301320314,
-46.0971144427993));
#39424=CARTESIAN_POINT('Ctrl Pts',(-11.1830270963695,-0.0286810896813166,
-46.0715069712718));
#39425=CARTESIAN_POINT('Ctrl Pts',(-11.0161473698877,-0.028769371570055,
-46.0471003452693));
#39426=CARTESIAN_POINT('Ctrl Pts',(-10.8501566632447,-0.0288779705235915,
-46.0238381222038));
#39427=CARTESIAN_POINT('Ctrl Pts',(-10.4732223772338,-0.0291245787213677,
-45.9710139031886));
#39428=CARTESIAN_POINT('Ctrl Pts',(-10.1008720497522,-0.0294794275624165,
-45.9240905189975));
#39429=CARTESIAN_POINT('Ctrl Pts',(-9.73236090663367,-0.0298927739575285,
-45.8824064986542));
#39430=CARTESIAN_POINT('Ctrl Pts',(-9.68205671591476,-0.0299491984545376,
-45.8767163561757));
#39431=CARTESIAN_POINT('Ctrl Pts',(-9.631824073381,-0.0300066355129424,
-45.8711238535276));
#39432=CARTESIAN_POINT('Ctrl Pts',(-9.58166109168264,-0.0300648897512124,
-45.8656273191521));
#39433=CARTESIAN_POINT('Ctrl Pts',(-9.24567084642815,-0.0304550750061715,
-45.828811685983));
#39434=CARTESIAN_POINT('Ctrl Pts',(-8.91274008570343,-0.0308847456751708,
-45.7963129911165));
#39435=CARTESIAN_POINT('Ctrl Pts',(-8.57742887241812,-0.03128402910407,
-45.7671425714244));
#39436=CARTESIAN_POINT('Ctrl Pts',(-8.49902646610787,-0.0313773894820865,
-45.7603219492492));
#39437=CARTESIAN_POINT('Ctrl Pts',(-8.42049382446556,-0.0314689376095564,
-45.7536834247549));
#39438=CARTESIAN_POINT('Ctrl Pts',(-8.34176123776652,-0.0315574694580133,
-45.7472145873094));
#39439=CARTESIAN_POINT('Ctrl Pts',(-8.08715481292663,-0.0318437648582421,
-45.7262955797686));
#39440=CARTESIAN_POINT('Ctrl Pts',(-7.83048096968442,-0.0320993774944369,
-45.7071512482778));
#39441=CARTESIAN_POINT('Ctrl Pts',(-7.57169189567683,-0.0322719886806445,
-45.6895230913565));
#39442=CARTESIAN_POINT('Ctrl Pts',(-7.20190019889642,-0.0325186381331987,
-45.6643336737429));
#39443=CARTESIAN_POINT('Ctrl Pts',(-6.82778698070184,-0.0325951368515084,
-45.6422400168539));
#39444=CARTESIAN_POINT('Ctrl Pts',(-6.44939824363277,-0.0325031565777305,
-45.6225053117476));
#39445=CARTESIAN_POINT('Ctrl Pts',(-6.44444500114691,-0.0325019525233935,
-45.6222469774733));
#39446=CARTESIAN_POINT('Ctrl Pts',(-6.43949102649156,-0.0325007193835964,
-45.6219890474588));
#39447=CARTESIAN_POINT('Ctrl Pts',(-6.43453631980744,-0.0324994571456015,
-45.6217315200549));
#39448=CARTESIAN_POINT('Ctrl Pts',(-6.21842329882119,-0.0324444011990702,
-45.6104987612247));
#39449=CARTESIAN_POINT('Ctrl Pts',(-6.00090618946411,-0.0323353474729835,
-45.6000308340222));
#39450=CARTESIAN_POINT('Ctrl Pts',(-5.77560994886962,-0.0321626830075255,
-45.5899650333598));
#39451=CARTESIAN_POINT('Ctrl Pts',(-5.74279596799418,-0.0321375347473838,
-45.5884989681048));
#39452=CARTESIAN_POINT('Ctrl Pts',(-5.70981670536415,-0.0321110076321296,
-45.5870414350255));
#39453=CARTESIAN_POINT('Ctrl Pts',(-5.6766789438265,-0.0320830654558977,
-45.5855923567214));
#39454=CARTESIAN_POINT('Ctrl Pts',(-5.34325440788587,-0.0318019177044804,
-45.5710120640674));
#39455=CARTESIAN_POINT('Ctrl Pts',(-4.99378241624136,-0.0313730561290432,
-45.5572877335279));
#39456=CARTESIAN_POINT('Ctrl Pts',(-4.63509797329108,-0.0308586817011578,
-45.5443778769458));
#39457=CARTESIAN_POINT('Ctrl Pts',(-4.35532338183212,-0.0304574686063414,
-45.5343081626829));
#39458=CARTESIAN_POINT('Ctrl Pts',(-4.0699446067672,-0.0300058174109945,
-45.5247339556168));
#39459=CARTESIAN_POINT('Ctrl Pts',(-3.78220667798257,-0.0295502499152284,
-45.5156356312772));
#39460=CARTESIAN_POINT('Ctrl Pts',(-3.46861138142814,-0.0290537431650103,
-45.5057196923827));
#39461=CARTESIAN_POINT('Ctrl Pts',(-3.1522146695807,-0.0285534430926371,
-45.4963690071689));
#39462=CARTESIAN_POINT('Ctrl Pts',(-2.83714271125343,-0.0280810467641607,
-45.4875460137214));
#39463=CARTESIAN_POINT('Ctrl Pts',(-2.51852111168483,-0.0276033283578366,
-45.478623619294));
#39464=CARTESIAN_POINT('Ctrl Pts',(-2.20128569847817,-0.0271549279698236,
-45.4702550907442));
#39465=CARTESIAN_POINT('Ctrl Pts',(-1.89031005001084,-0.0267655787251769,
-45.4624340903608));
#39466=CARTESIAN_POINT('Ctrl Pts',(-1.48085910226167,-0.0262529359571283,
-45.4521364479727));
#39467=CARTESIAN_POINT('Ctrl Pts',(-1.08225782611522,-0.0258445215130111,
-45.4427883875035));
#39468=CARTESIAN_POINT('Ctrl Pts',(-0.705597976452974,-0.0255659427647448,
-45.4344166975952));
#39469=CARTESIAN_POINT('Ctrl Pts',(-0.460130518267112,-0.0253843943005195,
-45.4289609065297));
#39470=CARTESIAN_POINT('Ctrl Pts',(-0.223981908421848,-0.0252572398727827,
-45.4239198757867));
#39471=CARTESIAN_POINT('Ctrl Pts',(-0.000229628303378027,-0.025181630927626,
-45.4193011387566));
#39472=CARTESIAN_POINT('Ctrl Pts',(-0.000153083802682067,-0.025181605062196,
-45.4192995587105));
#39473=CARTESIAN_POINT('Ctrl Pts',(-7.65407527787362E-5,-0.025181579202717,
-45.4192979787138));
#39474=CARTESIAN_POINT('Ctrl Pts',(8.46174760522986E-10,-0.0251815533491883,
-45.4192963987665));
#39475=CARTESIAN_POINT('',(18.0841508193839,0.0168309156012325,-47.6825044226343));
#39476=CARTESIAN_POINT('Ctrl Pts',(-1.26595091978188E-14,-0.0251265935465125,
-45.4192972571095));
#39477=CARTESIAN_POINT('Ctrl Pts',(1.86823193664136,-0.0257297519438969,
-45.4578611092371));
#39478=CARTESIAN_POINT('Ctrl Pts',(4.99154633771575,-0.0330411937754367,
-45.5347987761651));
#39479=CARTESIAN_POINT('Ctrl Pts',(7.59438888123013,-0.0326758765092276,
-45.6867097257879));
#39480=CARTESIAN_POINT('Ctrl Pts',(8.87729659300802,-0.0314509584309369,
-45.7887336658147));
#39481=CARTESIAN_POINT('Ctrl Pts',(10.1490597186576,-0.0297979816701636,
-45.9251950972821));
#39482=CARTESIAN_POINT('Ctrl Pts',(11.8978630897578,-0.0280707333736627,
-46.1680533783691));
#39483=CARTESIAN_POINT('Ctrl Pts',(13.9971210552705,-0.0295760205187906,
-46.5641348045042));
#39484=CARTESIAN_POINT('Ctrl Pts',(16.2942224646393,-0.020912204393549,
-47.1212890230629));
#39485=CARTESIAN_POINT('Ctrl Pts',(17.5354358574236,0.00240639897730605,
-47.4946669511334));
#39486=CARTESIAN_POINT('Ctrl Pts',(18.0841508193839,0.0168309156012325,
-47.6825044226343));
#39487=CARTESIAN_POINT('',(23.8932421744751,0.740634811882458,-53.9986859556419));
#39488=CARTESIAN_POINT('Ctrl Pts',(18.084150908273,0.0167426554045659,-47.6825109477353));
#39489=CARTESIAN_POINT('Ctrl Pts',(18.1987155194437,0.0195861254427249,
-47.7194117825297));
#39490=CARTESIAN_POINT('Ctrl Pts',(18.3103943645915,0.022475540768297,-47.7564347583435));
#39491=CARTESIAN_POINT('Ctrl Pts',(18.4193445590222,0.0254026786972833,
-47.7936289577478));
#39492=CARTESIAN_POINT('Ctrl Pts',(18.5282214999332,0.0283278485420727,
-47.8307981493399));
#39493=CARTESIAN_POINT('Ctrl Pts',(18.6343735286204,0.0312907237732249,
-47.8681382921366));
#39494=CARTESIAN_POINT('Ctrl Pts',(18.7379652732147,0.0342870063881137,
-47.9057497270012));
#39495=CARTESIAN_POINT('Ctrl Pts',(18.8428315995901,0.0373201549448468,
-47.9438239289503));
#39496=CARTESIAN_POINT('Ctrl Pts',(18.9450743118358,0.040387590032794,-47.982176137475));
#39497=CARTESIAN_POINT('Ctrl Pts',(19.0448712489869,0.0434882278119365,
-48.0209637155402));
#39498=CARTESIAN_POINT('Ctrl Pts',(19.0849372612699,0.044733057512033,-48.0365359728013));
#39499=CARTESIAN_POINT('Ctrl Pts',(19.1246091311894,0.0459832720316792,
-48.0521789977961));
#39500=CARTESIAN_POINT('Ctrl Pts',(19.1638986463213,0.0472389169849191,
-48.0679052958128));
#39501=CARTESIAN_POINT('Ctrl Pts',(19.2219450831028,0.0490940102624388,
-48.0911393713815));
#39502=CARTESIAN_POINT('Ctrl Pts',(19.2791569192096,0.0509609671828519,
-48.1145554898214));
#39503=CARTESIAN_POINT('Ctrl Pts',(19.3355727469523,0.0528341973035359,
-48.1381147405902));
#39504=CARTESIAN_POINT('Ctrl Pts',(19.4950924982023,0.0581308882294921,
-48.204730191832));
#39505=CARTESIAN_POINT('Ctrl Pts',(19.6482441434888,0.063505667847821,-48.2728646408851));
#39506=CARTESIAN_POINT('Ctrl Pts',(19.7949313158912,0.0688853311200943,
-48.3422730097862));
#39507=CARTESIAN_POINT('Ctrl Pts',(19.8168881712618,0.0696905855024445,
-48.3526623948463));
#39508=CARTESIAN_POINT('Ctrl Pts',(19.8387002488627,0.0704959647465784,
-48.3630802518836));
#39509=CARTESIAN_POINT('Ctrl Pts',(19.8603672871347,0.0713012414223432,
-48.3735256732479));
#39510=CARTESIAN_POINT('Ctrl Pts',(19.9107729332328,0.0731746165749647,
-48.3978256355237));
#39511=CARTESIAN_POINT('Ctrl Pts',(19.9603936428478,0.0750473763323183,
-48.4222748738969));
#39512=CARTESIAN_POINT('Ctrl Pts',(20.0092282211876,0.0769167885082638,
-48.4468652041084));
#39513=CARTESIAN_POINT('Ctrl Pts',(20.1312063825442,0.0815861737633733,
-48.5082865036942));
#39514=CARTESIAN_POINT('Ctrl Pts',(20.2482805495917,0.0862327145344832,
-48.5705874964604));
#39515=CARTESIAN_POINT('Ctrl Pts',(20.3604266550639,0.0908485352669065,
-48.6338442430478));
#39516=CARTESIAN_POINT('Ctrl Pts',(20.5132191095433,0.0971373187799356,
-48.7200278294754));
#39517=CARTESIAN_POINT('Ctrl Pts',(20.656840047702,0.10335686552353,-48.8078118787424));
#39518=CARTESIAN_POINT('Ctrl Pts',(20.7944734247409,0.10966857806978,-48.8991351066267));
#39519=CARTESIAN_POINT('Ctrl Pts',(20.9235524482946,0.115587997544541,-48.9847823045426));
#39520=CARTESIAN_POINT('Ctrl Pts',(21.0473616598833,0.12158880846096,-49.0735382248812));
#39521=CARTESIAN_POINT('Ctrl Pts',(21.16852043031,0.127827235660881,-49.1670105943016));
#39522=CARTESIAN_POINT('Ctrl Pts',(21.1762915499337,0.128227368180087,-49.1730059090586));
#39523=CARTESIAN_POINT('Ctrl Pts',(21.1840517734182,0.1286284868762,-49.1790206427108));
#39524=CARTESIAN_POINT('Ctrl Pts',(21.1918017959379,0.129030636814078,-49.1850552271197));
#39525=CARTESIAN_POINT('Ctrl Pts',(21.199328083761,0.129421177121913,-49.1909155996592));
#39526=CARTESIAN_POINT('Ctrl Pts',(21.2068449092765,0.129812697400302,-49.1967948066722));
#39527=CARTESIAN_POINT('Ctrl Pts',(21.2143527381798,0.130205290914701,-49.2026938820643));
#39528=CARTESIAN_POINT('Ctrl Pts',(21.3057065420645,0.134982292546271,-49.2744726856844));
#39529=CARTESIAN_POINT('Ctrl Pts',(21.3957264723332,0.139915989261395,-49.3491910673921));
#39530=CARTESIAN_POINT('Ctrl Pts',(21.4852627875948,0.145185702202063,-49.4286884617553));
#39531=CARTESIAN_POINT('Ctrl Pts',(21.562654034014,0.149740609912504,-49.4974025072112));
#39532=CARTESIAN_POINT('Ctrl Pts',(21.6396835855866,0.154546101638487,-49.5696869269092));
#39533=CARTESIAN_POINT('Ctrl Pts',(21.7169214420315,0.15974196995055,-49.6467493208211));
#39534=CARTESIAN_POINT('Ctrl Pts',(21.7881410900048,0.164532987323805,-49.7178071779264));
#39535=CARTESIAN_POINT('Ctrl Pts',(21.859537466347,0.169655261283032,-49.7929273233545));
#39536=CARTESIAN_POINT('Ctrl Pts',(21.9315818076129,0.17524815142689,-49.8730760608443));
#39537=CARTESIAN_POINT('Ctrl Pts',(21.937669704384,0.175720762283621,-49.8798487959628));
#39538=CARTESIAN_POINT('Ctrl Pts',(21.9437622455401,0.176196756270345,-49.886657451252));
#39539=CARTESIAN_POINT('Ctrl Pts',(21.949859725603,0.176676230825342,-49.893502617191));
#39540=CARTESIAN_POINT('Ctrl Pts',(22.024414003266,0.182538796793058,-49.9771988977529));
#39541=CARTESIAN_POINT('Ctrl Pts',(22.0996732772509,0.188916119582828,-50.0663301976786));
#39542=CARTESIAN_POINT('Ctrl Pts',(22.1749930865905,0.195943151743774,-50.1609225259217));
#39543=CARTESIAN_POINT('Ctrl Pts',(22.2476933313007,0.202725789168989,-50.2522250062555));
#39544=CARTESIAN_POINT('Ctrl Pts',(22.320450846829,0.210113748671374,-50.3486158005322));
#39545=CARTESIAN_POINT('Ctrl Pts',(22.392684004432,0.218275564232562,-50.4501150692848));
#39546=CARTESIAN_POINT('Ctrl Pts',(22.4611591436397,0.226012751353903,-50.5463337144049));
#39547=CARTESIAN_POINT('Ctrl Pts',(22.5291638692922,0.234445737880314,-50.6471434813298));
#39548=CARTESIAN_POINT('Ctrl Pts',(22.5961888185554,0.243758120959744,-50.7525521609327));
#39549=CARTESIAN_POINT('Ctrl Pts',(22.6130295110141,0.246097950847293,-50.7790371515992));
#39550=CARTESIAN_POINT('Ctrl Pts',(22.629808243826,0.248493487950718,-50.8058124139888));
#39551=CARTESIAN_POINT('Ctrl Pts',(22.646516690491,0.250948090769253,-50.8328781574941));
#39552=CARTESIAN_POINT('Ctrl Pts',(22.668560462742,0.254186495067567,-50.8685865089402));
#39553=CARTESIAN_POINT('Ctrl Pts',(22.6904819208903,0.257527697637064,-50.9048004771956));
#39554=CARTESIAN_POINT('Ctrl Pts',(22.7122612357526,0.260980254306303,-50.9415202972099));
#39555=CARTESIAN_POINT('Ctrl Pts',(22.7799397916474,0.271708968730789,-51.0556260166503));
#39556=CARTESIAN_POINT('Ctrl Pts',(22.8462191012757,0.283510533597232,-51.1745953303357));
#39557=CARTESIAN_POINT('Ctrl Pts',(22.9109154495669,0.296586488005412,-51.2978568518167));
#39558=CARTESIAN_POINT('Ctrl Pts',(22.9743577022108,0.309408973741241,-51.4187290307513));
#39559=CARTESIAN_POINT('Ctrl Pts',(23.0362779173961,0.323458065446983,-51.5437287398601));
#39560=CARTESIAN_POINT('Ctrl Pts',(23.0964575855699,0.338924255627626,-51.6722978795863));
#39561=CARTESIAN_POINT('Ctrl Pts',(23.1552286153321,0.354028425374639,-51.7978575738595));
#39562=CARTESIAN_POINT('Ctrl Pts',(23.2123393882499,0.370485159406622,-51.9268214888112));
#39563=CARTESIAN_POINT('Ctrl Pts',(23.267543575773,0.388456337883162,-52.0586509410712));
#39564=CARTESIAN_POINT('Ctrl Pts',(23.3069283752379,0.401277670687853,-52.1527031638061));
#39565=CARTESIAN_POINT('Ctrl Pts',(23.3453417948922,0.414869550872825,-52.2482135197643));
#39566=CARTESIAN_POINT('Ctrl Pts',(23.3826821376981,0.429281525652972,-52.3449808094157));
#39567=CARTESIAN_POINT('Ctrl Pts',(23.3842895172712,0.42990191400854,-52.3491463245943));
#39568=CARTESIAN_POINT('Ctrl Pts',(23.3858949397253,0.430523824532476,-52.3533141957799));
#39569=CARTESIAN_POINT('Ctrl Pts',(23.3874984084789,0.431147263946951,-52.3574844276811));
#39570=CARTESIAN_POINT('Ctrl Pts',(23.45025399397,0.455547056824136,-52.5206964291624));
#39571=CARTESIAN_POINT('Ctrl Pts',(23.5100190844356,0.48228532595743,-52.6875245048839));
#39572=CARTESIAN_POINT('Ctrl Pts',(23.5669861146598,0.511784370525597,-52.8582128818545));
#39573=CARTESIAN_POINT('Ctrl Pts',(23.6214149651037,0.539969078043565,-53.0212961969944));
#39574=CARTESIAN_POINT('Ctrl Pts',(23.6732893711278,0.570673497582892,-53.1879034344015));
#39575=CARTESIAN_POINT('Ctrl Pts',(23.7227566502917,0.604307975088757,-53.3582474117429));
#39576=CARTESIAN_POINT('Ctrl Pts',(23.7694381353582,0.636048296892312,-53.5189983155489));
#39577=CARTESIAN_POINT('Ctrl Pts',(23.8139759842495,0.670397707363726,-53.683076977716));
#39578=CARTESIAN_POINT('Ctrl Pts',(23.856476319499,0.707744562605335,-53.8506620217186));
#39579=CARTESIAN_POINT('Ctrl Pts',(23.8689008425278,0.718662520317364,-53.8996537349901));
#39580=CARTESIAN_POINT('Ctrl Pts',(23.8811511121812,0.729836956328725,-53.9489451074243));
#39581=CARTESIAN_POINT('Ctrl Pts',(23.8932294586005,0.741278376047805,-53.998540585514));
#39582=CARTESIAN_POINT('',(24.779917851313,2.95805914746005,-60.3565719312425));
#39583=CARTESIAN_POINT('Ctrl Pts',(23.8932421744751,0.740634811882458,-53.9986859556419));
#39584=CARTESIAN_POINT('Ctrl Pts',(24.1789074622363,1.00880462386192,-55.1614948960392));
#39585=CARTESIAN_POINT('Ctrl Pts',(24.4015168304308,1.52786212045763,-56.7701588656369));
#39586=CARTESIAN_POINT('Ctrl Pts',(24.6106655417996,2.23012064092564,-58.6108222610336));
#39587=CARTESIAN_POINT('Ctrl Pts',(24.6996147992407,2.59058304170841,-59.488342199932));
#39588=CARTESIAN_POINT('Ctrl Pts',(24.7614059735443,2.86919605364059,-60.1482578252368));
#39589=CARTESIAN_POINT('Ctrl Pts',(24.7799130650375,2.95812473554106,-60.3565443657544));
#39590=CARTESIAN_POINT('',(24.8514916543763,6.03923858554143,-66.5176896450865));
#39591=CARTESIAN_POINT('Ctrl Pts',(24.779917851313,2.95805914746005,-60.3565719312425));
#39592=CARTESIAN_POINT('Ctrl Pts',(24.7799895645231,2.95843001198034,-60.3574418978072));
#39593=CARTESIAN_POINT('Ctrl Pts',(24.7800612610776,2.95880082135715,-60.3583117041383));
#39594=CARTESIAN_POINT('Ctrl Pts',(24.7801329409828,2.95917157559642,-60.3591813503334));
#39595=CARTESIAN_POINT('Ctrl Pts',(24.782850114062,2.97322577160842,-60.3921470639848));
#39596=CARTESIAN_POINT('Ctrl Pts',(24.7854889932182,2.98775170779073,-60.4260593448895));
#39597=CARTESIAN_POINT('Ctrl Pts',(24.7880733411611,3.00245300125521,-60.4602186160377));
#39598=CARTESIAN_POINT('Ctrl Pts',(24.790657689104,3.01715429471969,-60.4943778871858));
#39599=CARTESIAN_POINT('Ctrl Pts',(24.7931875024825,3.03203104417362,-60.5287843802129));
#39600=CARTESIAN_POINT('Ctrl Pts',(24.7956852978824,3.04680849773651,-60.5627893873063));
#39601=CARTESIAN_POINT('Ctrl Pts',(24.7997592646229,3.07091089392493,-60.6182524039801));
#39602=CARTESIAN_POINT('Ctrl Pts',(24.8037477026985,3.09475532602969,-60.6726623536342));
#39603=CARTESIAN_POINT('Ctrl Pts',(24.807640058142,3.1185033429446,-60.7264536078775));
#39604=CARTESIAN_POINT('Ctrl Pts',(24.8086370145993,3.1245859680175,-60.7402312648892));
#39605=CARTESIAN_POINT('Ctrl Pts',(24.8096276727509,3.13066217248865,-60.753968082751));
#39606=CARTESIAN_POINT('Ctrl Pts',(24.8106118655328,3.13673447852751,-60.7676708548502));
#39607=CARTESIAN_POINT('Ctrl Pts',(24.8175901251703,3.17978918175043,-60.8648281427549));
#39608=CARTESIAN_POINT('Ctrl Pts',(24.8242436151014,3.22264459863511,-60.9602694931683));
#39609=CARTESIAN_POINT('Ctrl Pts',(24.8305948353243,3.2651730442168,-61.0539224311071));
#39610=CARTESIAN_POINT('Ctrl Pts',(24.8333537358119,3.28364693508087,-61.0946042413853));
#39611=CARTESIAN_POINT('Ctrl Pts',(24.8360555624196,3.30205957960063,-61.1349491214377));
#39612=CARTESIAN_POINT('Ctrl Pts',(24.8387019930301,3.32040245695602,-61.1749533980223));
#39613=CARTESIAN_POINT('Ctrl Pts',(24.8473299426402,3.38020429755557,-61.3053761951255));
#39614=CARTESIAN_POINT('Ctrl Pts',(24.8553694766898,3.43926203519713,-61.4321825541305));
#39615=CARTESIAN_POINT('Ctrl Pts',(24.8628528986356,3.49756785052833,-61.5558365171184));
#39616=CARTESIAN_POINT('Ctrl Pts',(24.8707807160366,3.55933609782335,-61.6868335458274));
#39617=CARTESIAN_POINT('Ctrl Pts',(24.878084408929,3.62026073480025,-61.8142924947148));
#39618=CARTESIAN_POINT('Ctrl Pts',(24.8847959620516,3.68037730644259,-61.9387294841922));
#39619=CARTESIAN_POINT('Ctrl Pts',(24.8855286870584,3.68694045428096,-61.9523147292617));
#39620=CARTESIAN_POINT('Ctrl Pts',(24.8862543485207,3.69349401005971,-61.9658639243795));
#39621=CARTESIAN_POINT('Ctrl Pts',(24.8869729838308,3.70003804787625,-61.9793777186503));
#39622=CARTESIAN_POINT('Ctrl Pts',(24.8941500846434,3.76539417284185,-62.1143416739154));
#39623=CARTESIAN_POINT('Ctrl Pts',(24.9006269211175,3.82979673956721,-62.2457759883461));
#39624=CARTESIAN_POINT('Ctrl Pts',(24.9064352343685,3.89331878396889,-62.3742333816749));
#39625=CARTESIAN_POINT('Ctrl Pts',(24.9127907163239,3.96282488488277,-62.5147920275426));
#39626=CARTESIAN_POINT('Ctrl Pts',(24.9183457611226,4.03127715580299,-62.6517867408018));
#39627=CARTESIAN_POINT('Ctrl Pts',(24.9231341915356,4.09882908674397,-62.7859194402446));
#39628=CARTESIAN_POINT('Ctrl Pts',(24.92841190277,4.17328345990476,-62.9337577909514));
#39629=CARTESIAN_POINT('Ctrl Pts',(24.9327582355061,4.24664478696968,-63.0781198376651));
#39630=CARTESIAN_POINT('Ctrl Pts',(24.9362103791751,4.31917689646916,-63.2199133595421));
#39631=CARTESIAN_POINT('Ctrl Pts',(24.938917382834,4.37605305940895,-63.3311009633458));
#39632=CARTESIAN_POINT('Ctrl Pts',(24.9410743459718,4.432420760898,-63.4407085438744));
#39633=CARTESIAN_POINT('Ctrl Pts',(24.9426970276412,4.48842376217373,-63.5491593895862));
#39634=CARTESIAN_POINT('Ctrl Pts',(24.9449724583695,4.56695484586879,-63.7012362827417));
#39635=CARTESIAN_POINT('Ctrl Pts',(24.9461971222277,4.6447690876326,-63.8510408186009));
#39636=CARTESIAN_POINT('Ctrl Pts',(24.946407595751,4.72229821683466,-63.9997135117098));
#39637=CARTESIAN_POINT('Ctrl Pts',(24.946506062956,4.75856917642749,-64.0692680301186));
#39638=CARTESIAN_POINT('Ctrl Pts',(24.9463825550078,4.79477795245802,-64.1385740912501));
#39639=CARTESIAN_POINT('Ctrl Pts',(24.9460409903019,4.83096908536384,-64.2077445975581));
#39640=CARTESIAN_POINT('Ctrl Pts',(24.9458654050398,4.84957355311802,-64.2433024911862));
#39641=CARTESIAN_POINT('Ctrl Pts',(24.9456382269762,4.86812945857314,-64.2787402545597));
#39642=CARTESIAN_POINT('Ctrl Pts',(24.9453594450881,4.886636828798,-64.3140620599136));
#39643=CARTESIAN_POINT('Ctrl Pts',(24.9437597620407,4.9928342815915,-64.5167427061147));
#39644=CARTESIAN_POINT('Ctrl Pts',(24.9404617573982,5.09743126890092,-64.715608986053));
#39645=CARTESIAN_POINT('Ctrl Pts',(24.9354637963307,5.20042818855995,-64.9113531224432));
#39646=CARTESIAN_POINT('Ctrl Pts',(24.9341520994142,5.22745935989115,-64.9627254674158));
#39647=CARTESIAN_POINT('Ctrl Pts',(24.9327232621582,5.25438044388104,-65.0138825151559));
#39648=CARTESIAN_POINT('Ctrl Pts',(24.9311771504824,5.28119160080954,-65.0648362277982));
#39649=CARTESIAN_POINT('Ctrl Pts',(24.9292934777797,5.31385641100498,-65.1269146139212));
#39650=CARTESIAN_POINT('Ctrl Pts',(24.9272357335071,5.34635806319471,-65.1886912006868));
#39651=CARTESIAN_POINT('Ctrl Pts',(24.9250033985565,5.37869693430714,-65.2501871378648));
#39652=CARTESIAN_POINT('Ctrl Pts',(24.9227624877507,5.41116004012454,-65.3119193210633));
#39653=CARTESIAN_POINT('Ctrl Pts',(24.920345643013,5.4434591252389,-65.373368702813));
#39654=CARTESIAN_POINT('Ctrl Pts',(24.9177526911727,5.47559663338616,-65.4345600259899));
#39655=CARTESIAN_POINT('Ctrl Pts',(24.9125444975047,5.5401479157627,-65.5574686959243));
#39656=CARTESIAN_POINT('Ctrl Pts',(24.9066258928006,5.60404780990366,-65.679336808958));
#39657=CARTESIAN_POINT('Ctrl Pts',(24.8999923148938,5.66728147743902,-65.8003020279644));
#39658=CARTESIAN_POINT('Ctrl Pts',(24.8966662667709,5.69898657296373,-65.8609534811103));
#39659=CARTESIAN_POINT('Ctrl Pts',(24.893160454361,5.73052406852277,-65.9213778014053));
#39660=CARTESIAN_POINT('Ctrl Pts',(24.8894744854003,5.76189345915637,-65.9815949128062));
#39661=CARTESIAN_POINT('Ctrl Pts',(24.8876301593938,5.77758957151306,-66.0117253848127));
#39662=CARTESIAN_POINT('Ctrl Pts',(24.8857407271724,5.79324358507265,-66.0418039679763));
#39663=CARTESIAN_POINT('Ctrl Pts',(24.8838061082895,5.80885572606948,-66.0718338287028));
#39664=CARTESIAN_POINT('Ctrl Pts',(24.8818710463165,5.82447144274909,-66.101870567234));
#39665=CARTESIAN_POINT('Ctrl Pts',(24.8798907769973,5.8400452681505,-66.1318585611686));
#39666=CARTESIAN_POINT('Ctrl Pts',(24.8778652734126,5.85557623163462,-66.1617986107554));
#39667=CARTESIAN_POINT('Ctrl Pts',(24.8697941592722,5.91746315197329,-66.2811020567788));
#39668=CARTESIAN_POINT('Ctrl Pts',(24.8610049424217,5.97867070779074,-66.3996450476185));
#39669=CARTESIAN_POINT('Ctrl Pts',(24.8514916543763,6.03923858554143,-66.5176896450865));
#39670=CARTESIAN_POINT('',(23.6735115908442,9.24321250611622,-72.561102470647));
#39671=CARTESIAN_POINT('Ctrl Pts',(24.8513977161428,6.03989465182049,-66.5188833083044));
#39672=CARTESIAN_POINT('Ctrl Pts',(24.8455563449766,6.07859700744056,-66.5943232191673));
#39673=CARTESIAN_POINT('Ctrl Pts',(24.8392456975847,6.11853992684884,-66.6719944461383));
#39674=CARTESIAN_POINT('Ctrl Pts',(24.8325458971074,6.15890669998349,-66.7502957817005));
#39675=CARTESIAN_POINT('Ctrl Pts',(24.8288926950955,6.18091750125012,-66.792991172046));
#39676=CARTESIAN_POINT('Ctrl Pts',(24.8251244574647,6.20305492610137,-66.835875661678));
#39677=CARTESIAN_POINT('Ctrl Pts',(24.8212608534789,6.22518355641302,-66.8786879369743));
#39678=CARTESIAN_POINT('Ctrl Pts',(24.8195825881908,6.2347957506915,-66.8972846554272));
#39679=CARTESIAN_POINT('Ctrl Pts',(24.8178866452593,6.24440485662598,-66.9158650238878));
#39680=CARTESIAN_POINT('Ctrl Pts',(24.8161739568127,6.25400514818417,-66.9344181693235));
#39681=CARTESIAN_POINT('Ctrl Pts',(24.8089951973117,6.29424491530175,-67.0121839587378));
#39682=CARTESIAN_POINT('Ctrl Pts',(24.801517394167,6.33436121211685,-67.0895325794895));
#39683=CARTESIAN_POINT('Ctrl Pts',(24.7937073724979,6.3744931447567,-67.1667457514888));
#39684=CARTESIAN_POINT('Ctrl Pts',(24.7891659179578,6.39782948816398,-67.2116444886992));
#39685=CARTESIAN_POINT('Ctrl Pts',(24.7845119935623,6.42117111645289,-67.2564973368654));
#39686=CARTESIAN_POINT('Ctrl Pts',(24.7797378488086,6.44454552107585,-67.3013593087938));
#39687=CARTESIAN_POINT('Ctrl Pts',(24.7596506163026,6.54289341888224,-67.4901162290998));
#39688=CARTESIAN_POINT('Ctrl Pts',(24.7374303353443,6.64182229051228,-67.6790337218885));
#39689=CARTESIAN_POINT('Ctrl Pts',(24.7128946885005,6.74137185376332,-67.8683499375534));
#39690=CARTESIAN_POINT('Ctrl Pts',(24.701588943133,6.78724315362051,-67.9555846838746));
#39691=CARTESIAN_POINT('Ctrl Pts',(24.689792372908,6.83324531621845,-68.0429026099102));
#39692=CARTESIAN_POINT('Ctrl Pts',(24.6774900108944,6.87938288129889,-68.1303294426426));
#39693=CARTESIAN_POINT('Ctrl Pts',(24.6464496443559,6.99579361036991,-68.3509180524012));
#39694=CARTESIAN_POINT('Ctrl Pts',(24.6121838247661,7.11308591791533,-68.5722375519615));
#39695=CARTESIAN_POINT('Ctrl Pts',(24.5743909110932,7.23163931920386,-68.7952844661815));
#39696=CARTESIAN_POINT('Ctrl Pts',(24.5598155341771,7.27736113158979,-68.8813056942052));
#39697=CARTESIAN_POINT('Ctrl Pts',(24.544723680255,7.32324646567535,-68.9675386393311));
#39698=CARTESIAN_POINT('Ctrl Pts',(24.5290841934132,7.36936421298444,-69.0541220985275));
#39699=CARTESIAN_POINT('Ctrl Pts',(24.5054539641581,7.43904507608807,-69.1849439733877));
#39700=CARTESIAN_POINT('Ctrl Pts',(24.480574481159,7.50925615086605,-69.3165654178659));
#39701=CARTESIAN_POINT('Ctrl Pts',(24.454478968152,7.58001729247573,-69.4490443969127));
#39702=CARTESIAN_POINT('Ctrl Pts',(24.4490308268951,7.5947905868306,-69.4767029522832));
#39703=CARTESIAN_POINT('Ctrl Pts',(24.4435290302948,7.60958954672013,-69.5044018522722));
#39704=CARTESIAN_POINT('Ctrl Pts',(24.4379734711635,7.62441430239803,-69.5321434571217));
#39705=CARTESIAN_POINT('Ctrl Pts',(24.4345989630252,7.63341902316507,-69.5489940151158));
#39706=CARTESIAN_POINT('Ctrl Pts',(24.4312055161453,7.64243086407736,-69.565855843189));
#39707=CARTESIAN_POINT('Ctrl Pts',(24.4277933102453,7.65144951807085,-69.582728481914));
#39708=CARTESIAN_POINT('Ctrl Pts',(24.3862613384946,7.76122087825921,-69.7880953253642));
#39709=CARTESIAN_POINT('Ctrl Pts',(24.3419502429364,7.87199934178849,-69.9950599001169));
#39710=CARTESIAN_POINT('Ctrl Pts',(24.2951968906539,7.98321493822236,-70.2027569600603));
#39711=CARTESIAN_POINT('Ctrl Pts',(24.2446138727013,8.10354043867051,-70.4274669241358));
#39712=CARTESIAN_POINT('Ctrl Pts',(24.1911719768325,8.2243777484948,-70.6530368414904));
#39713=CARTESIAN_POINT('Ctrl Pts',(24.1352980932057,8.34503713068008,-70.8784046499643));
#39714=CARTESIAN_POINT('Ctrl Pts',(24.0817771124609,8.46061543044053,-71.0942820036554));
#39715=CARTESIAN_POINT('Ctrl Pts',(24.0260241432573,8.57603160210702,-71.3099765369464));
#39716=CARTESIAN_POINT('Ctrl Pts',(23.9684197384083,8.69069685263161,-71.5245442088329));
#39717=CARTESIAN_POINT('Ctrl Pts',(23.9153048804812,8.79642537298955,-71.7223889993114));
#39718=CARTESIAN_POINT('Ctrl Pts',(23.8606155216188,8.90151629720597,-71.9192768214147));
#39719=CARTESIAN_POINT('Ctrl Pts',(23.8046611444706,9.00550935262722,-72.1144338489968));
#39720=CARTESIAN_POINT('Ctrl Pts',(23.761660871844,9.08542677754184,-72.2644097010878));
#39721=CARTESIAN_POINT('Ctrl Pts',(23.7179136506019,9.16470432536132,-72.4133583231326));
#39722=CARTESIAN_POINT('Ctrl Pts',(23.673567339905,9.24311393663887,-72.5609169730204));
#39723=CARTESIAN_POINT('',(21.0430574415837,12.442190173977,-78.5797217830346));
#39724=CARTESIAN_POINT('Ctrl Pts',(23.6734819284753,9.2432649519181,-72.5612011682563));
#39725=CARTESIAN_POINT('Ctrl Pts',(23.5615106118548,9.44235138733137,-72.9358619934788));
#39726=CARTESIAN_POINT('Ctrl Pts',(23.2106747185919,10.0332017364569,-74.0473320232884));
#39727=CARTESIAN_POINT('Ctrl Pts',(22.4162563803382,11.1958361188247,-76.2337986537702));
#39728=CARTESIAN_POINT('Ctrl Pts',(21.6377011779931,12.0078686581778,-77.7620529729162));
#39729=CARTESIAN_POINT('Ctrl Pts',(21.0430574415837,12.442190173977,-78.5797217830346));
#39730=CARTESIAN_POINT('',(20.8093219137291,12.6047243941762,-78.8857197857179));
#39731=CARTESIAN_POINT('Ctrl Pts',(21.0430574363752,12.4421970963867,-78.5797181023401));
#39732=CARTESIAN_POINT('Ctrl Pts',(20.966393338375,12.4981910797977,-78.6851364132037));
#39733=CARTESIAN_POINT('Ctrl Pts',(20.8885043059515,12.5523874433895,-78.7871760259047));
#39734=CARTESIAN_POINT('Ctrl Pts',(20.8093219137031,12.6047243946578,-78.8857197854716));
#39735=CARTESIAN_POINT('',(25.7013491764599,12.8213346415145,-79.293640964296));
#39736=CARTESIAN_POINT('Ctrl Pts',(20.8093219137031,12.6047243946579,-78.8857197854716));
#39737=CARTESIAN_POINT('Ctrl Pts',(20.7840585047214,12.6878774354483,-79.0421442877749));
#39738=CARTESIAN_POINT('Ctrl Pts',(20.7688933687643,12.7738276928524,-79.2038152925502));
#39739=CARTESIAN_POINT('Ctrl Pts',(20.7703883247029,12.8593245421261,-79.3646100531889));
#39740=CARTESIAN_POINT('Ctrl Pts',(20.7718832806414,12.9448213913999,-79.5254048138275));
#39741=CARTESIAN_POINT('Ctrl Pts',(20.7900383284828,13.0298648236847,-79.6853233350397));
#39742=CARTESIAN_POINT('Ctrl Pts',(20.8316864377639,13.1115279871602,-79.8388510633934));
#39743=CARTESIAN_POINT('Ctrl Pts',(20.8733345470451,13.1931911506358,-79.9923787917472));
#39744=CARTESIAN_POINT('Ctrl Pts',(20.9384757176957,13.2714741339522,-80.1395156801066));
#39745=CARTESIAN_POINT('Ctrl Pts',(21.0312181697793,13.3423337920754,-80.2726523540952));
#39746=CARTESIAN_POINT('Ctrl Pts',(21.1239606218628,13.4131934501986,-80.4057890280839));
#39747=CARTESIAN_POINT('Ctrl Pts',(21.2443043552774,13.4766299304238,-80.5249254093838));
#39748=CARTESIAN_POINT('Ctrl Pts',(21.3835931186265,13.5285264211225,-80.6223375406638));
#39749=CARTESIAN_POINT('Ctrl Pts',(21.4184153094637,13.5415005437972,-80.6466905734838));
#39750=CARTESIAN_POINT('Ctrl Pts',(21.4544215646831,13.5537534008702,-80.6696858493211));
#39751=CARTESIAN_POINT('Ctrl Pts',(21.4915342779707,13.5654172411284,-80.6915723859151));
#39752=CARTESIAN_POINT('Ctrl Pts',(21.5286469912584,13.5770810813866,-80.7134589225092));
#39753=CARTESIAN_POINT('Ctrl Pts',(21.5668661626148,13.5881559038188,-80.7342367203975));
#39754=CARTESIAN_POINT('Ctrl Pts',(21.6059140724305,13.5985438937157,-80.7537224018477));
#39755=CARTESIAN_POINT('Ctrl Pts',(21.6840098920621,13.6193198735095,-80.7926937647481));
#39756=CARTESIAN_POINT('Ctrl Pts',(21.7654206655389,13.6373485207903,-80.826496663157));
#39757=CARTESIAN_POINT('Ctrl Pts',(21.8485678910789,13.6530496506021,-80.8559244908226));
#39758=CARTESIAN_POINT('Ctrl Pts',(22.014862342159,13.6844519102255,-80.9147801461538));
#39759=CARTESIAN_POINT('Ctrl Pts',(22.1881026013518,13.7065442425174,-80.9561354427192));
#39760=CARTESIAN_POINT('Ctrl Pts',(22.3667510409472,13.7214448954529,-80.9839923851256));
#39761=CARTESIAN_POINT('Ctrl Pts',(22.4282524899153,13.7265745889906,-80.9935824063185));
#39762=CARTESIAN_POINT('Ctrl Pts',(22.490395192073,13.7308519682516,-81.0015727254715));
#39763=CARTESIAN_POINT('Ctrl Pts',(22.5528649735285,13.7343255298831,-81.0080555375436));
#39764=CARTESIAN_POINT('Ctrl Pts',(22.6718564286154,13.7409419153296,-81.0204038957984));
#39765=CARTESIAN_POINT('Ctrl Pts',(22.7920344808733,13.7446418002757,-81.0272827150941));
#39766=CARTESIAN_POINT('Ctrl Pts',(22.9112327926434,13.7457620573825,-81.0293291152419));
#39767=CARTESIAN_POINT('Ctrl Pts',(23.0930094843542,13.7474704425745,-81.0324498628704));
#39768=CARTESIAN_POINT('Ctrl Pts',(23.2725062469405,13.7431799593285,-81.024331855367));
#39769=CARTESIAN_POINT('Ctrl Pts',(23.453334415982,13.7329853385207,-81.0051586905715));
#39770=CARTESIAN_POINT('Ctrl Pts',(23.7245766695442,13.717693407309,-80.9763989433782));
#39771=CARTESIAN_POINT('Ctrl Pts',(23.9988145883369,13.6891140752413,-80.9227667359737));
#39772=CARTESIAN_POINT('Ctrl Pts',(24.2566884728839,13.645897639705,-80.8417199326631));
#39773=CARTESIAN_POINT('Ctrl Pts',(24.5145623574308,13.6026812041686,-80.7606731293525));
#39774=CARTESIAN_POINT('Ctrl Pts',(24.7560722095976,13.544828389164,-80.6522113451778));
#39775=CARTESIAN_POINT('Ctrl Pts',(24.9680647929619,13.4679875742907,-80.5080837891733));
#39776=CARTESIAN_POINT('Ctrl Pts',(25.1093931818714,13.4167603643751,-80.4119987518369));
#39777=CARTESIAN_POINT('Ctrl Pts',(25.2376027841621,13.3570942619928,-80.3000621441297));
#39778=CARTESIAN_POINT('Ctrl Pts',(25.3433331128627,13.289655597635,-80.1734804456779));
#39779=CARTESIAN_POINT('Ctrl Pts',(25.3519347957313,13.2841691302135,-80.1631824012054));
#39780=CARTESIAN_POINT('Ctrl Pts',(25.3603876963185,13.2786312235604,-80.1527874266039));
#39781=CARTESIAN_POINT('Ctrl Pts',(25.3686909709012,13.2730439238718,-80.1422993517087));
#39782=CARTESIAN_POINT('Ctrl Pts',(25.4624500443877,13.2099531472293,-80.0238699085973));
#39783=CARTESIAN_POINT('Ctrl Pts',(25.5371310844642,13.1405649390909,-79.8935692943807));
#39784=CARTESIAN_POINT('Ctrl Pts',(25.5915191111769,13.0678252000338,-79.7569144572679));
#39785=CARTESIAN_POINT('Ctrl Pts',(25.6507237247329,12.9886436521574,-79.6081575099976));
#39786=CARTESIAN_POINT('Ctrl Pts',(25.6858818958191,12.9054906353473,-79.4518710147319));
#39787=CARTESIAN_POINT('Ctrl Pts',(25.7013238222668,12.8213719704933,-79.2937110989762));
#39788=CARTESIAN_POINT('',(25.9521939529868,12.4413326875396,-78.5797156137649));
#39789=CARTESIAN_POINT('Ctrl Pts',(25.7013815084256,12.8212870391611,-79.293551527726));
#39790=CARTESIAN_POINT('Ctrl Pts',(25.7859000295341,12.6968486583446,-79.0597595468301));
#39791=CARTESIAN_POINT('Ctrl Pts',(25.8695209159813,12.5699441739082,-78.8213395443483));
#39792=CARTESIAN_POINT('Ctrl Pts',(25.952193952974,12.4413326879221,-78.5797156136114));
#39793=CARTESIAN_POINT('',(27.8032099026773,9.23603570625547,-72.5577783044314));
#39794=CARTESIAN_POINT('Ctrl Pts',(25.9521939530147,12.4413326882658,-78.5797156132792));
#39795=CARTESIAN_POINT('Ctrl Pts',(26.1287870546047,12.1667972870379,-78.0639430465837));
#39796=CARTESIAN_POINT('Ctrl Pts',(26.2992662638511,11.8864855960595,-77.5377185702874));
#39797=CARTESIAN_POINT('Ctrl Pts',(26.6249152504807,11.3331555384472,-76.4994184116619));
#39798=CARTESIAN_POINT('Ctrl Pts',(26.7835000842749,11.0543284251978,-75.9764391079278));
#39799=CARTESIAN_POINT('Ctrl Pts',(27.0855446094684,10.5155281999478,-74.9654367676289));
#39800=CARTESIAN_POINT('Ctrl Pts',(27.2314148704176,10.2516696780351,-74.470116440961));
#39801=CARTESIAN_POINT('Ctrl Pts',(27.4390175574596,9.87838321168263,-73.7683380431596));
#39802=CARTESIAN_POINT('Ctrl Pts',(27.5122084373452,9.74719436950816,-73.5215103039169));
#39803=CARTESIAN_POINT('Ctrl Pts',(27.620165889337,9.55564988556187,-73.1607059454969));
#39804=CARTESIAN_POINT('Ctrl Pts',(27.6566443739694,9.49125974573235,-73.0393458765082));
#39805=CARTESIAN_POINT('Ctrl Pts',(27.7114876925037,9.39517048279879,-72.858114884868));
#39806=CARTESIAN_POINT('Ctrl Pts',(27.7298944275117,9.36304055589236,-72.797494717765));
#39807=CARTESIAN_POINT('Ctrl Pts',(27.7708537404106,9.29185801117427,-72.6631426458087));
#39808=CARTESIAN_POINT('Ctrl Pts',(27.789295348826,9.26001909606324,-72.6030135173959));
#39809=CARTESIAN_POINT('Ctrl Pts',(27.8032099492931,9.23606309930771,-72.5577638163968));
#39810=CARTESIAN_POINT('',(30.3753540341101,6.01695723880264,-66.3794227429407));
#39811=CARTESIAN_POINT('Ctrl Pts',(27.8032099026773,9.23603570625547,-72.5577783044314));
#39812=CARTESIAN_POINT('Ctrl Pts',(28.1510242423018,8.65285503600956,-71.4562837782078));
#39813=CARTESIAN_POINT('Ctrl Pts',(28.8443112604251,7.45365732155485,-69.2995688107867));
#39814=CARTESIAN_POINT('Ctrl Pts',(29.7346820906896,6.49856484963839,-67.5354860661677));
#39815=CARTESIAN_POINT('Ctrl Pts',(30.3753540341101,6.01695723880264,-66.3794227429407));
#39816=CARTESIAN_POINT('',(33.2873624690393,4.35252899916091,-59.9316190686982));
#39817=CARTESIAN_POINT('Ctrl Pts',(30.3753540341101,6.01695723880265,-66.3794227429407));
#39818=CARTESIAN_POINT('Ctrl Pts',(30.7734090781721,5.72447094290213,-65.6771164512212));
#39819=CARTESIAN_POINT('Ctrl Pts',(31.4978217512257,5.28838679537279,-64.4647865749015));
#39820=CARTESIAN_POINT('Ctrl Pts',(32.3856289559011,4.77997444759906,-62.3963211915439));
#39821=CARTESIAN_POINT('Ctrl Pts',(32.8375602373923,4.5442896682234,-61.1512919674956));
#39822=CARTESIAN_POINT('Ctrl Pts',(33.0921495677964,4.42939107495768,-60.4613459843507));
#39823=CARTESIAN_POINT('Ctrl Pts',(33.2133445958773,4.37993836178462,-60.1301142016715));
#39824=CARTESIAN_POINT('Ctrl Pts',(33.2870419060244,4.35253527707261,-59.9326413364725));
#39825=CARTESIAN_POINT('',(36.1829914186425,4.79767940081217,-53.6562556717971));
#39826=CARTESIAN_POINT('Ctrl Pts',(33.2879498115781,4.35251749663435,-59.9297460474139));
#39827=CARTESIAN_POINT('Ctrl Pts',(33.3193429188025,4.33924707865741,-59.836759691682));
#39828=CARTESIAN_POINT('Ctrl Pts',(33.3527820526142,4.32635858806945,-59.7387076557157));
#39829=CARTESIAN_POINT('Ctrl Pts',(33.3885290935015,4.31421583300761,-59.635464898597));
#39830=CARTESIAN_POINT('Ctrl Pts',(33.4236835691159,4.30227436383656,-59.5339335578932));
#39831=CARTESIAN_POINT('Ctrl Pts',(33.4610701996642,4.29105457425154,-59.4273816074148));
#39832=CARTESIAN_POINT('Ctrl Pts',(33.5009269768532,4.28094099462918,-59.3157162971264));
#39833=CARTESIAN_POINT('Ctrl Pts',(33.5397082187402,4.27110032999598,-59.2070642757114));
#39834=CARTESIAN_POINT('Ctrl Pts',(33.5808284261384,4.2623077625252,-59.0935703856562));
#39835=CARTESIAN_POINT('Ctrl Pts',(33.6244906665991,4.25496188680782,-58.9751811881067));
#39836=CARTESIAN_POINT('Ctrl Pts',(33.6651578575728,4.24811990784578,-58.8649130008777));
#39837=CARTESIAN_POINT('Ctrl Pts',(33.7080229607883,4.24258396476386,-58.7503927918472));
#39838=CARTESIAN_POINT('Ctrl Pts',(33.7532493913408,4.2385859318034,-58.6316247260045));
#39839=CARTESIAN_POINT('Ctrl Pts',(33.7781485708435,4.23638483525158,-58.5662375761791));
#39840=CARTESIAN_POINT('Ctrl Pts',(33.8037624161283,4.23464993176182,-58.4995656615771));
#39841=CARTESIAN_POINT('Ctrl Pts',(33.830116374127,4.23342993811555,-58.431608832582));
#39842=CARTESIAN_POINT('Ctrl Pts',(33.8772223557387,4.23124927901796,-58.3101404316232));
#39843=CARTESIAN_POINT('Ctrl Pts',(33.9266919107457,4.23071374517117,-58.1845694789117));
#39844=CARTESIAN_POINT('Ctrl Pts',(33.9787951067483,4.23218950266131,-58.0550320213901));
#39845=CARTESIAN_POINT('Ctrl Pts',(34.0170138421718,4.23327200026974,-57.9600137078069));
#39846=CARTESIAN_POINT('Ctrl Pts',(34.0566502834616,4.23543688539143,-57.8628598169221));
#39847=CARTESIAN_POINT('Ctrl Pts',(34.0977995205523,4.23882699399173,-57.7636506686872));
#39848=CARTESIAN_POINT('Ctrl Pts',(34.1105235373635,4.23987527099202,-57.732973578194));
#39849=CARTESIAN_POINT('Ctrl Pts',(34.1233921062565,4.24104067164571,-57.7021001731857));
#39850=CARTESIAN_POINT('Ctrl Pts',(34.1364078860249,4.24232734701405,-57.6710331046924));
#39851=CARTESIAN_POINT('Ctrl Pts',(34.1493998562702,4.24361166869114,-57.6400228666078));
#39852=CARTESIAN_POINT('Ctrl Pts',(34.1625348460402,4.24501644543468,-57.6088283708759));
#39853=CARTESIAN_POINT('Ctrl Pts',(34.1758182484859,4.24654595697531,-57.5774455065173));
#39854=CARTESIAN_POINT('Ctrl Pts',(34.1922641067537,4.24843960810267,-57.5385911436089));
#39855=CARTESIAN_POINT('Ctrl Pts',(34.2089380837605,4.25052449795675,-57.49944651308));
#39856=CARTESIAN_POINT('Ctrl Pts',(34.2258536530513,4.25280960171236,-57.4599968745805));
#39857=CARTESIAN_POINT('Ctrl Pts',(34.2390115898942,4.25458709145444,-57.4293105971679));
#39858=CARTESIAN_POINT('Ctrl Pts',(34.2523157279084,4.25648573961938,-57.3984397369432));
#39859=CARTESIAN_POINT('Ctrl Pts',(34.26575497327,4.25850063205734,-57.3674086665775));
#39860=CARTESIAN_POINT('Ctrl Pts',(34.2781317989214,4.26035624014695,-57.3388307116878));
#39861=CARTESIAN_POINT('Ctrl Pts',(34.2906222853231,4.26231024523409,-57.3101189316576));
#39862=CARTESIAN_POINT('Ctrl Pts',(34.3032320058153,4.2643614058939,-57.281260241763));
#39863=CARTESIAN_POINT('Ctrl Pts',(34.3353173948163,4.26958057690682,-57.2078294078357));
#39864=CARTESIAN_POINT('Ctrl Pts',(34.3681640087544,4.2754259772561,-57.1334699365933));
#39865=CARTESIAN_POINT('Ctrl Pts',(34.4017682786756,4.28187637012116,-57.0582108210068));
#39866=CARTESIAN_POINT('Ctrl Pts',(34.4086934361437,4.28320566507165,-57.0427014459315));
#39867=CARTESIAN_POINT('Ctrl Pts',(34.415650780798,4.28456071279837,-57.027153953167));
#39868=CARTESIAN_POINT('Ctrl Pts',(34.4226403295208,4.28594142333925,-57.0115686651073));
#39869=CARTESIAN_POINT('Ctrl Pts',(34.4258994958212,4.28658523675896,-57.0043013796729));
#39870=CARTESIAN_POINT('Ctrl Pts',(34.429167321032,4.28723496733483,-56.9970222000307));
#39871=CARTESIAN_POINT('Ctrl Pts',(34.4324324617172,4.28788832163034,-56.9897563806894));
#39872=CARTESIAN_POINT('Ctrl Pts',(34.4652349505291,4.29445209606898,-56.9167619891382));
#39873=CARTESIAN_POINT('Ctrl Pts',(34.4979753191527,4.30142033433672,-56.8446463818856));
#39874=CARTESIAN_POINT('Ctrl Pts',(34.5306719667931,4.30874438156103,-56.7733274368403));
#39875=CARTESIAN_POINT('Ctrl Pts',(34.5600103523251,4.31531617826277,-56.7093336375833));
#39876=CARTESIAN_POINT('Ctrl Pts',(34.5893154621551,4.32217536766797,-56.6459775876097));
#39877=CARTESIAN_POINT('Ctrl Pts',(34.6186155012557,4.32930500506736,-56.5831926500093));
#39878=CARTESIAN_POINT('Ctrl Pts',(34.6267458294818,4.33128337417434,-56.5657707568646));
#39879=CARTESIAN_POINT('Ctrl Pts',(34.6348759116403,4.33328266952345,-56.548392652979));
#39880=CARTESIAN_POINT('Ctrl Pts',(34.6430101831854,4.33530366538436,-56.5310491039294));
#39881=CARTESIAN_POINT('Ctrl Pts',(34.6641901616557,4.34056592502068,-56.4858900514644));
#39882=CARTESIAN_POINT('Ctrl Pts',(34.685388439502,4.34597281030537,-56.4409868113198));
#39883=CARTESIAN_POINT('Ctrl Pts',(34.7065762247373,4.35151265306868,-56.3964075588278));
#39884=CARTESIAN_POINT('Ctrl Pts',(34.7269322203096,4.35683501279193,-56.353578397768));
#39885=CARTESIAN_POINT('Ctrl Pts',(34.7472784056529,4.3622800874029,-56.3110485760468));
#39886=CARTESIAN_POINT('Ctrl Pts',(34.7676538333411,4.36784902616682,-56.268736385199));
#39887=CARTESIAN_POINT('Ctrl Pts',(34.7779097223884,4.3706521289506,-56.2474387152152));
#39888=CARTESIAN_POINT('Ctrl Pts',(34.7881730263819,4.37348662257477,-56.2261961965177));
#39889=CARTESIAN_POINT('Ctrl Pts',(34.7984487796813,4.3763527052992,-56.2049984515675));
#39890=CARTESIAN_POINT('Ctrl Pts',(34.8084407611364,4.37913963921997,-56.1843860966128));
#39891=CARTESIAN_POINT('Ctrl Pts',(34.8184407814739,4.38195540987727,-56.1638238008178));
#39892=CARTESIAN_POINT('Ctrl Pts',(34.8284479955918,4.38479857514819,-56.1433131111396));
#39893=CARTESIAN_POINT('Ctrl Pts',(34.8744185960652,4.39785935442295,-56.0490922111449));
#39894=CARTESIAN_POINT('Ctrl Pts',(34.920552158193,4.41150287932467,-55.9559411034495));
#39895=CARTESIAN_POINT('Ctrl Pts',(34.966934193085,4.42562295944024,-55.8636347575493));
#39896=CARTESIAN_POINT('Ctrl Pts',(35.0057045413381,4.43742581424635,-55.7864766685424));
#39897=CARTESIAN_POINT('Ctrl Pts',(35.0446482571423,4.44956094597523,-55.7099084471863));
#39898=CARTESIAN_POINT('Ctrl Pts',(35.0838003791657,4.4619543730562,-55.6338032881274));
#39899=CARTESIAN_POINT('Ctrl Pts',(35.1033921354031,4.46815605484938,-55.5957201997113));
#39900=CARTESIAN_POINT('Ctrl Pts',(35.1230360065799,4.47442231987154,-55.5577528539355));
#39901=CARTESIAN_POINT('Ctrl Pts',(35.1427351931354,4.48074331663663,-55.5198857676554));
#39902=CARTESIAN_POINT('Ctrl Pts',(35.1515556497795,4.48357358974243,-55.5029304993841));
#39903=CARTESIAN_POINT('Ctrl Pts',(35.1603865099301,4.48641461662677,-55.4859966435756));
#39904=CARTESIAN_POINT('Ctrl Pts',(35.16922544088,4.48926466526989,-55.469087709146));
#39905=CARTESIAN_POINT('Ctrl Pts',(35.1800953274311,4.49276958069363,-55.4482935429746));
#39906=CARTESIAN_POINT('Ctrl Pts',(35.1909797949457,4.49628889993367,-55.4275324894031));
#39907=CARTESIAN_POINT('Ctrl Pts',(35.2018857234225,4.49982305678331,-55.4067896722193));
#39908=CARTESIAN_POINT('Ctrl Pts',(35.2251618051249,4.50736586469342,-55.3625191171226));
#39909=CARTESIAN_POINT('Ctrl Pts',(35.2485353596057,4.5149761197521,-55.3183319108149));
#39910=CARTESIAN_POINT('Ctrl Pts',(35.2719897294641,4.52263364313067,-55.274239624144));
#39911=CARTESIAN_POINT('Ctrl Pts',(35.2874168173186,4.52767037132342,-55.2452379675536));
#39912=CARTESIAN_POINT('Ctrl Pts',(35.3028783324909,4.53272739361122,-55.2162784591772));
#39913=CARTESIAN_POINT('Ctrl Pts',(35.3183720972909,4.53779994429228,-55.1873604599376));
#39914=CARTESIAN_POINT('Ctrl Pts',(35.3567990507267,4.55038066120243,-55.1156393111672));
#39915=CARTESIAN_POINT('Ctrl Pts',(35.3954510211321,4.56306580132258,-55.0441217312217));
#39916=CARTESIAN_POINT('Ctrl Pts',(35.4343467852101,4.57579980706008,-54.972723810768));
#39917=CARTESIAN_POINT('Ctrl Pts',(35.4580836639989,4.58357097592261,-54.9291518737267));
#39918=CARTESIAN_POINT('Ctrl Pts',(35.4819130032678,4.59136089096042,-54.8856219885748));
#39919=CARTESIAN_POINT('Ctrl Pts',(35.5058437810806,4.59915739223225,-54.8421114637831));
#39920=CARTESIAN_POINT('Ctrl Pts',(35.5166852243627,4.60268946824744,-54.8223997398101));
#39921=CARTESIAN_POINT('Ctrl Pts',(35.5275474313267,4.6062228600002,-54.8026921414144));
#39922=CARTESIAN_POINT('Ctrl Pts',(35.5384308800317,4.60975620962218,-54.7829874465923));
#39923=CARTESIAN_POINT('Ctrl Pts',(35.5428940276423,4.6112051860772,-54.7749068313391));
#39924=CARTESIAN_POINT('Ctrl Pts',(35.5473607443006,4.61265415344328,-54.7668267117997));
#39925=CARTESIAN_POINT('Ctrl Pts',(35.5518310486815,4.61410300911227,-54.7587470363111));
#39926=CARTESIAN_POINT('Ctrl Pts',(35.5559724443439,4.61544526325692,-54.7512618339241));
#39927=CARTESIAN_POINT('Ctrl Pts',(35.56011966303,4.61678830788818,-54.7437720684435));
#39928=CARTESIAN_POINT('Ctrl Pts',(35.5642570127954,4.61812698146163,-54.7363060240264));
#39929=CARTESIAN_POINT('Ctrl Pts',(35.604680894705,4.63120646120528,-54.663359206628));
#39930=CARTESIAN_POINT('Ctrl Pts',(35.6444001071669,4.64394591788954,-54.5922440303002));
#39931=CARTESIAN_POINT('Ctrl Pts',(35.6834479721225,4.65628937713368,-54.5228259069607));
#39932=CARTESIAN_POINT('Ctrl Pts',(35.695230871715,4.66001408118762,-54.5018786214141));
#39933=CARTESIAN_POINT('Ctrl Pts',(35.7069525999216,4.66370269122389,-54.4810861717907));
#39934=CARTESIAN_POINT('Ctrl Pts',(35.718613806074,4.66735348114836,-54.460445910469));
#39935=CARTESIAN_POINT('Ctrl Pts',(35.7417218506995,4.67458794861172,-54.4195448172657));
#39936=CARTESIAN_POINT('Ctrl Pts',(35.7645949778937,4.68167474578746,-54.3792365323959));
#39937=CARTESIAN_POINT('Ctrl Pts',(35.7872336535589,4.68860586750444,-54.3394930764735));
#39938=CARTESIAN_POINT('Ctrl Pts',(35.8109318354677,4.69586137068449,-54.2978895983346));
#39939=CARTESIAN_POINT('Ctrl Pts',(35.8343776374465,4.70294759661248,-54.2568972277437));
#39940=CARTESIAN_POINT('Ctrl Pts',(35.8575430046428,4.70984679047995,-54.2165339087682));
#39941=CARTESIAN_POINT('Ctrl Pts',(35.8863332239078,4.71842119823762,-54.1663698516339));
#39942=CARTESIAN_POINT('Ctrl Pts',(35.9146885521825,4.72670608754568,-54.1171804254787));
#39943=CARTESIAN_POINT('Ctrl Pts',(35.9425539712792,4.73466916979316,-54.0690003817303));
#39944=CARTESIAN_POINT('Ctrl Pts',(35.9557139144567,4.73842987798603,-54.0462464932703));
#39945=CARTESIAN_POINT('Ctrl Pts',(35.9687646274413,4.74211885856277,-54.0237176519991));
#39946=CARTESIAN_POINT('Ctrl Pts',(35.981699463113,4.7457327148002,-54.001418937057));
#39947=CARTESIAN_POINT('Ctrl Pts',(35.9904281226407,4.7481714099239,-53.9863713635451));
#39948=CARTESIAN_POINT('Ctrl Pts',(35.9991021184289,4.75057538140656,-53.9714318441434));
#39949=CARTESIAN_POINT('Ctrl Pts',(36.0077274345209,4.75294583366281,-53.9565881348688));
#39950=CARTESIAN_POINT('Ctrl Pts',(36.0300298181379,4.75907508562308,-53.9182069213559));
#39951=CARTESIAN_POINT('Ctrl Pts',(36.0520201758314,4.76498481343368,-53.880442836908));
#39952=CARTESIAN_POINT('Ctrl Pts',(36.0739039034926,4.77071695984771,-53.8429123359909));
#39953=CARTESIAN_POINT('Ctrl Pts',(36.082315379934,4.77292023230962,-53.8284866892645));
#39954=CARTESIAN_POINT('Ctrl Pts',(36.0907111626026,4.77509715849289,-53.8140954911172));
#39955=CARTESIAN_POINT('Ctrl Pts',(36.0991010506208,4.77724914208039,-53.7997202332773));
#39956=CARTESIAN_POINT('Ctrl Pts',(36.1184352358726,4.78220830831117,-53.7665929856289));
#39957=CARTESIAN_POINT('Ctrl Pts',(36.1377220120453,4.78702974102347,-53.7335782690287));
#39958=CARTESIAN_POINT('Ctrl Pts',(36.1567145307872,4.79164136430998,-53.7010756726801));
#39959=CARTESIAN_POINT('Ctrl Pts',(36.165518137879,4.79377899123678,-53.6860097358443));
#39960=CARTESIAN_POINT('Ctrl Pts',(36.1742588505742,4.79587179689088,-53.6710532217596));
#39961=CARTESIAN_POINT('Ctrl Pts',(36.1829138277446,4.79791400485598,-53.6562428681622));
#39962=CARTESIAN_POINT('',(38.0216852001562,4.87035269640389,-47.6589608371561));
#39963=CARTESIAN_POINT('Ctrl Pts',(36.1830969697801,4.79736025611348,-53.6562730892812));
#39964=CARTESIAN_POINT('Ctrl Pts',(36.183936161047,4.79755340016328,-53.6547287540334));
#39965=CARTESIAN_POINT('Ctrl Pts',(36.1847749166295,4.79774608622482,-53.6531833391776));
#39966=CARTESIAN_POINT('Ctrl Pts',(36.1856132372291,4.79793831318313,-53.6516368116431));
#39967=CARTESIAN_POINT('Ctrl Pts',(36.2353363294914,4.80933982089724,-53.5599080251673));
#39968=CARTESIAN_POINT('Ctrl Pts',(36.2838250944541,4.81981537446271,-53.4691803615298));
#39969=CARTESIAN_POINT('Ctrl Pts',(36.3311210963185,4.82950527468665,-53.379305289989));
#39970=CARTESIAN_POINT('Ctrl Pts',(36.382327292743,4.8399962869211,-53.2819998014581));
#39971=CARTESIAN_POINT('Ctrl Pts',(36.4321352795488,4.84956616905091,-53.185693829071));
#39972=CARTESIAN_POINT('Ctrl Pts',(36.4806030253521,4.85834600565935,-53.0901555874634));
#39973=CARTESIAN_POINT('Ctrl Pts',(36.5307167410359,4.86742400646695,-52.9913728568557));
#39974=CARTESIAN_POINT('Ctrl Pts',(36.5793976635715,4.87565684395552,-52.8934106499926));
#39975=CARTESIAN_POINT('Ctrl Pts',(36.6267155733464,4.88314763835947,-52.7959696942444));
#39976=CARTESIAN_POINT('Ctrl Pts',(36.6772824731675,4.89115277324405,-52.6918381493133));
#39977=CARTESIAN_POINT('Ctrl Pts',(36.7262928124926,4.89831011493297,-52.5883018726186));
#39978=CARTESIAN_POINT('Ctrl Pts',(36.7738376014596,4.904705500865,-52.4849490338879));
#39979=CARTESIAN_POINT('Ctrl Pts',(36.81088898026,4.9096893880983,-52.4044067649851));
#39980=CARTESIAN_POINT('Ctrl Pts',(36.8470504776515,4.91420964272209,-52.3239748839792));
#39981=CARTESIAN_POINT('Ctrl Pts',(36.8823668850021,4.91829385211365,-52.2434412285763));
#39982=CARTESIAN_POINT('Ctrl Pts',(36.9169119340263,4.92228885682225,-52.1646665376408));
#39983=CARTESIAN_POINT('Ctrl Pts',(36.9506484477767,4.9258665600734,-52.0857943442769));
#39984=CARTESIAN_POINT('Ctrl Pts',(36.9836202495651,4.92905006187823,-52.0066157573371));
#39985=CARTESIAN_POINT('Ctrl Pts',(37.0244261353492,4.9329899621565,-51.9086243768252));
#39986=CARTESIAN_POINT('Ctrl Pts',(37.0640788100562,4.93634183787733,-51.8102526024379));
#39987=CARTESIAN_POINT('Ctrl Pts',(37.1025879776156,4.93913229986728,-51.7112748626131));
#39988=CARTESIAN_POINT('Ctrl Pts',(37.1555435239945,4.9429695793696,-51.5751664857263));
#39989=CARTESIAN_POINT('Ctrl Pts',(37.2063364481489,4.94574534134144,-51.4379137453509));
#39990=CARTESIAN_POINT('Ctrl Pts',(37.2550159356616,4.94752183743243,-51.2988780651826));
#39991=CARTESIAN_POINT('Ctrl Pts',(37.3058849186964,4.94937823638262,-51.153588868088));
#39992=CARTESIAN_POINT('Ctrl Pts',(37.3544465987836,4.95014231523103,-51.0063527325029));
#39993=CARTESIAN_POINT('Ctrl Pts',(37.4007617379197,4.9498744481247,-50.856386642756));
#39994=CARTESIAN_POINT('Ctrl Pts',(37.410231376825,4.94981967975265,-50.8257244285334));
#39995=CARTESIAN_POINT('Ctrl Pts',(37.4196070999113,4.94972177133796,-50.7949479162553));
#39996=CARTESIAN_POINT('Ctrl Pts',(37.4288894174247,4.94958125584787,-50.7640501489819));
#39997=CARTESIAN_POINT('Ctrl Pts',(37.4743950672278,4.94889239246057,-50.6125768800247));
#39998=CARTESIAN_POINT('Ctrl Pts',(37.517656483668,4.94717786909833,-50.4581937142545));
#39999=CARTESIAN_POINT('Ctrl Pts',(37.5587354913008,4.94452707813926,-50.3000098640844));
#40000=CARTESIAN_POINT('Ctrl Pts',(37.5893664918137,4.94255048756646,-50.1820583877729));
#40001=CARTESIAN_POINT('Ctrl Pts',(37.618784061382,4.94006319661273,-50.0620609190039));
#40002=CARTESIAN_POINT('Ctrl Pts',(37.6468085603049,4.93721482921126,-49.9412776473568));
#40003=CARTESIAN_POINT('Ctrl Pts',(37.6746737760593,4.93438265110852,-49.8211808729869));
#40004=CARTESIAN_POINT('Ctrl Pts',(37.7011616853365,4.931194526339,-49.7003073206902));
#40005=CARTESIAN_POINT('Ctrl Pts',(37.7261170122967,4.92779364152766,-49.579942038672));
#40006=CARTESIAN_POINT('Ctrl Pts',(37.7408671357427,4.92578351074985,-49.5087988005482));
#40007=CARTESIAN_POINT('Ctrl Pts',(37.7550822582431,4.923698898499,-49.4378340007195));
#40008=CARTESIAN_POINT('Ctrl Pts',(37.7687338082478,4.92156650463797,-49.3673203123641));
#40009=CARTESIAN_POINT('Ctrl Pts',(37.7773608907145,4.9202189406116,-49.3227592622079));
#40010=CARTESIAN_POINT('Ctrl Pts',(37.7857562022919,4.9188575258676,-49.2784542891617));
#40011=CARTESIAN_POINT('Ctrl Pts',(37.7939305095075,4.91748741564007,-49.2344038995284));
#40012=CARTESIAN_POINT('Ctrl Pts',(37.8199143669757,4.91313221489596,-49.0943799176225));
#40013=CARTESIAN_POINT('Ctrl Pts',(37.843666168356,4.90869138538402,-48.9569322895143));
#40014=CARTESIAN_POINT('Ctrl Pts',(37.865517087473,4.9043315399468,-48.8221395022688));
#40015=CARTESIAN_POINT('Ctrl Pts',(37.8859210597262,4.90026039928434,-48.69627256385));
#40016=CARTESIAN_POINT('Ctrl Pts',(37.9046673858781,4.89625931178411,-48.5727196058065));
#40017=CARTESIAN_POINT('Ctrl Pts',(37.9220149739313,4.89244366591783,-48.4515107005609));
#40018=CARTESIAN_POINT('Ctrl Pts',(37.9342485601373,4.88975285769171,-48.3660337116726));
#40019=CARTESIAN_POINT('Ctrl Pts',(37.9457864755788,4.88715352624105,-48.2817167006948));
#40020=CARTESIAN_POINT('Ctrl Pts',(37.9567236321371,4.88466346217324,-48.1982533436109));
#40021=CARTESIAN_POINT('Ctrl Pts',(37.962989829765,4.88323683602303,-48.1504348921342));
#40022=CARTESIAN_POINT('Ctrl Pts',(37.9690587532084,4.88184608572439,-48.1028976671077));
#40023=CARTESIAN_POINT('Ctrl Pts',(37.9749476898649,4.88049461981221,-48.055591658421));
#40024=CARTESIAN_POINT('Ctrl Pts',(37.9814496169309,4.87900247729043,-48.0033614789831));
#40025=CARTESIAN_POINT('Ctrl Pts',(37.9877319798698,4.87755856000559,-47.9514181081798));
#40026=CARTESIAN_POINT('Ctrl Pts',(37.9938059210639,4.8761962760931,-47.9001933518132));
#40027=CARTESIAN_POINT('Ctrl Pts',(38.0000321368439,4.8747998395255,-47.847684383381));
#40028=CARTESIAN_POINT('Ctrl Pts',(38.0060393577986,4.87348916692692,-47.7959304224487));
#40029=CARTESIAN_POINT('Ctrl Pts',(38.0118410068565,4.87229617339883,-47.7453415826759));
#40030=CARTESIAN_POINT('Ctrl Pts',(38.0151649334287,4.87161267413012,-47.7163578252825));
#40031=CARTESIAN_POINT('Ctrl Pts',(38.0184214069431,4.8709677295453,-47.687755518355));
#40032=CARTESIAN_POINT('Ctrl Pts',(38.0216131392841,4.87036678928707,-47.65960415993));
#40033=CARTESIAN_POINT('Ctrl Pts',(38.0216374408772,4.87036221377633,-47.6593898177534));
#40034=CARTESIAN_POINT('Ctrl Pts',(38.0216617394702,4.87035763848295,-47.6591754855729));
#40035=CARTESIAN_POINT('Ctrl Pts',(38.0216860350653,4.87035306340718,-47.6589611633871));
#40036=CARTESIAN_POINT('',(38.8604541099242,4.82976572790836,-41.6539325852788));
#40037=CARTESIAN_POINT('Ctrl Pts',(38.0216847782692,4.87035252387637,-47.6589606733005));
#40038=CARTESIAN_POINT('Ctrl Pts',(38.0531429489832,4.8650107124254,-47.3901353023222));
#40039=CARTESIAN_POINT('Ctrl Pts',(38.0789292235204,4.86042782994193,-47.1515865306677));
#40040=CARTESIAN_POINT('Ctrl Pts',(38.1330392026837,4.85049018544439,-46.6247656528001));
#40041=CARTESIAN_POINT('Ctrl Pts',(38.1596864519082,4.8456555010739,-46.3559543002791));
#40042=CARTESIAN_POINT('Ctrl Pts',(38.2427598130137,4.83283230623519,-45.5385385890846));
#40043=CARTESIAN_POINT('Ctrl Pts',(38.2941022354012,4.82771455234146,-45.0623082156166));
#40044=CARTESIAN_POINT('Ctrl Pts',(38.4970335348424,4.81981565007625,-43.495441392056));
#40045=CARTESIAN_POINT('Ctrl Pts',(38.6580818054566,4.82748306299288,-42.6038309561148));
#40046=CARTESIAN_POINT('Ctrl Pts',(38.8604349389735,4.8298193957887,-41.6539286669107));
#40047=CARTESIAN_POINT('',(40.1355627916624,4.76730435185959,-35.666088699485));
#40048=CARTESIAN_POINT('Ctrl Pts',(38.8604541099242,4.82976572790836,-41.6539325852788));
#40049=CARTESIAN_POINT('Ctrl Pts',(39.0048197292983,4.83127154325761,-40.9682358462176));
#40050=CARTESIAN_POINT('Ctrl Pts',(39.2693233059464,4.83474737532154,-39.8104175938772));
#40051=CARTESIAN_POINT('Ctrl Pts',(39.6452981730948,4.8199494242592,-38.1129891991618));
#40052=CARTESIAN_POINT('Ctrl Pts',(39.8853277117453,4.79858865457864,-36.9461294764195));
#40053=CARTESIAN_POINT('Ctrl Pts',(40.0280907705529,4.78204396051868,-36.2245904908727));
#40054=CARTESIAN_POINT('Ctrl Pts',(40.1031985714104,4.7719144148413,-35.8353019842399));
#40055=CARTESIAN_POINT('Ctrl Pts',(40.1355627919427,4.76730435097364,-35.6660886995628));
#40056=CARTESIAN_POINT('',(41.4215456143027,4.68791021227265,-29.7512571116574));
#40057=CARTESIAN_POINT('Ctrl Pts',(40.1355627919427,4.76730435097364,-35.6660886995628));
#40058=CARTESIAN_POINT('Ctrl Pts',(40.302285441518,4.74136007283982,-34.7693736439926));
#40059=CARTESIAN_POINT('Ctrl Pts',(40.511283714206,4.72982184735761,-33.6344138386462));
#40060=CARTESIAN_POINT('Ctrl Pts',(40.7814488661554,4.71765074492916,-32.2936083574543));
#40061=CARTESIAN_POINT('Ctrl Pts',(40.942076978619,4.71061953663584,-31.5521512150188));
#40062=CARTESIAN_POINT('Ctrl Pts',(41.140790301564,4.70106929600114,-30.7187864537994));
#40063=CARTESIAN_POINT('Ctrl Pts',(41.3201726461196,4.69236271641177,-30.0753227275525));
#40064=CARTESIAN_POINT('Ctrl Pts',(41.4215456143027,4.68791021227266,-29.7512571116574));
#40065=CARTESIAN_POINT('',(44.8643748761838,5.20597739866059,-23.980151972059));
#40066=CARTESIAN_POINT('Ctrl Pts',(41.4215456143027,4.68791021227266,-29.7512571116574));
#40067=CARTESIAN_POINT('Ctrl Pts',(41.4802706020203,4.68413040514277,-29.5553552623875));
#40068=CARTESIAN_POINT('Ctrl Pts',(41.6778820652349,4.68063495532933,-28.9529142456678));
#40069=CARTESIAN_POINT('Ctrl Pts',(42.0667678924717,4.70419304693246,-27.964824273678));
#40070=CARTESIAN_POINT('Ctrl Pts',(42.6729216974824,4.823611553925,-26.7992794766923));
#40071=CARTESIAN_POINT('Ctrl Pts',(43.1602150679141,4.93691815783542,-26.0485095188922));
#40072=CARTESIAN_POINT('Ctrl Pts',(43.3508405942975,4.97964296442833,-25.7696090237298));
#40073=CARTESIAN_POINT('Ctrl Pts',(43.6185109451061,5.03817773651984,-25.3933166689187));
#40074=CARTESIAN_POINT('Ctrl Pts',(44.1126562896923,5.13439651094732,-24.7624182520843));
#40075=CARTESIAN_POINT('Ctrl Pts',(44.5974177071842,5.19048925540186,-24.2398142598933));
#40076=CARTESIAN_POINT('Ctrl Pts',(44.864374876377,5.20597739807143,-23.9801519722225));
#40077=CARTESIAN_POINT('',(57.8135230789767,6.69056632316042,-18.0349157106052));
#40078=CARTESIAN_POINT('Ctrl Pts',(44.864374876377,5.20597739807143,-23.9801519722225));
#40079=CARTESIAN_POINT('Ctrl Pts',(45.1224142763232,5.22734724195968,-23.7522227177446));
#40080=CARTESIAN_POINT('Ctrl Pts',(45.9649684987856,5.22804284539893,-23.0069752550256));
#40081=CARTESIAN_POINT('Ctrl Pts',(47.4758616466553,5.06915938849053,-21.7520512140078));
#40082=CARTESIAN_POINT('Ctrl Pts',(49.1569256056527,5.20366478491719,-20.7106555371184));
#40083=CARTESIAN_POINT('Ctrl Pts',(50.0106311017377,5.31735504507218,-20.255161743136));
#40084=CARTESIAN_POINT('Ctrl Pts',(50.9536821648416,5.47540829520537,-19.8330327894735));
#40085=CARTESIAN_POINT('Ctrl Pts',(52.3106429243915,5.72884656211269,-19.3291250816917));
#40086=CARTESIAN_POINT('Ctrl Pts',(54.584459674483,6.15313027810468,-18.7389663173459));
#40087=CARTESIAN_POINT('Ctrl Pts',(56.7527899477957,6.52682846803759,-18.2841549642181));
#40088=CARTESIAN_POINT('Ctrl Pts',(57.8135230791049,6.69056632259679,-18.0349157107808));
#40089=CARTESIAN_POINT('',(70.7282577520135,8.51486332053725,-11.8925191843911));
#40090=CARTESIAN_POINT('Ctrl Pts',(57.8135230791049,6.6905663225968,-18.0349157107808));
#40091=CARTESIAN_POINT('Ctrl Pts',(58.3834371192583,6.78492400902022,-17.921496800064));
#40092=CARTESIAN_POINT('Ctrl Pts',(60.069006328368,7.0315326697423,-17.5237672087188));
#40093=CARTESIAN_POINT('Ctrl Pts',(62.2034160825709,7.1647901104433,-16.747451663188));
#40094=CARTESIAN_POINT('Ctrl Pts',(64.7264374328703,7.37946418630416,-15.4764719489058));
#40095=CARTESIAN_POINT('Ctrl Pts',(66.8940351574184,7.74903378142021,-14.2111203469359));
#40096=CARTESIAN_POINT('Ctrl Pts',(68.5152601688859,8.12096232366399,-13.2306538995856));
#40097=CARTESIAN_POINT('Ctrl Pts',(69.7958454230149,8.37193054851245,-12.4618050355517));
#40098=CARTESIAN_POINT('Ctrl Pts',(70.4319511017933,8.47390908124125,-12.0750795994181));
#40099=CARTESIAN_POINT('Ctrl Pts',(70.7282577522084,8.51486331986406,-11.8925191845565));
#40100=CARTESIAN_POINT('',(77.5413122691233,9.45942207531685,-5.67964638243729));
#40101=CARTESIAN_POINT('Ctrl Pts',(70.7282577522084,8.51486331986405,-11.8925191845565));
#40102=CARTESIAN_POINT('Ctrl Pts',(71.1586139886749,8.57802101438411,-11.6423301611079));
#40103=CARTESIAN_POINT('Ctrl Pts',(71.9827018728919,8.65468599963629,-11.0972577103214));
#40104=CARTESIAN_POINT('Ctrl Pts',(73.1303575054126,8.72650011278445,-10.21988802762));
#40105=CARTESIAN_POINT('Ctrl Pts',(74.1065736572356,8.81331425878696,-9.37805983947955));
#40106=CARTESIAN_POINT('Ctrl Pts',(75.1777989853639,8.95359154800345,-8.37681652932542));
#40107=CARTESIAN_POINT('Ctrl Pts',(76.3760621018627,9.18465108771821,-7.13733271471052));
#40108=CARTESIAN_POINT('Ctrl Pts',(77.1569389883271,9.37730603443782,-6.18970317121555));
#40109=CARTESIAN_POINT('Ctrl Pts',(77.5413122691233,9.45942207531684,-5.67964638243731));
#40110=CARTESIAN_POINT('',(79.5980561166602,9.79488102651321,-1.92025417898536));
#40111=CARTESIAN_POINT('Ctrl Pts',(77.5413122691233,9.45942207531684,-5.67964638243731));
#40112=CARTESIAN_POINT('Ctrl Pts',(78.375913647818,9.63522559747283,-4.55505891458532));
#40113=CARTESIAN_POINT('Ctrl Pts',(79.119383339007,9.77540103482857,-3.21481989604027));
#40114=CARTESIAN_POINT('Ctrl Pts',(79.5980561168973,9.79488102600527,-1.92025417906537));
#40115=CARTESIAN_POINT('',(73.6764401502847,5.16864402629879,0.190816765641456));
#40116=CARTESIAN_POINT('Ctrl Pts',(79.5980561168973,9.79488102600527,-1.92025417906537));
#40117=CARTESIAN_POINT('Ctrl Pts',(79.1741566879662,9.55093781207194,-1.62747314540123));
#40118=CARTESIAN_POINT('Ctrl Pts',(78.5111339416338,9.08098342033927,-1.27556034622203));
#40119=CARTESIAN_POINT('Ctrl Pts',(77.4831763160976,8.21812193305731,-0.881741433435836));
#40120=CARTESIAN_POINT('Ctrl Pts',(76.6699028312841,7.50475073429994,-0.627389809719394));
#40121=CARTESIAN_POINT('Ctrl Pts',(75.80573025497,6.75707546613834,-0.393749096424453));
#40122=CARTESIAN_POINT('Ctrl Pts',(75.0458066034774,6.13922536294966,-0.198996877529824));
#40123=CARTESIAN_POINT('Ctrl Pts',(74.3631359901759,5.6296023451996,-0.0144922142290973));
#40124=CARTESIAN_POINT('Ctrl Pts',(73.9161602099363,5.32222124600158,0.115689882622076));
#40125=CARTESIAN_POINT('Ctrl Pts',(73.6764877132773,5.1685596047474,0.19079632099573));
#40126=CARTESIAN_POINT('',(66.7632138022084,3.27206535817644,6.63309335729773));
#40127=CARTESIAN_POINT('Ctrl Pts',(73.6755257075894,5.17026710901218,0.191209832939039));
#40128=CARTESIAN_POINT('Ctrl Pts',(73.5820796918697,5.11091856903798,0.219589144636978));
#40129=CARTESIAN_POINT('Ctrl Pts',(73.4858752309367,5.0511962114572,0.249512021491082));
#40130=CARTESIAN_POINT('Ctrl Pts',(73.3869816798903,4.9913985445888,0.281309980862911));
#40131=CARTESIAN_POINT('Ctrl Pts',(73.2902869491031,4.93293043177097,0.312400937639211));
#40132=CARTESIAN_POINT('Ctrl Pts',(73.191021158279,4.87439026430786,0.345284932597864));
#40133=CARTESIAN_POINT('Ctrl Pts',(73.089263706746,4.81610240265113,0.380260242493337));
#40134=CARTESIAN_POINT('Ctrl Pts',(72.9903546154458,4.75944611514159,0.414256535320878));
#40135=CARTESIAN_POINT('Ctrl Pts',(72.8890911547841,4.70302833913953,0.450229099490815));
#40136=CARTESIAN_POINT('Ctrl Pts',(72.7855635481439,4.64718964924717,0.488434895496889));
#40137=CARTESIAN_POINT('Ctrl Pts',(72.7308024362584,4.61765367479579,0.508643919327953));
#40138=CARTESIAN_POINT('Ctrl Pts',(72.6754081532722,4.58828044060218,0.529477456516567));
#40139=CARTESIAN_POINT('Ctrl Pts',(72.6193965038322,4.55912510610204,0.550970931020803));
#40140=CARTESIAN_POINT('Ctrl Pts',(72.5261115336594,4.51056816238732,0.586767379582583));
#40141=CARTESIAN_POINT('Ctrl Pts',(72.4310749804319,4.46259978603407,0.624408249719697));
#40142=CARTESIAN_POINT('Ctrl Pts',(72.3347504347956,4.4156675454695,0.663888051858643));
#40143=CARTESIAN_POINT('Ctrl Pts',(72.2418625645885,4.37040975742295,0.701959290219107));
#40144=CARTESIAN_POINT('Ctrl Pts',(72.1477772313745,4.32611625075105,0.741740417083424));
#40145=CARTESIAN_POINT('Ctrl Pts',(72.0529368199214,4.28315485360461,0.783206316147256));
#40146=CARTESIAN_POINT('Ctrl Pts',(71.962539835658,4.242206267635,0.822729470546409));
#40147=CARTESIAN_POINT('Ctrl Pts',(71.8714571976677,4.20246836735063,0.863782979464733));
#40148=CARTESIAN_POINT('Ctrl Pts',(71.7800923301779,4.16422001174982,0.9063294470121));
#40149=CARTESIAN_POINT('Ctrl Pts',(71.7368716737269,4.14612641535269,0.926456289064087));
#40150=CARTESIAN_POINT('Ctrl Pts',(71.6935881326869,4.12836551900764,0.946917017120839));
#40151=CARTESIAN_POINT('Ctrl Pts',(71.6502857816389,4.11096308649717,0.967706624656799));
#40152=CARTESIAN_POINT('Ctrl Pts',(71.5726520176656,4.0797634794231,1.00497886150965));
#40153=CARTESIAN_POINT('Ctrl Pts',(71.4949576430323,4.04971750824251,1.04330805975467));
#40154=CARTESIAN_POINT('Ctrl Pts',(71.4174691269399,4.02087317004293,1.08266200151297));
#40155=CARTESIAN_POINT('Ctrl Pts',(71.3536327008094,3.9971106880957,1.11508248292992));
#40156=CARTESIAN_POINT('Ctrl Pts',(71.2899407935869,3.97416790693136,1.14820120033015));
#40157=CARTESIAN_POINT('Ctrl Pts',(71.2269259559942,3.95219042132279,1.18171128723549));
#40158=CARTESIAN_POINT('Ctrl Pts',(71.1894170622134,3.93910856306922,1.20165780044306));
#40159=CARTESIAN_POINT('Ctrl Pts',(71.1521481315531,3.92636766968791,1.22174306636928));
#40160=CARTESIAN_POINT('Ctrl Pts',(71.1152315400551,3.91398981467949,1.24190348951963));
#40161=CARTESIAN_POINT('Ctrl Pts',(71.0354159426054,3.88722824616644,1.28549137651809));
#40162=CARTESIAN_POINT('Ctrl Pts',(70.9572542145306,3.86215910818005,1.32942580059498));
#40163=CARTESIAN_POINT('Ctrl Pts',(70.8804278798133,3.83851758671466,1.37384802610265));
#40164=CARTESIAN_POINT('Ctrl Pts',(70.8620232274237,3.83285398209086,1.38448989287729));
#40165=CARTESIAN_POINT('Ctrl Pts',(70.8436951679833,3.82727254040222,1.39515976751782));
#40166=CARTESIAN_POINT('Ctrl Pts',(70.8254392477934,3.82177004629204,1.40585961048212));
#40167=CARTESIAN_POINT('Ctrl Pts',(70.714142899413,3.78822435289081,1.47109069375712));
#40168=CARTESIAN_POINT('Ctrl Pts',(70.6055211244504,3.75761012028982,1.53744133052309));
#40169=CARTESIAN_POINT('Ctrl Pts',(70.4997817703001,3.7295890075074,1.60467058390328));
#40170=CARTESIAN_POINT('Ctrl Pts',(70.4260311776581,3.71004497216883,1.6515613306788));
#40171=CARTESIAN_POINT('Ctrl Pts',(70.3536820295784,3.69176235831917,1.69888024428319));
#40172=CARTESIAN_POINT('Ctrl Pts',(70.2827935127124,3.67462778803868,1.74655537625686));
#40173=CARTESIAN_POINT('Ctrl Pts',(70.1816200961733,3.65017300900184,1.8145982159011));
#40174=CARTESIAN_POINT('Ctrl Pts',(70.0834250059408,3.62805484101416,1.88336363179219));
#40175=CARTESIAN_POINT('Ctrl Pts',(69.9881855044465,3.60792581144506,1.95274040185771));
#40176=CARTESIAN_POINT('Ctrl Pts',(69.9210193305481,3.59373012709947,2.00166728754712));
#40177=CARTESIAN_POINT('Ctrl Pts',(69.8553223782819,3.58052444170591,2.05089878906696));
#40178=CARTESIAN_POINT('Ctrl Pts',(69.791076817367,3.56819685019557,2.10040256093751));
#40179=CARTESIAN_POINT('Ctrl Pts',(69.7134049543905,3.55329298781217,2.16025183504746));
#40180=CARTESIAN_POINT('Ctrl Pts',(69.6378589189134,3.53967072030751,2.22049587198181));
#40181=CARTESIAN_POINT('Ctrl Pts',(69.5640380577044,3.52709664497903,2.28126322686332));
#40182=CARTESIAN_POINT('Ctrl Pts',(69.5271276270999,3.52080960731478,2.31164690430409));
#40183=CARTESIAN_POINT('Ctrl Pts',(69.4906482126204,3.51478661703879,2.34216143218193));
#40184=CARTESIAN_POINT('Ctrl Pts',(69.4550109833168,3.50906985735859,2.3725916283862));
#40185=CARTESIAN_POINT('Ctrl Pts',(69.4193737540132,3.5033530976784,2.40302182459044));
#40186=CARTESIAN_POINT('Ctrl Pts',(69.3845790920987,3.49793934079213,2.43336770489355));
#40187=CARTESIAN_POINT('Ctrl Pts',(69.3498330799623,3.4926920257565,2.46398464800622));
#40188=CARTESIAN_POINT('Ctrl Pts',(69.2896247814923,3.48359941655028,2.5170380471109));
#40189=CARTESIAN_POINT('Ctrl Pts',(69.2296102593908,3.47501734135315,2.57085342398526));
#40190=CARTESIAN_POINT('Ctrl Pts',(69.1694253615057,3.46685718341993,2.62639316269928));
#40191=CARTESIAN_POINT('Ctrl Pts',(69.1069888381267,3.45839173927236,2.68401074313119));
#40192=CARTESIAN_POINT('Ctrl Pts',(69.0443685754615,3.45038104759951,2.74348439598306));
#40193=CARTESIAN_POINT('Ctrl Pts',(68.9811856468568,3.44276220137922,2.80585531536981));
#40194=CARTESIAN_POINT('Ctrl Pts',(68.9168073375991,3.43499921145475,2.86940625271379));
#40195=CARTESIAN_POINT('Ctrl Pts',(68.8518446835568,3.4276440543443,2.93596529709815));
#40196=CARTESIAN_POINT('Ctrl Pts',(68.7859294095244,3.42065385850673,3.00659652686413));
#40197=CARTESIAN_POINT('Ctrl Pts',(68.718344605385,3.41348661201471,3.07901673447066));
#40198=CARTESIAN_POINT('Ctrl Pts',(68.6497584139789,3.40670451572753,3.15571813494658));
#40199=CARTESIAN_POINT('Ctrl Pts',(68.5798088336028,3.40026713156069,3.23780643100444));
#40200=CARTESIAN_POINT('Ctrl Pts',(68.5515071958064,3.39766256246869,3.27101939968653));
#40201=CARTESIAN_POINT('Ctrl Pts',(68.5229827499876,3.39511436007263,3.30511374067851));
#40202=CARTESIAN_POINT('Ctrl Pts',(68.4942129036598,3.39261916495141,3.34016082576519));
#40203=CARTESIAN_POINT('Ctrl Pts',(68.4619893586378,3.38982443218114,3.37941516558042));
#40204=CARTESIAN_POINT('Ctrl Pts',(68.4294149535231,3.38709221292072,3.41988751388573));
#40205=CARTESIAN_POINT('Ctrl Pts',(68.3965806450077,3.38442708502318,3.46156378462874));
#40206=CARTESIAN_POINT('Ctrl Pts',(68.347076532678,3.38040888586572,3.52439887638567));
#40207=CARTESIAN_POINT('Ctrl Pts',(68.2969825696369,3.37654398048543,3.58997028569425));
#40208=CARTESIAN_POINT('Ctrl Pts',(68.2465830018763,3.37283705789084,3.65823607603959));
#40209=CARTESIAN_POINT('Ctrl Pts',(68.1859376180816,3.3683765485366,3.74037973796942));
#40210=CARTESIAN_POINT('Ctrl Pts',(68.1248508938036,3.36414515624265,3.82642422986708));
#40211=CARTESIAN_POINT('Ctrl Pts',(68.0637806680368,3.36012805833028,3.91630856639725));
#40212=CARTESIAN_POINT('Ctrl Pts',(68.0020010445552,3.35606429741571,4.00723700817083));
#40213=CARTESIAN_POINT('Ctrl Pts',(67.9402384693474,3.35221938996863,4.10209499325176));
#40214=CARTESIAN_POINT('Ctrl Pts',(67.8789232542081,3.34855084749676,4.2008365426439));
#40215=CARTESIAN_POINT('Ctrl Pts',(67.8157330182447,3.34477012090365,4.30259761110501));
#40216=CARTESIAN_POINT('Ctrl Pts',(67.7530181004581,3.34117618230318,4.40848346717966));
#40217=CARTESIAN_POINT('Ctrl Pts',(67.6912005113719,3.33770132789118,4.51846170635032));
#40218=CARTESIAN_POINT('Ctrl Pts',(67.647034253233,3.33521867984191,4.5970368719735));
#40219=CARTESIAN_POINT('Ctrl Pts',(67.6033249805881,3.33279635196203,4.67770142782428));
#40220=CARTESIAN_POINT('Ctrl Pts',(67.560211592247,3.33040570470243,4.7604482025443));
#40221=CARTESIAN_POINT('Ctrl Pts',(67.5030340789018,3.32723519848964,4.87018800722854));
#40222=CARTESIAN_POINT('Ctrl Pts',(67.4469958924026,3.32412842972577,4.9836052813711));
#40223=CARTESIAN_POINT('Ctrl Pts',(67.3922782031099,3.32097851832306,5.09928652163564));
#40224=CARTESIAN_POINT('Ctrl Pts',(67.3817314770598,3.32037137914968,5.12158385118265));
#40225=CARTESIAN_POINT('Ctrl Pts',(67.3712337501578,3.31976269008265,5.14396542535823));
#40226=CARTESIAN_POINT('Ctrl Pts',(67.3607862519462,3.31915177658107,5.16642130746712));
#40227=CARTESIAN_POINT('Ctrl Pts',(67.3039017197311,3.3158254751013,5.28868908137495));
#40228=CARTESIAN_POINT('Ctrl Pts',(67.2485058467987,3.31242967257486,5.41315817519173));
#40229=CARTESIAN_POINT('Ctrl Pts',(67.1947972253839,3.30887182807225,5.5383406212005));
#40230=CARTESIAN_POINT('Ctrl Pts',(67.1753348086868,3.30758257039947,5.58370303906188));
#40231=CARTESIAN_POINT('Ctrl Pts',(67.1560940283144,3.30627247758143,5.629159280694));
#40232=CARTESIAN_POINT('Ctrl Pts',(67.137084892584,3.30493882395428,5.67463873313827));
#40233=CARTESIAN_POINT('Ctrl Pts',(67.1054532744659,3.30271959511434,5.7503175379157));
#40234=CARTESIAN_POINT('Ctrl Pts',(67.0744664739271,3.30044219646204,5.8265021274338));
#40235=CARTESIAN_POINT('Ctrl Pts',(67.0439283533832,3.2980713592277,5.90308348319905));
#40236=CARTESIAN_POINT('Ctrl Pts',(67.0104544275529,3.29547259976495,5.98702704544908));
#40237=CARTESIAN_POINT('Ctrl Pts',(66.977519486075,3.29276151625854,6.07144315063479));
#40238=CARTESIAN_POINT('Ctrl Pts',(66.9448701424927,3.28989842821305,6.15588714158495));
#40239=CARTESIAN_POINT('Ctrl Pts',(66.9303273345756,3.28862313949581,6.19350053914223));
#40240=CARTESIAN_POINT('Ctrl Pts',(66.9158412634233,3.28731774542639,6.23112011639764));
#40241=CARTESIAN_POINT('Ctrl Pts',(66.901389897882,3.28597900649281,6.26870995157757));
#40242=CARTESIAN_POINT('Ctrl Pts',(66.8814989574804,3.284136358733,6.32044881107371));
#40243=CARTESIAN_POINT('Ctrl Pts',(66.8616737379568,3.28223055848634,6.37213594417084));
#40244=CARTESIAN_POINT('Ctrl Pts',(66.8418573733355,3.28025518624225,6.42417246121676));
#40245=CARTESIAN_POINT('Ctrl Pts',(66.822565995373,3.27833214670874,6.47483039658318));
#40246=CARTESIAN_POINT('Ctrl Pts',(66.8032830102522,3.27634316919812,6.52581955560616));
#40247=CARTESIAN_POINT('Ctrl Pts',(66.7839566804709,3.27428245778291,6.57746051724003));
#40248=CARTESIAN_POINT('Ctrl Pts',(66.7770581476665,3.27354688690841,6.5958937568626));
#40249=CARTESIAN_POINT('Ctrl Pts',(66.770154099003,3.27280217762856,6.61440956897775));
#40250=CARTESIAN_POINT('Ctrl Pts',(66.7632422045598,3.27204807172044,6.63302090600835));
#40251=CARTESIAN_POINT('',(64.4551540394283,2.94901890714283,12.6430799879059));
#40252=CARTESIAN_POINT('Ctrl Pts',(66.7626079618727,3.27243408934811,6.63463878967692));
#40253=CARTESIAN_POINT('Ctrl Pts',(66.7582438740882,3.27195413689024,6.64675428470166));
#40254=CARTESIAN_POINT('Ctrl Pts',(66.7538841597794,3.27147418576871,6.65888415304361));
#40255=CARTESIAN_POINT('Ctrl Pts',(66.7495284430053,3.27099416305559,6.67102845311044));
#40256=CARTESIAN_POINT('Ctrl Pts',(66.744846305267,3.27047816704921,6.68408285691971));
#40257=CARTESIAN_POINT('Ctrl Pts',(66.7401657718722,3.26996175625489,6.69716233557186));
#40258=CARTESIAN_POINT('Ctrl Pts',(66.7354845820625,3.26944463942253,6.71027211865419));
#40259=CARTESIAN_POINT('Ctrl Pts',(66.6809666044278,3.26342220387788,6.8629510079821));
#40260=CARTESIAN_POINT('Ctrl Pts',(66.6264369335311,3.25731251986083,7.01953283719209));
#40261=CARTESIAN_POINT('Ctrl Pts',(66.571060967788,3.25095694222195,7.18059086773355));
#40262=CARTESIAN_POINT('Ctrl Pts',(66.5446749256618,3.24792857897688,7.2573332580759));
#40263=CARTESIAN_POINT('Ctrl Pts',(66.5180964371422,3.24484435668027,7.3350913428522));
#40264=CARTESIAN_POINT('Ctrl Pts',(66.4912348586684,3.2416871768498,7.41392273497785));
#40265=CARTESIAN_POINT('Ctrl Pts',(66.4405666300019,3.23573187866256,7.56262013957055));
#40266=CARTESIAN_POINT('Ctrl Pts',(66.3888905563711,3.22951681633887,7.71513726506168));
#40267=CARTESIAN_POINT('Ctrl Pts',(66.3355831927921,3.22293399710941,7.87189817464005));
#40268=CARTESIAN_POINT('Ctrl Pts',(66.308765753888,3.2196223654576,7.95076018980873));
#40269=CARTESIAN_POINT('Ctrl Pts',(66.2815357166608,3.21621771829495,8.03069556540575));
#40270=CARTESIAN_POINT('Ctrl Pts',(66.2538159346678,3.21270677850378,8.11175363983937));
#40271=CARTESIAN_POINT('Ctrl Pts',(66.1991717354852,3.20578563845603,8.2715439861641));
#40272=CARTESIAN_POINT('Ctrl Pts',(66.1426207789929,3.19846053540797,8.4357013913799));
#40273=CARTESIAN_POINT('Ctrl Pts',(66.0835682271523,3.19060269005156,8.60465395408236));
#40274=CARTESIAN_POINT('Ctrl Pts',(66.0617317921506,3.18769701834,8.66712918231278));
#40275=CARTESIAN_POINT('Ctrl Pts',(66.0395535824283,3.18471855611422,8.73025968650451));
#40276=CARTESIAN_POINT('Ctrl Pts',(66.0170046138161,3.18166100123051,8.79406563030403));
#40277=CARTESIAN_POINT('Ctrl Pts',(65.9943401000079,3.17858777885512,8.85819852787281));
#40278=CARTESIAN_POINT('Ctrl Pts',(65.9713403757572,3.17544058934947,8.92290296450967));
#40279=CARTESIAN_POINT('Ctrl Pts',(65.9479113350192,3.17220436938723,8.98838307743012));
#40280=CARTESIAN_POINT('Ctrl Pts',(65.9119955708399,3.1672433761355,9.08876142071671));
#40281=CARTESIAN_POINT('Ctrl Pts',(65.8750725641278,3.16207354628284,9.19096145543401));
#40282=CARTESIAN_POINT('Ctrl Pts',(65.8371161191711,3.15668978690338,9.29487750489127));
#40283=CARTESIAN_POINT('Ctrl Pts',(65.8192619842666,3.1541573483053,9.34375803540111));
#40284=CARTESIAN_POINT('Ctrl Pts',(65.8011786230049,3.15157745031492,9.39301896048947));
#40285=CARTESIAN_POINT('Ctrl Pts',(65.7828612214198,3.14894903800416,9.44264976966276));
#40286=CARTESIAN_POINT('Ctrl Pts',(65.7719027971886,3.14737658478136,9.47234150619706));
#40287=CARTESIAN_POINT('Ctrl Pts',(65.7608572760255,3.14578636360764,9.50217457066608));
#40288=CARTESIAN_POINT('Ctrl Pts',(65.7497218072676,3.14417797450116,9.53215067526452));
#40289=CARTESIAN_POINT('Ctrl Pts',(65.7369478785919,3.14233292889279,9.56653742901881));
#40290=CARTESIAN_POINT('Ctrl Pts',(65.7241525267092,3.14047797905138,9.60085143804542));
#40291=CARTESIAN_POINT('Ctrl Pts',(65.7113335685273,3.13861315887182,9.63509460891077));
#40292=CARTESIAN_POINT('Ctrl Pts',(65.675285029997,3.13336904767802,9.73139075457402));
#40293=CARTESIAN_POINT('Ctrl Pts',(65.6389780277389,3.12803839930249,9.82731896967742));
#40294=CARTESIAN_POINT('Ctrl Pts',(65.6024906864775,3.1226370759973,9.92255311418928));
#40295=CARTESIAN_POINT('Ctrl Pts',(65.556412456212,3.11581598653473,10.0428200530305));
#40296=CARTESIAN_POINT('Ctrl Pts',(65.5100459047643,3.1088821443127,10.1619850432727));
#40297=CARTESIAN_POINT('Ctrl Pts',(65.463212531056,3.10183216685072,10.2806741465391));
#40298=CARTESIAN_POINT('Ctrl Pts',(65.3879225999276,3.0904985328299,10.4714802683934));
#40299=CARTESIAN_POINT('Ctrl Pts',(65.3116519243754,3.07889057491832,10.6604749294055));
#40300=CARTESIAN_POINT('Ctrl Pts',(65.234506165267,3.06710243124938,10.8480506983372));
#40301=CARTESIAN_POINT('Ctrl Pts',(65.2117989721025,3.063632692168,10.9032620186656));
#40302=CARTESIAN_POINT('Ctrl Pts',(65.1890159374527,3.06014733840129,10.9583503403728));
#40303=CARTESIAN_POINT('Ctrl Pts',(65.1661480826901,3.05664663471501,11.0133411959318));
#40304=CARTESIAN_POINT('Ctrl Pts',(65.1491066523579,3.05403786364302,11.054321114846));
#40305=CARTESIAN_POINT('Ctrl Pts',(65.1320205196827,3.05142106746363,11.0952410669356));
#40306=CARTESIAN_POINT('Ctrl Pts',(65.1148886686486,3.04879690068722,11.1361052727008));
#40307=CARTESIAN_POINT('Ctrl Pts',(65.0917641754397,3.04525481252177,11.1912635884499));
#40308=CARTESIAN_POINT('Ctrl Pts',(65.0685599925776,3.04170057085351,11.2463115263669));
#40309=CARTESIAN_POINT('Ctrl Pts',(65.0452684027928,3.03813443698347,11.3012725404979));
#40310=CARTESIAN_POINT('Ctrl Pts',(64.9618817011173,3.02536724745703,11.4980396024053));
#40311=CARTESIAN_POINT('Ctrl Pts',(64.8773749226518,3.01244768631303,11.6936927880249));
#40312=CARTESIAN_POINT('Ctrl Pts',(64.7918465919002,2.99946266463069,11.8887146066709));
#40313=CARTESIAN_POINT('Ctrl Pts',(64.6957882909471,2.98487896926703,12.1077468780047));
#40314=CARTESIAN_POINT('Ctrl Pts',(64.5984198280383,2.9702283213973,12.3260248599227));
#40315=CARTESIAN_POINT('Ctrl Pts',(64.4999193330072,2.95563529360733,12.5441356757672));
#40316=CARTESIAN_POINT('Ctrl Pts',(64.4850232036326,2.95342840490227,12.5771203519336));
#40317=CARTESIAN_POINT('Ctrl Pts',(64.4701012223787,2.95122280440128,12.6101011343138));
#40318=CARTESIAN_POINT('Ctrl Pts',(64.4551540394283,2.94901890714283,12.6430799879059));
#40319=CARTESIAN_POINT('',(61.5166583930919,2.54671945820444,18.6669577091217));
#40320=CARTESIAN_POINT('Ctrl Pts',(64.455131965346,2.94901573117602,12.6431286671725));
#40321=CARTESIAN_POINT('Ctrl Pts',(64.3756406866424,2.93729544625666,12.8183754180639));
#40322=CARTESIAN_POINT('Ctrl Pts',(64.2949735702456,2.92553927651984,12.9941893144439));
#40323=CARTESIAN_POINT('Ctrl Pts',(64.1453393500078,2.90398855251153,13.3183226136813));
#40324=CARTESIAN_POINT('Ctrl Pts',(64.0517379200529,2.89064511331178,13.520320295579));
#40325=CARTESIAN_POINT('Ctrl Pts',(63.8113439371817,2.85680317093103,14.0344315980323));
#40326=CARTESIAN_POINT('Ctrl Pts',(63.6411847868847,2.8333580159102,14.392662513831));
#40327=CARTESIAN_POINT('Ctrl Pts',(63.367659946999,2.7962459604253,14.9686646720361));
#40328=CARTESIAN_POINT('Ctrl Pts',(63.2444061328582,2.77968504765282,15.2284282557368));
#40329=CARTESIAN_POINT('Ctrl Pts',(62.886939604599,2.73188620171305,15.9801214605262));
#40330=CARTESIAN_POINT('Ctrl Pts',(62.6232915029037,2.69700497899866,16.53067421596));
#40331=CARTESIAN_POINT('Ctrl Pts',(62.1036482761331,2.6273101994606,17.5771759416381));
#40332=CARTESIAN_POINT('Ctrl Pts',(61.8045070651265,2.58662238128951,18.1611507203481));
#40333=CARTESIAN_POINT('Ctrl Pts',(61.5166583935928,2.54671945895772,18.6669577094661));
#40334=CARTESIAN_POINT('',(49.3675957670801,0.956505486201908,24.6840252059531));
#40335=CARTESIAN_POINT('Ctrl Pts',(61.5166583915077,2.5467194586667,18.6669577089628));
#40336=CARTESIAN_POINT('Ctrl Pts',(61.5166207736063,2.54671424394586,18.6670239120275));
#40337=CARTESIAN_POINT('Ctrl Pts',(61.5165831563685,2.54670902930684,18.6670901132125));
#40338=CARTESIAN_POINT('Ctrl Pts',(61.5165455397943,2.54670381474961,18.6671563125178));
#40339=CARTESIAN_POINT('Ctrl Pts',(61.440598562313,2.53617574652035,18.8008111509416));
#40340=CARTESIAN_POINT('Ctrl Pts',(61.3673089566769,2.52599500692197,18.926675616836));
#40341=CARTESIAN_POINT('Ctrl Pts',(61.2953855126163,2.51598545816718,19.0465923056338));
#40342=CARTESIAN_POINT('Ctrl Pts',(61.2181583162547,2.50523778892978,19.1753518470292));
#40343=CARTESIAN_POINT('Ctrl Pts',(61.1425070165007,2.49468764125461,19.2972541878678));
#40344=CARTESIAN_POINT('Ctrl Pts',(61.0668941562081,2.48412302983043,19.4145920223673));
#40345=CARTESIAN_POINT('Ctrl Pts',(60.9832401113652,2.47243490595301,19.5444083582525));
#40346=CARTESIAN_POINT('Ctrl Pts',(60.899633716831,2.46072921556197,19.6686377804292));
#40347=CARTESIAN_POINT('Ctrl Pts',(60.8140534103825,2.44872366676954,19.7903973547229));
#40348=CARTESIAN_POINT('Ctrl Pts',(60.8085305719405,2.44794890083169,19.7982549855902));
#40349=CARTESIAN_POINT('Ctrl Pts',(60.8029995299401,2.44717288716868,19.8061023341489));
#40350=CARTESIAN_POINT('Ctrl Pts',(60.7974597477827,2.44639555031116,19.8139402396247));
#40351=CARTESIAN_POINT('Ctrl Pts',(60.6275577239221,2.42255506316564,20.0543244217698));
#40352=CARTESIAN_POINT('Ctrl Pts',(60.4492882397345,2.39744916755369,20.285799444722));
#40353=CARTESIAN_POINT('Ctrl Pts',(60.2598484860335,2.37067877124953,20.5074382120966));
#40354=CARTESIAN_POINT('Ctrl Pts',(60.0546114750151,2.34167600908422,20.747559291506));
#40355=CARTESIAN_POINT('Ctrl Pts',(59.8362641090708,2.31071933158198,20.9761348857896));
#40356=CARTESIAN_POINT('Ctrl Pts',(59.6012986958576,2.27731469479028,21.1920080513495));
#40357=CARTESIAN_POINT('Ctrl Pts',(59.5483682209496,2.2697896583803,21.2406376305575));
#40358=CARTESIAN_POINT('Ctrl Pts',(59.4945946258952,2.26214045636031,21.2886227035624));
#40359=CARTESIAN_POINT('Ctrl Pts',(59.4399380897665,2.25436154671837,21.3359502099995));
#40360=CARTESIAN_POINT('Ctrl Pts',(59.3251199132003,2.23802022170907,21.4353721341723));
#40361=CARTESIAN_POINT('Ctrl Pts',(59.2064051575535,2.22110625075009,21.5318921728796));
#40362=CARTESIAN_POINT('Ctrl Pts',(59.0834292363997,2.20357785323861,21.6253876201116));
#40363=CARTESIAN_POINT('Ctrl Pts',(59.0632484738035,2.20070138420669,21.6407305377064));
#40364=CARTESIAN_POINT('Ctrl Pts',(59.0429527992837,2.19780835258924,21.6559919699139));
#40365=CARTESIAN_POINT('Ctrl Pts',(59.0225450240649,2.19489921098158,21.6711714773165));
#40366=CARTESIAN_POINT('Ctrl Pts',(58.8001707963232,2.16319962043547,21.8365756529287));
#40367=CARTESIAN_POINT('Ctrl Pts',(58.5644828709371,2.12958414079278,21.9922525289487));
#40368=CARTESIAN_POINT('Ctrl Pts',(58.3191411311679,2.09465967824874,22.1376328116747));
#40369=CARTESIAN_POINT('Ctrl Pts',(58.2069674438234,2.07869172373037,22.2041027176757));
#40370=CARTESIAN_POINT('Ctrl Pts',(58.0927762566005,2.06245063882631,22.2684201738044));
#40371=CARTESIAN_POINT('Ctrl Pts',(57.9769203136681,2.04599642011994,22.3305308335531));
#40372=CARTESIAN_POINT('Ctrl Pts',(57.7755910457054,2.01740301590426,22.438463955872));
#40373=CARTESIAN_POINT('Ctrl Pts',(57.5692249334683,1.98816219670544,22.5397333935213));
#40374=CARTESIAN_POINT('Ctrl Pts',(57.3531349720908,1.95767600444684,22.6371193347432));
#40375=CARTESIAN_POINT('Ctrl Pts',(57.1479418687527,1.92872715204006,22.7295943547462));
#40376=CARTESIAN_POINT('Ctrl Pts',(56.9339817287562,1.89865408522091,22.8185679023946));
#40377=CARTESIAN_POINT('Ctrl Pts',(56.7072181447654,1.86698155708814,22.9064219236721));
#40378=CARTESIAN_POINT('Ctrl Pts',(56.6795557795455,1.86311789862399,22.9171390325652));
#40379=CARTESIAN_POINT('Ctrl Pts',(56.6517031245348,1.85923055057753,22.9278394762033));
#40380=CARTESIAN_POINT('Ctrl Pts',(56.6238148783573,1.85534126944944,22.9384756468297));
#40381=CARTESIAN_POINT('Ctrl Pts',(56.5343603223993,1.8428659809679,22.9725923106896));
#40382=CARTESIAN_POINT('Ctrl Pts',(56.4445386642837,1.83037181694639,23.0060476860461));
#40383=CARTESIAN_POINT('Ctrl Pts',(56.3594657709293,1.81856838050457,23.037270574256));
#40384=CARTESIAN_POINT('Ctrl Pts',(56.2881077385875,1.80866781210787,23.0634599252799));
#40385=CARTESIAN_POINT('Ctrl Pts',(56.2200877909376,1.79924885481185,23.0880785380807));
#40386=CARTESIAN_POINT('Ctrl Pts',(56.1411095920773,1.78834134685333,23.1157628475816));
#40387=CARTESIAN_POINT('Ctrl Pts',(56.0965756774391,1.78219086437399,23.1313733666099));
#40388=CARTESIAN_POINT('Ctrl Pts',(56.0485570767083,1.77556757273511,23.1479586453918));
#40389=CARTESIAN_POINT('Ctrl Pts',(55.9944861447575,1.76812431597734,23.1663498795247));
#40390=CARTESIAN_POINT('Ctrl Pts',(55.9834762727519,1.76660872707862,23.1700946852183));
#40391=CARTESIAN_POINT('Ctrl Pts',(55.9722155459999,1.76505917553994,23.173914352136));
#40392=CARTESIAN_POINT('Ctrl Pts',(55.9607053836033,1.7634759418204,23.1778074609361));
#40393=CARTESIAN_POINT('Ctrl Pts',(55.8442429111033,1.74745641862258,23.2171988318781));
#40394=CARTESIAN_POINT('Ctrl Pts',(55.7022443876334,1.7279845356483,23.264109262772));
#40395=CARTESIAN_POINT('Ctrl Pts',(55.5361736098594,1.70537682788494,23.3170673603437));
#40396=CARTESIAN_POINT('Ctrl Pts',(55.378986512611,1.68397848191223,23.3671925524134));
#40397=CARTESIAN_POINT('Ctrl Pts',(55.2002330785305,1.65977062163439,23.4227357204199));
#40398=CARTESIAN_POINT('Ctrl Pts',(55.0011514813534,1.63306739719635,23.4824469066612));
#40399=CARTESIAN_POINT('Ctrl Pts',(54.8650711105551,1.61481465694027,23.5232619316547));
#40400=CARTESIAN_POINT('Ctrl Pts',(54.7194928057945,1.59539694607339,23.566024319518));
#40401=CARTESIAN_POINT('Ctrl Pts',(54.5648131060747,1.57492870704247,23.6103341755122));
#40402=CARTESIAN_POINT('Ctrl Pts',(54.3281046519902,1.54360588169681,23.6781421524613));
#40403=CARTESIAN_POINT('Ctrl Pts',(54.0700905768493,1.50982335770047,23.7495805755989));
#40404=CARTESIAN_POINT('Ctrl Pts',(53.7943690560697,1.47432005250733,23.8225022067969));
#40405=CARTESIAN_POINT('Ctrl Pts',(53.4973758221844,1.43607769335773,23.9010496883589));
#40406=CARTESIAN_POINT('Ctrl Pts',(53.1798365176838,1.39584378645511,23.9813174692087));
#40407=CARTESIAN_POINT('Ctrl Pts',(52.8462862359951,1.35449227659147,24.0606355793502));
#40408=CARTESIAN_POINT('Ctrl Pts',(52.647437516317,1.32984023687047,24.1079217173474));
#40409=CARTESIAN_POINT('Ctrl Pts',(52.4428992466314,1.30479073854547,24.1548704602671));
#40410=CARTESIAN_POINT('Ctrl Pts',(52.2336396985611,1.27952382229616,24.2009170329423));
#40411=CARTESIAN_POINT('Ctrl Pts',(51.8629974700757,1.23477085292413,24.2824751002697));
#40412=CARTESIAN_POINT('Ctrl Pts',(51.4775197598703,1.18933379101783,24.3611984471246));
#40413=CARTESIAN_POINT('Ctrl Pts',(51.0806283298492,1.1439453075006,24.4331895149969));
#40414=CARTESIAN_POINT('Ctrl Pts',(51.0384353196498,1.13912011702501,24.4408427915135));
#40415=CARTESIAN_POINT('Ctrl Pts',(50.9961133574418,1.13429544845148,24.4484199862611));
#40416=CARTESIAN_POINT('Ctrl Pts',(50.953666582741,1.12947216046453,24.4559164186186));
#40417=CARTESIAN_POINT('Ctrl Pts',(50.6003160043242,1.08932042662669,24.5183208940646));
#40418=CARTESIAN_POINT('Ctrl Pts',(50.2383145786455,1.04926822505876,24.5751286405623));
#40419=CARTESIAN_POINT('Ctrl Pts',(49.8700363839702,1.00972402104231,24.6236399656901));
#40420=CARTESIAN_POINT('Ctrl Pts',(49.7037634610372,0.991870315658882,24.6455422122553));
#40421=CARTESIAN_POINT('Ctrl Pts',(49.5362113339751,0.974119523575312,24.6657533142736));
#40422=CARTESIAN_POINT('Ctrl Pts',(49.3675995744407,0.956505883929035,24.6840247933719));
#40423=CARTESIAN_POINT('Ctrl Pts',(49.3675983053205,0.956505751353318,24.684024930899));
#40424=CARTESIAN_POINT('Ctrl Pts',(49.3675970362003,0.956505618777609,24.6840250684261));
#40425=CARTESIAN_POINT('Ctrl Pts',(49.3675957670801,0.956505486201908,24.6840252059531));
#40426=CARTESIAN_POINT('',(44.3052665433902,0.501764637226403,24.6839663391593));
#40427=CARTESIAN_POINT('Ctrl Pts',(49.367596314931,0.956500241803234,24.6840252060176));
#40428=CARTESIAN_POINT('Ctrl Pts',(48.9249563174813,0.91026051062961,24.7319912218939));
#40429=CARTESIAN_POINT('Ctrl Pts',(48.2454451876077,0.842024097628023,24.7841312821754));
#40430=CARTESIAN_POINT('Ctrl Pts',(46.6888479202391,0.694486082024801,24.8361224907741));
#40431=CARTESIAN_POINT('Ctrl Pts',(45.4053646426555,0.584777912483909,24.7905806974873));
#40432=CARTESIAN_POINT('Ctrl Pts',(44.3052665433902,0.501764637226404,24.6839663391593));
#40433=CARTESIAN_POINT('',(30.3222847657761,-0.00413284663037694,18.6660068644684));
#40434=CARTESIAN_POINT('Ctrl Pts',(44.3052665433902,0.501764637226404,24.6839663391593));
#40435=CARTESIAN_POINT('Ctrl Pts',(43.5184633083404,0.442392556145283,24.6077156960038));
#40436=CARTESIAN_POINT('Ctrl Pts',(42.2816666702738,0.357564010552012,24.4340698272278));
#40437=CARTESIAN_POINT('Ctrl Pts',(39.7590447329804,0.209255798855571,23.9283169242352));
#40438=CARTESIAN_POINT('Ctrl Pts',(36.2988021098604,0.0624334299665293,
22.7904348263529));
#40439=CARTESIAN_POINT('Ctrl Pts',(33.2830669754168,0.0134785075079505,
20.9642163836828));
#40440=CARTESIAN_POINT('Ctrl Pts',(31.3601866444384,-0.00140202227099839,
19.5546871871865));
#40441=CARTESIAN_POINT('Ctrl Pts',(30.6635153578141,-0.00339250812609648,
18.9682311100362));
#40442=CARTESIAN_POINT('Ctrl Pts',(30.3222847657761,-0.00413284663037694,
18.6660068644684));
#40443=CARTESIAN_POINT('',(25.4512489032773,0.000555756585220059,12.648002570409));
#40444=CARTESIAN_POINT('Ctrl Pts',(30.3222847579815,-0.00412925426626926,
18.6660068644463));
#40445=CARTESIAN_POINT('Ctrl Pts',(29.3243355961853,-0.00630000276266593,
17.7821469838973));
#40446=CARTESIAN_POINT('Ctrl Pts',(28.4882783945593,-0.00480235629088497,
16.8802696648002));
#40447=CARTESIAN_POINT('Ctrl Pts',(27.2613257884266,-0.00266691039312472,
15.2953825351106));
#40448=CARTESIAN_POINT('Ctrl Pts',(26.8875894678604,-0.00191427135626064,
14.7718457182022));
#40449=CARTESIAN_POINT('Ctrl Pts',(26.340767674565,-0.000872705426741305,
13.9769047302795));
#40450=CARTESIAN_POINT('Ctrl Pts',(26.1604061374871,-0.000538421769267547,
13.7098371610195));
#40451=CARTESIAN_POINT('Ctrl Pts',(25.8945556885661,-8.20109892347277E-5,
13.3131630236195));
#40452=CARTESIAN_POINT('Ctrl Pts',(25.8053019634277,6.50220491256103E-5,
13.1794702756233));
#40453=CARTESIAN_POINT('Ctrl Pts',(25.6290023245359,0.000339467860826898,
12.9149907782377));
#40454=CARTESIAN_POINT('Ctrl Pts',(25.5412899884507,0.000468171758386591,
12.783207411861));
#40455=CARTESIAN_POINT('Ctrl Pts',(25.4512489498233,0.000589988472317472,
12.6480025702534));
#40456=CARTESIAN_POINT('',(21.143061504949,0.000717013383189543,6.63001173766479));
#40457=CARTESIAN_POINT('Ctrl Pts',(25.4512489060474,0.000557793871117651,
12.6480025703997));
#40458=CARTESIAN_POINT('Ctrl Pts',(25.2761532109731,0.000795927984841995,
12.3850804994989));
#40459=CARTESIAN_POINT('Ctrl Pts',(25.0385405727546,0.00107944402204348,
12.0284981506081));
#40460=CARTESIAN_POINT('Ctrl Pts',(24.5346770904967,0.00153952329737014,
11.2801401659155));
#40461=CARTESIAN_POINT('Ctrl Pts',(23.7748717062593,0.00195060306715209,
10.1720733370841));
#40462=CARTESIAN_POINT('Ctrl Pts',(22.5874547933106,0.00176250665503241,
8.52818644438044));
#40463=CARTESIAN_POINT('Ctrl Pts',(21.7214346225638,0.00113305483753488,
7.38990420970681));
#40464=CARTESIAN_POINT('Ctrl Pts',(21.143061504949,0.000717013383189635,
6.63001173766479));
#40465=CARTESIAN_POINT('',(16.6859947282585,-0.000213685071588365,0.653010349651272));
#40466=CARTESIAN_POINT('Ctrl Pts',(21.143061504949,0.000717013383189635,
6.63001173766479));
#40467=CARTESIAN_POINT('Ctrl Pts',(21.0596090213757,0.000656984091852039,
6.5204775896832));
#40468=CARTESIAN_POINT('Ctrl Pts',(20.9749493812227,0.000581686629534018,
6.40937966448351));
#40469=CARTESIAN_POINT('Ctrl Pts',(20.8887163398544,0.000503337030319878,
6.29615377755028));
#40470=CARTESIAN_POINT('Ctrl Pts',(20.8782653958811,0.000493841513766926,
6.28243145740597));
#40471=CARTESIAN_POINT('Ctrl Pts',(20.8677913737256,0.000484599446368201,
6.26867792435866));
#40472=CARTESIAN_POINT('Ctrl Pts',(20.8572936227993,0.000475319602753722,
6.25489217579666));
#40473=CARTESIAN_POINT('Ctrl Pts',(20.7639844529272,0.000392835791668964,
6.13235766688846));
#40474=CARTESIAN_POINT('Ctrl Pts',(20.6688013656666,0.00030697584799982,
6.00727901155367));
#40475=CARTESIAN_POINT('Ctrl Pts',(20.5713613914627,0.000230367938072254,
5.87904920835524));
#40476=CARTESIAN_POINT('Ctrl Pts',(20.4390491065871,0.000126343201973351,
5.70492787479612));
#40477=CARTESIAN_POINT('Ctrl Pts',(20.302572845078,4.62809998690632E-5,
5.52499310762258));
#40478=CARTESIAN_POINT('Ctrl Pts',(20.1609437810453,2.88128682006106E-5,
5.33768334477713));
#40479=CARTESIAN_POINT('Ctrl Pts',(20.1049955882517,2.19123749649575E-5,
5.26368975599391));
#40480=CARTESIAN_POINT('Ctrl Pts',(20.0482435177667,2.45223961111146E-5,
5.18854554072461));
#40481=CARTESIAN_POINT('Ctrl Pts',(19.9906274051637,3.89817441291494E-5,
5.11215529601011));
#40482=CARTESIAN_POINT('Ctrl Pts',(19.9637371164834,4.57301348963764E-5,
5.0765028432512));
#40483=CARTESIAN_POINT('Ctrl Pts',(19.9366587691311,5.50600375822944E-5,
5.04057917079713));
#40484=CARTESIAN_POINT('Ctrl Pts',(19.9093864780487,6.75721501229822E-5,
5.00437426454754));
#40485=CARTESIAN_POINT('Ctrl Pts',(19.8219754132208,0.000107675017795418,
4.88833306369241));
#40486=CARTESIAN_POINT('Ctrl Pts',(19.7325741562302,0.000181835093669053,
4.76940538345263));
#40487=CARTESIAN_POINT('Ctrl Pts',(19.640991672691,0.00030893622753794,
4.64726735002378));
#40488=CARTESIAN_POINT('Ctrl Pts',(19.6046361822504,0.00035939155347774,
4.5987822256294));
#40489=CARTESIAN_POINT('Ctrl Pts',(19.5679372662935,0.000418182392978269,
4.54979164217064));
#40490=CARTESIAN_POINT('Ctrl Pts',(19.5308843034958,0.000486453624597445,
4.50027729897209));
#40491=CARTESIAN_POINT('Ctrl Pts',(19.4649269930547,0.000607982012022067,
4.41213771014967));
#40492=CARTESIAN_POINT('Ctrl Pts',(19.3979604575256,0.000755754893077826,
4.32248935160143));
#40493=CARTESIAN_POINT('Ctrl Pts',(19.32967497191,0.000939646903500107,
4.23089537491404));
#40494=CARTESIAN_POINT('Ctrl Pts',(19.3260653667936,0.000949367527666284,
4.22605367123578));
#40495=CARTESIAN_POINT('Ctrl Pts',(19.3224520692927,0.000959189247964836,
4.22120652086859));
#40496=CARTESIAN_POINT('Ctrl Pts',(19.3188350312757,0.000969113583970318,
4.21635385578221));
#40497=CARTESIAN_POINT('Ctrl Pts',(19.2777054431015,0.00108196389156541,
4.16117386718128));
#40498=CARTESIAN_POINT('Ctrl Pts',(19.2360924231322,0.00120807388850654,
4.10528115905047));
#40499=CARTESIAN_POINT('Ctrl Pts',(19.1941052786264,0.00134680194697621,
4.04882712612678));
#40500=CARTESIAN_POINT('Ctrl Pts',(19.1255959475606,0.00157316090988453,
3.95671254969881));
#40501=CARTESIAN_POINT('Ctrl Pts',(19.0558951897339,0.00183348354698827,
3.86284161002992));
#40502=CARTESIAN_POINT('Ctrl Pts',(18.9849352541343,0.00212458137739411,
3.76713326639925));
#40503=CARTESIAN_POINT('Ctrl Pts',(18.9473688786483,0.00227868933011117,
3.71646501897776));
#40504=CARTESIAN_POINT('Ctrl Pts',(18.9100686735636,0.00243890737907993,
3.66611665801017));
#40505=CARTESIAN_POINT('Ctrl Pts',(18.8730284743227,0.00260445671863931,
3.61608395584742));
#40506=CARTESIAN_POINT('Ctrl Pts',(18.7755646591026,0.00304006642299761,
3.48443298910044));
#40507=CARTESIAN_POINT('Ctrl Pts',(18.679648004789,0.00351385896967246,
3.35462748521827));
#40508=CARTESIAN_POINT('Ctrl Pts',(18.5857625174182,0.00401352288344629,
3.22736737383541));
#40509=CARTESIAN_POINT('Ctrl Pts',(18.535886146263,0.00427896777289746,
3.15976083818942));
#40510=CARTESIAN_POINT('Ctrl Pts',(18.4865835643325,0.0045518186419106,
3.0928728969965));
#40511=CARTESIAN_POINT('Ctrl Pts',(18.4376106715998,0.00482723791978553,
3.02638559791964));
#40512=CARTESIAN_POINT('Ctrl Pts',(18.3555927639463,0.00528849947976878,
2.9150352395573));
#40513=CARTESIAN_POINT('Ctrl Pts',(18.2748688846044,0.00575567155003901,
2.80530938048468));
#40514=CARTESIAN_POINT('Ctrl Pts',(18.1953681077857,0.0061993131329244,
2.69717844492762));
#40515=CARTESIAN_POINT('Ctrl Pts',(18.131947821558,0.00655322006685646,
2.61091897480016));
#40516=CARTESIAN_POINT('Ctrl Pts',(18.0693048287704,0.00689210898023805,
2.5256731902104));
#40517=CARTESIAN_POINT('Ctrl Pts',(18.0073887079404,0.00720102569903335,
2.44140765258671));
#40518=CARTESIAN_POINT('Ctrl Pts',(17.9720494218701,0.00737734320974101,
2.39331219860742));
#40519=CARTESIAN_POINT('Ctrl Pts',(17.9369644798575,0.00754381435446798,
2.3455599795844));
#40520=CARTESIAN_POINT('Ctrl Pts',(17.9021016613117,0.0076978459350133,
2.2981136802392));
#40521=CARTESIAN_POINT('Ctrl Pts',(17.7975276756785,0.00815987674499643,
2.15579447505053));
#40522=CARTESIAN_POINT('Ctrl Pts',(17.694951671179,0.00850987289057204,
2.01622713361538));
#40523=CARTESIAN_POINT('Ctrl Pts',(17.5943127853703,0.00864476446222271,
1.87944134538212));
#40524=CARTESIAN_POINT('Ctrl Pts',(17.4946689503696,0.00877832231513908,
1.74400800464469));
#40525=CARTESIAN_POINT('Ctrl Pts',(17.3968684248807,0.00870150263032668,
1.61122539970131));
#40526=CARTESIAN_POINT('Ctrl Pts',(17.3007553288245,0.00831336603052086,
1.48099171860255));
#40527=CARTESIAN_POINT('Ctrl Pts',(17.2909959501874,0.00827395441861914,
1.46776771628336));
#40528=CARTESIAN_POINT('Ctrl Pts',(17.2812539945132,0.00823132892112186,
1.45457003148099));
#40529=CARTESIAN_POINT('Ctrl Pts',(17.2715293155224,0.00818538078796312,
1.44139858314228));
#40530=CARTESIAN_POINT('Ctrl Pts',(17.2513591319137,0.00809007869283378,
1.41407937480295));
#40531=CARTESIAN_POINT('Ctrl Pts',(17.2312632696569,0.00798048367228278,
1.38687303087359));
#40532=CARTESIAN_POINT('Ctrl Pts',(17.211237278093,0.0078553703108523,1.3597745396171));
#40533=CARTESIAN_POINT('Ctrl Pts',(17.1601159789753,0.00753598749512902,
1.29059893486631));
#40534=CARTESIAN_POINT('Ctrl Pts',(17.1094635746198,0.00711965377695296,
1.22214448899761));
#40535=CARTESIAN_POINT('Ctrl Pts',(17.0592536261995,0.00658289176926766,
1.15439218065909));
#40536=CARTESIAN_POINT('Ctrl Pts',(16.9522296725837,0.00543876806429331,
1.00997618078031));
#40537=CARTESIAN_POINT('Ctrl Pts',(16.8472142918112,0.00375032947837653,
0.868748571791631));
#40538=CARTESIAN_POINT('Ctrl Pts',(16.7439590026656,0.00130420671304145,
0.730530474948701));
#40539=CARTESIAN_POINT('Ctrl Pts',(16.7246782284289,0.00084744424417522,
0.704721124718759));
#40540=CARTESIAN_POINT('Ctrl Pts',(16.7054587525926,0.000364295203661793,
0.679016585636762));
#40541=CARTESIAN_POINT('Ctrl Pts',(16.6862988702478,-0.00014658020414501,
0.653415534774706));
#40542=CARTESIAN_POINT('',(11.7470010947906,-1.24897189209217,-5.16040757331412));
#40543=CARTESIAN_POINT('Ctrl Pts',(16.6859947282585,-0.000213685071588365,
0.653010349651272));
#40544=CARTESIAN_POINT('Ctrl Pts',(16.4192854137287,-0.0072433137319682,
0.300858250357417));
#40545=CARTESIAN_POINT('Ctrl Pts',(15.9095207379221,-0.0351396207084642,
-0.370166803666931));
#40546=CARTESIAN_POINT('Ctrl Pts',(15.1895782981127,-0.127632624932323,
-1.30811589893802));
#40547=CARTESIAN_POINT('Ctrl Pts',(14.4478451522131,-0.294302251982803,
-2.24397964816492));
#40548=CARTESIAN_POINT('Ctrl Pts',(13.3092516261401,-0.649917867944524,
-3.60699541669691));
#40549=CARTESIAN_POINT('Ctrl Pts',(12.4232261256394,-1.01937922958051,-4.52402251923096));
#40550=CARTESIAN_POINT('Ctrl Pts',(11.7470010949101,-1.24897189262897,-5.16040757324743));
#40551=CARTESIAN_POINT('Ctrl Pts',(11.7470010949101,-1.24897189262897,-5.16040757324743));
#40552=CARTESIAN_POINT('Ctrl Pts',(10.7125397951466,-1.59144123476306,-6.0634775436082));
#40553=CARTESIAN_POINT('Ctrl Pts',(9.24118021009056,-1.93913982160653,-6.97487125430323));
#40554=CARTESIAN_POINT('Ctrl Pts',(7.87873760695008,-2.09354224390961,-7.58570787305198));
#40555=CARTESIAN_POINT('Ctrl Pts',(7.28211573159564,-2.13599647613335,-7.80368259116433));
#40556=CARTESIAN_POINT('Ctrl Pts',(6.7745203245172,-2.15695778989224,-7.96476246664597));
#40557=CARTESIAN_POINT('Ctrl Pts',(6.29786588949097,-2.16773371799523,-8.09674109067091));
#40558=CARTESIAN_POINT('Ctrl Pts',(5.00815621212858,-2.16216752644387,-8.38292053232245));
#40559=CARTESIAN_POINT('Ctrl Pts',(3.22852047111695,-2.04767166606362,-8.49451211875645));
#40560=CARTESIAN_POINT('Ctrl Pts',(1.19527622155365,-1.93132215124059,-8.55306594389669));
#40561=CARTESIAN_POINT('Ctrl Pts',(6.41902973990636E-15,-1.93207323326078,
-8.62957429809281));
#40562=CARTESIAN_POINT('',(-36.1915542569364,0.0787940302150566,-5.40804187715572));
#40563=CARTESIAN_POINT('',(-35.11517701784,0.0508510909662735,-2.65562493453964));
#40564=CARTESIAN_POINT('Ctrl Pts',(-36.190739898305,0.0787719633382659,
-5.40642988539957));
#40565=CARTESIAN_POINT('Ctrl Pts',(-35.7431048645438,0.0666427433527001,
-4.52019980252406));
#40566=CARTESIAN_POINT('Ctrl Pts',(-35.3838115012789,0.0575373937785139,
-3.5969362359802));
#40567=CARTESIAN_POINT('Ctrl Pts',(-35.11517701784,0.0508510909662703,-2.65562493453964));
#40568=CARTESIAN_POINT('',(-41.6364777727387,0.319028652933056,-11.5323619171013));
#40569=CARTESIAN_POINT('Ctrl Pts',(-41.6333832694247,0.318726115297504,
-11.530271378588));
#40570=CARTESIAN_POINT('Ctrl Pts',(-40.469472385245,0.204977053081564,-10.7437628031316));
#40571=CARTESIAN_POINT('Ctrl Pts',(-38.3559078896116,0.147573716864128,
-8.89963534126349));
#40572=CARTESIAN_POINT('Ctrl Pts',(-36.8151557983613,0.095692551513825,
-6.64222332188911));
#40573=CARTESIAN_POINT('Ctrl Pts',(-36.1917138133952,0.0787983537557951,
-5.4083577130619));
#40574=CARTESIAN_POINT('',(-58.6294249853169,3.50507048772823,-12.1300984569962));
#40575=CARTESIAN_POINT('Ctrl Pts',(-58.6294249853169,3.50507048772823,-12.1300984569962));
#40576=CARTESIAN_POINT('Ctrl Pts',(-57.9716624173195,3.44148099145208,-12.5594172014826));
#40577=CARTESIAN_POINT('Ctrl Pts',(-56.9350672575427,3.39429553816601,-13.1429311762582));
#40578=CARTESIAN_POINT('Ctrl Pts',(-54.8001566067438,3.30035269345341,-14.0186136905654));
#40579=CARTESIAN_POINT('Ctrl Pts',(-52.5620566289039,3.10483667886162,-14.5433464527275));
#40580=CARTESIAN_POINT('Ctrl Pts',(-49.295584910841,2.34465836914774,-14.632672959566));
#40581=CARTESIAN_POINT('Ctrl Pts',(-46.4621628306032,1.23462273661855,-14.0012119190018));
#40582=CARTESIAN_POINT('Ctrl Pts',(-43.6129610195816,0.540799292570524,
-12.7246728134981));
#40583=CARTESIAN_POINT('Ctrl Pts',(-42.2733694331884,0.381318100537509,
-11.9625083064448));
#40584=CARTESIAN_POINT('Ctrl Pts',(-41.6364777727387,0.319028652933056,
-11.5323619171013));
#40585=CARTESIAN_POINT('',(-64.2985865890396,3.08034664292734,-5.85430278968146));
#40586=CARTESIAN_POINT('Ctrl Pts',(-64.2984271691748,3.08038932251095,-5.85463968857846));
#40587=CARTESIAN_POINT('Ctrl Pts',(-64.2149763686856,3.10273760294942,-6.03098199576973));
#40588=CARTESIAN_POINT('Ctrl Pts',(-63.5361674281905,3.32898348528657,-7.40198206074098));
#40589=CARTESIAN_POINT('Ctrl Pts',(-62.3504191551611,3.80834832178581,-9.12254403970273));
#40590=CARTESIAN_POINT('Ctrl Pts',(-60.6939165981419,3.73345458801685,-10.6556781858428));
#40591=CARTESIAN_POINT('Ctrl Pts',(-59.5525626426981,3.61048189569459,-11.5252172226885));
#40592=CARTESIAN_POINT('Ctrl Pts',(-58.9445304645418,3.53557780820992,-11.9244241512045));
#40593=CARTESIAN_POINT('Ctrl Pts',(-58.6320070381566,3.50532029143236,-12.1284131364863));
#40594=CARTESIAN_POINT('',(-65.940882311202,3.18169312325483,0.560736956423784));
#40595=CARTESIAN_POINT('Ctrl Pts',(-65.9408665795194,3.18169905920862,0.560433515178698));
#40596=CARTESIAN_POINT('Ctrl Pts',(-65.9143728994958,3.19163129587113,0.0501692994464946));
#40597=CARTESIAN_POINT('Ctrl Pts',(-65.7949103863174,3.14832895362465,-1.25211448306953));
#40598=CARTESIAN_POINT('Ctrl Pts',(-65.3271399010989,2.96188037443542,-3.39681624176221));
#40599=CARTESIAN_POINT('Ctrl Pts',(-64.6778756435701,2.97883584484194,-5.05270118071992));
#40600=CARTESIAN_POINT('Ctrl Pts',(-64.2988876471629,3.08026604421803,-5.85366656941012));
#40601=CARTESIAN_POINT('',(-65.1818229259373,3.08339058983654,6.62273332431001));
#40602=CARTESIAN_POINT('Ctrl Pts',(-65.1820138144051,3.08344362593875,6.62193263425266));
#40603=CARTESIAN_POINT('Ctrl Pts',(-65.2023991572908,3.0862917576968,6.56019789543742));
#40604=CARTESIAN_POINT('Ctrl Pts',(-65.2223744107905,3.08902484343314,6.49853102562792));
#40605=CARTESIAN_POINT('Ctrl Pts',(-65.2419378771287,3.09164815398979,6.43685530311948));
#40606=CARTESIAN_POINT('Ctrl Pts',(-65.2615689182929,3.09428052581152,6.37496654442693));
#40607=CARTESIAN_POINT('Ctrl Pts',(-65.2807853319273,3.09680238556488,6.31306895097167));
#40608=CARTESIAN_POINT('Ctrl Pts',(-65.2995864378602,3.0992186946728,6.25102614942384));
#40609=CARTESIAN_POINT('Ctrl Pts',(-65.328858256588,3.10298069476203,6.15443046793842));
#40610=CARTESIAN_POINT('Ctrl Pts',(-65.3571231565645,3.10648660394772,6.05746651472737));
#40611=CARTESIAN_POINT('Ctrl Pts',(-65.3843787248702,3.10975354311192,5.96022145009967));
#40612=CARTESIAN_POINT('Ctrl Pts',(-65.3919295545984,3.1106586095954,5.93328086619102));
#40613=CARTESIAN_POINT('Ctrl Pts',(-65.3994029474697,3.11154534378614,5.9063190073824));
#40614=CARTESIAN_POINT('Ctrl Pts',(-65.4067965504853,3.11241384365897,5.87933776802483));
#40615=CARTESIAN_POINT('Ctrl Pts',(-65.4502767239497,3.11752130277536,5.72066695961275));
#40616=CARTESIAN_POINT('Ctrl Pts',(-65.4910054802836,3.12199916303113,5.56133319312213));
#40617=CARTESIAN_POINT('Ctrl Pts',(-65.5290825875995,3.12593851324299,5.401417880817));
#40618=CARTESIAN_POINT('Ctrl Pts',(-65.5641348605888,3.12956492262019,5.25420619439375));
#40619=CARTESIAN_POINT('Ctrl Pts',(-65.5969413278409,3.13273509500721,5.10649720222318));
#40620=CARTESIAN_POINT('Ctrl Pts',(-65.6275443166768,3.13551583469991,4.95832938162754));
#40621=CARTESIAN_POINT('Ctrl Pts',(-65.6663255026627,3.13903968603937,4.77056589753007));
#40622=CARTESIAN_POINT('Ctrl Pts',(-65.7015662727776,3.14193797149757,4.58207020571463));
#40623=CARTESIAN_POINT('Ctrl Pts',(-65.7333517374092,3.14434707116289,4.39298046147203));
#40624=CARTESIAN_POINT('Ctrl Pts',(-65.7540687165909,3.14591726270142,4.26973644599696));
#40625=CARTESIAN_POINT('Ctrl Pts',(-65.7733177100259,3.14727965268877,4.14624240801174));
#40626=CARTESIAN_POINT('Ctrl Pts',(-65.7911247600377,3.1484722064521,4.02254559511262));
#40627=CARTESIAN_POINT('Ctrl Pts',(-65.7969314450796,3.14886108524418,3.9822094118193));
#40628=CARTESIAN_POINT('Ctrl Pts',(-65.8025848056586,3.14923190422925,3.9418518235844));
#40629=CARTESIAN_POINT('Ctrl Pts',(-65.8080857829282,3.14958597965166,3.90147479140268));
#40630=CARTESIAN_POINT('Ctrl Pts',(-65.8122533101222,3.14985422634299,3.87088524860251));
#40631=CARTESIAN_POINT('Ctrl Pts',(-65.8163333772144,3.15011286303388,3.84028454606075));
#40632=CARTESIAN_POINT('Ctrl Pts',(-65.8203264104579,3.1503624622411,3.80967353994764));
#40633=CARTESIAN_POINT('Ctrl Pts',(-65.8234339407524,3.1505567098345,3.78585089108904));
#40634=CARTESIAN_POINT('Ctrl Pts',(-65.8264893985082,3.1507455242109,3.76201719191869));
#40635=CARTESIAN_POINT('Ctrl Pts',(-65.8294939234993,3.15092922842115,3.73816463867714));
#40636=CARTESIAN_POINT('Ctrl Pts',(-65.8331602401737,3.15115339623844,3.70905820290531));
#40637=CARTESIAN_POINT('Ctrl Pts',(-65.8367502423687,3.15136992509179,3.67992730670294));
#40638=CARTESIAN_POINT('Ctrl Pts',(-65.8402641068065,3.15157928490807,3.65077229499262));
#40639=CARTESIAN_POINT('Ctrl Pts',(-65.8615591734033,3.15284806784186,3.47408422776829));
#40640=CARTESIAN_POINT('Ctrl Pts',(-65.8800565538659,3.15385321994246,3.29650470733162));
#40641=CARTESIAN_POINT('Ctrl Pts',(-65.8957954274969,3.15479469408719,3.11815426760985));
#40642=CARTESIAN_POINT('Ctrl Pts',(-65.9104251056954,3.15566981794246,2.95237305601382));
#40643=CARTESIAN_POINT('Ctrl Pts',(-65.9226716782155,3.15649018549394,2.78592275316682));
#40644=CARTESIAN_POINT('Ctrl Pts',(-65.9325836358646,3.15741782690276,2.61893372892488));
#40645=CARTESIAN_POINT('Ctrl Pts',(-65.9378901130687,3.15791445008898,2.52953429020231));
#40646=CARTESIAN_POINT('Ctrl Pts',(-65.9425278145653,3.15844183471541,2.43997962823197));
#40647=CARTESIAN_POINT('Ctrl Pts',(-65.9465061693714,3.15902460511505,2.35030054189828));
#40648=CARTESIAN_POINT('Ctrl Pts',(-65.9499589751705,3.15953039032363,2.27246825080328));
#40649=CARTESIAN_POINT('Ctrl Pts',(-65.9529154178099,3.16007791310227,2.19453831713516));
#40650=CARTESIAN_POINT('Ctrl Pts',(-65.9553831634599,3.16068322693473,2.11651288325481));
#40651=CARTESIAN_POINT('Ctrl Pts',(-65.9570020166317,3.16108031575857,2.06532781840632));
#40652=CARTESIAN_POINT('Ctrl Pts',(-65.9584105277869,3.16150225489745,2.01410341967322));
#40653=CARTESIAN_POINT('Ctrl Pts',(-65.9596098983724,3.1619500963955,1.96285658232393));
#40654=CARTESIAN_POINT('Ctrl Pts',(-65.9620404632496,3.1628576622711,1.85900314084093));
#40655=CARTESIAN_POINT('Ctrl Pts',(-65.9636135459671,3.16387181256393,1.7550240340113));
#40656=CARTESIAN_POINT('Ctrl Pts',(-65.9643350584048,3.16500289072531,1.6509649698538));
#40657=CARTESIAN_POINT('Ctrl Pts',(-65.9645966980952,3.16541304989168,1.61323037248798));
#40658=CARTESIAN_POINT('Ctrl Pts',(-65.9647462801353,3.16583859524181,1.57548525747449));
#40659=CARTESIAN_POINT('Ctrl Pts',(-65.9647838219684,3.16628005752532,1.53773183134651));
#40660=CARTESIAN_POINT('Ctrl Pts',(-65.964814152205,3.16663671713484,1.50723064761264));
#40661=CARTESIAN_POINT('Ctrl Pts',(-65.9647713681457,3.16700374895558,1.47672527941099));
#40662=CARTESIAN_POINT('Ctrl Pts',(-65.9646553256625,3.16738159960587,1.44620476843088));
#40663=CARTESIAN_POINT('Ctrl Pts',(-65.9645189092163,3.16782579074596,1.4103256702788));
#40664=CARTESIAN_POINT('Ctrl Pts',(-65.964281214949,3.1682848589196,1.37443237344843));
#40665=CARTESIAN_POINT('Ctrl Pts',(-65.9639422079975,3.16875903076749,1.33854708614654));
#40666=CARTESIAN_POINT('Ctrl Pts',(-65.9630174029551,3.17005256328616,1.24065264919655));
#40667=CARTESIAN_POINT('Ctrl Pts',(-65.9613372844884,3.17145872738211,1.14281766425937));
#40668=CARTESIAN_POINT('Ctrl Pts',(-65.9589158777346,3.17299774944126,1.04494380771358));
#40669=CARTESIAN_POINT('Ctrl Pts',(-65.9587830004562,3.17308220491834,1.03957287543947));
#40670=CARTESIAN_POINT('Ctrl Pts',(-65.9586478955613,3.17316705961954,1.03420182780611));
#40671=CARTESIAN_POINT('Ctrl Pts',(-65.958510566995,3.17325231657106,1.02883064941742));
#40672=CARTESIAN_POINT('Ctrl Pts',(-65.9583795817216,3.1733336354503,1.02370756914105));
#40673=CARTESIAN_POINT('Ctrl Pts',(-65.9582468049946,3.17341517649201,1.01859342997896));
#40674=CARTESIAN_POINT('Ctrl Pts',(-65.9581122745334,3.17349693078692,1.01348869045227));
#40675=CARTESIAN_POINT('Ctrl Pts',(-65.9566984971929,3.17435608468119,0.959843107075385));
#40676=CARTESIAN_POINT('Ctrl Pts',(-65.955093127377,3.17523907659001,0.907177309217897));
#40677=CARTESIAN_POINT('Ctrl Pts',(-65.9532671389238,3.17617002788351,0.854114316309088));
#40678=CARTESIAN_POINT('Ctrl Pts',(-65.9521293961761,3.17675008800426,0.821051656330386));
#40679=CARTESIAN_POINT('Ctrl Pts',(-65.9509051456926,3.17734891470678,0.787834642983174));
#40680=CARTESIAN_POINT('Ctrl Pts',(-65.9495788904456,3.17797408345389,0.754124291378267));
#40681=CARTESIAN_POINT('Ctrl Pts',(-65.9486209022187,3.17842565889602,0.729774438637609));
#40682=CARTESIAN_POINT('Ctrl Pts',(-65.9476094927885,3.17889112211251,0.705163238122186));
#40683=CARTESIAN_POINT('Ctrl Pts',(-65.9465425041965,3.17936386644549,0.680489633390043));
#40684=CARTESIAN_POINT('Ctrl Pts',(-65.9456241685326,3.17977074800368,0.659253557060112));
#40685=CARTESIAN_POINT('Ctrl Pts',(-65.9446646284688,3.18018304018358,0.637970848329328));
#40686=CARTESIAN_POINT('Ctrl Pts',(-65.9436620707991,3.1805956413506,0.616805703615335));
#40687=CARTESIAN_POINT('Ctrl Pts',(-65.9428109180125,3.18094593205576,0.598836890002149));
#40688=CARTESIAN_POINT('Ctrl Pts',(-65.9419287464167,3.1812964441945,0.58095295893464));
#40689=CARTESIAN_POINT('Ctrl Pts',(-65.9410143684102,3.18164329479668,0.563284147647862));
#40690=CARTESIAN_POINT('',(-61.4911136899846,2.54023943605001,12.6453526575845));
#40691=CARTESIAN_POINT('Ctrl Pts',(-61.492579746848,2.54044123593051,12.6438559805174));
#40692=CARTESIAN_POINT('Ctrl Pts',(-61.6274523636194,2.55900663594459,12.5061409518654));
#40693=CARTESIAN_POINT('Ctrl Pts',(-61.7598465090111,2.57732079123508,12.3659924353731));
#40694=CARTESIAN_POINT('Ctrl Pts',(-61.8897040632185,2.59541821568171,12.2235148275418));
#40695=CARTESIAN_POINT('Ctrl Pts',(-61.9897936428061,2.60936706613971,12.1136981599209));
#40696=CARTESIAN_POINT('Ctrl Pts',(-62.0883755887928,2.62318675732009,12.0024985721511));
#40697=CARTESIAN_POINT('Ctrl Pts',(-62.1854109821693,2.6368833832955,11.889978089556));
#40698=CARTESIAN_POINT('Ctrl Pts',(-62.3238252998524,2.65642067863669,11.7294753566682));
#40699=CARTESIAN_POINT('Ctrl Pts',(-62.4590940743637,2.67570916811489,11.566288083022));
#40700=CARTESIAN_POINT('Ctrl Pts',(-62.5910712856209,2.69473476474226,11.4005537560769));
#40701=CARTESIAN_POINT('Ctrl Pts',(-62.6611812893503,2.70484169636926,11.3125110237785));
#40702=CARTESIAN_POINT('Ctrl Pts',(-62.7303615707873,2.71487377663084,11.2237492830725));
#40703=CARTESIAN_POINT('Ctrl Pts',(-62.7985844799531,2.72482496592381,11.134287123968));
#40704=CARTESIAN_POINT('Ctrl Pts',(-62.9431636119667,2.74591369298148,10.9446974176723));
#40705=CARTESIAN_POINT('Ctrl Pts',(-63.0834410426147,2.76664159563338,10.751962951605));
#40706=CARTESIAN_POINT('Ctrl Pts',(-63.2191716943302,2.78691893809744,10.5562648470109));
#40707=CARTESIAN_POINT('Ctrl Pts',(-63.3535448424178,2.8069934776897,10.3625240076594));
#40708=CARTESIAN_POINT('Ctrl Pts',(-63.4834608710437,2.82662525100169,10.1658788201834));
#40709=CARTESIAN_POINT('Ctrl Pts',(-63.6087184396249,2.84569774795751,9.96648572222226));
#40710=CARTESIAN_POINT('Ctrl Pts',(-63.67949054989,2.85647394992979,9.85382610033401));
#40711=CARTESIAN_POINT('Ctrl Pts',(-63.7487762439001,2.86707116758227,9.74028885547898));
#40712=CARTESIAN_POINT('Ctrl Pts',(-63.8165455959749,2.87746643979862,9.62589900736996));
#40713=CARTESIAN_POINT('Ctrl Pts',(-63.9248200021698,2.89407486074408,9.4431395076914));
#40714=CARTESIAN_POINT('Ctrl Pts',(-64.0292220240533,2.91016730101018,9.25820452933871));
#40715=CARTESIAN_POINT('Ctrl Pts',(-64.1296563228998,2.92565150500005,9.07117745884888));
#40716=CARTESIAN_POINT('Ctrl Pts',(-64.2384680726629,2.94242728129537,8.86855003946347));
#40717=CARTESIAN_POINT('Ctrl Pts',(-64.3426275897165,2.95848842946922,8.66351672570398));
#40718=CARTESIAN_POINT('Ctrl Pts',(-64.4421008134935,2.97373763848325,8.4562287198291));
#40719=CARTESIAN_POINT('Ctrl Pts',(-64.5422735745952,2.98909408631466,8.24748297797682));
#40720=CARTESIAN_POINT('Ctrl Pts',(-64.6376943180403,3.003626370476,8.03645036383814));
#40721=CARTESIAN_POINT('Ctrl Pts',(-64.7283703588063,3.01726328798042,7.82326802272764));
#40722=CARTESIAN_POINT('Ctrl Pts',(-64.8217603485428,3.0313083606922,7.60370509871675));
#40723=CARTESIAN_POINT('Ctrl Pts',(-64.9101179346527,3.04440303516322,7.38186138031529));
#40724=CARTESIAN_POINT('Ctrl Pts',(-64.993488227946,3.0565104069069,7.15787463734448));
#40725=CARTESIAN_POINT('Ctrl Pts',(-65.0593066522129,3.06606882512404,6.98104361160777));
#40726=CARTESIAN_POINT('Ctrl Pts',(-65.1220175846494,3.07501276033487,6.80287657192886));
#40727=CARTESIAN_POINT('Ctrl Pts',(-65.181654605396,3.08334382396569,6.62343935220894));
#40728=CARTESIAN_POINT('',(-39.0604050365398,0.183119270849635,12.6471138640382));
#40729=CARTESIAN_POINT('Ctrl Pts',(-39.0604050365398,0.183119270849635,
12.6471138640382));
#40730=CARTESIAN_POINT('Ctrl Pts',(-39.0606668888501,0.183131142235521,
12.6473775711718));
#40731=CARTESIAN_POINT('Ctrl Pts',(-39.0609287502018,0.183143014646322,
12.6476412700229));
#40732=CARTESIAN_POINT('Ctrl Pts',(-39.0611906205948,0.183154888082176,
12.6479049605897));
#40733=CARTESIAN_POINT('Ctrl Pts',(-39.2840366840252,0.193258926222401,
12.8722999526221));
#40734=CARTESIAN_POINT('Ctrl Pts',(-39.5128971796941,0.204080431476651,
13.0905291572134));
#40735=CARTESIAN_POINT('Ctrl Pts',(-39.7477834050656,0.215700609772212,
13.3015853068891));
#40736=CARTESIAN_POINT('Ctrl Pts',(-39.902683352274,0.223363745410276,13.4407700819481));
#40737=CARTESIAN_POINT('Ctrl Pts',(-40.0602034639206,0.231374318042895,
13.5768350566888));
#40738=CARTESIAN_POINT('Ctrl Pts',(-40.2203420197422,0.239753276541817,
13.7094884715307));
#40739=CARTESIAN_POINT('Ctrl Pts',(-40.4916274961205,0.253947795383785,
13.9342122718297));
#40740=CARTESIAN_POINT('Ctrl Pts',(-40.7702788233318,0.269192848806674,
14.1490879279519));
#40741=CARTESIAN_POINT('Ctrl Pts',(-41.0556719421123,0.285548471670355,
14.3539554115054));
#40742=CARTESIAN_POINT('Ctrl Pts',(-41.085318076012,0.287247464930951,14.3752366844214));
#40743=CARTESIAN_POINT('Ctrl Pts',(-41.1150369180175,0.288958427338304,
14.3964099463438));
#40744=CARTESIAN_POINT('Ctrl Pts',(-41.1448277413998,0.290681415935031,
14.4174750072174));
#40745=CARTESIAN_POINT('Ctrl Pts',(-41.4545942194746,0.308597137918321,
14.6365105683868));
#40746=CARTESIAN_POINT('Ctrl Pts',(-41.7721472637896,0.327815031465181,
14.8438489703323));
#40747=CARTESIAN_POINT('Ctrl Pts',(-42.0966485620468,0.348385513803167,
15.0392663439725));
#40748=CARTESIAN_POINT('Ctrl Pts',(-42.2446048226632,0.357764618485189,
15.1283668314546));
#40749=CARTESIAN_POINT('Ctrl Pts',(-42.3940049066234,0.367424596614065,
15.2149888136249));
#40750=CARTESIAN_POINT('Ctrl Pts',(-42.5447664170058,0.377368657537596,
15.2991099938131));
#40751=CARTESIAN_POINT('Ctrl Pts',(-42.7671859547678,0.392039201952269,
15.423214574392));
#40752=CARTESIAN_POINT('Ctrl Pts',(-42.9925689275241,0.407328091485488,
15.5418760411507));
#40753=CARTESIAN_POINT('Ctrl Pts',(-43.2206488887303,0.423241653007795,
15.6550241882715));
#40754=CARTESIAN_POINT('Ctrl Pts',(-43.6176817449801,0.450943371084633,
15.8519881468463));
#40755=CARTESIAN_POINT('Ctrl Pts',(-44.0228896448743,0.480539226963428,
16.032246467644));
#40756=CARTESIAN_POINT('Ctrl Pts',(-44.4348255327009,0.512045625941868,
16.1954177560798));
#40757=CARTESIAN_POINT('Ctrl Pts',(-44.7387179971087,0.535288459385418,
16.3157921309005));
#40758=CARTESIAN_POINT('Ctrl Pts',(-45.0462708019942,0.559570753892732,
16.426866915952));
#40759=CARTESIAN_POINT('Ctrl Pts',(-45.3568885891016,0.5848900031984,16.5284829339606));
#40760=CARTESIAN_POINT('Ctrl Pts',(-45.7630705890824,0.617998935615831,
16.6613619870541));
#40761=CARTESIAN_POINT('Ctrl Pts',(-46.1744954614692,0.65288278895461,16.77806697134));
#40762=CARTESIAN_POINT('Ctrl Pts',(-46.5898247303867,0.689544215461607,
16.8782249009176));
#40763=CARTESIAN_POINT('Ctrl Pts',(-47.0240057882049,0.727869703533806,
16.9829289973234));
#40764=CARTESIAN_POINT('Ctrl Pts',(-47.4624513529612,0.768138554332072,
17.0695489583781));
#40765=CARTESIAN_POINT('Ctrl Pts',(-47.9036097711811,0.810306044668031,
17.1376550430375));
#40766=CARTESIAN_POINT('Ctrl Pts',(-47.9500332036625,0.814743361422456,
17.1448218976008));
#40767=CARTESIAN_POINT('Ctrl Pts',(-47.99648667759,0.819201655130773,17.1517837424007));
#40768=CARTESIAN_POINT('Ctrl Pts',(-48.0429683888055,0.823680839660802,
17.1585400804775));
#40769=CARTESIAN_POINT('Ctrl Pts',(-48.0905363285643,0.828264698006835,
17.1654543070458));
#40770=CARTESIAN_POINT('Ctrl Pts',(-48.1381338407373,0.832870435007399,
17.1721533097098));
#40771=CARTESIAN_POINT('Ctrl Pts',(-48.1857589944567,0.837497951118463,
17.1786365573383));
#40772=CARTESIAN_POINT('Ctrl Pts',(-48.5894375001487,0.876721526118069,
17.2335896128204));
#40773=CARTESIAN_POINT('Ctrl Pts',(-48.9950997343204,0.917513509102992,
17.273040738628));
#40774=CARTESIAN_POINT('Ctrl Pts',(-49.4015504710882,0.959821260145756,
17.2966290468743));
#40775=CARTESIAN_POINT('Ctrl Pts',(-49.70885328167,0.991808631870625,17.3144633199245));
#40776=CARTESIAN_POINT('Ctrl Pts',(-50.0166070974792,1.02466130307784,17.3232301877965));
#40777=CARTESIAN_POINT('Ctrl Pts',(-50.3243092135675,1.0583429324575,17.3227777244192));
#40778=CARTESIAN_POINT('Ctrl Pts',(-50.5598248881171,1.08412290356764,17.3224314082519));
#40779=CARTESIAN_POINT('Ctrl Pts',(-50.7953336343792,1.11039082495756,17.3167118478853));
#40780=CARTESIAN_POINT('Ctrl Pts',(-51.0305863517201,1.13712426615352,17.3056788143251));
#40781=CARTESIAN_POINT('Ctrl Pts',(-51.4761245154068,1.18775393978326,17.2847836783712));
#40782=CARTESIAN_POINT('Ctrl Pts',(-51.9207412909683,1.24005387209177,17.2448303381155));
#40783=CARTESIAN_POINT('Ctrl Pts',(-52.3625858524104,1.2936972330631,17.1862403088709));
#40784=CARTESIAN_POINT('Ctrl Pts',(-52.4264742939416,1.30145378600056,17.1777684932499));
#40785=CARTESIAN_POINT('Ctrl Pts',(-52.4903048604507,1.30923840713047,17.1689070336471));
#40786=CARTESIAN_POINT('Ctrl Pts',(-52.5540720323581,1.31705009289058,17.1596572113284));
#40787=CARTESIAN_POINT('Ctrl Pts',(-53.003553927648,1.37211308558476,17.0944570849539));
#40788=CARTESIAN_POINT('Ctrl Pts',(-53.4498856007116,1.42852058127125,17.0099600355678));
#40789=CARTESIAN_POINT('Ctrl Pts',(-53.8911418598714,1.48592156034486,16.9066194449686));
#40790=CARTESIAN_POINT('Ctrl Pts',(-53.9875034657967,1.49845679448691,16.8840519117934));
#40791=CARTESIAN_POINT('Ctrl Pts',(-54.0836230056315,1.51103942881208,16.8605857879481));
#40792=CARTESIAN_POINT('Ctrl Pts',(-54.1794803052346,1.52366130162109,16.8362272941616));
#40793=CARTESIAN_POINT('Ctrl Pts',(-54.5812987873487,1.57657017548416,16.7341203806515));
#40794=CARTESIAN_POINT('Ctrl Pts',(-54.9787920780597,1.63020748646383,16.6159478440198));
#40795=CARTESIAN_POINT('Ctrl Pts',(-55.3707700094445,1.68400548366404,16.4823550595151));
#40796=CARTESIAN_POINT('Ctrl Pts',(-55.7254062830265,1.73267843110742,16.361488950786));
#40797=CARTESIAN_POINT('Ctrl Pts',(-56.0755280958839,1.78148331561148,16.2280022066449));
#40798=CARTESIAN_POINT('Ctrl Pts',(-56.4202194358333,1.82997079988972,16.0823687023087));
#40799=CARTESIAN_POINT('Ctrl Pts',(-56.5357517080917,1.84622264200326,16.0335558436062));
#40800=CARTESIAN_POINT('Ctrl Pts',(-56.6506736005584,1.86243855447853,15.9833782377977));
#40801=CARTESIAN_POINT('Ctrl Pts',(-56.7649497587316,1.87860083920917,15.9318530432299));
#40802=CARTESIAN_POINT('Ctrl Pts',(-56.9620517553632,1.90647733279682,15.8429830734261));
#40803=CARTESIAN_POINT('Ctrl Pts',(-57.1572326127867,1.9341941425919,15.7501044856584));
#40804=CARTESIAN_POINT('Ctrl Pts',(-57.3503735845836,1.96167081317485,15.6532998685256));
#40805=CARTESIAN_POINT('Ctrl Pts',(-57.62978046508,2.00141986663867,15.513257722941));
#40806=CARTESIAN_POINT('Ctrl Pts',(-57.9049183209555,2.04066520647406,15.3650015932308));
#40807=CARTESIAN_POINT('Ctrl Pts',(-58.1754298370156,2.07917259253651,15.2087506681607));
#40808=CARTESIAN_POINT('Ctrl Pts',(-58.4302797952656,2.11545055169057,15.0615460599776));
#40809=CARTESIAN_POINT('Ctrl Pts',(-58.6810244436519,2.15107239926173,14.9072461379215));
#40810=CARTESIAN_POINT('Ctrl Pts',(-58.9273599534012,2.18586651354731,14.7459925951525));
#40811=CARTESIAN_POINT('Ctrl Pts',(-59.1409340208908,2.21603317738004,14.6061850007812));
#40812=CARTESIAN_POINT('Ctrl Pts',(-59.3511944237414,2.24557728638283,14.461150039835));
#40813=CARTESIAN_POINT('Ctrl Pts',(-59.5579291538172,2.27441462267184,14.3109480361353));
#40814=CARTESIAN_POINT('Ctrl Pts',(-59.5896414679669,2.27883815938143,14.2879076252402));
#40815=CARTESIAN_POINT('Ctrl Pts',(-59.6212707800306,2.28324513082026,14.2647455684019));
#40816=CARTESIAN_POINT('Ctrl Pts',(-59.6528162738773,2.28763530890052,14.241462012894));
#40817=CARTESIAN_POINT('Ctrl Pts',(-59.8518978018344,2.31534143277572,14.094521032058));
#40818=CARTESIAN_POINT('Ctrl Pts',(-60.047644383031,2.34237709488712,13.9427405811155));
#40819=CARTESIAN_POINT('Ctrl Pts',(-60.2398413018096,2.36880093753368,13.7861505347015));
#40820=CARTESIAN_POINT('Ctrl Pts',(-60.4212087887707,2.39373591550897,13.6383836330169));
#40821=CARTESIAN_POINT('Ctrl Pts',(-60.5994160124284,2.41812677579402,13.4863335428754));
#40822=CARTESIAN_POINT('Ctrl Pts',(-60.7742400315841,2.44203497255451,13.3300325388928));
#40823=CARTESIAN_POINT('Ctrl Pts',(-60.9362372604305,2.46418903147968,13.1851992966795));
#40824=CARTESIAN_POINT('Ctrl Pts',(-61.0953297847282,2.48592927582932,13.0367159414217));
#40825=CARTESIAN_POINT('Ctrl Pts',(-61.251296640164,2.50730614462313,12.8846171702282));
#40826=CARTESIAN_POINT('Ctrl Pts',(-61.3318896415521,2.51835224805042,12.8060229301655));
#40827=CARTESIAN_POINT('Ctrl Pts',(-61.4116472956318,2.52930129871605,12.7264634937059));
#40828=CARTESIAN_POINT('Ctrl Pts',(-61.4905336880022,2.54015959990334,12.6459447735438));
#40829=CARTESIAN_POINT('',(-35.3373097934181,0.0544178896829728,6.63137155234305));
#40830=CARTESIAN_POINT('Ctrl Pts',(-35.3376973936001,0.0544271591152199,
6.63251752009926));
#40831=CARTESIAN_POINT('Ctrl Pts',(-35.8138531895274,0.0658148084159087,
8.03995386779416));
#40832=CARTESIAN_POINT('Ctrl Pts',(-36.9028760126082,0.0948092812359606,
10.1871843261409));
#40833=CARTESIAN_POINT('Ctrl Pts',(-38.4270467968691,0.154379143867951,
12.0091830811851));
#40834=CARTESIAN_POINT('Ctrl Pts',(-39.059611759677,0.183132402525965,12.6463171581384));
#40835=CARTESIAN_POINT('',(-34.5485284593044,0.0369496769146498,0.611350965839471));
#40836=CARTESIAN_POINT('Ctrl Pts',(-34.5485283758344,0.03694967497705,0.611352241800955));
#40837=CARTESIAN_POINT('Ctrl Pts',(-34.4156250594086,0.0338645726825741,
2.642977068212));
#40838=CARTESIAN_POINT('Ctrl Pts',(-34.6822137461999,0.0387518832851432,
4.69404824512284));
#40839=CARTESIAN_POINT('Ctrl Pts',(-35.3369428780847,0.0544091149274879,
6.63028674082642));
#40840=CARTESIAN_POINT('Origin',(-42.8058228112322,0.246536164900552,0.301815738582165));
#40841=CARTESIAN_POINT('',(-2.90417482900993,-2.04618953971544,-29.4756275701078));
#40842=CARTESIAN_POINT('',(1.92208295535431,-2.10378908788117,-32.4806927333858));
#40843=CARTESIAN_POINT('Ctrl Pts',(-2.90469444443151,-2.04568606478228,
-29.4775763495009));
#40844=CARTESIAN_POINT('Ctrl Pts',(-3.02250615524581,-2.05288116339367,
-29.9513503562729));
#40845=CARTESIAN_POINT('Ctrl Pts',(-3.00491991129501,-2.09425330667714,
-30.9658956033376));
#40846=CARTESIAN_POINT('Ctrl Pts',(-2.22452399291722,-2.12061194796893,
-32.362721059084));
#40847=CARTESIAN_POINT('Ctrl Pts',(-0.907169341450753,-2.06911023237464,
-33.2201637931267));
#40848=CARTESIAN_POINT('Ctrl Pts',(0.615978874200203,-2.06181054642213,
-33.3001206932397));
#40849=CARTESIAN_POINT('Ctrl Pts',(1.5420796957956,-2.09550075658161,-32.818473935249));
#40850=CARTESIAN_POINT('Ctrl Pts',(1.92209690915283,-2.10352759449249,-32.4807021153953));
#40851=CARTESIAN_POINT('',(2.90362501667649,-2.04722624614018,-29.4766633543452));
#40852=CARTESIAN_POINT('Ctrl Pts',(2.90308452694824,-2.04719239277948,-29.474406698116));
#40853=CARTESIAN_POINT('Ctrl Pts',(2.88735153351078,-2.04620772726132,-29.4089081520382));
#40854=CARTESIAN_POINT('Ctrl Pts',(2.86940368652239,-2.04508734517392,-29.3434470545767));
#40855=CARTESIAN_POINT('Ctrl Pts',(2.84929693172628,-2.04383765038075,-29.2786192026188));
#40856=CARTESIAN_POINT('Ctrl Pts',(2.82919017693018,-2.04258795558759,-29.2137913506608));
#40857=CARTESIAN_POINT('Ctrl Pts',(2.80692451694612,-2.04120892472319,-29.1495967442315));
#40858=CARTESIAN_POINT('Ctrl Pts',(2.7825317098188,-2.03970656265669,-29.0861967026844));
#40859=CARTESIAN_POINT('Ctrl Pts',(2.73374609556417,-2.03670183852368,-28.9593966195901));
#40860=CARTESIAN_POINT('Ctrl Pts',(2.67645197152196,-2.03320240315436,-28.8357747958726));
#40861=CARTESIAN_POINT('Ctrl Pts',(2.61179122164448,-2.02932718705402,-28.7171887138959));
#40862=CARTESIAN_POINT('Ctrl Pts',(2.54713047176699,-2.02545197095368,-28.5986026319191));
#40863=CARTESIAN_POINT('Ctrl Pts',(2.47510323222483,-2.02119934730129,-28.4850522930688));
#40864=CARTESIAN_POINT('Ctrl Pts',(2.3955719043754,-2.01664372796269,-28.3761609709903));
#40865=CARTESIAN_POINT('Ctrl Pts',(2.31604057652597,-2.01208810862409,-28.2672696489119));
#40866=CARTESIAN_POINT('Ctrl Pts',(2.2290050097441,-2.00723040475461,-28.1630373398676));
#40867=CARTESIAN_POINT('Ctrl Pts',(2.13573747909507,-2.00226792456411,-28.0654780193846));
#40868=CARTESIAN_POINT('Ctrl Pts',(2.10510252136045,-2.00063793211297,-28.0334333663438));
#40869=CARTESIAN_POINT('Ctrl Pts',(2.07379026957427,-1.99899664908459,-28.0021082308194));
#40870=CARTESIAN_POINT('Ctrl Pts',(2.04183842704365,-1.99735154115993,-27.9715221607636));
#40871=CARTESIAN_POINT('Ctrl Pts',(1.96415372391943,-1.99335178056358,-27.8971580683097));
#40872=CARTESIAN_POINT('Ctrl Pts',(1.88268977963344,-1.98932850068838,-27.8271627986765));
#40873=CARTESIAN_POINT('Ctrl Pts',(1.79797339964551,-1.98539854586267,-27.7618102269358));
#40874=CARTESIAN_POINT('Ctrl Pts',(1.68751703571273,-1.9802745247403,-27.6766011156733));
#40875=CARTESIAN_POINT('Ctrl Pts',(1.57153248611584,-1.97531224434771,-27.5992844729345));
#40876=CARTESIAN_POINT('Ctrl Pts',(1.45116736980479,-1.97070354368304,-27.5304674892138));
#40877=CARTESIAN_POINT('Ctrl Pts',(1.3307473501235,-1.96609274080465,-27.4616191152993));
#40878=CARTESIAN_POINT('Ctrl Pts',(1.20594261715742,-1.96183640196311,-27.4012780911951));
#40879=CARTESIAN_POINT('Ctrl Pts',(1.07785376018322,-1.95810634097014,-27.3500520637452));
#40880=CARTESIAN_POINT('Ctrl Pts',(0.980716380361522,-1.95527761441273,
-27.3112043278632));
#40881=CARTESIAN_POINT('Ctrl Pts',(0.881689174663142,-1.95275119975537,
-27.2775986958651));
#40882=CARTESIAN_POINT('Ctrl Pts',(0.781235294330189,-1.95059127976565,
-27.2495003578474));
#40883=CARTESIAN_POINT('Ctrl Pts',(0.65354375093492,-1.94784570621304,-27.213783269205));
#40884=CARTESIAN_POINT('Ctrl Pts',(0.523559123780202,-1.94569474885112,
-27.1869677858605));
#40885=CARTESIAN_POINT('Ctrl Pts',(0.392452217526058,-1.94424311303873,
-27.1690991815742));
#40886=CARTESIAN_POINT('Ctrl Pts',(0.261961270808454,-1.94279829722498,
-27.1513145266199));
#40887=CARTESIAN_POINT('Ctrl Pts',(0.130357497803029,-1.94204670075839,
-27.1423928625267));
#40888=CARTESIAN_POINT('Ctrl Pts',(-0.0012244446283809,-1.94204416881763,
-27.1423803600789));
#40889=CARTESIAN_POINT('Ctrl Pts',(-0.132937227564624,-1.94204163435919,
-27.1423678451991));
#40890=CARTESIAN_POINT('Ctrl Pts',(-0.264629521271901,-1.94278968028664,
-27.1512822184035));
#40891=CARTESIAN_POINT('Ctrl Pts',(-0.395211802238616,-1.94423427599342,
-27.1691724987033));
#40892=CARTESIAN_POINT('Ctrl Pts',(-0.525191584400474,-1.94567220642233,
-27.1869802343238));
#40893=CARTESIAN_POINT('Ctrl Pts',(-0.654073098514614,-1.94779976552174,
-27.2136812604207));
#40894=CARTESIAN_POINT('Ctrl Pts',(-0.780761159825137,-1.95051665312194,
-27.2493254261413));
#40895=CARTESIAN_POINT('Ctrl Pts',(-0.905730503191791,-1.95319668197301,
-27.284486024061));
#40896=CARTESIAN_POINT('Ctrl Pts',(-1.02847993168707,-1.95644703883071,
-27.3283458553242));
#40897=CARTESIAN_POINT('Ctrl Pts',(-1.14812360802916,-1.9601403266743,-27.380250679094));
#40898=CARTESIAN_POINT('Ctrl Pts',(-1.26522460546488,-1.96375512440974,
-27.4310524165615));
#40899=CARTESIAN_POINT('Ctrl Pts',(-1.37935085255374,-1.96779375243808,
-27.4895608744682));
#40900=CARTESIAN_POINT('Ctrl Pts',(-1.48962667553174,-1.97211585340783,
-27.5551628282496));
#40901=CARTESIAN_POINT('Ctrl Pts',(-1.5966495103396,-1.97631045822345,-27.6188296127996));
#40902=CARTESIAN_POINT('Ctrl Pts',(-1.70004567430087,-1.98077163288984,
-27.6891776063067));
#40903=CARTESIAN_POINT('Ctrl Pts',(-1.79896953891725,-1.98535773050927,
-27.7656458759941));
#40904=CARTESIAN_POINT('Ctrl Pts',(-1.88227805225432,-1.98921990245508,
-27.8300434598311));
#40905=CARTESIAN_POINT('Ctrl Pts',(-1.96241327293777,-1.99316904229066,
-27.8987816629645));
#40906=CARTESIAN_POINT('Ctrl Pts',(-2.03883360446083,-1.99709174802028,
-27.9715254605583));
#40907=CARTESIAN_POINT('Ctrl Pts',(-2.07163284680243,-1.99877535463775,
-28.0027467520468));
#40908=CARTESIAN_POINT('Ctrl Pts',(-2.1037475964743,-2.00045425090691,-28.0347059052958));
#40909=CARTESIAN_POINT('Ctrl Pts',(-2.13513427484619,-2.00212021210337,
-28.0673759138912));
#40910=CARTESIAN_POINT('Ctrl Pts',(-2.23341005555917,-2.00733655373979,
-28.1696699687946));
#40911=CARTESIAN_POINT('Ctrl Pts',(-2.32464409832483,-2.01242717098687,
-28.2789336743929));
#40912=CARTESIAN_POINT('Ctrl Pts',(-2.40797105482908,-2.01720078911666,
-28.3945871456283));
#40913=CARTESIAN_POINT('Ctrl Pts',(-2.48245612953968,-2.02146787527885,
-28.4979685459206));
#40914=CARTESIAN_POINT('Ctrl Pts',(-2.5506222869504,-2.02548272140289,-28.6064554636897));
#40915=CARTESIAN_POINT('Ctrl Pts',(-2.61184466862664,-2.0291407687602,-28.7196209343883));
#40916=CARTESIAN_POINT('Ctrl Pts',(-2.68434196982149,-2.03347249440997,
-28.8536273384104));
#40917=CARTESIAN_POINT('Ctrl Pts',(-2.74710988830725,-2.037304020544,-28.9942033551653));
#40918=CARTESIAN_POINT('Ctrl Pts',(-2.79941817523428,-2.04052343290909,
-29.1362172253607));
#40919=CARTESIAN_POINT('Ctrl Pts',(-2.84069994926609,-2.04306419770141,
-29.2482947725946));
#40920=CARTESIAN_POINT('Ctrl Pts',(-2.87546707541627,-2.0452247984993,-29.3612672939009));
#40921=CARTESIAN_POINT('Ctrl Pts',(-2.90337385306132,-2.04696563544976,
-29.4726235687673));
#40922=CARTESIAN_POINT('Ctrl Pts',(1.92207267078475,-2.1039818201281,-32.4806858184279));
#40923=CARTESIAN_POINT('Ctrl Pts',(1.94570149082075,-2.10449565912181,-32.4596820712235));
#40924=CARTESIAN_POINT('Ctrl Pts',(1.96901911603971,-2.1049796930935,-32.4382919517595));
#40925=CARTESIAN_POINT('Ctrl Pts',(1.99201749223354,-2.10543071793912,-32.4165308998389));
#40926=CARTESIAN_POINT('Ctrl Pts',(2.06732876952195,-2.10690765948167,-32.3452714073658));
#40927=CARTESIAN_POINT('Ctrl Pts',(2.13921799697769,-2.10802702932969,-32.2700343379296));
#40928=CARTESIAN_POINT('Ctrl Pts',(2.20739068358619,-2.10870039618712,-32.191359200355));
#40929=CARTESIAN_POINT('Ctrl Pts',(2.27504610063264,-2.10936865378164,-32.1132810211224));
#40930=CARTESIAN_POINT('Ctrl Pts',(2.33904087107875,-2.10959750519711,-32.0318171289645));
#40931=CARTESIAN_POINT('Ctrl Pts',(2.39907206939851,-2.10934954213335,-31.9474917835656));
#40932=CARTESIAN_POINT('Ctrl Pts',(2.45953044016332,-2.10909981460393,-31.8625663924407));
#40933=CARTESIAN_POINT('Ctrl Pts',(2.51596829845644,-2.10836641745561,-31.7747390657846));
#40934=CARTESIAN_POINT('Ctrl Pts',(2.56806548722448,-2.10716268647844,-31.6845364347016));
#40935=CARTESIAN_POINT('Ctrl Pts',(2.62076318314301,-2.10594508049043,-31.5932940675744));
#40936=CARTESIAN_POINT('Ctrl Pts',(2.66901916924568,-2.10424639435496,-31.4996217130001));
#40937=CARTESIAN_POINT('Ctrl Pts',(2.71249669614725,-2.10213221353835,-31.4040494206905));
#40938=CARTESIAN_POINT('Ctrl Pts',(2.75731514920407,-2.09995282753284,-31.3055295047323));
#40939=CARTESIAN_POINT('Ctrl Pts',(2.79705536527492,-2.09733221388986,-31.2049911191522));
#40940=CARTESIAN_POINT('Ctrl Pts',(2.83134952205391,-2.09439377260728,-31.1029922953511));
#40941=CARTESIAN_POINT('Ctrl Pts',(2.8551918307538,-2.09235088160964,-31.0320797063708));
#40942=CARTESIAN_POINT('Ctrl Pts',(2.87640183846363,-2.09015549991434,-30.960460741654));
#40943=CARTESIAN_POINT('Ctrl Pts',(2.89485812731065,-2.08786139532915,-30.8883150573738));
#40944=CARTESIAN_POINT('Ctrl Pts',(2.90485621446488,-2.08661863966067,-30.8492325069643));
#40945=CARTESIAN_POINT('Ctrl Pts',(2.91404624218871,-2.08534708334318,-30.8099952396228));
#40946=CARTESIAN_POINT('Ctrl Pts',(2.92240935668647,-2.0840546461131,-30.7706352155149));
#40947=CARTESIAN_POINT('Ctrl Pts',(2.94423157437584,-2.08068223663669,-30.6679314901779));
#40948=CARTESIAN_POINT('Ctrl Pts',(2.96042458860711,-2.07716776638078,-30.5643979173112));
#40949=CARTESIAN_POINT('Ctrl Pts',(2.97105097182711,-2.07369775772111,-30.460872438973));
#40950=CARTESIAN_POINT('Ctrl Pts',(2.98105660782707,-2.07043045191757,-30.3633944700792));
#40951=CARTESIAN_POINT('Ctrl Pts',(2.98612711938388,-2.06720357050776,-30.265923986485));
#40952=CARTESIAN_POINT('Ctrl Pts',(2.98633045828053,-2.06416780224706,-30.1691214121975));
#40953=CARTESIAN_POINT('Ctrl Pts',(2.98636573781319,-2.06364109295896,-30.1523260541168));
#40954=CARTESIAN_POINT('Ctrl Pts',(2.98625453975004,-2.06312010372482,-30.1355506971481));
#40955=CARTESIAN_POINT('Ctrl Pts',(2.98599726747777,-2.06260556427644,-30.1187951986278));
#40956=CARTESIAN_POINT('Ctrl Pts',(2.98514166557009,-2.06089437740919,-30.0630719900135));
#40957=CARTESIAN_POINT('Ctrl Pts',(2.9826718792187,-2.05922215959374,-30.0064291308722));
#40958=CARTESIAN_POINT('Ctrl Pts',(2.97858161858244,-2.05764921751408,-29.949628457099));
#40959=CARTESIAN_POINT('Ctrl Pts',(2.97549374305047,-2.05646175055467,-29.9067477151756));
#40960=CARTESIAN_POINT('Ctrl Pts',(2.97148236537055,-2.05533058902833,-29.8637753993326));
#40961=CARTESIAN_POINT('Ctrl Pts',(2.96654581446586,-2.05427308936306,-29.8210264932436));
#40962=CARTESIAN_POINT('Ctrl Pts',(2.96231247261508,-2.05336622996333,-29.7843671461173));
#40963=CARTESIAN_POINT('Ctrl Pts',(2.95739877849598,-2.05251344145991,-29.7478747275606));
#40964=CARTESIAN_POINT('Ctrl Pts',(2.95180427171811,-2.05171931701828,-29.7121213665861));
#40965=CARTESIAN_POINT('Ctrl Pts',(2.94850476819136,-2.05125096180845,-29.69103490708));
#40966=CARTESIAN_POINT('Ctrl Pts',(2.94496846414992,-2.05080291548886,-29.6702049581298));
#40967=CARTESIAN_POINT('Ctrl Pts',(2.94119535400504,-2.05037525312523,-29.64973985319));
#40968=CARTESIAN_POINT('Ctrl Pts',(2.93747306284587,-2.04995335082869,-29.6295503871357));
#40969=CARTESIAN_POINT('Ctrl Pts',(2.93352030186384,-2.04955128589555,-29.609711353304));
#40970=CARTESIAN_POINT('Ctrl Pts',(2.92933714208969,-2.04916851502035,-29.5898408349141));
#40971=CARTESIAN_POINT('Ctrl Pts',(2.92545273819812,-2.048813081148,-29.5713894433516));
#40972=CARTESIAN_POINT('Ctrl Pts',(2.92136967055431,-2.04847427759482,-29.5529106469571));
#40973=CARTESIAN_POINT('Ctrl Pts',(2.91708804313664,-2.04815118292927,-29.5341422151136));
#40974=CARTESIAN_POINT('Ctrl Pts',(2.91287958321207,-2.04783360953504,-29.5156945115759));
#40975=CARTESIAN_POINT('Ctrl Pts',(2.9084792919759,-2.04753121099856,-29.4969665520236));
#40976=CARTESIAN_POINT('Ctrl Pts',(2.90388731009679,-2.04724267478498,-29.4777584835398));
#40977=CARTESIAN_POINT('',(-3.07785474838095,-2.05544258673707,-11.3802428859977));
#40978=CARTESIAN_POINT('',(-2.61114764827022,-2.0293363270777,-11.4114346363442));
#40979=CARTESIAN_POINT('Ctrl Pts',(-3.07785472543547,-2.0554425853949,-11.3802428874211));
#40980=CARTESIAN_POINT('Ctrl Pts',(-2.92178819655231,-2.04631362593077,
-11.3899240379752));
#40981=CARTESIAN_POINT('Ctrl Pts',(-2.76624123292387,-2.03739189066906,
-11.4002647340113));
#40982=CARTESIAN_POINT('Ctrl Pts',(-2.61113444695314,-2.02883635882995,
-11.4108058436411));
#40983=CARTESIAN_POINT('',(2.61122247994174,-2.02926323098797,-11.4125016806131));
#40984=CARTESIAN_POINT('Ctrl Pts',(2.61122237625547,-2.02965625320091,-11.4128346487702));
#40985=CARTESIAN_POINT('Ctrl Pts',(2.39875792985278,-2.01772426094543,-11.4270868286368));
#40986=CARTESIAN_POINT('Ctrl Pts',(2.1871564334896,-2.00643541293128,-11.4410322220247));
#40987=CARTESIAN_POINT('Ctrl Pts',(1.97613297653908,-1.99640438922013,-11.4539962913991));
#40988=CARTESIAN_POINT('Ctrl Pts',(1.91789246634328,-1.99363592003114,-11.4575742538943));
#40989=CARTESIAN_POINT('Ctrl Pts',(1.859695749177,-1.99096338945399,-11.4610776073231));
#40990=CARTESIAN_POINT('Ctrl Pts',(1.80153632549014,-1.98839997822234,-11.4644926311939));
#40991=CARTESIAN_POINT('Ctrl Pts',(1.59873281478295,-1.97946129272292,-11.4764009133992));
#40992=CARTESIAN_POINT('Ctrl Pts',(1.39638417062112,-1.9718500439803,-11.4872313448092));
#40993=CARTESIAN_POINT('Ctrl Pts',(1.19437115603402,-1.96568856683472,-11.4964386378558));
#40994=CARTESIAN_POINT('Ctrl Pts',(0.980675451148058,-1.9591707629969,-11.5061784013147));
#40995=CARTESIAN_POINT('Ctrl Pts',(0.767354975171277,-1.95427561618771,
-11.5141021933605));
#40996=CARTESIAN_POINT('Ctrl Pts',(0.554249877638709,-1.95113788380568,
-11.5196211009003));
#40997=CARTESIAN_POINT('Ctrl Pts',(0.369028086300903,-1.94841070168162,
-11.5244178981266));
#40998=CARTESIAN_POINT('Ctrl Pts',(0.183968471591849,-1.94701109754869,
-11.5273997130952));
#40999=CARTESIAN_POINT('Ctrl Pts',(-0.00104078931658883,-1.94701860388953,
-11.5282019238506));
#41000=CARTESIAN_POINT('Ctrl Pts',(-0.20445415490362,-1.94702685693614,
-11.5290839358583));
#41001=CARTESIAN_POINT('Ctrl Pts',(-0.407807096520058,-1.94873642445981,
-11.5273306514672));
#41002=CARTESIAN_POINT('Ctrl Pts',(-0.611415636147186,-1.95203148158355,
-11.5224797887525));
#41003=CARTESIAN_POINT('Ctrl Pts',(-0.809364164139178,-1.95523494106756,
-11.5177637727365));
#41004=CARTESIAN_POINT('Ctrl Pts',(-1.00739173111074,-1.95993310178898,
-11.5100789145489));
#41005=CARTESIAN_POINT('Ctrl Pts',(-1.20576775842101,-1.96602432643602,
-11.5003732163943));
#41006=CARTESIAN_POINT('Ctrl Pts',(-1.40414378573127,-1.97211555108305,
-11.4906675182397));
#41007=CARTESIAN_POINT('Ctrl Pts',(-1.60286886520362,-1.97959958284084,
-11.4789414813465));
#41008=CARTESIAN_POINT('Ctrl Pts',(-1.80218974550519,-1.98836758664635,
-11.4661962804132));
#41009=CARTESIAN_POINT('Ctrl Pts',(-1.99103922808684,-1.99667496006071,
-11.4541206534241));
#41010=CARTESIAN_POINT('Ctrl Pts',(-2.18042304860645,-2.00613336719599,
-11.4411345888113));
#41011=CARTESIAN_POINT('Ctrl Pts',(-2.37035555543366,-2.01629257404216,
-11.4281032174532));
#41012=CARTESIAN_POINT('Ctrl Pts',(-2.45052349742492,-2.02058063783243,
-11.4226028518731));
#41013=CARTESIAN_POINT('Ctrl Pts',(-2.53078895766986,-2.02499373517506,
-11.4170941227293));
#41014=CARTESIAN_POINT('Ctrl Pts',(-2.61115194137134,-2.02949891799445,
-11.411639121294));
#41015=CARTESIAN_POINT('',(3.07783214882012,-2.05593621639069,-11.3803366865443));
#41016=CARTESIAN_POINT('Ctrl Pts',(2.61122263327693,-2.02868201487814,-11.4120092747117));
#41017=CARTESIAN_POINT('Ctrl Pts',(2.76631582482945,-2.03712920349075,-11.4015963148637));
#41018=CARTESIAN_POINT('Ctrl Pts',(2.92183777297706,-2.04606748664476,-11.3909675841183));
#41019=CARTESIAN_POINT('Ctrl Pts',(3.07786335075085,-2.05541632542898,-11.3803478078873));
#41020=CARTESIAN_POINT('',(3.2359026159775,-2.06532548171789,-11.3703777985423));
#41021=CARTESIAN_POINT('Ctrl Pts',(3.07779520430534,-2.05655179109612,-11.3803235183648));
#41022=CARTESIAN_POINT('Ctrl Pts',(3.13041748499745,-2.0596409038771,-11.3767435349223));
#41023=CARTESIAN_POINT('Ctrl Pts',(3.18311592723968,-2.06275417483888,-11.3736233513253));
#41024=CARTESIAN_POINT('Ctrl Pts',(3.23586984059878,-2.06586860583926,-11.3703662673297));
#41025=CARTESIAN_POINT('',(3.23664856024641,-2.06541997225008,-17.2991999978929));
#41026=CARTESIAN_POINT('Ctrl Pts',(3.23664856024641,-2.06541997225008,-17.2991999978929));
#41027=CARTESIAN_POINT('Ctrl Pts',(3.23681728092954,-2.06558188082221,-17.1465460270592));
#41028=CARTESIAN_POINT('Ctrl Pts',(3.2378092903911,-2.06653538159817,-16.7935834100567));
#41029=CARTESIAN_POINT('Ctrl Pts',(3.24099557149147,-2.06963003990913,-16.2391544763694));
#41030=CARTESIAN_POINT('Ctrl Pts',(3.24554996678201,-2.07412283442935,-15.6358291186907));
#41031=CARTESIAN_POINT('Ctrl Pts',(3.25030484001515,-2.07889552730337,-15.0311078760445));
#41032=CARTESIAN_POINT('Ctrl Pts',(3.25441336551011,-2.08309603063915,-14.42527398279));
#41033=CARTESIAN_POINT('Ctrl Pts',(3.25707692954116,-2.08586417392827,-13.8179806012891));
#41034=CARTESIAN_POINT('Ctrl Pts',(3.25752083357516,-2.08636008311531,-13.2096246578577));
#41035=CARTESIAN_POINT('Ctrl Pts',(3.25495835163609,-2.0836979792605,-12.5981980422748));
#41036=CARTESIAN_POINT('Ctrl Pts',(3.24852404096208,-2.07718177263222,-11.9897144106618));
#41037=CARTESIAN_POINT('Ctrl Pts',(3.24098309020377,-2.06950210825037,-11.5754888699177));
#41038=CARTESIAN_POINT('Ctrl Pts',(3.23609357785739,-2.06492021774181,-11.3768457644699));
#41039=CARTESIAN_POINT('Ctrl Pts',(3.23601450783738,-2.06484630648251,-11.373619320441));
#41040=CARTESIAN_POINT('Ctrl Pts',(3.23593596564798,-2.06477284094976,-11.3703895318054));
#41041=CARTESIAN_POINT('',(3.23657188269419,-2.06534153551088,-17.9847374128284));
#41042=CARTESIAN_POINT('Ctrl Pts',(3.23664856024641,-2.06541997225008,-17.2991999978929));
#41043=CARTESIAN_POINT('Ctrl Pts',(3.23659586671488,-2.06536940622408,-17.3468756987971));
#41044=CARTESIAN_POINT('Ctrl Pts',(3.23656856170872,-2.06534326877989,-17.3945522866107));
#41045=CARTESIAN_POINT('Ctrl Pts',(3.23656896082705,-2.06534377018181,-17.6221221200761));
#41046=CARTESIAN_POINT('Ctrl Pts',(3.23657012615242,-2.06534337879792,-17.8038210873795));
#41047=CARTESIAN_POINT('Ctrl Pts',(3.23657188269388,-2.06534153551086,-17.9847374128284));
#41048=CARTESIAN_POINT('',(-2.61111949366609,-2.02928657753388,-17.9437023142098));
#41049=CARTESIAN_POINT('Ctrl Pts',(-2.6111194931606,-2.02928657750628,-17.9437023141764));
#41050=CARTESIAN_POINT('Ctrl Pts',(-1.57600593216534,-1.97277420562122,
-17.8752896129969));
#41051=CARTESIAN_POINT('Ctrl Pts',(0.353906469946108,-1.90148014402363,
-17.7529935172544));
#41052=CARTESIAN_POINT('Ctrl Pts',(2.29676905143962,-2.00870599133178,-17.924480085149));
#41053=CARTESIAN_POINT('Ctrl Pts',(3.2365718826948,-2.06534153551092,-17.9847374128284));
#41054=CARTESIAN_POINT('',(-3.2365718826939,-2.06534153551084,-17.9847374128283));
#41055=CARTESIAN_POINT('Ctrl Pts',(-2.61111949366609,-2.02928657753388,
-17.9437023142098));
#41056=CARTESIAN_POINT('Ctrl Pts',(-2.81875234052328,-2.0406223624171,-17.9574251794512));
#41057=CARTESIAN_POINT('Ctrl Pts',(-3.02717407631301,-2.05272254957051,
-17.9713114560054));
#41058=CARTESIAN_POINT('Ctrl Pts',(-3.23657188269391,-2.06534153551084,
-17.9847374128283));
#41059=CARTESIAN_POINT('',(-3.23593596335375,-2.06477283939947,-11.3703894654623));
#41060=CARTESIAN_POINT('Ctrl Pts',(-3.23593596401738,-2.06477283942456,
-11.3703894647525));
#41061=CARTESIAN_POINT('Ctrl Pts',(-3.23601450622251,-2.06484630497268,
-11.3736192543818));
#41062=CARTESIAN_POINT('Ctrl Pts',(-3.2360940577226,-2.06491840819467,-11.3767602403348));
#41063=CARTESIAN_POINT('Ctrl Pts',(-3.28422590292882,-2.11198472512398,
-13.4234076931397));
#41064=CARTESIAN_POINT('Ctrl Pts',(-3.23652783128775,-2.06535065050216,
-15.4352998782646));
#41065=CARTESIAN_POINT('Ctrl Pts',(-3.23657277689822,-2.06534385547269,
-17.6226933437992));
#41066=CARTESIAN_POINT('Ctrl Pts',(-3.23657012621139,-2.06534337873604,
-17.8038271587737));
#41067=CARTESIAN_POINT('Ctrl Pts',(-3.2365718826939,-2.06534153551084,-17.9847374128284));
#41068=CARTESIAN_POINT('Ctrl Pts',(-3.23593596401738,-2.06477283942457,
-11.3703894647526));
#41069=CARTESIAN_POINT('Ctrl Pts',(-3.18318064607444,-2.06164678027482,
-11.3736469970726));
#41070=CARTESIAN_POINT('Ctrl Pts',(-3.13048329082671,-2.05852104088958,
-11.3769782285977));
#41071=CARTESIAN_POINT('Ctrl Pts',(-3.07785477132643,-2.05544258807925,
-11.3802428845744));
#41072=CARTESIAN_POINT('',(-2.63912633614846,-2.0305825038593,-23.4602042419168));
#41073=CARTESIAN_POINT('',(1.94660615461814,-1.99343809749213,-24.3399007166515));
#41074=CARTESIAN_POINT('Ctrl Pts',(-2.63891815890426,-2.03090937194728,
-23.4605640099381));
#41075=CARTESIAN_POINT('Ctrl Pts',(-2.57069092949632,-2.02697783307983,
-23.5905899220032));
#41076=CARTESIAN_POINT('Ctrl Pts',(-2.49280814932383,-2.02253779605632,
-23.7152970983048));
#41077=CARTESIAN_POINT('Ctrl Pts',(-2.40655502964787,-2.01775533738805,
-23.8336815307012));
#41078=CARTESIAN_POINT('Ctrl Pts',(-2.32446314413585,-2.01320360579925,
-23.9463545714816));
#41079=CARTESIAN_POINT('Ctrl Pts',(-2.23479011295999,-2.00834158165483,
-24.0532985809489));
#41080=CARTESIAN_POINT('Ctrl Pts',(-2.13862719628931,-2.00335509341864,
-24.1536460659598));
#41081=CARTESIAN_POINT('Ctrl Pts',(-2.12093352671768,-2.00243759550751,
-24.1721096827427));
#41082=CARTESIAN_POINT('Ctrl Pts',(-2.10302007685531,-2.00151600931177,
-24.190349985842));
#41083=CARTESIAN_POINT('Ctrl Pts',(-2.08489354548269,-2.00059166263827,
-24.2083615856434));
#41084=CARTESIAN_POINT('Ctrl Pts',(-1.99543563554869,-1.99602983446685,
-24.2972522862234));
#41085=CARTESIAN_POINT('Ctrl Pts',(-1.90078990820332,-1.99139836734861,
-24.3805725948069));
#41086=CARTESIAN_POINT('Ctrl Pts',(-1.80174732651187,-1.98687547582441,
-24.4576762292758));
#41087=CARTESIAN_POINT('Ctrl Pts',(-1.69898972684165,-1.982182933802,-24.5376719671551));
#41088=CARTESIAN_POINT('Ctrl Pts',(-1.59150114951611,-1.97761033049424,
-24.6109757740146));
#41089=CARTESIAN_POINT('Ctrl Pts',(-1.48009773821805,-1.97331306608969,
-24.6768689330204));
#41090=CARTESIAN_POINT('Ctrl Pts',(-1.36905360466076,-1.96902966042993,
-24.7425495855596));
#41091=CARTESIAN_POINT('Ctrl Pts',(-1.25411981359012,-1.96502024562575,
-24.8008672655674));
#41092=CARTESIAN_POINT('Ctrl Pts',(-1.13605319549524,-1.96142991286828,
-24.8511135069562));
#41093=CARTESIAN_POINT('Ctrl Pts',(-1.11041960758882,-1.96065041133061,
-24.8620225298993));
#41094=CARTESIAN_POINT('Ctrl Pts',(-1.08463815715074,-1.95989061731232,
-24.8725511010247));
#41095=CARTESIAN_POINT('Ctrl Pts',(-1.05871627923612,-1.95915192999953,
-24.8826919936357));
#41096=CARTESIAN_POINT('Ctrl Pts',(-0.985241244461081,-1.95705813586262,
-24.9114361471148));
#41097=CARTESIAN_POINT('Ctrl Pts',(-0.910681653336464,-1.95513549044351,
-24.9370675670189));
#41098=CARTESIAN_POINT('Ctrl Pts',(-0.835278052412186,-1.95341456979757,
-24.9595801877773));
#41099=CARTESIAN_POINT('Ctrl Pts',(-0.712322279460726,-1.95060837585437,
-24.9962900617433));
#41100=CARTESIAN_POINT('Ctrl Pts',(-0.587123850541278,-1.94834073444966,
-25.0247068773822));
#41101=CARTESIAN_POINT('Ctrl Pts',(-0.460692338166107,-1.9467150574206,
-25.0448084797718));
#41102=CARTESIAN_POINT('Ctrl Pts',(-0.331909263579163,-1.94505914362068,
-25.0652839618033));
#41103=CARTESIAN_POINT('Ctrl Pts',(-0.201845369292106,-1.94406993971383,
-25.0771320454022));
#41104=CARTESIAN_POINT('Ctrl Pts',(-0.0715420642523354,-1.94381084899931,
-25.0803345004781));
#41105=CARTESIAN_POINT('Ctrl Pts',(-0.0480902413338543,-1.94376421818243,
-25.0809108742648));
#41106=CARTESIAN_POINT('Ctrl Pts',(-0.0246306324117139,-1.94374110538926,
-25.0812072091216));
#41107=CARTESIAN_POINT('Ctrl Pts',(-0.00116928290565843,-1.94374170274464,
-25.0812234161527));
#41108=CARTESIAN_POINT('Ctrl Pts',(0.128803537399696,-1.94374501201559,
-25.0813132009939));
#41109=CARTESIAN_POINT('Ctrl Pts',(0.258830619866978,-1.94448011545841,
-25.0728054144191));
#41110=CARTESIAN_POINT('Ctrl Pts',(0.387837616754974,-1.94589346353832,
-25.055688816754));
#41111=CARTESIAN_POINT('Ctrl Pts',(0.51707907690444,-1.94730938030216,-25.0385411105954));
#41112=CARTESIAN_POINT('Ctrl Pts',(0.645297809325559,-1.94940553453171,
-25.012753246554));
#41113=CARTESIAN_POINT('Ctrl Pts',(0.771393514954707,-1.95208063276428,
-24.9783191341716));
#41114=CARTESIAN_POINT('Ctrl Pts',(0.793305539292303,-1.95254549250938,
-24.9723354164486));
#41115=CARTESIAN_POINT('Ctrl Pts',(0.815153383398775,-1.95302772984231,
-24.9660906209875));
#41116=CARTESIAN_POINT('Ctrl Pts',(0.836931176722144,-1.95352668545461,
-24.9595847330815));
#41117=CARTESIAN_POINT('Ctrl Pts',(0.901500092336839,-1.95500603748753,
-24.9402954450915));
#41118=CARTESIAN_POINT('Ctrl Pts',(0.965453424995386,-1.95663253784695,
-24.9187109635716));
#41119=CARTESIAN_POINT('Ctrl Pts',(1.02863637449105,-1.9583872698216,-24.8948311706605));
#41120=CARTESIAN_POINT('Ctrl Pts',(1.15265648240947,-1.96183158590056,-24.847958169043));
#41121=CARTESIAN_POINT('Ctrl Pts',(1.27374678785909,-1.9657722892421,-24.7922297062563));
#41122=CARTESIAN_POINT('Ctrl Pts',(1.3908276584165,-1.97004779084986,-24.7285336236751));
#41123=CARTESIAN_POINT('Ctrl Pts',(1.50924541800924,-1.97437211231343,-24.6641102267684));
#41124=CARTESIAN_POINT('Ctrl Pts',(1.62356190778831,-1.9790382618604,-24.591536283455));
#41125=CARTESIAN_POINT('Ctrl Pts',(1.73261065266286,-1.98385876331907,-24.5117343231421));
#41126=CARTESIAN_POINT('Ctrl Pts',(1.75557148880081,-1.98487374743671,-24.4949315645562));
#41127=CARTESIAN_POINT('Ctrl Pts',(1.77829860862472,-1.98589552411659,-24.4778083726114));
#41128=CARTESIAN_POINT('Ctrl Pts',(1.80078084202138,-1.98692227374157,-24.4603733756465));
#41129=CARTESIAN_POINT('Ctrl Pts',(1.8506274960014,-1.98919873944575,-24.4217172401318));
#41130=CARTESIAN_POINT('Ctrl Pts',(1.89927055199605,-1.99149949877641,-24.3815283365078));
#41131=CARTESIAN_POINT('Ctrl Pts',(1.94658876137122,-1.99379905023128,-24.3399008862741));
#41132=CARTESIAN_POINT('',(2.6385842279831,-2.03021101218547,-23.4598822017706));
#41133=CARTESIAN_POINT('Ctrl Pts',(2.63870147030063,-2.03006717564156,-23.4598499951656));
#41134=CARTESIAN_POINT('Ctrl Pts',(3.02841473772455,-2.05254216577806,-22.7219672093624));
#41135=CARTESIAN_POINT('Ctrl Pts',(3.12535689549827,-2.05736702644637,-21.3572451381931));
#41136=CARTESIAN_POINT('Ctrl Pts',(2.24443363996642,-2.0075727180072,-19.8991125414343));
#41137=CARTESIAN_POINT('Ctrl Pts',(0.875888921590289,-1.93951562021359,
-18.8989839842624));
#41138=CARTESIAN_POINT('Ctrl Pts',(-0.876166156177594,-1.94068888543705,
-18.9034203539545));
#41139=CARTESIAN_POINT('Ctrl Pts',(-2.24514248919297,-2.008276670812,-19.8989668914236));
#41140=CARTESIAN_POINT('Ctrl Pts',(-2.79206912005562,-2.03859979060451,
-20.8121851494891));
#41141=CARTESIAN_POINT('Ctrl Pts',(-3.08399217684054,-2.05645735956288,
-22.0442240090313));
#41142=CARTESIAN_POINT('Ctrl Pts',(-2.93065240429659,-2.0466350002413,-22.9044061081406));
#41143=CARTESIAN_POINT('Ctrl Pts',(-2.63925053477479,-2.03038749422856,
-23.4599896041728));
#41144=CARTESIAN_POINT('Ctrl Pts',(1.94658876137122,-1.99379905023128,-24.3399008862741));
#41145=CARTESIAN_POINT('Ctrl Pts',(1.99464098969257,-1.99613427324596,-24.2976276944209));
#41146=CARTESIAN_POINT('Ctrl Pts',(2.04142781673245,-1.9984731378491,-24.2537468856496));
#41147=CARTESIAN_POINT('Ctrl Pts',(2.08685895123224,-2.00079368617497,-24.2083598616942));
#41148=CARTESIAN_POINT('Ctrl Pts',(2.18080318813562,-2.00559220472556,-24.1145068382608));
#41149=CARTESIAN_POINT('Ctrl Pts',(2.26895279483658,-2.01030987186438,-24.0142130776004));
#41150=CARTESIAN_POINT('Ctrl Pts',(2.35047939148303,-2.0147823881411,-23.9083777871828));
#41151=CARTESIAN_POINT('Ctrl Pts',(2.3694324676969,-2.01582214627338,-23.8837734935178));
#41152=CARTESIAN_POINT('Ctrl Pts',(2.38802744952198,-2.01684882264998,-23.8588697164727));
#41153=CARTESIAN_POINT('Ctrl Pts',(2.40625367999039,-2.01786065239614,-23.8336777755453));
#41154=CARTESIAN_POINT('Ctrl Pts',(2.4920251890086,-2.02262226036265,-23.7151260655696));
#41155=CARTESIAN_POINT('Ctrl Pts',(2.56963226957361,-2.02705128970956,-23.5901943757206));
#41156=CARTESIAN_POINT('Ctrl Pts',(2.63794735430056,-2.03099234874833,-23.4600571517336));
#41157=CARTESIAN_POINT('Ctrl Pts',(45.4957186312967,4.13505468146236,-12.2876753485083));
#41158=CARTESIAN_POINT('Ctrl Pts',(46.5747881377784,4.51315986439798,-12.6511164012708));
#41159=CARTESIAN_POINT('Ctrl Pts',(48.7315111185874,5.55100447935154,-13.1127068857499));
#41160=CARTESIAN_POINT('Ctrl Pts',(52.2255324170519,6.61037667463491,-13.0603457351622));
#41161=CARTESIAN_POINT('Ctrl Pts',(55.7352401406832,6.78357937642121,-12.1273823391115));
#41162=CARTESIAN_POINT('Ctrl Pts',(57.8454449537772,6.76763575867449,-10.9565650346632));
#41163=CARTESIAN_POINT('Ctrl Pts',(58.9417818399741,6.90315486069136,-10.1604688849966));
#41164=CARTESIAN_POINT('Ctrl Pts',(59.1869377879013,6.93283823797164,-9.9764403477307));
#41165=CARTESIAN_POINT('Ctrl Pts',(59.6656000071998,6.98501272405032,-9.59287808094242));
#41166=CARTESIAN_POINT('Ctrl Pts',(60.4698386743377,7.03851518962114,-8.88527771072978));
#41167=CARTESIAN_POINT('Ctrl Pts',(61.935425590422,6.93159705832345,-7.32309238219473));
#41168=CARTESIAN_POINT('Ctrl Pts',(62.898870223949,6.33243798646893,-5.81981710521227));
#41169=CARTESIAN_POINT('Ctrl Pts',(63.6271064539284,6.1172012971021,-4.30394126827215));
#41170=CARTESIAN_POINT('Ctrl Pts',(63.9964631920437,6.08157109535702,-3.43096909542246));
#41171=CARTESIAN_POINT('Ctrl Pts',(64.4196909334568,6.16095583450854,-2.0750183342162));
#41172=CARTESIAN_POINT('Ctrl Pts',(64.7075353735302,6.25611577526355,-0.705188274299797));
#41173=CARTESIAN_POINT('Ctrl Pts',(64.8131179042321,6.27855936375402,0.234551382385882));
#41174=CARTESIAN_POINT('Ctrl Pts',(64.8578334301675,6.26126913644566,0.94307726867782));
#41175=CARTESIAN_POINT('Ctrl Pts',(64.8763131687878,6.25212971761612,1.41873044327074));
#41176=CARTESIAN_POINT('Ctrl Pts',(64.8669425474595,6.24148249015893,2.37159989960793));
#41177=CARTESIAN_POINT('Ctrl Pts',(64.7293383040315,6.23744524570034,4.02825143678288));
#41178=CARTESIAN_POINT('Ctrl Pts',(64.4090264396697,6.21556997011337,5.41180556034465));
#41179=CARTESIAN_POINT('Ctrl Pts',(63.392616944205,6.06901676370829,8.4362633730038));
#41180=CARTESIAN_POINT('Ctrl Pts',(62.2029128798603,5.85755777132363,10.3600282958658));
#41181=CARTESIAN_POINT('Ctrl Pts',(57.9137758164067,5.23547967962912,14.7285512014021));
#41182=CARTESIAN_POINT('Ctrl Pts',(50.2340493278717,3.97178337193033,17.9121952059345));
#41183=CARTESIAN_POINT('Ctrl Pts',(42.4627846177445,3.39626629188669,14.7465965189029));
#41184=CARTESIAN_POINT('Ctrl Pts',(38.1616839203783,3.18800029201627,10.3559731559896));
#41185=CARTESIAN_POINT('Ctrl Pts',(36.9711393616719,3.15313406811575,8.42495263430108));
#41186=CARTESIAN_POINT('Ctrl Pts',(35.6532723602024,3.11897952995874,4.50504080276018));
#41187=CARTESIAN_POINT('Ctrl Pts',(35.4035953598297,3.11401329970943,2.5854570740989));
#41188=CARTESIAN_POINT('Ctrl Pts',(35.6531385708734,3.12046556629585,-1.27776505111417));
#41189=CARTESIAN_POINT('Ctrl Pts',(36.175035699066,3.13335329444264,-3.19875344300605));
#41190=CARTESIAN_POINT('Ctrl Pts',(37.619750560802,3.17534463244499,-6.07811908458911));
#41191=CARTESIAN_POINT('Ctrl Pts',(39.0211463611516,3.22647042745986,-8.16085205297379));
#41192=CARTESIAN_POINT('Ctrl Pts',(40.9332506662835,3.2798490343456,-9.84541367809451));
#41193=CARTESIAN_POINT('Ctrl Pts',(42.2378053070641,3.41504440953276,-10.725652165237));
#41194=CARTESIAN_POINT('Ctrl Pts',(42.8038448826665,3.4807437957151,-11.0806258189848));
#41195=CARTESIAN_POINT('Ctrl Pts',(43.981345015687,3.67284868940879,-11.7113672365034));
#41196=CARTESIAN_POINT('Ctrl Pts',(44.8918845743013,3.92347165996875,-12.0842981943491));
#41197=CARTESIAN_POINT('Ctrl Pts',(45.4957186312967,4.13505468146236,-12.2876753485083));
#41198=CARTESIAN_POINT('Ctrl Pts',(45.4226909351084,4.3829089607378,-12.2630789136873));
#41199=CARTESIAN_POINT('Ctrl Pts',(46.4885376077135,4.73594338198905,-12.6289760053212));
#41200=CARTESIAN_POINT('Ctrl Pts',(48.6563981762571,5.73344573284324,-13.1089448312689));
#41201=CARTESIAN_POINT('Ctrl Pts',(52.2019430219846,6.78342595894654,-13.0678581912781));
#41202=CARTESIAN_POINT('Ctrl Pts',(55.7389585640039,6.9553202878816,-12.1264740028574));
#41203=CARTESIAN_POINT('Ctrl Pts',(57.8403370940749,6.95575633967418,-10.9585779856605));
#41204=CARTESIAN_POINT('Ctrl Pts',(58.9264187763328,7.10412715681792,-10.1717777373723));
#41205=CARTESIAN_POINT('Ctrl Pts',(59.1736262174514,7.13246285828779,-9.98671186741939));
#41206=CARTESIAN_POINT('Ctrl Pts',(59.6556436943423,7.18385453217346,-9.60140532586356));
#41207=CARTESIAN_POINT('Ctrl Pts',(60.4705001186037,7.23456742927621,-8.88509390469854));
#41208=CARTESIAN_POINT('Ctrl Pts',(61.9608263373809,7.1262553463295,-7.29673934126728));
#41209=CARTESIAN_POINT('Ctrl Pts',(62.9304716293567,6.54211572529945,-5.76158733043494));
#41210=CARTESIAN_POINT('Ctrl Pts',(63.6321908187021,6.36074410415715,-4.29220747239235));
#41211=CARTESIAN_POINT('Ctrl Pts',(63.9940798094662,6.33427373390901,-3.43607273910697));
#41212=CARTESIAN_POINT('Ctrl Pts',(64.4146420733654,6.42472104796742,-2.09374987503663));
#41213=CARTESIAN_POINT('Ctrl Pts',(64.7054278241187,6.52953208474263,-0.71990867105941));
#41214=CARTESIAN_POINT('Ctrl Pts',(64.8128653718556,6.55685484276445,0.231003469905035));
#41215=CARTESIAN_POINT('Ctrl Pts',(64.8580472393094,6.5414965438589,0.95160233440216));
#41216=CARTESIAN_POINT('Ctrl Pts',(64.876095206118,6.5340459390533,1.42254718097353));
#41217=CARTESIAN_POINT('Ctrl Pts',(64.8666543146928,6.5242433141999,2.37413725116621));
#41218=CARTESIAN_POINT('Ctrl Pts',(64.7292489158462,6.51789648322309,4.02837788027091));
#41219=CARTESIAN_POINT('Ctrl Pts',(64.4075066260974,6.49250579105984,5.41929417877616));
#41220=CARTESIAN_POINT('Ctrl Pts',(63.3835505344909,6.34444534627468,8.45633506936137));
#41221=CARTESIAN_POINT('Ctrl Pts',(62.1894742836605,6.13520939625073,10.3796948486764));
#41222=CARTESIAN_POINT('Ctrl Pts',(57.8817168152093,5.51782830014487,14.7492052945439));
#41223=CARTESIAN_POINT('Ctrl Pts',(50.1889367119781,4.27174239122586,17.9080324411693));
#41224=CARTESIAN_POINT('Ctrl Pts',(42.4513123201647,3.7027604475385,14.7350414399812));
#41225=CARTESIAN_POINT('Ctrl Pts',(38.1580401199668,3.49283715598917,10.3507391715678));
#41226=CARTESIAN_POINT('Ctrl Pts',(36.9697716264182,3.45725996326839,8.42121430282625));
#41227=CARTESIAN_POINT('Ctrl Pts',(35.6532386126616,3.42202646347052,4.50394140790714));
#41228=CARTESIAN_POINT('Ctrl Pts',(35.4037695650286,3.41684585962461,2.58491200481547));
#41229=CARTESIAN_POINT('Ctrl Pts',(35.6530418433231,3.42350542454771,-1.27617009765779));
#41230=CARTESIAN_POINT('Ctrl Pts',(36.1745351298173,3.4366362204548,-3.19650288315925));
#41231=CARTESIAN_POINT('Ctrl Pts',(37.6174484445499,3.47973090050457,-6.07366716564505));
#41232=CARTESIAN_POINT('Ctrl Pts',(39.0177744495317,3.53068548887777,-8.15722126293493));
#41233=CARTESIAN_POINT('Ctrl Pts',(40.9267557148107,3.58453856247977,-9.83812324731517));
#41234=CARTESIAN_POINT('Ctrl Pts',(42.2154596021336,3.71009055098709,-10.7107480567621));
#41235=CARTESIAN_POINT('Ctrl Pts',(42.7766214516271,3.77492500412091,-11.0639711667881));
#41236=CARTESIAN_POINT('Ctrl Pts',(43.9336311230074,3.9542166984862,-11.687940244315));
#41237=CARTESIAN_POINT('Ctrl Pts',(44.8262562137227,4.1853552298959,-12.0583273903082));
#41238=CARTESIAN_POINT('Ctrl Pts',(45.4226909351084,4.3829089607378,-12.2630789136873));
#41239=CARTESIAN_POINT('Ctrl Pts',(45.2362559210283,4.81395978114001,-12.3967533670572));
#41240=CARTESIAN_POINT('Ctrl Pts',(46.3031207984177,5.12499660732279,-12.7410768028134));
#41241=CARTESIAN_POINT('Ctrl Pts',(48.51867911769,6.05214572917268,-13.2054239348972));
#41242=CARTESIAN_POINT('Ctrl Pts',(52.1723223958436,7.08619467178563,-13.1602949061944));
#41243=CARTESIAN_POINT('Ctrl Pts',(55.774901305395,7.25546503413852,-12.199711943089));
#41244=CARTESIAN_POINT('Ctrl Pts',(57.8793869234972,7.28458661649953,-11.04383767945));
#41245=CARTESIAN_POINT('Ctrl Pts',(58.9653776144854,7.45501929857546,-10.2803849930773));
#41246=CARTESIAN_POINT('Ctrl Pts',(59.2169323719478,7.4810504105106,-10.0906577031871));
#41247=CARTESIAN_POINT('Ctrl Pts',(59.7076295156488,7.53110130805176,-9.69852527008054));
#41248=CARTESIAN_POINT('Ctrl Pts',(60.5438525648364,7.5771049587259,-8.95863731260499));
#41249=CARTESIAN_POINT('Ctrl Pts',(62.0884747892352,7.46627421307784,-7.31479565231356));
#41250=CARTESIAN_POINT('Ctrl Pts',(63.0932644635168,6.90857606179419,-5.72668888160001));
#41251=CARTESIAN_POINT('Ctrl Pts',(63.7895723587306,6.78515334133648,-4.33844754181989));
#41252=CARTESIAN_POINT('Ctrl Pts',(64.1548219109931,6.77419647605495,-3.50652508171551));
#41253=CARTESIAN_POINT('Ctrl Pts',(64.5933355322215,6.88323321345314,-2.17605782839782));
#41254=CARTESIAN_POINT('Ctrl Pts',(64.9078972715697,7.00416841028133,-0.779117188900245));
#41255=CARTESIAN_POINT('Ctrl Pts',(65.0272679117268,7.03970770065191,0.203945258498023));
#41256=CARTESIAN_POINT('Ctrl Pts',(65.0775628156496,7.02755258341766,0.955800165700155));
#41257=CARTESIAN_POINT('Ctrl Pts',(65.097818958486,7.02290128163086,1.4257561538819));
#41258=CARTESIAN_POINT('Ctrl Pts',(65.0895377707789,7.01451194446682,2.38992058125223));
#41259=CARTESIAN_POINT('Ctrl Pts',(64.9461830318912,7.00445388751589,4.06526506532641));
#41260=CARTESIAN_POINT('Ctrl Pts',(64.6115433183857,6.97329492674332,5.48770512704195));
#41261=CARTESIAN_POINT('Ctrl Pts',(63.5587315973221,6.82268765355066,8.58954807570769));
#41262=CARTESIAN_POINT('Ctrl Pts',(62.3429488193778,6.61708776059798,10.5421828944442));
#41263=CARTESIAN_POINT('Ctrl Pts',(57.9482932775536,6.0075841917312,14.9849327447503));
#41264=CARTESIAN_POINT('Ctrl Pts',(50.120992280796,4.7907537093198,18.1842129862357));
#41265=CARTESIAN_POINT('Ctrl Pts',(42.2914692710772,4.23252014330705,14.9529853278185));
#41266=CARTESIAN_POINT('Ctrl Pts',(37.937704741533,4.02000608144395,10.4970477594956));
#41267=CARTESIAN_POINT('Ctrl Pts',(36.7331397611778,3.98325676303847,8.53535003460254));
#41268=CARTESIAN_POINT('Ctrl Pts',(35.3975369817611,3.94626884381358,4.55234212195737));
#41269=CARTESIAN_POINT('Ctrl Pts',(35.1444459825535,3.94073405856047,2.60094188977881));
#41270=CARTESIAN_POINT('Ctrl Pts',(35.3972682786971,3.947715411657,-1.3248018941845));
#41271=CARTESIAN_POINT('Ctrl Pts',(35.926694176603,3.96126168526223,-3.2774721598599));
#41272=CARTESIAN_POINT('Ctrl Pts',(37.3901262851908,4.00601018812854,-6.20291896929763));
#41273=CARTESIAN_POINT('Ctrl Pts',(38.8134827657176,4.05684134261308,-8.32453245845042));
#41274=CARTESIAN_POINT('Ctrl Pts',(40.7511286928979,4.11081645998679,-10.0306407741865));
#41275=CARTESIAN_POINT('Ctrl Pts',(42.0428239458654,4.22042746992371,-10.8926234608938));
#41276=CARTESIAN_POINT('Ctrl Pts',(42.6054806472463,4.28363615455033,-11.2484717789448));
#41277=CARTESIAN_POINT('Ctrl Pts',(43.7559350871281,4.44202305995758,-11.8552481254079));
#41278=CARTESIAN_POINT('Ctrl Pts',(44.6392514247374,4.63990738924053,-12.2040741968255));
#41279=CARTESIAN_POINT('Ctrl Pts',(45.2362559210283,4.81395978114001,-12.3967533670572));
#41280=CARTESIAN_POINT('Ctrl Pts',(45.0393082808176,5.03095193627101,-12.7701404172511));
#41281=CARTESIAN_POINT('Ctrl Pts',(46.1334687087117,5.35176317337511,-13.0718012479004));
#41282=CARTESIAN_POINT('Ctrl Pts',(48.4047643981397,6.28128470705804,-13.4535437106496));
#41283=CARTESIAN_POINT('Ctrl Pts',(52.1693689098252,7.31892628045186,-13.3716165012657));
#41284=CARTESIAN_POINT('Ctrl Pts',(55.8543152135557,7.48812989610121,-12.3862535247233));
#41285=CARTESIAN_POINT('Ctrl Pts',(57.9923320772498,7.52622499658178,-11.2496579661572));
#41286=CARTESIAN_POINT('Ctrl Pts',(59.1068119148139,7.6978190428995,-10.5096866568958));
#41287=CARTESIAN_POINT('Ctrl Pts',(59.3629402571142,7.72383493669142,-10.3124417661215));
#41288=CARTESIAN_POINT('Ctrl Pts',(59.8647407600303,7.77395345886841,-9.90933860675373));
#41289=CARTESIAN_POINT('Ctrl Pts',(60.7218337050463,7.82050499147147,-9.14015892556009));
#41290=CARTESIAN_POINT('Ctrl Pts',(62.3247704239217,7.7061385428919,-7.43738447894348));
#41291=CARTESIAN_POINT('Ctrl Pts',(63.3886024430437,7.14841447789296,-5.82205137164671));
#41292=CARTESIAN_POINT('Ctrl Pts',(64.1366259862645,7.02254302921227,-4.47918514639915));
#41293=CARTESIAN_POINT('Ctrl Pts',(64.5266343691297,7.00658243194664,-3.64991069569223));
#41294=CARTESIAN_POINT('Ctrl Pts',(65.0054037197404,7.10634554942755,-2.30157654706013));
#41295=CARTESIAN_POINT('Ctrl Pts',(65.3561087229281,7.21883370016228,-0.863559409343484));
#41296=CARTESIAN_POINT('Ctrl Pts',(65.4922044619082,7.24991771370432,0.156636010686802));
#41297=CARTESIAN_POINT('Ctrl Pts',(65.5502525107814,7.23511124126408,0.939802923614275));
#41298=CARTESIAN_POINT('Ctrl Pts',(65.5750930683425,7.22873886389136,1.42145069534216));
#41299=CARTESIAN_POINT('Ctrl Pts',(65.5687887080707,7.21933156229316,2.41592252691496));
#41300=CARTESIAN_POINT('Ctrl Pts',(65.414725807752,7.21198235972297,4.14322185797141));
#41301=CARTESIAN_POINT('Ctrl Pts',(65.0596681727028,7.18443986743527,5.61298191689179));
#41302=CARTESIAN_POINT('Ctrl Pts',(63.9672133193117,7.03419770034737,8.81868578869884));
#41303=CARTESIAN_POINT('Ctrl Pts',(62.7161166820525,6.82577914982853,10.8349003538464));
#41304=CARTESIAN_POINT('Ctrl Pts',(58.1850006970887,6.20879216622989,15.4282146019174));
#41305=CARTESIAN_POINT('Ctrl Pts',(50.1104914220837,4.9684119737969,18.7709296527553));
#41306=CARTESIAN_POINT('Ctrl Pts',(41.9978933461976,4.40390858006523,15.4335469013269));
#41307=CARTESIAN_POINT('Ctrl Pts',(37.493584849084,4.19415487226654,10.8143287573227));
#41308=CARTESIAN_POINT('Ctrl Pts',(36.2484614816851,4.15867987120878,8.78180343114533));
#41309=CARTESIAN_POINT('Ctrl Pts',(34.8683368651209,4.12336748697614,4.65611205748337));
#41310=CARTESIAN_POINT('Ctrl Pts',(34.6069082029005,4.11816980101638,2.63537705212125));
#41311=CARTESIAN_POINT('Ctrl Pts',(34.8681508421745,4.12485500101605,-1.42986135097754));
#41312=CARTESIAN_POINT('Ctrl Pts',(35.4155051923742,4.13797466334024,-3.45205726244952));
#41313=CARTESIAN_POINT('Ctrl Pts',(36.9285012394375,4.18123249165731,-6.48311952745601));
#41314=CARTESIAN_POINT('Ctrl Pts',(38.4015645590874,4.23156809046291,-8.68099638738615));
#41315=CARTESIAN_POINT('Ctrl Pts',(40.4097975334022,4.28659532550123,-10.4483512133793));
#41316=CARTESIAN_POINT('Ctrl Pts',(41.7493555547286,4.40717619984816,-11.317445711143));
#41317=CARTESIAN_POINT('Ctrl Pts',(42.3294549111165,4.47074736329829,-11.6836732045952));
#41318=CARTESIAN_POINT('Ctrl Pts',(43.5186765626443,4.64093291483995,-12.282897501734));
#41319=CARTESIAN_POINT('Ctrl Pts',(44.4270295293464,4.85142990393974,-12.6013347174204));
#41320=CARTESIAN_POINT('Ctrl Pts',(45.0393082808176,5.03095193627101,-12.7701404172511));
#41321=CARTESIAN_POINT('Ctrl Pts',(44.9671960021647,5.06936132425713,-12.9468323394379));
#41322=CARTESIAN_POINT('Ctrl Pts',(46.0737017506393,5.40581314007301,-13.2335334133338));
#41323=CARTESIAN_POINT('Ctrl Pts',(48.3643075999864,6.35380835363947,-13.5778554041427));
#41324=CARTESIAN_POINT('Ctrl Pts',(52.1729677903268,7.39852199644268,-13.4768906188369));
#41325=CARTESIAN_POINT('Ctrl Pts',(55.8938002527975,7.56810054532598,-12.4809580618348));
#41326=CARTESIAN_POINT('Ctrl Pts',(58.0500408302575,7.60482227579029,-11.352167081635));
#41327=CARTESIAN_POINT('Ctrl Pts',(59.1799059046439,7.77152332437818,-10.6198965981888));
#41328=CARTESIAN_POINT('Ctrl Pts',(59.4379281617953,7.7981238809332,-10.4193877736077));
#41329=CARTESIAN_POINT('Ctrl Pts',(59.9445192777259,7.84863591825408,-10.0113807547288));
#41330=CARTESIAN_POINT('Ctrl Pts',(60.809824883128,7.8967925806761,-9.23021697908096));
#41331=CARTESIAN_POINT('Ctrl Pts',(62.4360688307817,7.7807213081155,-7.50363616006776));
#41332=CARTESIAN_POINT('Ctrl Pts',(63.5247667463043,7.21631726880368,-5.882214856638));
#41333=CARTESIAN_POINT('Ctrl Pts',(64.2978125074662,7.07524290401267,-4.54781307837155));
#41334=CARTESIAN_POINT('Ctrl Pts',(64.6990534903062,7.0525690841578,-3.71481086803514));
#41335=CARTESIAN_POINT('Ctrl Pts',(65.1937668335651,7.14243217860219,-2.35375057630837));
#41336=CARTESIAN_POINT('Ctrl Pts',(65.5570967288631,7.2462698730418,-0.89745620523494));
#41337=CARTESIAN_POINT('Ctrl Pts',(65.6986423579354,7.27296271621864,0.136607376960506));
#41338=CARTESIAN_POINT('Ctrl Pts',(65.7592354870047,7.25589970503656,0.930580036746943));
#41339=CARTESIAN_POINT('Ctrl Pts',(65.7856454558346,7.24790516504022,1.41859891137044));
#41340=CARTESIAN_POINT('Ctrl Pts',(65.7799206851199,7.23760363176885,2.42672092669585));
#41341=CARTESIAN_POINT('Ctrl Pts',(65.6219675454031,7.23269723783848,4.17753766607333));
#41342=CARTESIAN_POINT('Ctrl Pts',(65.2593810692705,7.20859173918288,5.66675087052868));
#41343=CARTESIAN_POINT('Ctrl Pts',(64.1513986946448,7.05911518128976,8.91567711964445));
#41344=CARTESIAN_POINT('Ctrl Pts',(62.8850361125523,6.84822040784708,10.9598101495106));
#41345=CARTESIAN_POINT('Ctrl Pts',(58.2964793934186,6.2251056267945,15.6180768610311));
#41346=CARTESIAN_POINT('Ctrl Pts',(50.1158709003265,4.96503903391737,19.021940331474));
#41347=CARTESIAN_POINT('Ctrl Pts',(41.8772269224742,4.39494460937913,15.639166517446));
#41348=CARTESIAN_POINT('Ctrl Pts',(37.3065111143528,4.18729150714763,10.9500795882153));
#41349=CARTESIAN_POINT('Ctrl Pts',(36.0433455999976,4.1527741837325,8.88726750897097));
#41350=CARTESIAN_POINT('Ctrl Pts',(34.643523589437,4.11877042040954,4.70052993027424));
#41351=CARTESIAN_POINT('Ctrl Pts',(34.3784008811423,4.11383558693573,2.65012644089586));
#41352=CARTESIAN_POINT('Ctrl Pts',(34.6433770295448,4.12027840323245,-1.47489204003542));
#41353=CARTESIAN_POINT('Ctrl Pts',(35.1985818678004,4.13308125156768,-3.52683212118584));
#41354=CARTESIAN_POINT('Ctrl Pts',(36.7334877998714,4.17508278517857,-6.60303135134555));
#41355=CARTESIAN_POINT('Ctrl Pts',(38.2279573123907,4.22527365145291,-8.83301677026279));
#41356=CARTESIAN_POINT('Ctrl Pts',(40.2667716354802,4.28049099639363,-10.6271201515531));
#41357=CARTESIAN_POINT('Ctrl Pts',(41.6289539539425,4.41064411427425,-11.5039959467974));
#41358=CARTESIAN_POINT('Ctrl Pts',(42.2177215221571,4.474688119656,-11.8752322978503));
#41359=CARTESIAN_POINT('Ctrl Pts',(43.4267198452443,4.65618460624521,-12.4764006835622));
#41360=CARTESIAN_POINT('Ctrl Pts',(44.3480089607584,4.88108701596907,-12.786397935949));
#41361=CARTESIAN_POINT('Ctrl Pts',(44.9671960021647,5.06936132425713,-12.9468323394379));
#41362=CARTESIAN_POINT('',(44.9671960021647,5.06936132425713,-12.9468323394379));
#41363=CARTESIAN_POINT('Ctrl Pts',(44.9671960021647,5.06936132425713,-12.9468323394379));
#41364=CARTESIAN_POINT('Ctrl Pts',(45.0393082808176,5.03095193627101,-12.7701404172511));
#41365=CARTESIAN_POINT('Ctrl Pts',(45.2362559210283,4.81395978114001,-12.3967533670572));
#41366=CARTESIAN_POINT('Ctrl Pts',(45.4226909351084,4.3829089607378,-12.2630789136873));
#41367=CARTESIAN_POINT('Ctrl Pts',(45.4957186312967,4.13505468146236,-12.2876753485083));
#41368=CARTESIAN_POINT('',(41.3411273923048,4.38314300528299,-11.3187137406582));
#41369=CARTESIAN_POINT('Ctrl Pts',(44.9671960021647,5.06936132425713,-12.9468323394379));
#41370=CARTESIAN_POINT('Ctrl Pts',(44.3480089607584,4.88108701596907,-12.786397935949));
#41371=CARTESIAN_POINT('Ctrl Pts',(43.4267198452443,4.65618460624521,-12.4764006835622));
#41372=CARTESIAN_POINT('Ctrl Pts',(42.2177215221571,4.474688119656,-11.8752322978503));
#41373=CARTESIAN_POINT('Ctrl Pts',(41.6289539539425,4.41064411427425,-11.5039959467974));
#41374=CARTESIAN_POINT('Ctrl Pts',(41.3411273923048,4.38314300528299,-11.3187137406582));
#41375=CARTESIAN_POINT('',(36.135527542684,4.15872006235187,-5.40462207903584));
#41376=CARTESIAN_POINT('Ctrl Pts',(41.3386675640102,4.38290809676367,-11.3171298578528));
#41377=CARTESIAN_POINT('Ctrl Pts',(40.2652156414254,4.28044885388744,-10.6257507841702));
#41378=CARTESIAN_POINT('Ctrl Pts',(38.2281132730671,4.22527416890354,-8.83280500219181));
#41379=CARTESIAN_POINT('Ctrl Pts',(36.7345527005594,4.17511854755004,-6.60462019357029));
#41380=CARTESIAN_POINT('Ctrl Pts',(36.1359227536501,4.15873087918382,-5.4054139657304));
#41381=CARTESIAN_POINT('',(34.5091948905088,4.11701580411013,0.61399232466525));
#41382=CARTESIAN_POINT('Ctrl Pts',(36.1346424692247,4.15869583809775,-5.40284865178772));
#41383=CARTESIAN_POINT('Ctrl Pts',(35.1990480848672,4.13309400924318,-3.52776649543769));
#41384=CARTESIAN_POINT('Ctrl Pts',(34.6439301778968,4.1202911596584,-1.47693598688928));
#41385=CARTESIAN_POINT('Ctrl Pts',(34.5092829751989,4.11701794563615,0.612623215338439));
#41386=CARTESIAN_POINT('',(35.2891842733433,4.13445448140289,6.63164062429908));
#41387=CARTESIAN_POINT('Ctrl Pts',(34.509081999843,4.11701305949813,0.615746995805597));
#41388=CARTESIAN_POINT('Ctrl Pts',(34.3784661277573,4.11383717338778,2.64911071365206));
#41389=CARTESIAN_POINT('Ctrl Pts',(34.6432589465792,4.11876549469344,4.69848247877565));
#41390=CARTESIAN_POINT('Ctrl Pts',(35.2886534294729,4.13444158703147,6.63005240363038));
#41391=CARTESIAN_POINT('',(38.9650172416945,4.26263943020926,12.6515372403238));
#41392=CARTESIAN_POINT('Ctrl Pts',(35.2896208971195,4.13446508713737,6.63294694983923));
#41393=CARTESIAN_POINT('Ctrl Pts',(36.0433455999976,4.1527741837325,8.88726750897097));
#41394=CARTESIAN_POINT('Ctrl Pts',(37.3065111143528,4.18729150714763,10.9500795882153));
#41395=CARTESIAN_POINT('Ctrl Pts',(38.9648272977679,4.26263080069001,12.6513423808761));
#41396=CARTESIAN_POINT('',(61.2178517606911,6.62182084999648,12.6523225981111));
#41397=CARTESIAN_POINT('Ctrl Pts',(38.9650172416945,4.26263943020926,12.6515372403238));
#41398=CARTESIAN_POINT('Ctrl Pts',(41.8774060263554,4.39495700302059,15.6392400564092));
#41399=CARTESIAN_POINT('Ctrl Pts',(50.1159598214397,4.9650527305176,19.0219033323523));
#41400=CARTESIAN_POINT('Ctrl Pts',(58.2964793934186,6.2251056267945,15.6180768610311));
#41401=CARTESIAN_POINT('Ctrl Pts',(61.2178517606911,6.62182084999648,12.6523225981111));
#41402=CARTESIAN_POINT('',(64.9287215031429,7.16301726873607,6.63668503037258));
#41403=CARTESIAN_POINT('Ctrl Pts',(61.2181484097314,6.62066005626491,12.6521825294247));
#41404=CARTESIAN_POINT('Ctrl Pts',(61.2184817862553,6.62070599214976,12.6518439895148));
#41405=CARTESIAN_POINT('Ctrl Pts',(61.2188151436046,6.62075192600279,12.6515054358842));
#41406=CARTESIAN_POINT('Ctrl Pts',(61.2191484817782,6.62079785782461,12.6511668685336));
#41407=CARTESIAN_POINT('Ctrl Pts',(61.3585198686239,6.64000232408162,12.5096091205001));
#41408=CARTESIAN_POINT('Ctrl Pts',(61.4948662035403,6.65890301905649,12.3657092611848));
#41409=CARTESIAN_POINT('Ctrl Pts',(61.6281869302241,6.67754009064395,12.2194998303496));
#41410=CARTESIAN_POINT('Ctrl Pts',(61.7230124842131,6.69079587376165,12.1155070707672));
#41411=CARTESIAN_POINT('Ctrl Pts',(61.8163080541546,6.70391793770475,12.0103450216132));
#41412=CARTESIAN_POINT('Ctrl Pts',(61.9080811679174,6.71691444214465,11.9040128177346));
#41413=CARTESIAN_POINT('Ctrl Pts',(61.9456900876825,6.72224045182945,11.8604375356053));
#41414=CARTESIAN_POINT('Ctrl Pts',(61.9830433964093,6.72754531096285,11.8166655938875));
#41415=CARTESIAN_POINT('Ctrl Pts',(62.0201418786322,6.73282929205629,11.7726977909551));
#41416=CARTESIAN_POINT('Ctrl Pts',(62.1561084355408,6.75219517100867,11.6115550589251));
#41417=CARTESIAN_POINT('Ctrl Pts',(62.2886541368923,6.7712840398024,11.4477805493039));
#41418=CARTESIAN_POINT('Ctrl Pts',(62.4178458249931,6.79009941384757,11.2814180648038));
#41419=CARTESIAN_POINT('Ctrl Pts',(62.4499480296618,6.79477475323972,11.2400794724755));
#41420=CARTESIAN_POINT('Ctrl Pts',(62.4818430174384,6.79943299647369,11.1985811492951));
#41421=CARTESIAN_POINT('Ctrl Pts',(62.5135315437829,6.80407378816793,11.1569239057277));
#41422=CARTESIAN_POINT('Ctrl Pts',(62.6418377521643,6.82286426077312,10.9882545610051));
#41423=CARTESIAN_POINT('Ctrl Pts',(62.7667618614452,6.84137151992753,10.8169790114194));
#41424=CARTESIAN_POINT('Ctrl Pts',(62.888333557696,6.85954888471648,10.6431486339496));
#41425=CARTESIAN_POINT('Ctrl Pts',(63.0088431539118,6.87756744461603,10.4708369097163));
#41426=CARTESIAN_POINT('Ctrl Pts',(63.1260591461416,6.89526116929565,10.2960145222447));
#41427=CARTESIAN_POINT('Ctrl Pts',(63.2399722491003,6.91255371978634,10.1187451005626));
#41428=CARTESIAN_POINT('Ctrl Pts',(63.3333417291813,6.92672765067446,9.97344527721647));
#41429=CARTESIAN_POINT('Ctrl Pts',(63.4244916019108,6.94063128924984,9.82650167738523));
#41430=CARTESIAN_POINT('Ctrl Pts',(63.5133942469259,6.95421218942382,9.67795776882544));
#41431=CARTESIAN_POINT('Ctrl Pts',(63.5173580953864,6.95481771280547,9.67133473142122));
#41432=CARTESIAN_POINT('Ctrl Pts',(63.5213174728839,6.95542259352705,9.66470851402652));
#41433=CARTESIAN_POINT('Ctrl Pts',(63.5252723753743,6.95602682667384,9.65807912151982));
#41434=CARTESIAN_POINT('Ctrl Pts',(63.6435744367229,6.9741011096611,9.45977567385646));
#41435=CARTESIAN_POINT('Ctrl Pts',(63.7578761830907,6.9915949103269,9.25862943060299));
#41436=CARTESIAN_POINT('Ctrl Pts',(63.8680452798276,7.00838069986764,9.05478280687235));
#41437=CARTESIAN_POINT('Ctrl Pts',(63.9757163373921,7.02478587850157,8.85555832189317));
#41438=CARTESIAN_POINT('Ctrl Pts',(64.0794401717447,7.04051441179248,8.65375513836877));
#41439=CARTESIAN_POINT('Ctrl Pts',(64.1790492592415,7.05546338414968,8.44952127121358));
#41440=CARTESIAN_POINT('Ctrl Pts',(64.2136493607692,7.06065604251341,8.3785788229234));
#41441=CARTESIAN_POINT('Ctrl Pts',(64.2477525747637,7.06575480881764,8.3073431861715));
#41442=CARTESIAN_POINT('Ctrl Pts',(64.2813505141886,7.07075593400366,8.23582079704894));
#41443=CARTESIAN_POINT('Ctrl Pts',(64.2946901741793,7.07274157094135,8.20742368791221));
#41444=CARTESIAN_POINT('Ctrl Pts',(64.3079501755489,7.07471181916513,8.17898137608073));
#41445=CARTESIAN_POINT('Ctrl Pts',(64.3211299659384,7.07666644901065,8.15049424887497));
#41446=CARTESIAN_POINT('Ctrl Pts',(64.4110197913255,7.08999756660192,7.95620414147232));
#41447=CARTESIAN_POINT('Ctrl Pts',(64.4971824252759,7.1026000785673,7.75982946344119));
#41448=CARTESIAN_POINT('Ctrl Pts',(64.5794112867232,7.11441613487273,7.56149561010692));
#41449=CARTESIAN_POINT('Ctrl Pts',(64.6655794624388,7.12679825956799,7.35366023425911));
#41450=CARTESIAN_POINT('Ctrl Pts',(64.7474272412586,7.13831620850769,7.14367380505442));
#41451=CARTESIAN_POINT('Ctrl Pts',(64.8246711519124,7.14893800982192,6.93167689573328));
#41452=CARTESIAN_POINT('Ctrl Pts',(64.8603292248536,7.15384134735136,6.8338128545176));
#41453=CARTESIAN_POINT('Ctrl Pts',(64.8950056468963,7.15855423653779,6.73552029375412));
#41454=CARTESIAN_POINT('Ctrl Pts',(64.9286699552961,7.16307609763269,6.63681248550691));
#41455=CARTESIAN_POINT('',(65.7391367015185,7.26119855263812,0.666704654999593));
#41456=CARTESIAN_POINT('Ctrl Pts',(64.9288018797564,7.16309381772388,6.63642564979216));
#41457=CARTESIAN_POINT('Ctrl Pts',(64.9288458571943,7.16309972467879,6.63629669110962));
#41458=CARTESIAN_POINT('Ctrl Pts',(64.9288898326923,7.16310563127935,6.63616773234612));
#41459=CARTESIAN_POINT('Ctrl Pts',(64.9289338062505,7.16311153752559,6.63603877350158));
#41460=CARTESIAN_POINT('Ctrl Pts',(64.9503545652844,7.16598863646083,6.57321928728059));
#41461=CARTESIAN_POINT('Ctrl Pts',(64.971388959141,7.16876609138983,6.51005745533909));
#41462=CARTESIAN_POINT('Ctrl Pts',(64.9920390165022,7.17144233608347,6.44669889230024));
#41463=CARTESIAN_POINT('Ctrl Pts',(65.0126890738633,7.17411858077712,6.3833403292614));
#41464=CARTESIAN_POINT('Ctrl Pts',(65.0329547982903,7.17669360798898,6.31978511582696));
#41465=CARTESIAN_POINT('Ctrl Pts',(65.0528373460216,7.17916647493196,6.25624184522514));
#41466=CARTESIAN_POINT('Ctrl Pts',(65.0561770622229,7.17958184794677,6.24556833933532));
#41467=CARTESIAN_POINT('Ctrl Pts',(65.0595059651528,7.17999434009969,6.23489531721834));
#41468=CARTESIAN_POINT('Ctrl Pts',(65.0628240555067,7.18040395591848,6.224222671335));
#41469=CARTESIAN_POINT('Ctrl Pts',(65.0931664635859,7.18414970392527,6.12662624021454));
#41470=CARTESIAN_POINT('Ctrl Pts',(65.1226050606912,7.18765453668743,6.02906556129779));
#41471=CARTESIAN_POINT('Ctrl Pts',(65.1511379065764,7.19092499995632,5.93142984372355));
#41472=CARTESIAN_POINT('Ctrl Pts',(65.1565797849785,7.19154875348933,5.9128084378924));
#41473=CARTESIAN_POINT('Ctrl Pts',(65.161988703818,7.19216399537294,5.89418415118355));
#41474=CARTESIAN_POINT('Ctrl Pts',(65.1673646324934,7.19277079005854,5.87555600259647));
#41475=CARTESIAN_POINT('Ctrl Pts',(65.2154331838497,7.19819640919683,5.70899350315027));
#41476=CARTESIAN_POINT('Ctrl Pts',(65.2608667358397,7.20294399273001,5.54211906858637));
#41477=CARTESIAN_POINT('Ctrl Pts',(65.3036270097848,7.20706869339074,5.37495061458637));
#41478=CARTESIAN_POINT('Ctrl Pts',(65.3257800655607,7.20920560027571,5.28834471280473));
#41479=CARTESIAN_POINT('Ctrl Pts',(65.3472150985877,7.21117586345505,5.20166043892277));
#41480=CARTESIAN_POINT('Ctrl Pts',(65.3679238187994,7.21299045865816,5.11490335790102));
#41481=CARTESIAN_POINT('Ctrl Pts',(65.4115654921534,7.21681454678692,4.9320709977942));
#41482=CARTESIAN_POINT('Ctrl Pts',(65.4519830723729,7.21994485461651,4.74891823145015));
#41483=CARTESIAN_POINT('Ctrl Pts',(65.489077587359,7.22252585471296,4.56541184608723));
#41484=CARTESIAN_POINT('Ctrl Pts',(65.5282164754697,7.22524910029323,4.37179195681246));
#41485=CARTESIAN_POINT('Ctrl Pts',(65.5636555909094,7.22736125746581,4.17777881063003));
#41486=CARTESIAN_POINT('Ctrl Pts',(65.5952517618632,7.22907154405549,3.9832989377398));
#41487=CARTESIAN_POINT('Ctrl Pts',(65.6118700002137,7.22997108185823,3.88101081913205));
#41488=CARTESIAN_POINT('Ctrl Pts',(65.6274247555755,7.23076005347637,3.7785929856992));
#41489=CARTESIAN_POINT('Ctrl Pts',(65.6418928693717,7.23147220065846,3.67603076236863));
#41490=CARTESIAN_POINT('Ctrl Pts',(65.6452225762008,7.23163609495518,3.65242698510805));
#41491=CARTESIAN_POINT('Ctrl Pts',(65.6484956836855,7.23179605039584,3.62882003309272));
#41492=CARTESIAN_POINT('Ctrl Pts',(65.6517118944198,7.23195248664629,3.60520988238758));
#41493=CARTESIAN_POINT('Ctrl Pts',(65.6809645779071,7.23337533499121,3.39046640855726));
#41494=CARTESIAN_POINT('Ctrl Pts',(65.7055108831295,7.23450635373548,3.17546255458444));
#41495=CARTESIAN_POINT('Ctrl Pts',(65.7251244766241,7.23564865272918,2.96012537847259));
#41496=CARTESIAN_POINT('Ctrl Pts',(65.7443070624322,7.2367658497625,2.74952022549235));
#41497=CARTESIAN_POINT('Ctrl Pts',(65.7587707928361,7.23789538119044,2.53859610056453));
#41498=CARTESIAN_POINT('Ctrl Pts',(65.7683035228476,7.23931496822057,2.32723654627968));
#41499=CARTESIAN_POINT('Ctrl Pts',(65.7706053312466,7.23965774697809,2.27620088318106));
#41500=CARTESIAN_POINT('Ctrl Pts',(65.7726196584985,7.24001735093067,2.22513961330637));
#41501=CARTESIAN_POINT('Ctrl Pts',(65.7743435705949,7.24039748436144,2.17405067881274));
#41502=CARTESIAN_POINT('Ctrl Pts',(65.7789289220895,7.24140858312839,2.03816166067096));
#41503=CARTESIAN_POINT('Ctrl Pts',(65.7814658400794,7.24256751566722,1.90208027562438));
#41504=CARTESIAN_POINT('Ctrl Pts',(65.7818938839385,7.24392674011077,1.76655218109663));
#41505=CARTESIAN_POINT('Ctrl Pts',(65.7822577194509,7.24508207527429,1.65135386046897));
#41506=CARTESIAN_POINT('Ctrl Pts',(65.7810981991626,7.24638198058078,1.53655483801955));
#41507=CARTESIAN_POINT('Ctrl Pts',(65.778398635131,7.24784312512079,1.42259784523347));
#41508=CARTESIAN_POINT('Ctrl Pts',(65.7759936138484,7.24914484779693,1.32107441784296));
#41509=CARTESIAN_POINT('Ctrl Pts',(65.7723418318705,7.25057459162317,1.21984766497745));
#41510=CARTESIAN_POINT('Ctrl Pts',(65.7674933210383,7.25218497646143,1.11758555148493));
#41511=CARTESIAN_POINT('Ctrl Pts',(65.7629022371217,7.25370985950005,1.02075294436282));
#41512=CARTESIAN_POINT('Ctrl Pts',(65.757238274101,7.25539653525347,0.922992088228064));
#41513=CARTESIAN_POINT('Ctrl Pts',(65.7505069779292,7.25730958972767,0.823191555098794));
#41514=CARTESIAN_POINT('Ctrl Pts',(65.7471237017694,7.25827112691603,0.773029928591891));
#41515=CARTESIAN_POINT('Ctrl Pts',(65.7434701828239,7.25929018905904,0.722353333373553));
#41516=CARTESIAN_POINT('Ctrl Pts',(65.7395430551969,7.26037728034992,0.67102260240682));
#41517=CARTESIAN_POINT('',(64.0813578732502,7.1147451735158,-4.9214479327892));
#41518=CARTESIAN_POINT('Ctrl Pts',(65.7389291876497,7.26161795425529,0.664499595664831));
#41519=CARTESIAN_POINT('Ctrl Pts',(65.6986423579354,7.27296271621864,0.136607376960506));
#41520=CARTESIAN_POINT('Ctrl Pts',(65.5570967288631,7.2462698730418,-0.89745620523494));
#41521=CARTESIAN_POINT('Ctrl Pts',(65.1937668335651,7.14243217860219,-2.35375057630837));
#41522=CARTESIAN_POINT('Ctrl Pts',(64.6990534903062,7.0525690841578,-3.71481086803514));
#41523=CARTESIAN_POINT('Ctrl Pts',(64.2978125074662,7.07524290401267,-4.54781307837155));
#41524=CARTESIAN_POINT('Ctrl Pts',(64.0834287546126,7.11436614001603,-4.91787404424419));
#41525=CARTESIAN_POINT('',(59.0519282969413,7.75264142256226,-10.7028394440091));
#41526=CARTESIAN_POINT('Ctrl Pts',(64.0813578732502,7.1147451735158,-4.9214479327892));
#41527=CARTESIAN_POINT('Ctrl Pts',(63.522973579707,7.21724646178511,-5.88488505418209));
#41528=CARTESIAN_POINT('Ctrl Pts',(62.4349210154288,7.7808032321029,-7.50485479394792));
#41529=CARTESIAN_POINT('Ctrl Pts',(60.809824883128,7.8967925806761,-9.23021697908096));
#41530=CARTESIAN_POINT('Ctrl Pts',(59.9445192777259,7.84863591825408,-10.0113807547288));
#41531=CARTESIAN_POINT('Ctrl Pts',(59.4379281617953,7.7981238809332,-10.4193877736077));
#41532=CARTESIAN_POINT('Ctrl Pts',(59.1799059046439,7.77152332437818,-10.6198965981888));
#41533=CARTESIAN_POINT('Ctrl Pts',(59.0519282969413,7.75264142256226,-10.7028394440091));
#41534=CARTESIAN_POINT('Ctrl Pts',(59.0488631773053,7.75218963151952,-10.7048255423251));
#41535=CARTESIAN_POINT('Ctrl Pts',(58.0478420217809,7.60478481070341,-11.3533179919244));
#41536=CARTESIAN_POINT('Ctrl Pts',(55.8925355385909,7.56804290542898,-12.4812965801815));
#41537=CARTESIAN_POINT('Ctrl Pts',(52.1729677903268,7.39852199644268,-13.4768906188369));
#41538=CARTESIAN_POINT('Ctrl Pts',(48.3643075999864,6.35380835363947,-13.5778554041427));
#41539=CARTESIAN_POINT('Ctrl Pts',(46.0737017506393,5.40581314007301,-13.2335334133338));
#41540=CARTESIAN_POINT('Ctrl Pts',(44.9671960021647,5.06936132425713,-12.9468323394379));
#41541=CARTESIAN_POINT('Ctrl Pts',(-78.4945771627079,9.05474218205592,24.842213566055));
#41542=CARTESIAN_POINT('Ctrl Pts',(-78.4942430393453,9.0549729145804,24.7937000767725));
#41543=CARTESIAN_POINT('Ctrl Pts',(-78.493893310809,9.05521430182308,24.7452145480178));
#41544=CARTESIAN_POINT('Ctrl Pts',(-78.4897721700274,9.05806595339949,24.1983805187352));
#41545=CARTESIAN_POINT('Ctrl Pts',(-78.4800323908824,9.0588894037684,23.1810818557846));
#41546=CARTESIAN_POINT('Ctrl Pts',(-78.453292839765,9.059173840812,21.18718883834));
#41547=CARTESIAN_POINT('Ctrl Pts',(-78.4267803867925,9.07675855169213,19.7108117288188));
#41548=CARTESIAN_POINT('Ctrl Pts',(-78.4038531589849,9.1189183801019,18.4955202792461));
#41549=CARTESIAN_POINT('Ctrl Pts',(-78.3943810292591,9.13428496488478,17.9735826164074));
#41550=CARTESIAN_POINT('Ctrl Pts',(-78.3757398731157,9.158365928414,16.9680205844024));
#41551=CARTESIAN_POINT('Ctrl Pts',(-78.3430924629631,9.20103363542677,15.2406507036223));
#41552=CARTESIAN_POINT('Ctrl Pts',(-78.3160481524978,9.29112547810365,13.8416236115423));
#41553=CARTESIAN_POINT('Ctrl Pts',(-78.2931666472542,9.45650110611498,12.7110809531426));
#41554=CARTESIAN_POINT('Ctrl Pts',(-78.2830149502941,9.53239101935469,12.2435591992148));
#41555=CARTESIAN_POINT('Ctrl Pts',(-78.2621377476868,9.7127340787664,11.3046239100435));
#41556=CARTESIAN_POINT('Ctrl Pts',(-78.233855153337,9.98806838959211,10.1083484386801));
#41557=CARTESIAN_POINT('Ctrl Pts',(-78.1944828593662,10.3777342049461,8.64934200022291));
#41558=CARTESIAN_POINT('Ctrl Pts',(-78.1618184396354,10.6635084371553,7.66205018358527));
#41559=CARTESIAN_POINT('Ctrl Pts',(-78.1387930513469,10.8452663063005,7.04333861977662));
#41560=CARTESIAN_POINT('Ctrl Pts',(-78.133402700815,10.912869808309,6.83011671310147));
#41561=CARTESIAN_POINT('Ctrl Pts',(-78.1149695289094,11.064995924835,6.37324722091285));
#41562=CARTESIAN_POINT('Ctrl Pts',(-78.0725840850058,11.3579840167717,5.55881334907034));
#41563=CARTESIAN_POINT('Ctrl Pts',(-77.9532365531557,12.0288854151737,3.83067012142867));
#41564=CARTESIAN_POINT('Ctrl Pts',(-77.8411159275384,12.6322932422376,2.21795993639161));
#41565=CARTESIAN_POINT('Ctrl Pts',(-77.8221287620908,12.9420213178242,0.991067409735633));
#41566=CARTESIAN_POINT('Ctrl Pts',(-77.8217435561929,12.9760180772211,0.857310714534967));
#41567=CARTESIAN_POINT('Ctrl Pts',(-77.8220736569469,13.0435990014378,0.583493345690348));
#41568=CARTESIAN_POINT('Ctrl Pts',(-77.8278046968341,13.1564804673548,0.109426405530356));
#41569=CARTESIAN_POINT('Ctrl Pts',(-77.8482438214774,13.304977041924,-0.565538588983384));
#41570=CARTESIAN_POINT('Ctrl Pts',(-77.8892172593172,13.4622340620191,-1.36766559761172));
#41571=CARTESIAN_POINT('Ctrl Pts',(-77.959952732425,13.6450724388,-2.42940282804239));
#41572=CARTESIAN_POINT('Ctrl Pts',(-78.0675394978228,13.824152611481,-3.74125436564201));
#41573=CARTESIAN_POINT('Ctrl Pts',(-78.1459494468364,13.9210022962567,-4.77639531899031));
#41574=CARTESIAN_POINT('Ctrl Pts',(-78.1832005730778,13.9704832935621,-5.42026978261095));
#41575=CARTESIAN_POINT('Ctrl Pts',(-78.1979784088637,13.9887758338138,-5.70207633600367));
#41576=CARTESIAN_POINT('Ctrl Pts',(-78.2284833960188,14.0140574631234,-6.2466200716614));
#41577=CARTESIAN_POINT('Ctrl Pts',(-78.2828487750725,14.034352423442,-7.19391985365614));
#41578=CARTESIAN_POINT('Ctrl Pts',(-78.3592784126476,14.0116276257462,-8.50392380560081));
#41579=CARTESIAN_POINT('Ctrl Pts',(-78.4241139961074,13.9655621504964,-9.76132886787205));
#41580=CARTESIAN_POINT('Ctrl Pts',(-78.4590782716348,13.9419667305869,-10.6099301044122));
#41581=CARTESIAN_POINT('Ctrl Pts',(-78.4754805876884,13.9336604987353,-11.0859876724879));
#41582=CARTESIAN_POINT('Ctrl Pts',(-78.4823943700663,13.9316620148722,-11.320827749481));
#41583=CARTESIAN_POINT('Ctrl Pts',(-78.4870806277781,13.9311209038135,-11.4967547220627));
#41584=CARTESIAN_POINT('Ctrl Pts',(-78.4900109429774,13.9307491749155,-11.6230481807716));
#41585=CARTESIAN_POINT('Ctrl Pts',(-78.4950039243602,13.9302052683135,-11.8709752846205));
#41586=CARTESIAN_POINT('Ctrl Pts',(-78.50158798223,13.9296731190014,-12.306866865955));
#41587=CARTESIAN_POINT('Ctrl Pts',(-78.5070362894155,13.9302180558575,-13.1764566391381));
#41588=CARTESIAN_POINT('Ctrl Pts',(-78.497971327531,13.9345131198473,-14.4200831305645));
#41589=CARTESIAN_POINT('Ctrl Pts',(-78.482140644731,13.939588022815,-15.5449301391067));
#41590=CARTESIAN_POINT('Ctrl Pts',(-78.4736152025284,13.9422773104388,-16.299632681148));
#41591=CARTESIAN_POINT('Ctrl Pts',(-78.4688194777899,13.9438174524136,-16.8040925592002));
#41592=CARTESIAN_POINT('Ctrl Pts',(-78.4666111678699,13.9446078703403,-17.1842824856503));
#41593=CARTESIAN_POINT('Ctrl Pts',(-78.4659788038903,13.944970277296,-17.5013553829099));
#41594=CARTESIAN_POINT('Ctrl Pts',(-78.4657361371791,13.9451041184716,-17.6259545333056));
#41595=CARTESIAN_POINT('Ctrl Pts',(-78.4652797768498,13.9453411302425,-17.8757845538622));
#41596=CARTESIAN_POINT('Ctrl Pts',(-78.4648652232822,13.9455334668203,-18.1255165553471));
#41597=CARTESIAN_POINT('Ctrl Pts',(-78.4644893805365,13.9456854776639,-18.3754472022896));
#41598=CARTESIAN_POINT('Ctrl Pts',(-78.4642698390973,13.9457647728761,-18.5316752423212));
#41599=CARTESIAN_POINT('Ctrl Pts',(-78.4641030424882,13.9458192895378,-18.6566913664842));
#41600=CARTESIAN_POINT('Ctrl Pts',(-78.463982245853,13.9458558892278,-18.7504648090307));
#41601=CARTESIAN_POINT('Ctrl Pts',(-78.4638850796552,13.9458829377025,-18.8286218460667));
#41602=CARTESIAN_POINT('Ctrl Pts',(-78.4638093983772,13.9459025641903,-18.8911536255898));
#41603=CARTESIAN_POINT('Ctrl Pts',(-78.4631775351181,13.9460583154654,-19.422716488597));
#41604=CARTESIAN_POINT('Ctrl Pts',(-78.4623252407263,13.9460139894593,-20.4402842043313));
#41605=CARTESIAN_POINT('Ctrl Pts',(-78.461663196691,13.9455458166235,-21.9471797599321));
#41606=CARTESIAN_POINT('Ctrl Pts',(-78.46133516632,13.9453589828729,-22.954942534609));
#41607=CARTESIAN_POINT('Ctrl Pts',(-78.4610782904957,13.9454019364029,-23.5841024904954));
#41608=CARTESIAN_POINT('Ctrl Pts',(-78.4609887806561,13.9454201016436,-23.8333894280329));
#41609=CARTESIAN_POINT('Ctrl Pts',(-78.4608536657511,13.9454604662962,-24.3326208461672));
#41610=CARTESIAN_POINT('Ctrl Pts',(-78.46072122286,13.9455386704867,-25.2081915803845));
#41611=CARTESIAN_POINT('Ctrl Pts',(-78.4607646129605,13.9456564764122,-26.4630707118391));
#41612=CARTESIAN_POINT('Ctrl Pts',(-78.4609833447558,13.9457527260614,-27.9715986022803));
#41613=CARTESIAN_POINT('Ctrl Pts',(-78.4611025507938,13.9457535017472,-28.976520387269));
#41614=CARTESIAN_POINT('Ctrl Pts',(-78.4611236704402,13.9457254084153,-29.5408216774617));
#41615=CARTESIAN_POINT('Ctrl Pts',(-78.4611270417918,13.9457179309976,-29.6662231218047));
#41616=CARTESIAN_POINT('Ctrl Pts',(-78.4611289989437,13.9456985609124,-29.9170775247896));
#41617=CARTESIAN_POINT('Ctrl Pts',(-78.4611213062099,13.9456539467802,-30.356213341546));
#41618=CARTESIAN_POINT('Ctrl Pts',(-78.4610732406616,13.9455273503159,-31.2348958611842));
#41619=CARTESIAN_POINT('Ctrl Pts',(-78.4609779260847,13.9452750970535,-32.4906412748349));
#41620=CARTESIAN_POINT('Ctrl Pts',(-78.4610256022749,13.9450184448771,-33.7450945614149));
#41621=CARTESIAN_POINT('Ctrl Pts',(-78.461256827609,13.9448645106084,-34.7467138664715));
#41622=CARTESIAN_POINT('Ctrl Pts',(-78.461454504277,13.944814809868,-35.2466998259681));
#41623=CARTESIAN_POINT('Ctrl Pts',(-78.4616408300557,13.9447904868293,-35.6223062979808));
#41624=CARTESIAN_POINT('Ctrl Pts',(-78.4617840518671,13.9447551008324,-35.8741696983526));
#41625=CARTESIAN_POINT('Ctrl Pts',(-78.4621352014927,13.9446227499953,-36.3769681150403));
#41626=CARTESIAN_POINT('Ctrl Pts',(-78.4628959419818,13.9442741979241,-37.2553128798882));
#41627=CARTESIAN_POINT('Ctrl Pts',(-78.4648207036372,13.9434162779456,-39.0069967221859));
#41628=CARTESIAN_POINT('Ctrl Pts',(-78.4665267377335,13.9435422548098,-40.5068899792746));
#41629=CARTESIAN_POINT('Ctrl Pts',(-78.4672797289669,13.9453373815765,-41.761281264071));
#41630=CARTESIAN_POINT('Ctrl Pts',(-78.46744861403,13.9454019902603,-42.1397854152623));
#41631=CARTESIAN_POINT('Ctrl Pts',(-78.4675940368839,13.9449412810732,-42.6420714244579));
#41632=CARTESIAN_POINT('Ctrl Pts',(-78.4676956880371,13.9442556435418,-43.1445884596069));
#41633=CARTESIAN_POINT('Ctrl Pts',(-78.4677599030067,13.9432273462217,-43.7718110326914));
#41634=CARTESIAN_POINT('Ctrl Pts',(-78.4677971292163,13.9425265168204,-44.5229801602098));
#41635=CARTESIAN_POINT('Ctrl Pts',(-78.4678464599873,13.9430529812452,-45.1471072402556));
#41636=CARTESIAN_POINT('Ctrl Pts',(-78.4679291472011,13.9445307104614,-45.6451047526845));
#41637=CARTESIAN_POINT('Ctrl Pts',(-78.468020348216,13.9462682631092,-46.0178540945607));
#41638=CARTESIAN_POINT('Ctrl Pts',(-78.468148706838,13.9487332459747,-46.3898211447335));
#41639=CARTESIAN_POINT('Ctrl Pts',(-78.4683807861075,13.9531152796023,-46.8845673874527));
#41640=CARTESIAN_POINT('Ctrl Pts',(-78.4686337170895,13.9577929720615,-47.2543487105996));
#41641=CARTESIAN_POINT('Ctrl Pts',(-78.4689592301306,13.9635854610414,-47.6235305242231));
#41642=CARTESIAN_POINT('Ctrl Pts',(-78.4692251198566,13.9686209787161,-47.8578271164692));
#41643=CARTESIAN_POINT('Ctrl Pts',(-78.4697866257101,13.9835436409415,-48.3393103705291));
#41644=CARTESIAN_POINT('Ctrl Pts',(-78.470862112878,14.0198646528519,-49.1904283836821));
#41645=CARTESIAN_POINT('Ctrl Pts',(-78.4724213367011,14.0887986766884,-50.4447004208244));
#41646=CARTESIAN_POINT('Ctrl Pts',(-78.4743226796318,14.1545233458233,-52.0044960456846));
#41647=CARTESIAN_POINT('Ctrl Pts',(-78.4760762905936,14.1541375255512,-53.0821713269056));
#41648=CARTESIAN_POINT('Ctrl Pts',(-78.4776544781521,14.1284631318028,-53.7698156147898));
#41649=CARTESIAN_POINT('Ctrl Pts',(-78.4785936774332,14.1115115093101,-54.0753552476011));
#41650=CARTESIAN_POINT('Ctrl Pts',(-78.4807458995816,14.0605153672445,-54.6538882081308));
#41651=CARTESIAN_POINT('Ctrl Pts',(-78.4848308816969,13.9360332161937,-55.6360647071896));
#41652=CARTESIAN_POINT('Ctrl Pts',(-78.491877924565,13.6174829420838,-57.4442356893185));
#41653=CARTESIAN_POINT('Ctrl Pts',(-78.4899803670269,13.4538371774993,-58.73175430535));
#41654=CARTESIAN_POINT('Ctrl Pts',(-78.4939878848484,13.5005570278821,-59.4963920718888));
#41655=CARTESIAN_POINT('Ctrl Pts',(-78.494330086782,13.5081132678948,-59.6097203027396));
#41656=CARTESIAN_POINT('Ctrl Pts',(-78.4951351392656,13.52569399078,-59.8258300441764));
#41657=CARTESIAN_POINT('Ctrl Pts',(-78.4965765226948,13.5647737988659,-60.2118618597667));
#41658=CARTESIAN_POINT('Ctrl Pts',(-78.4997259099805,13.6737008935838,-60.9876947457136));
#41659=CARTESIAN_POINT('Ctrl Pts',(-78.5035267773202,13.8644901121535,-61.8929344593412));
#41660=CARTESIAN_POINT('Ctrl Pts',(-78.5071315715766,14.110557833353,-62.8075866929281));
#41661=CARTESIAN_POINT('Ctrl Pts',(-78.5090479495058,14.2673734772625,-63.3251314989186));
#41662=CARTESIAN_POINT('Ctrl Pts',(-78.5102654963792,14.3786007391778,-63.670806276571));
#41663=CARTESIAN_POINT('Ctrl Pts',(-78.5110606059872,14.4544665900404,-63.9014452479474));
#41664=CARTESIAN_POINT('Ctrl Pts',(-78.5118344655014,14.5327699112622,-64.1321796205846));
#41665=CARTESIAN_POINT('Ctrl Pts',(-78.5124870725892,14.6032711905195,-64.3342200226466));
#41666=CARTESIAN_POINT('Ctrl Pts',(-78.5128531780397,14.6440966265582,-64.4496929118452));
#41667=CARTESIAN_POINT('Ctrl Pts',(-78.5133969953046,14.7058497796128,-64.6228914162233));
#41668=CARTESIAN_POINT('Ctrl Pts',(-78.5138341200789,14.7583905987037,-64.7672726597123));
#41669=CARTESIAN_POINT('Ctrl Pts',(-78.5145728733114,14.8464089436773,-65.0056542132996));
#41670=CARTESIAN_POINT('Ctrl Pts',(-78.5170679509954,14.9292431087916,-65.2185839665801));
#41671=CARTESIAN_POINT('Ctrl Pts',(-78.5208802770348,15.1184939346135,-65.6685774085504));
#41672=CARTESIAN_POINT('Ctrl Pts',(-78.5273486236522,15.4869686409682,-66.4580791550208));
#41673=CARTESIAN_POINT('Ctrl Pts',(-78.5357663537906,16.3671014409282,-68.0970395735812));
#41674=CARTESIAN_POINT('Ctrl Pts',(-78.5339375754532,17.265256936789,-69.5915577692196));
#41675=CARTESIAN_POINT('Ctrl Pts',(-78.5285044735435,17.8967482249873,-70.7930139720104));
#41676=CARTESIAN_POINT('Ctrl Pts',(-78.5289803247857,18.0256326228804,-71.037566404661));
#41677=CARTESIAN_POINT('Ctrl Pts',(-78.5289445405091,18.2909799306739,-71.5400815342296));
#41678=CARTESIAN_POINT('Ctrl Pts',(-78.5292654390903,18.6209759850393,-72.1628107133783));
#41679=CARTESIAN_POINT('Ctrl Pts',(-78.5293800439328,19.0200253462203,-72.9134949573155));
#41680=CARTESIAN_POINT('Ctrl Pts',(-78.5296335577199,19.8195296036977,-74.4139812794394));
#41681=CARTESIAN_POINT('Ctrl Pts',(-78.5295981985945,20.4894190367254,-75.6668216819808));
#41682=CARTESIAN_POINT('Ctrl Pts',(-78.5293329625961,21.4611343311253,-77.4942136478313));
#41683=CARTESIAN_POINT('Ctrl Pts',(-78.5294483398302,21.8968341110043,-78.3135083159309));
#41684=CARTESIAN_POINT('Ctrl Pts',(-78.5294483398211,22.3333556983922,-79.1344860180165));
#41685=CARTESIAN_POINT('Ctrl Pts',(-77.5605622313936,8.92234122508525,24.8316381486366));
#41686=CARTESIAN_POINT('Ctrl Pts',(-77.5604387774315,8.92234787215812,24.7827885464113));
#41687=CARTESIAN_POINT('Ctrl Pts',(-77.5603096057366,8.92235475347985,24.7339548758836));
#41688=CARTESIAN_POINT('Ctrl Pts',(-77.5587942555384,8.92244266640463,24.1833219152387));
#41689=CARTESIAN_POINT('Ctrl Pts',(-77.554258549875,8.91820891771524,23.1672059573088));
#41690=CARTESIAN_POINT('Ctrl Pts',(-77.541451457475,8.90545403671313,21.1638359878524));
#41691=CARTESIAN_POINT('Ctrl Pts',(-77.5317639126002,8.90605198121365,19.6764549410896));
#41692=CARTESIAN_POINT('Ctrl Pts',(-77.5283075185792,8.92708953511933,18.4485053088963));
#41693=CARTESIAN_POINT('Ctrl Pts',(-77.5287626473163,8.93213707683049,17.9183678770559));
#41694=CARTESIAN_POINT('Ctrl Pts',(-77.5347537825327,8.9333601545357,16.903190119934));
#41695=CARTESIAN_POINT('Ctrl Pts',(-77.5518195499198,8.93282314541542,15.168894290023));
#41696=CARTESIAN_POINT('Ctrl Pts',(-77.5546312711207,8.9885250482066,13.7837693440693));
#41697=CARTESIAN_POINT('Ctrl Pts',(-77.53359507326,9.12199597784422,12.672244322638));
#41698=CARTESIAN_POINT('Ctrl Pts',(-77.5229667840858,9.18515494747207,12.2030199939226));
#41699=CARTESIAN_POINT('Ctrl Pts',(-77.4981187857294,9.3358461525626,11.2681351002097));
#41700=CARTESIAN_POINT('Ctrl Pts',(-77.4600782135362,9.5697676915878,10.0771246130041));
#41701=CARTESIAN_POINT('Ctrl Pts',(-77.403506324231,9.91002280123826,8.62883552518502));
#41702=CARTESIAN_POINT('Ctrl Pts',(-77.3557053914638,10.1680431025947,7.65099599076623));
#41703=CARTESIAN_POINT('Ctrl Pts',(-77.3215767830405,10.3355620495419,7.03954778271346));
#41704=CARTESIAN_POINT('Ctrl Pts',(-77.3107744956535,10.3973824621495,6.82725579207872));
#41705=CARTESIAN_POINT('Ctrl Pts',(-77.2797725803335,10.5379845248233,6.37265413598938));
#41706=CARTESIAN_POINT('Ctrl Pts',(-77.2107099444863,10.8112098277032,5.56059953382364));
#41707=CARTESIAN_POINT('Ctrl Pts',(-77.0244810600929,11.4499454185789,3.83707431163502));
#41708=CARTESIAN_POINT('Ctrl Pts',(-76.8477432926891,12.0395828792395,2.23630315428687));
#41709=CARTESIAN_POINT('Ctrl Pts',(-76.8046079877836,12.364444511154,1.0247750956615));
#41710=CARTESIAN_POINT('Ctrl Pts',(-76.8019223014061,12.3999715081068,0.895013675434835));
#41711=CARTESIAN_POINT('Ctrl Pts',(-76.7976649249607,12.4720640570219,0.62764000810655));
#41712=CARTESIAN_POINT('Ctrl Pts',(-76.7962844213738,12.5955669638363,0.164676117981452));
#41713=CARTESIAN_POINT('Ctrl Pts',(-76.8083097193984,12.7670560255125,-0.497218249202318));
#41714=CARTESIAN_POINT('Ctrl Pts',(-76.8424049921976,12.9615331517708,-1.2878859532549));
#41715=CARTESIAN_POINT('Ctrl Pts',(-76.9076048367717,13.2025207156588,-2.34038669747703));
#41716=CARTESIAN_POINT('Ctrl Pts',(-77.0165986235876,13.4605791888376,-3.65307361606854));
#41717=CARTESIAN_POINT('Ctrl Pts',(-77.1017170835597,13.609227067021,-4.7029565071481));
#41718=CARTESIAN_POINT('Ctrl Pts',(-77.1431811253545,13.6838611873837,-5.36001763704743));
#41719=CARTESIAN_POINT('Ctrl Pts',(-77.1600451514562,13.7125934766704,-5.6412449157383));
#41720=CARTESIAN_POINT('Ctrl Pts',(-77.1965197113903,13.7579444542025,-6.18838193223148));
#41721=CARTESIAN_POINT('Ctrl Pts',(-77.2651383971875,13.8118043448065,-7.13931324784504));
#41722=CARTESIAN_POINT('Ctrl Pts',(-77.3690417908761,13.830839847122,-8.45694301051994));
#41723=CARTESIAN_POINT('Ctrl Pts',(-77.4621505355479,13.8168121760837,-9.72343570812446));
#41724=CARTESIAN_POINT('Ctrl Pts',(-77.5129001275405,13.8093477664188,-10.5800393080932));
#41725=CARTESIAN_POINT('Ctrl Pts',(-77.5363598234594,13.8083967802335,-11.0609170898356));
#41726=CARTESIAN_POINT('Ctrl Pts',(-77.5460246624927,13.8094608419419,-11.2982581903072));
#41727=CARTESIAN_POINT('Ctrl Pts',(-77.5524436116671,13.8110046780333,-11.4761248034273));
#41728=CARTESIAN_POINT('Ctrl Pts',(-77.5564449255508,13.8120124718556,-11.6047405441445));
#41729=CARTESIAN_POINT('Ctrl Pts',(-77.5632774692677,13.8137480384397,-11.8565145078029));
#41730=CARTESIAN_POINT('Ctrl Pts',(-77.5722937764428,13.8161794316539,-12.2989111630824));
#41731=CARTESIAN_POINT('Ctrl Pts',(-77.5797445566846,13.818941441053,-13.1791401492147));
#41732=CARTESIAN_POINT('Ctrl Pts',(-77.5674968670907,13.8186385187503,-14.4318739954401));
#41733=CARTESIAN_POINT('Ctrl Pts',(-77.5461666858491,13.81583301518,-15.5574007012155));
#41734=CARTESIAN_POINT('Ctrl Pts',(-77.534708353667,13.8142366747743,-16.3094388277202));
#41735=CARTESIAN_POINT('Ctrl Pts',(-77.528288033385,13.8133710490608,-16.8112944245664));
#41736=CARTESIAN_POINT('Ctrl Pts',(-77.5253230418953,13.813039309252,-17.1885873651413));
#41737=CARTESIAN_POINT('Ctrl Pts',(-77.5245053831638,13.8130914149489,-17.5028070181097));
#41738=CARTESIAN_POINT('Ctrl Pts',(-77.5241930537433,13.813110936165,-17.6275815282398));
#41739=CARTESIAN_POINT('Ctrl Pts',(-77.5236099127463,13.8131423047389,-17.8770136375089));
#41740=CARTESIAN_POINT('Ctrl Pts',(-77.5230795711236,13.8131600529192,-18.1266467012188));
#41741=CARTESIAN_POINT('Ctrl Pts',(-77.5226080070204,13.8131705608945,-18.3763473173682));
#41742=CARTESIAN_POINT('Ctrl Pts',(-77.5223335142488,13.8131728699296,-18.5324722230117));
#41743=CARTESIAN_POINT('Ctrl Pts',(-77.522126959027,13.8131730148287,-18.6573974883988));
#41744=CARTESIAN_POINT('Ctrl Pts',(-77.5219778740186,13.8131720644925,-18.7511081445821));
#41745=CARTESIAN_POINT('Ctrl Pts',(-77.5218584026611,13.8131704404636,-18.8292132885579));
#41746=CARTESIAN_POINT('Ctrl Pts',(-77.5217657900787,13.8131687381478,-18.8917050333239));
#41747=CARTESIAN_POINT('Ctrl Pts',(-77.5209932738126,13.8131511529393,-19.4229325698188));
#41748=CARTESIAN_POINT('Ctrl Pts',(-77.5199706551422,13.8130279794193,-20.4400524685141));
#41749=CARTESIAN_POINT('Ctrl Pts',(-77.5192704733705,13.8127761979766,-21.9468150252231));
#41750=CARTESIAN_POINT('Ctrl Pts',(-77.5188911458241,13.8126627894026,-22.9548469725142));
#41751=CARTESIAN_POINT('Ctrl Pts',(-77.518568691947,13.8126460353685,-23.5842755507642));
#41752=CARTESIAN_POINT('Ctrl Pts',(-77.5184561260384,13.8126414861031,-23.833527095969));
#41753=CARTESIAN_POINT('Ctrl Pts',(-77.5182802283595,13.8126387384901,-24.332765842506));
#41754=CARTESIAN_POINT('Ctrl Pts',(-77.5180898702341,13.8126484042317,-25.208305279854));
#41755=CARTESIAN_POINT('Ctrl Pts',(-77.5180804863412,13.8126898608283,-26.4631542351967));
#41756=CARTESIAN_POINT('Ctrl Pts',(-77.5182771608326,13.812743634875,-27.9716121803736));
#41757=CARTESIAN_POINT('Ctrl Pts',(-77.5183897450772,13.8127538497128,-28.9764797182323));
#41758=CARTESIAN_POINT('Ctrl Pts',(-77.518409404043,13.8127449387252,-29.5407448559064));
#41759=CARTESIAN_POINT('Ctrl Pts',(-77.5184126615536,13.8127424447381,-29.6661318629424));
#41760=CARTESIAN_POINT('Ctrl Pts',(-77.5184139821417,13.8127352953142,-29.9169626055781));
#41761=CARTESIAN_POINT('Ctrl Pts',(-77.5184042983497,13.8127176675713,-30.3560588133006));
#41762=CARTESIAN_POINT('Ctrl Pts',(-77.5183512122079,13.8126652565372,-31.2346783702434));
#41763=CARTESIAN_POINT('Ctrl Pts',(-77.518256016693,13.8125623200684,-32.4903746976785));
#41764=CARTESIAN_POINT('Ctrl Pts',(-77.5183410107469,13.8124753380149,-33.7448350377107));
#41765=CARTESIAN_POINT('Ctrl Pts',(-77.5186420139193,13.8124473588727,-34.7464932442673));
#41766=CARTESIAN_POINT('Ctrl Pts',(-77.5188895728758,13.8124531071784,-35.2465100432844));
#41767=CARTESIAN_POINT('Ctrl Pts',(-77.5191205277262,13.8124664844248,-35.6221434557117));
#41768=CARTESIAN_POINT('Ctrl Pts',(-77.5192975405256,13.8124566477443,-35.8740055899186));
#41769=CARTESIAN_POINT('Ctrl Pts',(-77.5197301121733,13.8123761438697,-36.3768125041924));
#41770=CARTESIAN_POINT('Ctrl Pts',(-77.5206639247282,13.8121190691633,-37.255166775776));
#41771=CARTESIAN_POINT('Ctrl Pts',(-77.5230204521266,13.8114433402877,-39.0068749104896));
#41772=CARTESIAN_POINT('Ctrl Pts',(-77.5251060267396,13.8117025312366,-40.5067885445302));
#41773=CARTESIAN_POINT('Ctrl Pts',(-77.5260313793896,13.81357505,-41.7611984172332));
#41774=CARTESIAN_POINT('Ctrl Pts',(-77.5262400106917,13.8136607899694,-42.1397051347198));
#41775=CARTESIAN_POINT('Ctrl Pts',(-77.5264214202809,13.8132243812615,-42.641997009049));
#41776=CARTESIAN_POINT('Ctrl Pts',(-77.5265497432783,13.812560662035,-43.1445200214958));
#41777=CARTESIAN_POINT('Ctrl Pts',(-77.5266338491028,13.8115556437239,-43.7717512237256));
#41778=CARTESIAN_POINT('Ctrl Pts',(-77.5266860831431,13.8108773220283,-44.5229321628846));
#41779=CARTESIAN_POINT('Ctrl Pts',(-77.5267510857491,13.8114189789815,-45.1470704258221));
#41780=CARTESIAN_POINT('Ctrl Pts',(-77.5268546649749,13.8129073872144,-45.6450777096892));
#41781=CARTESIAN_POINT('Ctrl Pts',(-77.5269672404777,13.8146523264497,-46.0178347862417));
#41782=CARTESIAN_POINT('Ctrl Pts',(-77.5271242715448,13.8171242298824,-46.3898099774271));
#41783=CARTESIAN_POINT('Ctrl Pts',(-77.5274064571625,13.8215150706867,-46.8845676431613));
#41784=CARTESIAN_POINT('Ctrl Pts',(-77.5277125964672,13.8261991156127,-47.2543581434956));
#41785=CARTESIAN_POINT('Ctrl Pts',(-77.5281051874555,13.8319981148867,-47.6235496848856));
#41786=CARTESIAN_POINT('Ctrl Pts',(-77.528417512923,13.8370375676126,-47.8578552969448));
#41787=CARTESIAN_POINT('Ctrl Pts',(-77.5290784121588,13.8519659591563,-48.3393536095675));
#41788=CARTESIAN_POINT('Ctrl Pts',(-77.5303452532985,13.8882920897764,-49.1904951739617));
#41789=CARTESIAN_POINT('Ctrl Pts',(-77.5322298106515,13.9572226845556,-50.4447903896764));
#41790=CARTESIAN_POINT('Ctrl Pts',(-77.5346109148192,14.0229378429031,-52.004597757606));
#41791=CARTESIAN_POINT('Ctrl Pts',(-77.5367463120574,14.0225525269654,-53.0822685809883));
#41792=CARTESIAN_POINT('Ctrl Pts',(-77.5385840020939,13.9968841947445,-53.7699063146854));
#41793=CARTESIAN_POINT('Ctrl Pts',(-77.5396350492413,13.9799334558601,-54.0754551446048));
#41794=CARTESIAN_POINT('Ctrl Pts',(-77.5420353655896,13.9289417295368,-54.6539965423128));
#41795=CARTESIAN_POINT('Ctrl Pts',(-77.5466086990039,13.8044720837318,-55.6361844457582));
#41796=CARTESIAN_POINT('Ctrl Pts',(-77.5547711897704,13.4859675619227,-57.4443539913586));
#41797=CARTESIAN_POINT('Ctrl Pts',(-77.5537829988704,13.3223909757157,-58.73184362296));
#41798=CARTESIAN_POINT('Ctrl Pts',(-77.5581488466774,13.3691402428739,-59.4964364928422));
#41799=CARTESIAN_POINT('Ctrl Pts',(-77.5585332519993,13.3766995350279,-59.6097599795229));
#41800=CARTESIAN_POINT('Ctrl Pts',(-77.5594169699108,13.3942864670697,-59.8258604061041));
#41801=CARTESIAN_POINT('Ctrl Pts',(-77.5609817760681,13.433376654244,-60.2118774312076));
#41802=CARTESIAN_POINT('Ctrl Pts',(-77.5643257108139,13.5423234571866,-60.9876860163811));
#41803=CARTESIAN_POINT('Ctrl Pts',(-77.5682512471025,13.733133786666,-61.8929101105795));
#41804=CARTESIAN_POINT('Ctrl Pts',(-77.5719270540266,13.9792222036695,-62.8075574722455));
#41805=CARTESIAN_POINT('Ctrl Pts',(-77.5738716287693,14.1360492148047,-63.3251033426239));
#41806=CARTESIAN_POINT('Ctrl Pts',(-77.5751065662629,14.2472839188875,-63.6707803575806));
#41807=CARTESIAN_POINT('Ctrl Pts',(-77.5759131347471,14.3231546834061,-63.9014212267432));
#41808=CARTESIAN_POINT('Ctrl Pts',(-77.5766985861895,14.4014628472646,-64.1321580938732));
#41809=CARTESIAN_POINT('Ctrl Pts',(-77.5773620846279,14.4719682833765,-64.3342012106559));
#41810=CARTESIAN_POINT('Ctrl Pts',(-77.5777347139773,14.5127960706364,-64.449675803314));
#41811=CARTESIAN_POINT('Ctrl Pts',(-77.5782886620031,14.5745527225633,-64.6228770100818));
#41812=CARTESIAN_POINT('Ctrl Pts',(-77.5787350351066,14.6270964076299,-64.7672608325005));
#41813=CARTESIAN_POINT('Ctrl Pts',(-77.5794906598248,14.7151193616744,-65.0056469690786));
#41814=CARTESIAN_POINT('Ctrl Pts',(-77.5820005722859,14.797955593113,-65.218575733287));
#41815=CARTESIAN_POINT('Ctrl Pts',(-77.5858348074542,14.9872106092925,-65.668570377743));
#41816=CARTESIAN_POINT('Ctrl Pts',(-77.5923226968906,15.3556889863614,-66.4580724359124));
#41817=CARTESIAN_POINT('Ctrl Pts',(-77.6007229792136,16.2358205060688,-68.0970342827442));
#41818=CARTESIAN_POINT('Ctrl Pts',(-77.5988428319072,17.1339682870552,-69.5915519625025));
#41819=CARTESIAN_POINT('Ctrl Pts',(-77.5934123976625,17.7654604108893,-70.7930076399653));
#41820=CARTESIAN_POINT('Ctrl Pts',(-77.5938881334521,17.8943448958101,-71.0375601872648));
#41821=CARTESIAN_POINT('Ctrl Pts',(-77.5938524835593,18.1596923809589,-71.5400754049442));
#41822=CARTESIAN_POINT('Ctrl Pts',(-77.5941733219395,18.4896885503407,-72.1628047092907));
#41823=CARTESIAN_POINT('Ctrl Pts',(-77.594287879392,18.8887379623775,-72.9134890543831));
#41824=CARTESIAN_POINT('Ctrl Pts',(-77.5945411639157,19.6882421618109,-74.4139755229999));
#41825=CARTESIAN_POINT('Ctrl Pts',(-77.5945055628805,20.3581313177361,-75.6668158185921));
#41826=CARTESIAN_POINT('Ctrl Pts',(-77.5942404436912,21.329846512682,-77.4942075142949));
#41827=CARTESIAN_POINT('Ctrl Pts',(-77.5943557645253,21.7655463117544,-78.3135022346463));
#41828=CARTESIAN_POINT('Ctrl Pts',(-77.5943557645153,22.2020678991426,-79.1344799367424));
#41829=CARTESIAN_POINT('Ctrl Pts',(-75.6921159965246,8.65897413900046,24.8219423290036));
#41830=CARTESIAN_POINT('Ctrl Pts',(-75.6923447613647,8.65879522040642,24.7727884167587));
#41831=CARTESIAN_POINT('Ctrl Pts',(-75.6925847365169,8.65860782647033,24.7236365407136));
#41832=CARTESIAN_POINT('Ctrl Pts',(-75.6954155315407,8.65639934571804,24.1696381817257));
#41833=CARTESIAN_POINT('Ctrl Pts',(-75.6994921847873,8.64926564283647,23.1576310625885));
#41834=CARTESIAN_POINT('Ctrl Pts',(-75.7102951838337,8.62911964770645,21.1444014910015));
#41835=CARTESIAN_POINT('Ctrl Pts',(-75.7290344711282,8.61493829029717,19.6425156660459));
#41836=CARTESIAN_POINT('Ctrl Pts',(-75.759278305029,8.61193125725722,18.3971139448735));
#41837=CARTESIAN_POINT('Ctrl Pts',(-75.7765502794134,8.60616141273255,17.8648515751132));
#41838=CARTESIAN_POINT('Ctrl Pts',(-75.8248824601033,8.58551179224008,16.8429356054507));
#41839=CARTESIAN_POINT('Ctrl Pts',(-75.929640513178,8.54295467644432,15.098977383154));
#41840=CARTESIAN_POINT('Ctrl Pts',(-75.997603174384,8.55594794995412,13.7000298821579));
#41841=CARTESIAN_POINT('Ctrl Pts',(-75.9829940661346,8.64280327427609,12.5772729490234));
#41842=CARTESIAN_POINT('Ctrl Pts',(-75.9733493918736,8.6841735069898,12.0967648569456));
#41843=CARTESIAN_POINT('Ctrl Pts',(-75.9416242162755,8.78166381994826,11.1511668134419));
#41844=CARTESIAN_POINT('Ctrl Pts',(-75.8808356906706,8.93169360542806,9.95649943037897));
#41845=CARTESIAN_POINT('Ctrl Pts',(-75.7828579358023,9.15097965676827,8.52048566943689));
#41846=CARTESIAN_POINT('Ctrl Pts',(-75.7043210034514,9.32436933204821,7.55803023860428));
#41847=CARTESIAN_POINT('Ctrl Pts',(-75.6511581152083,9.44176191124195,6.9578249226186));
#41848=CARTESIAN_POINT('Ctrl Pts',(-75.628363393581,9.48735617559372,6.73793790452049));
#41849=CARTESIAN_POINT('Ctrl Pts',(-75.5741769251662,9.58680749797722,6.27838908714747));
#41850=CARTESIAN_POINT('Ctrl Pts',(-75.4623493303006,9.77638255963925,5.46024348137765));
#41851=CARTESIAN_POINT('Ctrl Pts',(-75.2050639128527,10.2138340247438,3.74232314061025));
#41852=CARTESIAN_POINT('Ctrl Pts',(-75.0098015096056,10.663415287569,2.17056181264629));
#41853=CARTESIAN_POINT('Ctrl Pts',(-74.9456166558476,10.9820988934014,1.03851406443687));
#41854=CARTESIAN_POINT('Ctrl Pts',(-74.9408920572205,11.0178662505396,0.918945979694379));
#41855=CARTESIAN_POINT('Ctrl Pts',(-74.9313758811006,11.0933095500304,0.671107632293839));
#41856=CARTESIAN_POINT('Ctrl Pts',(-74.9190173258224,11.2300190033541,0.241491523103302));
#41857=CARTESIAN_POINT('Ctrl Pts',(-74.9108524012778,11.4382770412393,-0.376413458452138));
#41858=CARTESIAN_POINT('Ctrl Pts',(-74.9166341377895,11.6992118543583,-1.12272086716767));
#41859=CARTESIAN_POINT('Ctrl Pts',(-74.9432675005682,12.0514832952064,-2.13113802139702));
#41860=CARTESIAN_POINT('Ctrl Pts',(-75.0080517507911,12.4809013027542,-3.42363524866221));
#41861=CARTESIAN_POINT('Ctrl Pts',(-75.0748004827117,12.7669916964717,-4.50470312477017));
#41862=CARTESIAN_POINT('Ctrl Pts',(-75.1114900539174,12.9121996468757,-5.19585586668643));
#41863=CARTESIAN_POINT('Ctrl Pts',(-75.1270219536629,12.9687856032635,-5.4660722503953));
#41864=CARTESIAN_POINT('Ctrl Pts',(-75.1647137181936,13.0729691030591,-6.00823556293463));
#41865=CARTESIAN_POINT('Ctrl Pts',(-75.2447328180899,13.2331229490125,-6.95057580271206));
#41866=CARTESIAN_POINT('Ctrl Pts',(-75.3885826331589,13.3990097777801,-8.28181093903442));
#41867=CARTESIAN_POINT('Ctrl Pts',(-75.5306746339452,13.4951208489467,-9.57980856854873));
#41868=CARTESIAN_POINT('Ctrl Pts',(-75.6076564304303,13.5418799491235,-10.4683980241704));
#41869=CARTESIAN_POINT('Ctrl Pts',(-75.6426977577952,13.5653647317475,-10.9705730285057));
#41870=CARTESIAN_POINT('Ctrl Pts',(-75.6567932523914,13.5763949616513,-11.21968403738));
#41871=CARTESIAN_POINT('Ctrl Pts',(-75.665967802336,13.5845892879007,-11.4068849713555));
#41872=CARTESIAN_POINT('Ctrl Pts',(-75.6716767264812,13.5900584416014,-11.5428852548299));
#41873=CARTESIAN_POINT('Ctrl Pts',(-75.6815252715505,13.5991851699896,-11.8080322118912));
#41874=CARTESIAN_POINT('Ctrl Pts',(-75.6947836859738,13.6113211144299,-12.2724048014959));
#41875=CARTESIAN_POINT('Ctrl Pts',(-75.7071707703566,13.6215936347519,-13.1892081062607));
#41876=CARTESIAN_POINT('Ctrl Pts',(-75.6937744661824,13.6061651387076,-14.4733910901186));
#41877=CARTESIAN_POINT('Ctrl Pts',(-75.6670757378233,13.5780267593918,-15.6009938779762));
#41878=CARTESIAN_POINT('Ctrl Pts',(-75.6527894765495,13.562799510879,-16.3435925262125));
#41879=CARTESIAN_POINT('Ctrl Pts',(-75.6448300448953,13.5542712485532,-16.8363372080636));
#41880=CARTESIAN_POINT('Ctrl Pts',(-75.641343095406,13.5504597280976,-17.2035568900481));
#41881=CARTESIAN_POINT('Ctrl Pts',(-75.6405970526558,13.5495515514651,-17.5079024946932));
#41882=CARTESIAN_POINT('Ctrl Pts',(-75.6403086742588,13.5492098226299,-17.6332552488187));
#41883=CARTESIAN_POINT('Ctrl Pts',(-75.6397615638604,13.5485941867171,-17.881274919397));
#41884=CARTESIAN_POINT('Ctrl Pts',(-75.6392583532568,13.5480779667676,-18.1305314212828));
#41885=CARTESIAN_POINT('Ctrl Pts',(-75.6387937274463,13.5476482161608,-18.379407794415));
#41886=CARTESIAN_POINT('Ctrl Pts',(-75.6385194129121,13.5474146201461,-18.5351594934329));
#41887=CARTESIAN_POINT('Ctrl Pts',(-75.6383088963852,13.5472471341751,-18.659758006526));
#41888=CARTESIAN_POINT('Ctrl Pts',(-75.6381554906238,13.5471310613474,-18.7532425003298));
#41889=CARTESIAN_POINT('Ctrl Pts',(-75.638031303301,13.5470420138082,-18.8311610906567));
#41890=CARTESIAN_POINT('Ctrl Pts',(-75.6379340475833,13.5469752106932,-18.8935087206951));
#41891=CARTESIAN_POINT('Ctrl Pts',(-75.6371195986504,13.5464324576899,-19.4235310655964));
#41892=CARTESIAN_POINT('Ctrl Pts',(-75.6359439274737,13.5461618762464,-20.4390743303277));
#41893=CARTESIAN_POINT('Ctrl Pts',(-75.634864971159,13.5467473242472,-21.9453895012519));
#41894=CARTESIAN_POINT('Ctrl Pts',(-75.6343245502054,13.5469551304571,-22.9544210717622));
#41895=CARTESIAN_POINT('Ctrl Pts',(-75.6339553824512,13.5467702978225,-23.584833399548));
#41896=CARTESIAN_POINT('Ctrl Pts',(-75.6338241245163,13.5467000977553,-23.8339615872695));
#41897=CARTESIAN_POINT('Ctrl Pts',(-75.6336169104993,13.5465709414473,-24.3332354712502));
#41898=CARTESIAN_POINT('Ctrl Pts',(-75.633385180036,13.5463734807082,-25.2086755739493));
#41899=CARTESIAN_POINT('Ctrl Pts',(-75.6333480779871,13.5461804995033,-26.4634304778581));
#41900=CARTESIAN_POINT('Ctrl Pts',(-75.6335152876745,13.5460910742537,-27.9716539612101));
#41901=CARTESIAN_POINT('Ctrl Pts',(-75.6335968855616,13.5461354282596,-28.9763368670655));
#41902=CARTESIAN_POINT('Ctrl Pts',(-75.6335855550659,13.5461879021644,-29.5404783410885));
#41903=CARTESIAN_POINT('Ctrl Pts',(-75.6335806332078,13.5462007412436,-29.6658174535336));
#41904=CARTESIAN_POINT('Ctrl Pts',(-75.633562342921,13.5462316844819,-29.916569276828));
#41905=CARTESIAN_POINT('Ctrl Pts',(-75.6335106440104,13.546299471024,-30.3555335376507));
#41906=CARTESIAN_POINT('Ctrl Pts',(-75.6333487173523,13.5464831048139,-31.2339430110599));
#41907=CARTESIAN_POINT('Ctrl Pts',(-75.6330652885746,13.5468592114955,-32.4894754032597));
#41908=CARTESIAN_POINT('Ctrl Pts',(-75.6330206994714,13.5473116404508,-33.743958832858));
#41909=CARTESIAN_POINT('Ctrl Pts',(-75.633313476897,13.5476727368069,-34.745746801062));
#41910=CARTESIAN_POINT('Ctrl Pts',(-75.6336001558874,13.5478488490821,-35.245866546638));
#41911=CARTESIAN_POINT('Ctrl Pts',(-75.6338801375847,13.5479750387175,-35.6215898145587));
#41912=CARTESIAN_POINT('Ctrl Pts',(-75.6340982843881,13.5480410686006,-35.8734477474361));
#41913=CARTESIAN_POINT('Ctrl Pts',(-75.6346422595824,13.5481116777071,-36.3762829408899));
#41914=CARTESIAN_POINT('Ctrl Pts',(-75.6358387140055,13.5481207949868,-37.2546696620858));
#41915=CARTESIAN_POINT('Ctrl Pts',(-75.6389085318736,13.5479548706782,-39.0064589406112));
#41916=CARTESIAN_POINT('Ctrl Pts',(-75.6416606556734,13.5485909875611,-40.5064448190074));
#41917=CARTESIAN_POINT('Ctrl Pts',(-75.6428684946547,13.5506879531502,-41.7609185403146));
#41918=CARTESIAN_POINT('Ctrl Pts',(-75.6431384271574,13.5508353275622,-42.1394337958565));
#41919=CARTESIAN_POINT('Ctrl Pts',(-75.6433691289682,13.5504705830997,-42.6417451415882));
#41920=CARTESIAN_POINT('Ctrl Pts',(-75.6435296071986,13.5498727505972,-43.1442881511953));
#41921=CARTESIAN_POINT('Ctrl Pts',(-75.6436299000572,13.5489391994608,-43.7715483625547));
#41922=CARTESIAN_POINT('Ctrl Pts',(-75.6436894358512,13.5483311083971,-44.5227694286739));
#41923=CARTESIAN_POINT('Ctrl Pts',(-75.6437723235048,13.5489197957315,-45.146946138206));
#41924=CARTESIAN_POINT('Ctrl Pts',(-75.6439101440714,13.5504390634564,-45.6449865082951));
#41925=CARTESIAN_POINT('Ctrl Pts',(-75.6440617719633,13.5522043159601,-46.0177699219705));
#41926=CARTESIAN_POINT('Ctrl Pts',(-75.6442744865655,13.5546938354661,-46.389772918041));
#41927=CARTESIAN_POINT('Ctrl Pts',(-75.6446573797619,13.559104895256,-46.8845694663249));
#41928=CARTESIAN_POINT('Ctrl Pts',(-75.6450739944625,13.5638006721358,-47.2543918244836));
#41929=CARTESIAN_POINT('Ctrl Pts',(-75.6456069604917,13.5696097310337,-47.6236166737643));
#41930=CARTESIAN_POINT('Ctrl Pts',(-75.6460176039176,13.5746544762556,-47.8579539210514));
#41931=CARTESIAN_POINT('Ctrl Pts',(-75.6468926688973,13.5895854830564,-48.3395044348218));
#41932=CARTESIAN_POINT('Ctrl Pts',(-75.6485797019952,13.6258983739338,-49.1907272539963));
#41933=CARTESIAN_POINT('Ctrl Pts',(-75.6511923920832,13.6947642150988,-50.4451004143629));
#41934=CARTESIAN_POINT('Ctrl Pts',(-75.6546407320632,13.7603715617149,-52.0049430108417));
#41935=CARTESIAN_POINT('Ctrl Pts',(-75.6576093036443,13.7599216629611,-53.0825950363202));
#41936=CARTESIAN_POINT('Ctrl Pts',(-75.6600038773525,13.7342295213886,-53.7702081331066));
#41937=CARTESIAN_POINT('Ctrl Pts',(-75.6612950918065,13.7172632093226,-54.075784837558));
#41938=CARTESIAN_POINT('Ctrl Pts',(-75.6642262716333,13.6662448593001,-54.6543512556725));
#41939=CARTESIAN_POINT('Ctrl Pts',(-75.6698408369108,13.5417335232503,-55.6365742588973));
#41940=CARTESIAN_POINT('Ctrl Pts',(-75.6803639426854,13.2231870482516,-57.4447436616881));
#41941=CARTESIAN_POINT('Ctrl Pts',(-75.681282064688,13.059670403835,-58.7321430875395));
#41942=CARTESIAN_POINT('Ctrl Pts',(-75.6863956938303,13.1064525118599,-59.4965891093409));
#41943=CARTESIAN_POINT('Ctrl Pts',(-75.6868679897915,13.1140146369142,-59.6098969334171));
#41944=CARTESIAN_POINT('Ctrl Pts',(-75.6879149993631,13.1316083652691,-59.8259666891569));
#41945=CARTESIAN_POINT('Ctrl Pts',(-75.6897345617221,13.1707110281061,-60.2119348572073));
#41946=CARTESIAN_POINT('Ctrl Pts',(-75.6934742771951,13.2796876085821,-60.9876632047891));
#41947=CARTESIAN_POINT('Ctrl Pts',(-75.6976408619348,13.4705431429276,-61.8928361581727));
#41948=CARTESIAN_POINT('Ctrl Pts',(-75.701444272716,13.7166853950894,-62.8074689649149));
#41949=CARTESIAN_POINT('Ctrl Pts',(-75.7034366519234,13.873544319781,-63.3250195269508));
#41950=CARTESIAN_POINT('Ctrl Pts',(-75.7047012154514,13.9848001926648,-63.6707047148809));
#41951=CARTESIAN_POINT('Ctrl Pts',(-75.7055274561093,14.0606850141304,-63.9013523952973));
#41952=CARTESIAN_POINT('Ctrl Pts',(-75.7063332430143,14.1390069406578,-64.1320979910642));
#41953=CARTESIAN_POINT('Ctrl Pts',(-75.707016474211,14.2095241235918,-64.3341505038452));
#41954=CARTESIAN_POINT('Ctrl Pts',(-75.7074011288797,14.2503585013626,-64.4496309575972));
#41955=CARTESIAN_POINT('Ctrl Pts',(-75.7079739620691,14.3121249045545,-64.6228414340704));
#41956=CARTESIAN_POINT('Ctrl Pts',(-75.708438040624,14.3646763995539,-64.7672340258762));
#41957=CARTESIAN_POINT('Ctrl Pts',(-75.7092266721553,14.4527116415818,-65.005635688223));
#41958=CARTESIAN_POINT('Ctrl Pts',(-75.7117667830696,14.5355526360062,-65.2185617805244));
#41959=CARTESIAN_POINT('Ctrl Pts',(-75.7156454045534,14.724818485127,-65.668561251195));
#41960=CARTESIAN_POINT('Ctrl Pts',(-75.7221741072873,15.0933070411488,-66.4580654331261));
#41961=CARTESIAN_POINT('Ctrl Pts',(-75.7305427718633,15.9734396090043,-68.0970327921023));
#41962=CARTESIAN_POINT('Ctrl Pts',(-75.7285600851967,16.8715705729392,-69.5915485739548));
#41963=CARTESIAN_POINT('Ctrl Pts',(-75.7231320655152,17.5030633452021,-70.793001962088));
#41964=CARTESIAN_POINT('Ctrl Pts',(-75.7236077231866,17.6319482655893,-71.0375549507293));
#41965=CARTESIAN_POINT('Ctrl Pts',(-75.7235722165254,17.8972962896899,-71.540070471556));
#41966=CARTESIAN_POINT('Ctrl Pts',(-75.7238930232004,18.2272929043099,-72.1628002331602));
#41967=CARTESIAN_POINT('Ctrl Pts',(-75.7240075301994,18.6263425104643,-72.9134849283308));
#41968=CARTESIAN_POINT('Ctrl Pts',(-75.7242605650699,19.4258466085276,-74.4139719006252));
#41969=CARTESIAN_POINT('Ctrl Pts',(-75.7242247109526,20.0957347727082,-75.6668117968037));
#41970=CARTESIAN_POINT('Ctrl Pts',(-75.7239597457827,21.0674494694115,-77.4942025512152));
#41971=CARTESIAN_POINT('Ctrl Pts',(-75.7240750175091,21.5031493372222,-78.3134974540841));
#41972=CARTESIAN_POINT('Ctrl Pts',(-75.7240750175066,21.939670924612,-79.1344751561986));
#41973=CARTESIAN_POINT('Ctrl Pts',(-72.8865680674535,8.26575232185009,24.8276912522435));
#41974=CARTESIAN_POINT('Ctrl Pts',(-72.8869414421383,8.26573286341148,24.7787178932437));
#41975=CARTESIAN_POINT('Ctrl Pts',(-72.8873327680767,8.26571236274712,24.729744826743));
#41976=CARTESIAN_POINT('Ctrl Pts',(-72.8919550651354,8.26547621202624,24.1779986734955));
#41977=CARTESIAN_POINT('Ctrl Pts',(-72.8989341377874,8.26453602047102,23.1728399881855));
#41978=CARTESIAN_POINT('Ctrl Pts',(-72.9174048097993,8.26169786168248,21.1618965904426));
#41979=CARTESIAN_POINT('Ctrl Pts',(-72.9481006229035,8.25999530162877,19.6554113963992));
#41980=CARTESIAN_POINT('Ctrl Pts',(-72.9959818140564,8.26039309449099,18.4026337347238));
#41981=CARTESIAN_POINT('Ctrl Pts',(-73.0210030137968,8.25960530135002,17.8902665411261));
#41982=CARTESIAN_POINT('Ctrl Pts',(-73.0875426278879,8.25565539996311,16.8799446059181));
#41983=CARTESIAN_POINT('Ctrl Pts',(-73.229943398351,8.24611163285477,15.1296376299366));
#41984=CARTESIAN_POINT('Ctrl Pts',(-73.3374512605349,8.24874818684716,13.6575521217196));
#41985=CARTESIAN_POINT('Ctrl Pts',(-73.3533279432813,8.27501923579358,12.439741783186));
#41986=CARTESIAN_POINT('Ctrl Pts',(-73.3567837062602,8.28502742178981,11.9323235896795));
#41987=CARTESIAN_POINT('Ctrl Pts',(-73.3521445253704,8.3043377425253,10.9376815727366));
#41988=CARTESIAN_POINT('Ctrl Pts',(-73.3246186828076,8.3312814040697,9.70190084284496));
#41989=CARTESIAN_POINT('Ctrl Pts',(-73.2567457688751,8.37994614453916,8.2446764166352));
#41990=CARTESIAN_POINT('Ctrl Pts',(-73.1890088003569,8.43111706791072,7.28737224708644));
#41991=CARTESIAN_POINT('Ctrl Pts',(-73.1399135755569,8.47187327739597,6.69378252491712));
#41992=CARTESIAN_POINT('Ctrl Pts',(-73.1173392770425,8.48995716105188,6.43996597869799));
#41993=CARTESIAN_POINT('Ctrl Pts',(-73.0652853571013,8.52137581014927,5.94571821208205));
#41994=CARTESIAN_POINT('Ctrl Pts',(-72.9585437937225,8.5706759054832,5.08330708674856));
#41995=CARTESIAN_POINT('Ctrl Pts',(-72.710409440949,8.65655741011438,3.39659394490956));
#41996=CARTESIAN_POINT('Ctrl Pts',(-72.5373531107517,8.79271546662842,1.99110235750803));
#41997=CARTESIAN_POINT('Ctrl Pts',(-72.486130774036,9.02060243584483,1.02407232192719));
#41998=CARTESIAN_POINT('Ctrl Pts',(-72.4814597395665,9.0467585181321,0.919658573672963));
#41999=CARTESIAN_POINT('Ctrl Pts',(-72.4717982353608,9.10540038958677,0.7018507216913));
#42000=CARTESIAN_POINT('Ctrl Pts',(-72.4561006574169,9.22010108007979,0.317554629446909));
#42001=CARTESIAN_POINT('Ctrl Pts',(-72.434475200519,9.41780924635723,-0.250230368461771));
#42002=CARTESIAN_POINT('Ctrl Pts',(-72.4071883371743,9.69723158663515,-0.954375802733552));
#42003=CARTESIAN_POINT('Ctrl Pts',(-72.3679637323457,10.1098687883021,-1.92235452420412));
#42004=CARTESIAN_POINT('Ctrl Pts',(-72.315204166524,10.6685800030012,-3.18449761246109));
#42005=CARTESIAN_POINT('Ctrl Pts',(-72.2846125510446,11.095248182418,-4.26272411289597));
#42006=CARTESIAN_POINT('Ctrl Pts',(-72.277107189919,11.3322228678791,-4.96422958465152));
#42007=CARTESIAN_POINT('Ctrl Pts',(-72.2820261073132,11.4180006409522,-5.20171825302269));
#42008=CARTESIAN_POINT('Ctrl Pts',(-72.2959241019649,11.5997573778334,-5.70456172189619));
#42009=CARTESIAN_POINT('Ctrl Pts',(-72.3402000381889,11.9221019350025,-6.58073860490952));
#42010=CARTESIAN_POINT('Ctrl Pts',(-72.4485572929506,12.3824063008201,-7.87143171517512));
#42011=CARTESIAN_POINT('Ctrl Pts',(-72.5868739232216,12.7734181938476,-9.21275087736498));
#42012=CARTESIAN_POINT('Ctrl Pts',(-72.6695584917179,12.9827799224197,-10.180743840257));
#42013=CARTESIAN_POINT('Ctrl Pts',(-72.7080669955866,13.0813270808735,-10.7403067660567));
#42014=CARTESIAN_POINT('Ctrl Pts',(-72.7236469770478,13.1231949475135,-11.022237072098));
#42015=CARTESIAN_POINT('Ctrl Pts',(-72.7337116967939,13.1518582962864,-11.2354778521101));
#42016=CARTESIAN_POINT('Ctrl Pts',(-72.7400437346278,13.1708727140572,-11.3844506421277));
#42017=CARTESIAN_POINT('Ctrl Pts',(-72.75183445656,13.203182773435,-11.6768142474498));
#42018=CARTESIAN_POINT('Ctrl Pts',(-72.7698806280746,13.2475047047871,-12.1844701611177));
#42019=CARTESIAN_POINT('Ctrl Pts',(-72.7963087796921,13.2920790566331,-13.175224571561));
#42020=CARTESIAN_POINT('Ctrl Pts',(-72.810913539449,13.266201707407,-14.5238487361184));
#42021=CARTESIAN_POINT('Ctrl Pts',(-72.8100289523327,13.2060455556474,-15.6607798739506));
#42022=CARTESIAN_POINT('Ctrl Pts',(-72.8095164431849,13.1755895645277,-16.3891086797765));
#42023=CARTESIAN_POINT('Ctrl Pts',(-72.8096395484204,13.1592459050039,-16.8669798526424));
#42024=CARTESIAN_POINT('Ctrl Pts',(-72.8107379701226,13.1531058507421,-17.2167843215973));
#42025=CARTESIAN_POINT('Ctrl Pts',(-72.8127847793528,13.1530562057521,-17.5037849767314));
#42026=CARTESIAN_POINT('Ctrl Pts',(-72.8135450880309,13.1529895968429,-17.631465345179));
#42027=CARTESIAN_POINT('Ctrl Pts',(-72.8148441009318,13.1528746224633,-17.8787508000146));
#42028=CARTESIAN_POINT('Ctrl Pts',(-72.815834791024,13.1527349638102,-18.1292304775296));
#42029=CARTESIAN_POINT('Ctrl Pts',(-72.8165477639545,13.152592856749,-18.3782516548426));
#42030=CARTESIAN_POINT('Ctrl Pts',(-72.8168850950152,13.1524983325586,-18.5343165379471));
#42031=CARTESIAN_POINT('Ctrl Pts',(-72.8170938851606,13.1524214947919,-18.6590680081469));
#42032=CARTESIAN_POINT('Ctrl Pts',(-72.8172210419957,13.1523626742158,-18.7526857093762));
#42033=CARTESIAN_POINT('Ctrl Pts',(-72.8173033240809,13.1523128478981,-18.8307023222607));
#42034=CARTESIAN_POINT('Ctrl Pts',(-72.8173554323772,13.1522726266496,-18.8931289934987));
#42035=CARTESIAN_POINT('Ctrl Pts',(-72.8177222997263,13.151927576941,-19.4238049830459));
#42036=CARTESIAN_POINT('Ctrl Pts',(-72.8160783882301,13.1511531583128,-20.4402734819812));
#42037=CARTESIAN_POINT('Ctrl Pts',(-72.8111063553451,13.1500545858526,-21.9467249018876));
#42038=CARTESIAN_POINT('Ctrl Pts',(-72.8089203623372,13.1494766711097,-22.9551277264119));
#42039=CARTESIAN_POINT('Ctrl Pts',(-72.8087826744896,13.1492380882382,-23.5849128827914));
#42040=CARTESIAN_POINT('Ctrl Pts',(-72.8087463021177,13.1491493109577,-23.8341081872102));
#42041=CARTESIAN_POINT('Ctrl Pts',(-72.8087378441687,13.148986603098,-24.333334836021));
#42042=CARTESIAN_POINT('Ctrl Pts',(-72.8088675228599,13.1487395044348,-25.2087791315747));
#42043=CARTESIAN_POINT('Ctrl Pts',(-72.809320336019,13.1484986769883,-26.4634752931833));
#42044=CARTESIAN_POINT('Ctrl Pts',(-72.8098331928483,13.1483899012864,-27.9716152992162));
#42045=CARTESIAN_POINT('Ctrl Pts',(-72.8098480232188,13.1484405227099,-28.976217642425));
#42046=CARTESIAN_POINT('Ctrl Pts',(-72.8096797178121,13.1485023055856,-29.5403032171419));
#42047=CARTESIAN_POINT('Ctrl Pts',(-72.8096343913625,13.1485177135259,-29.6656190121026));
#42048=CARTESIAN_POINT('Ctrl Pts',(-72.8095143066656,13.1485545150383,-29.9163326943316));
#42049=CARTESIAN_POINT('Ctrl Pts',(-72.8092326749967,13.1486349098195,-30.3552337608238));
#42050=CARTESIAN_POINT('Ctrl Pts',(-72.8084334077922,13.1488518912644,-31.2335434893697));
#42051=CARTESIAN_POINT('Ctrl Pts',(-72.8068941888047,13.1492995404523,-32.489001190465));
#42052=CARTESIAN_POINT('Ctrl Pts',(-72.8055717125501,13.1498467714524,-33.7435017093954));
#42053=CARTESIAN_POINT('Ctrl Pts',(-72.8050922656081,13.1502919622503,-34.7453540357136));
#42054=CARTESIAN_POINT('Ctrl Pts',(-72.8051181249078,13.1505133837545,-35.2455261813069));
#42055=CARTESIAN_POINT('Ctrl Pts',(-72.8052663797821,13.1506736703081,-35.6212940420671));
#42056=CARTESIAN_POINT('Ctrl Pts',(-72.8054103276837,13.1507642395526,-35.8731501737671));
#42057=CARTESIAN_POINT('Ctrl Pts',(-72.8058573239597,13.1508887209446,-36.3759995572946));
#42058=CARTESIAN_POINT('Ctrl Pts',(-72.8070018602344,13.1510064726944,-37.2544049579662));
#42059=CARTESIAN_POINT('Ctrl Pts',(-72.8103329337767,13.151083984824,-39.0062374472486));
#42060=CARTESIAN_POINT('Ctrl Pts',(-72.8135288102678,13.1519316475286,-40.5062668572796));
#42061=CARTESIAN_POINT('Ctrl Pts',(-72.8147940400713,13.1541324879213,-41.7607748435403));
#42062=CARTESIAN_POINT('Ctrl Pts',(-72.8150508433956,13.1543051922145,-42.139293505977));
#42063=CARTESIAN_POINT('Ctrl Pts',(-72.8152250149216,13.1539653770489,-42.6416139194372));
#42064=CARTESIAN_POINT('Ctrl Pts',(-72.8153098594775,13.1533881732182,-43.1441664804877));
#42065=CARTESIAN_POINT('Ctrl Pts',(-72.8152935731392,13.1524735165275,-43.7714412043856));
#42066=CARTESIAN_POINT('Ctrl Pts',(-72.8152214340072,13.1518824373665,-44.5226834273021));
#42067=CARTESIAN_POINT('Ctrl Pts',(-72.8152377100189,13.1524849569531,-45.146881417179));
#42068=CARTESIAN_POINT('Ctrl Pts',(-72.8153700975781,13.1540170297017,-45.6449400484013));
#42069=CARTESIAN_POINT('Ctrl Pts',(-72.8155469327632,13.1557937148195,-46.0177382696206));
#42070=CARTESIAN_POINT('Ctrl Pts',(-72.8158196149017,13.1582970756863,-46.3897570995508));
#42071=CARTESIAN_POINT('Ctrl Pts',(-72.8163359950318,13.1627306891508,-46.8845758998427));
#42072=CARTESIAN_POINT('Ctrl Pts',(-72.8169213641905,13.1674489540909,-47.2544170165257));
#42073=CARTESIAN_POINT('Ctrl Pts',(-72.8176800146892,13.1732856641719,-47.6236613330653));
#42074=CARTESIAN_POINT('Ctrl Pts',(-72.8182543664395,13.1783499070941,-47.8580189203204));
#42075=CARTESIAN_POINT('Ctrl Pts',(-72.8195030698015,13.1933212767559,-48.3396013453518));
#42076=CARTESIAN_POINT('Ctrl Pts',(-72.8219596249252,13.229709474452,-49.1908719162654));
#42077=CARTESIAN_POINT('Ctrl Pts',(-72.8259700723709,13.2986915340731,-50.4452830186504));
#42078=CARTESIAN_POINT('Ctrl Pts',(-72.8314710092657,13.3644612971796,-52.0051294364399));
#42079=CARTESIAN_POINT('Ctrl Pts',(-72.8359995992376,13.364139636692,-53.0827593739283));
#42080=CARTESIAN_POINT('Ctrl Pts',(-72.8394107859471,13.3385396684649,-53.7703518384481));
#42081=CARTESIAN_POINT('Ctrl Pts',(-72.8411415506986,13.3216111243518,-54.0759351268447));
#42082=CARTESIAN_POINT('Ctrl Pts',(-72.8450429256167,13.2706795792392,-54.6545057657787));
#42083=CARTESIAN_POINT('Ctrl Pts',(-72.852555674139,13.1463416430414,-55.6367389748052));
#42084=CARTESIAN_POINT('Ctrl Pts',(-72.8673335059477,12.8281990268769,-57.4449208146386));
#42085=CARTESIAN_POINT('Ctrl Pts',(-72.8716432703236,12.6650429159702,-58.7322956460207));
#42086=CARTESIAN_POINT('Ctrl Pts',(-72.8780587972058,12.7119721350998,-59.4966749041411));
#42087=CARTESIAN_POINT('Ctrl Pts',(-72.8786824357828,12.719550818378,-59.6099750270973));
#42088=CARTESIAN_POINT('Ctrl Pts',(-72.8800079592648,12.7371757831492,-59.8260300265551));
#42089=CARTESIAN_POINT('Ctrl Pts',(-72.8822536109264,12.7763270405229,-60.2119744961277));
#42090=CARTESIAN_POINT('Ctrl Pts',(-72.8866228266663,12.8853804043739,-60.9876644881528));
#42091=CARTESIAN_POINT('Ctrl Pts',(-72.8911029626343,13.0762882899736,-61.8928156844469));
#42092=CARTESIAN_POINT('Ctrl Pts',(-72.8950199421075,13.3224683876046,-62.8074470955451));
#42093=CARTESIAN_POINT('Ctrl Pts',(-72.8970393317336,13.4793462452144,-63.3250036462584));
#42094=CARTESIAN_POINT('Ctrl Pts',(-72.8983224238168,13.5906149021888,-63.6706953025752));
#42095=CARTESIAN_POINT('Ctrl Pts',(-72.8991621720125,13.6665083868823,-63.9013479527401));
#42096=CARTESIAN_POINT('Ctrl Pts',(-72.8999848651695,13.7448392040268,-64.1320994034226));
#42097=CARTESIAN_POINT('Ctrl Pts',(-72.9006885231233,13.8153646331157,-64.3341578281979));
#42098=CARTESIAN_POINT('Ctrl Pts',(-72.9010868611603,13.8562038708251,-64.4496418724454));
#42099=CARTESIAN_POINT('Ctrl Pts',(-72.901682426375,13.9179777271408,-64.6228579385507));
#42100=CARTESIAN_POINT('Ctrl Pts',(-72.902170464986,13.9705357796231,-64.7672556263047));
#42101=CARTESIAN_POINT('Ctrl Pts',(-72.9030076305139,14.0585824816158,-65.0056661064065));
#42102=CARTESIAN_POINT('Ctrl Pts',(-72.9055969738179,14.1414324975294,-65.2185926643699));
#42103=CARTESIAN_POINT('Ctrl Pts',(-72.9095482917182,14.3307137143814,-65.6685970674762));
#42104=CARTESIAN_POINT('Ctrl Pts',(-72.9161514089217,14.6992194686521,-66.4581056413799));
#42105=CARTESIAN_POINT('Ctrl Pts',(-72.9244946737035,15.579356371815,-68.097078216371));
#42106=CARTESIAN_POINT('Ctrl Pts',(-72.9223549274365,16.4774628368235,-69.5915927640089));
#42107=CARTESIAN_POINT('Ctrl Pts',(-72.9169103750747,17.1089503039591,-70.7930434498888));
#42108=CARTESIAN_POINT('Ctrl Pts',(-72.9173870473759,17.237835907039,-71.0375968471999));
#42109=CARTESIAN_POINT('Ctrl Pts',(-72.9173509939031,17.5031841378782,-71.5401125637486));
#42110=CARTESIAN_POINT('Ctrl Pts',(-72.917672410201,17.8331812855221,-72.1628427052565));
#42111=CARTESIAN_POINT('Ctrl Pts',(-72.9177872026895,18.2322311103456,-72.9135276335728));
#42112=CARTESIAN_POINT('Ctrl Pts',(-72.9180413274558,19.0317354550891,-74.4140149336155));
#42113=CARTESIAN_POINT('Ctrl Pts',(-72.9180063208637,19.70162313999,-75.6668545626666));
#42114=CARTESIAN_POINT('Ctrl Pts',(-72.917740703414,20.6733372941337,-77.4942447409276));
#42115=CARTESIAN_POINT('Ctrl Pts',(-72.917856315526,21.1090373153559,-78.3135397879966));
#42116=CARTESIAN_POINT('Ctrl Pts',(-72.9178563155317,21.5455589027462,-79.1345174901012));
#42117=CARTESIAN_POINT('Ctrl Pts',(-70.0797300922936,7.87083409769097,24.8336095804827));
#42118=CARTESIAN_POINT('Ctrl Pts',(-70.0799646667605,7.87093845762237,24.7848236666139));
#42119=CARTESIAN_POINT('Ctrl Pts',(-70.0802106206726,7.87104776413738,24.7360406870304));
#42120=CARTESIAN_POINT('Ctrl Pts',(-70.0831162832123,7.87233944489162,24.1865206508717));
#42121=CARTESIAN_POINT('Ctrl Pts',(-70.0856956491753,7.87502546693778,23.1838837033978));
#42122=CARTESIAN_POINT('Ctrl Pts',(-70.0918978853719,7.88239184231991,21.1771390793342));
#42123=CARTESIAN_POINT('Ctrl Pts',(-70.1112127705556,7.89097251402827,19.672722175038));
#42124=CARTESIAN_POINT('Ctrl Pts',(-70.1504440078457,7.90066506163222,18.4211235716628));
#42125=CARTESIAN_POINT('Ctrl Pts',(-70.1697003096978,7.90590967768963,17.9236165225639));
#42126=CARTESIAN_POINT('Ctrl Pts',(-70.2188717945085,7.92010557264673,16.9233332269309));
#42127=CARTESIAN_POINT('Ctrl Pts',(-70.3245072267018,7.95020258260261,15.1692690929129));
#42128=CARTESIAN_POINT('Ctrl Pts',(-70.4196449338281,7.96904497304481,13.6495592012489));
#42129=CARTESIAN_POINT('Ctrl Pts',(-70.4695606398365,7.96298537878605,12.3710022159992));
#42130=CARTESIAN_POINT('Ctrl Pts',(-70.490216149405,7.95733326394079,11.8533220878073));
#42131=CARTESIAN_POINT('Ctrl Pts',(-70.53210178241,7.93718721593872,10.8325501005278));
#42132=CARTESIAN_POINT('Ctrl Pts',(-70.5812230449941,7.90165812831565,9.57061253256148));
#42133=CARTESIAN_POINT('Ctrl Pts',(-70.6213518385245,7.86263523571733,8.08298723669083));
#42134=CARTESIAN_POINT('Ctrl Pts',(-70.6263413494506,7.85051196817903,7.10760374122982));
#42135=CARTESIAN_POINT('Ctrl Pts',(-70.6199133696501,7.85046321124629,6.50252850665239));
#42136=CARTESIAN_POINT('Ctrl Pts',(-70.6171502217435,7.84849425242508,6.22778268160475));
#42137=CARTESIAN_POINT('Ctrl Pts',(-70.6099046660388,7.83921247672353,5.7061450396773));
#42138=CARTESIAN_POINT('Ctrl Pts',(-70.5921107527037,7.81304674889243,4.80420574951403));
#42139=CARTESIAN_POINT('Ctrl Pts',(-70.5320835521922,7.75566715378061,3.09229665864847));
#42140=CARTESIAN_POINT('Ctrl Pts',(-70.425694019437,7.78731605055769,1.78224082503292));
#42141=CARTESIAN_POINT('Ctrl Pts',(-70.3395780432339,7.91047947804615,0.920418189731267));
#42142=CARTESIAN_POINT('Ctrl Pts',(-70.3281862757546,7.9265152414774,0.81546603095744));
#42143=CARTESIAN_POINT('Ctrl Pts',(-70.3034672863993,7.96089874100147,0.604597509478728));
#42144=CARTESIAN_POINT('Ctrl Pts',(-70.254815071026,8.02834317441377,0.229801605440034));
#42145=CARTESIAN_POINT('Ctrl Pts',(-70.1738770417327,8.14462932123709,-0.32043261565958));
#42146=CARTESIAN_POINT('Ctrl Pts',(-70.0675190259357,8.31623264682582,-1.005864139264));
#42147=CARTESIAN_POINT('Ctrl Pts',(-69.9234752204677,8.58551139528495,-1.94994725910126));
#42148=CARTESIAN_POINT('Ctrl Pts',(-69.7537363853315,8.99303427045749,-3.18139531531514));
#42149=CARTESIAN_POINT('Ctrl Pts',(-69.6555765300377,9.37167205002254,-4.2050076167861));
#42150=CARTESIAN_POINT('Ctrl Pts',(-69.6175750115734,9.61674332323064,-4.8518866619604));
#42151=CARTESIAN_POINT('Ctrl Pts',(-69.614996384641,9.70391730270588,-5.05492488932629));
#42152=CARTESIAN_POINT('Ctrl Pts',(-69.6082938426236,9.91073799703179,-5.50489344233537));
#42153=CARTESIAN_POINT('Ctrl Pts',(-69.6106257681355,10.318486485829,-6.30250377295544));
#42154=CARTESIAN_POINT('Ctrl Pts',(-69.634414507676,11.0005103287512,-7.52679652658411));
#42155=CARTESIAN_POINT('Ctrl Pts',(-69.6766863625143,11.6866796254722,-8.85991637902529));
#42156=CARTESIAN_POINT('Ctrl Pts',(-69.7071716493671,12.0968998297548,-9.87706752674961));
#42157=CARTESIAN_POINT('Ctrl Pts',(-69.722762042575,12.2973318855679,-10.4847897843783));
#42158=CARTESIAN_POINT('Ctrl Pts',(-69.7294646151064,12.3838364503264,-10.7982059734627));
#42159=CARTESIAN_POINT('Ctrl Pts',(-69.7339098166316,12.4427321913131,-11.0376746143682));
#42160=CARTESIAN_POINT('Ctrl Pts',(-69.7373366428525,12.4792362201273,-11.191032336319));
#42161=CARTESIAN_POINT('Ctrl Pts',(-69.7451836481932,12.5453552435596,-11.4998982538861));
#42162=CARTESIAN_POINT('Ctrl Pts',(-69.7614512775317,12.641968099703,-12.0328224750319));
#42163=CARTESIAN_POINT('Ctrl Pts',(-69.8018292172795,12.767713728289,-13.0749517757829));
#42164=CARTESIAN_POINT('Ctrl Pts',(-69.8692804996059,12.8027391307006,-14.4766171192183));
#42165=CARTESIAN_POINT('Ctrl Pts',(-69.9236037530677,12.7681274810262,-15.6326832106271));
#42166=CARTESIAN_POINT('Ctrl Pts',(-69.9528293609611,12.7525926142196,-16.3621025680776));
#42167=CARTESIAN_POINT('Ctrl Pts',(-69.9702257048737,12.7458542468064,-16.8377075153323));
#42168=CARTESIAN_POINT('Ctrl Pts',(-69.9806833299977,12.7469682670916,-17.1822224171611));
#42169=CARTESIAN_POINT('Ctrl Pts',(-69.9876533243847,12.7532730120962,-17.4633727546574));
#42170=CARTESIAN_POINT('Ctrl Pts',(-69.9901878041358,12.7559302447579,-17.5957832338958));
#42171=CARTESIAN_POINT('Ctrl Pts',(-69.9946058127628,12.7604059255415,-17.8480854166894));
#42172=CARTESIAN_POINT('Ctrl Pts',(-69.9980492085591,12.7640263564037,-18.1046796823426));
#42173=CARTESIAN_POINT('Ctrl Pts',(-70.0006278395402,12.7667954845501,-18.3585667860185));
#42174=CARTESIAN_POINT('Ctrl Pts',(-70.0018985491503,12.7682120625135,-18.5176708497133));
#42175=CARTESIAN_POINT('Ctrl Pts',(-70.0027234975775,12.7691626491919,-18.6446737562696));
#42176=CARTESIAN_POINT('Ctrl Pts',(-70.0032495291657,12.7697890061634,-18.7399419573746));
#42177=CARTESIAN_POINT('Ctrl Pts',(-70.0036134451858,12.7702402913664,-18.8192804051432));
#42178=CARTESIAN_POINT('Ctrl Pts',(-70.0038613073673,12.7705610527564,-18.8827386925231));
#42179=CARTESIAN_POINT('Ctrl Pts',(-70.0057291557627,12.7730591465881,-19.4220221149389));
#42180=CARTESIAN_POINT('Ctrl Pts',(-70.0018986583592,12.770776648951,-20.4500653832152));
#42181=CARTESIAN_POINT('Ctrl Pts',(-69.9879997992902,12.7594571042562,-21.9592664440623));
#42182=CARTESIAN_POINT('Ctrl Pts',(-69.981963518983,12.7544602708346,-22.960197688122));
#42183=CARTESIAN_POINT('Ctrl Pts',(-69.9818921980815,12.7546653219054,-23.5825699741119));
#42184=CARTESIAN_POINT('Ctrl Pts',(-69.981894991941,12.7547519566139,-23.8326565024476));
#42185=CARTESIAN_POINT('Ctrl Pts',(-69.9820122597349,12.7549340746958,-24.3315249118144));
#42186=CARTESIAN_POINT('Ctrl Pts',(-69.9824658818906,12.7552624643131,-25.2074809115996));
#42187=CARTESIAN_POINT('Ctrl Pts',(-69.9835672729193,12.7557137255404,-26.4623716600327));
#42188=CARTESIAN_POINT('Ctrl Pts',(-69.9847896256528,12.7560536229567,-27.971270691958));
#42189=CARTESIAN_POINT('Ctrl Pts',(-69.9849923393715,12.7560277680565,-28.9763997254712));
#42190=CARTESIAN_POINT('Ctrl Pts',(-69.9847790976071,12.7559071214205,-29.5408320492003));
#42191=CARTESIAN_POINT('Ctrl Pts',(-69.9847190327587,12.7558758616894,-29.6662774310689));
#42192=CARTESIAN_POINT('Ctrl Pts',(-69.984552223832,12.7557959781981,-29.9172053601299));
#42193=CARTESIAN_POINT('Ctrl Pts',(-69.9841465990849,12.755614662297,-30.3564674006169));
#42194=CARTESIAN_POINT('Ctrl Pts',(-69.9829532444279,12.755104651033,-31.2353562879841));
#42195=CARTESIAN_POINT('Ctrl Pts',(-69.9805687035159,12.7540941885417,-32.4912820588143));
#42196=CARTESIAN_POINT('Ctrl Pts',(-69.9783817358907,12.753042894257,-33.7457473070251));
#42197=CARTESIAN_POINT('Ctrl Pts',(-69.9774127622085,12.7523768445192,-34.7472551726568));
#42198=CARTESIAN_POINT('Ctrl Pts',(-69.9772980945349,12.7521433192641,-35.247158075241));
#42199=CARTESIAN_POINT('Ctrl Pts',(-69.9773927097792,12.7520138717686,-35.622686066461));
#42200=CARTESIAN_POINT('Ctrl Pts',(-69.9775133714002,12.7519146402004,-35.8745548934899));
#42201=CARTESIAN_POINT('Ctrl Pts',(-69.9779586307213,12.7516764180863,-36.3773291823379));
#42202=CARTESIAN_POINT('Ctrl Pts',(-69.9792060003252,12.7512071226226,-37.2556581271203));
#42203=CARTESIAN_POINT('Ctrl Pts',(-69.9830484660371,12.7502671745843,-39.0072803971456));
#42204=CARTESIAN_POINT('Ctrl Pts',(-69.9868358117171,12.7504863846341,-40.5071496610249));
#42205=CARTESIAN_POINT('Ctrl Pts',(-69.9882537365034,12.7522335185554,-41.7614999300598));
#42206=CARTESIAN_POINT('Ctrl Pts',(-69.988523924384,12.7522689106951,-42.1399969035111));
#42207=CARTESIAN_POINT('Ctrl Pts',(-69.9886722200598,12.7517528417585,-42.6422651008279));
#42208=CARTESIAN_POINT('Ctrl Pts',(-69.9887094014331,12.7510060141183,-43.1447647900567));
#42209=CARTESIAN_POINT('Ctrl Pts',(-69.9886054825973,12.7498953589051,-43.7719630105579));
#42210=CARTESIAN_POINT('Ctrl Pts',(-69.988425173086,12.749106300016,-44.5231007995684));
#42211=CARTESIAN_POINT('Ctrl Pts',(-69.988383644029,12.7495845265692,-45.1472004354468));
#42212=CARTESIAN_POINT('Ctrl Pts',(-69.9885096857935,12.7510464325718,-45.6451717793566));
#42213=CARTESIAN_POINT('Ctrl Pts',(-69.9887071266115,12.7527869079614,-46.017901097045));
#42214=CARTESIAN_POINT('Ctrl Pts',(-69.9890309693273,12.7552717791395,-46.3898474617455));
#42215=CARTESIAN_POINT('Ctrl Pts',(-69.9896632214316,12.7597063096198,-46.8845642943284));
#42216=CARTESIAN_POINT('Ctrl Pts',(-69.9903971337144,12.7644558765816,-47.254324379301));
#42217=CARTESIAN_POINT('Ctrl Pts',(-69.9913561982648,12.7703474655071,-47.6234819913124));
#42218=CARTESIAN_POINT('Ctrl Pts',(-69.9920745336061,12.7754555967541,-47.8577571348398));
#42219=CARTESIAN_POINT('Ctrl Pts',(-69.9936461974301,12.7905471997396,-48.3392030878483));
#42220=CARTESIAN_POINT('Ctrl Pts',(-69.9967581941422,12.8272250940851,-49.1902610781344));
#42221=CARTESIAN_POINT('Ctrl Pts',(-70.0019464278965,12.8968161905817,-50.4444677902403));
#42222=CARTESIAN_POINT('Ctrl Pts',(-70.0092115061526,12.9635283622005,-52.0042169411895));
#42223=CARTESIAN_POINT('Ctrl Pts',(-70.0151328854528,12.9638783345927,-53.0818951197487));
#42224=CARTESIAN_POINT('Ctrl Pts',(-70.0194805733487,12.9386820326978,-53.7695514912596));
#42225=CARTESIAN_POINT('Ctrl Pts',(-70.021616000932,12.9219428845158,-54.0750564285113));
#42226=CARTESIAN_POINT('Ctrl Pts',(-70.026421203681,12.8714101731903,-54.6535562856163));
#42227=CARTESIAN_POINT('Ctrl Pts',(-70.0357215940866,12.7478235203842,-55.6356921285918));
#42228=CARTESIAN_POINT('Ctrl Pts',(-70.0545706652888,12.4312446036475,-57.443882033324));
#42229=CARTESIAN_POINT('Ctrl Pts',(-70.0621906425967,12.2690752169479,-58.7315035512416));
#42230=CARTESIAN_POINT('Ctrl Pts',(-70.0698682848343,12.3163671846014,-59.4962771807332));
#42231=CARTESIAN_POINT('Ctrl Pts',(-70.0706383028307,12.3239921932981,-59.609619365006));
#42232=CARTESIAN_POINT('Ctrl Pts',(-70.0722338644273,12.3416983613519,-59.8257567538662));
#42233=CARTESIAN_POINT('Ctrl Pts',(-70.0748935291213,12.3809699258908,-60.2118321945912));
#42234=CARTESIAN_POINT('Ctrl Pts',(-70.0798793331697,12.490177829677,-60.9877372918059));
#42235=CARTESIAN_POINT('Ctrl Pts',(-70.084679822235,12.6810981003491,-61.8930259126653));
#42236=CARTESIAN_POINT('Ctrl Pts',(-70.0887291925924,12.9272005920432,-62.8076987730538));
#42237=CARTESIAN_POINT('Ctrl Pts',(-70.0907884488415,13.0840177628279,-63.3252448496941));
#42238=CARTESIAN_POINT('Ctrl Pts',(-70.0920985582379,13.1952454731271,-63.6709159868783));
#42239=CARTESIAN_POINT('Ctrl Pts',(-70.0929574092067,13.2711121021537,-63.9015513719062));
#42240=CARTESIAN_POINT('Ctrl Pts',(-70.0938023132969,13.3494172624026,-64.1322802790929));
#42241=CARTESIAN_POINT('Ctrl Pts',(-70.094530689255,13.4199226892588,-64.3343142963286));
#42242=CARTESIAN_POINT('Ctrl Pts',(-70.0949450256968,13.46075135641,-64.4497830538115));
#42243=CARTESIAN_POINT('Ctrl Pts',(-70.0955666466438,13.5225103365915,-64.6229748956723));
#42244=CARTESIAN_POINT('Ctrl Pts',(-70.0960810583999,13.5750580934916,-64.7673495223908));
#42245=CARTESIAN_POINT('Ctrl Pts',(-70.0969701168715,13.6630921096615,-65.0057190804797));
#42246=CARTESIAN_POINT('Ctrl Pts',(-70.0996087278747,13.7459487610903,-65.2186539217629));
#42247=CARTESIAN_POINT('Ctrl Pts',(-70.1036343446273,13.9352298848311,-65.6686469867403));
#42248=CARTESIAN_POINT('Ctrl Pts',(-70.1103127543902,14.3037368141752,-66.4581519152683));
#42249=CARTESIAN_POINT('Ctrl Pts',(-70.1186303204434,15.1838581762324,-68.0971112119206));
#42250=CARTESIAN_POINT('Ctrl Pts',(-70.1163303848665,16.0819463876766,-69.5916304392682));
#42251=CARTESIAN_POINT('Ctrl Pts',(-70.1108693306998,16.7134282989604,-70.7930862089204));
#42252=CARTESIAN_POINT('Ctrl Pts',(-70.1113470826655,16.8423130561934,-71.0376385468314));
#42253=CARTESIAN_POINT('Ctrl Pts',(-70.1113105709919,17.1076598182307,-71.5401534806291));
#42254=CARTESIAN_POINT('Ctrl Pts',(-70.1116326619803,17.4376558910464,-72.1628824859081));
#42255=CARTESIAN_POINT('Ctrl Pts',(-70.111747802197,17.8367052278182,-72.9135665131352));
#42256=CARTESIAN_POINT('Ctrl Pts',(-70.1120030741606,18.6362099071052,-74.4140525108728));
#42257=CARTESIAN_POINT('Ctrl Pts',(-70.1119687058294,19.3060997676304,-75.6668931110029));
#42258=CARTESIAN_POINT('Ctrl Pts',(-70.1117021926187,20.2778148148096,-77.4942856965309));
#42259=CARTESIAN_POINT('Ctrl Pts',(-70.1118181513274,20.7135146017487,-78.3135802751711));
#42260=CARTESIAN_POINT('Ctrl Pts',(-70.1118181513289,21.1500361891381,-79.1345579772626));
#42261=CARTESIAN_POINT('Ctrl Pts',(-67.2754322320213,7.4757630221787,24.8321255810971));
#42262=CARTESIAN_POINT('Ctrl Pts',(-67.2755705809386,7.47581763243593,24.7832923099026));
#42263=CARTESIAN_POINT('Ctrl Pts',(-67.2757157318436,7.47587475234481,24.7344612301898));
#42264=CARTESIAN_POINT('Ctrl Pts',(-67.2774319088059,7.47655431889977,24.1843846336179));
#42265=CARTESIAN_POINT('Ctrl Pts',(-67.2774494651673,7.47755687413155,23.1805744464059));
#42266=CARTESIAN_POINT('Ctrl Pts',(-67.2766235035466,7.48011201430047,21.1730765472028));
#42267=CARTESIAN_POINT('Ctrl Pts',(-67.2881197826209,7.4845991280751,19.6694790344265));
#42268=CARTESIAN_POINT('Ctrl Pts',(-67.3189731485589,7.49180979772324,18.4189751922483));
#42269=CARTESIAN_POINT('Ctrl Pts',(-67.3332328314049,7.4956322349772,17.9199743333444));
#42270=CARTESIAN_POINT('Ctrl Pts',(-67.3681259975055,7.50594132134161,16.9185156642757));
#42271=CARTESIAN_POINT('Ctrl Pts',(-67.4432905113739,7.52812635253163,15.1635432795567));
#42272=CARTESIAN_POINT('Ctrl Pts',(-67.522772202602,7.54446416298015,13.648896070725));
#42273=CARTESIAN_POINT('Ctrl Pts',(-67.5872153009134,7.54582825987786,12.3786335598512));
#42274=CARTESIAN_POINT('Ctrl Pts',(-67.6154204776456,7.54540033180308,11.8709509904796));
#42275=CARTESIAN_POINT('Ctrl Pts',(-67.6787468185927,7.5412077711249,10.8599911652357));
#42276=CARTESIAN_POINT('Ctrl Pts',(-67.7651833140421,7.53071460451453,9.60191254014628));
#42277=CARTESIAN_POINT('Ctrl Pts',(-67.8630876090932,7.51397052777016,8.10026383947153));
#42278=CARTESIAN_POINT('Ctrl Pts',(-67.9126109843987,7.50342730317955,7.10301976831543));
#42279=CARTESIAN_POINT('Ctrl Pts',(-67.9350070138697,7.4984053138877,6.48056930618348));
#42280=CARTESIAN_POINT('Ctrl Pts',(-67.9444957931639,7.49500156432598,6.21395100057163));
#42281=CARTESIAN_POINT('Ctrl Pts',(-67.9652928589601,7.48429166055158,5.69653581018919));
#42282=CARTESIAN_POINT('Ctrl Pts',(-68.0044466838936,7.45799259920056,4.79761339447914));
#42283=CARTESIAN_POINT('Ctrl Pts',(-68.0793245519533,7.39327191476882,3.05333199869326));
#42284=CARTESIAN_POINT('Ctrl Pts',(-68.0845307050997,7.39164300891083,1.64861862663291));
#42285=CARTESIAN_POINT('Ctrl Pts',(-68.0031627403797,7.4622667172992,0.710098961592749));
#42286=CARTESIAN_POINT('Ctrl Pts',(-67.9923709016977,7.47255008470439,0.579449910835283));
#42287=CARTESIAN_POINT('Ctrl Pts',(-67.9672546452685,7.49147815214768,0.331053566575222));
#42288=CARTESIAN_POINT('Ctrl Pts',(-67.9144380698456,7.5238364670556,-0.103990457920467));
#42289=CARTESIAN_POINT('Ctrl Pts',(-67.8174273409239,7.56603084566458,-0.707454744008557));
#42290=CARTESIAN_POINT('Ctrl Pts',(-67.6796650820582,7.61274839096469,-1.41320481599388));
#42291=CARTESIAN_POINT('Ctrl Pts',(-67.4859137058936,7.67763165669604,-2.33059832461395));
#42292=CARTESIAN_POINT('Ctrl Pts',(-67.2607353653355,7.78643519277926,-3.44759918903815));
#42293=CARTESIAN_POINT('Ctrl Pts',(-67.1478083966393,7.97895549501847,-4.3222442690895));
#42294=CARTESIAN_POINT('Ctrl Pts',(-67.1058926808869,8.15325576339432,-4.85873369997395));
#42295=CARTESIAN_POINT('Ctrl Pts',(-67.0971683145861,8.21760514823808,-5.02933657075882));
#42296=CARTESIAN_POINT('Ctrl Pts',(-67.0760798163985,8.39201841664085,-5.42526239502765));
#42297=CARTESIAN_POINT('Ctrl Pts',(-67.03904188196,8.78206000803595,-6.16219966869188));
#42298=CARTESIAN_POINT('Ctrl Pts',(-66.9674979596952,9.53618905798644,-7.35158730514667));
#42299=CARTESIAN_POINT('Ctrl Pts',(-66.8802894966432,10.372303287372,-8.66590951801085));
#42300=CARTESIAN_POINT('Ctrl Pts',(-66.8243846116526,10.9059313183747,-9.68399100585595));
#42301=CARTESIAN_POINT('Ctrl Pts',(-66.7972919426213,11.1783971007118,-10.3028728735934));
#42302=CARTESIAN_POINT('Ctrl Pts',(-66.7860516655838,11.3002413050387,-10.626878444251));
#42303=CARTESIAN_POINT('Ctrl Pts',(-66.77887046776,11.3847166946218,-10.8762865151733));
#42304=CARTESIAN_POINT('Ctrl Pts',(-66.7772989784454,11.4332747003404,-11.0205302214951));
#42305=CARTESIAN_POINT('Ctrl Pts',(-66.7756940985764,11.5284492720659,-11.320889056081));
#42306=CARTESIAN_POINT('Ctrl Pts',(-66.7809843984739,11.6784361246504,-11.8366659747363));
#42307=CARTESIAN_POINT('Ctrl Pts',(-66.8177655934338,11.924917887323,-12.8582347187859));
#42308=CARTESIAN_POINT('Ctrl Pts',(-66.9274108154291,12.1408200082236,-14.2621470942844));
#42309=CARTESIAN_POINT('Ctrl Pts',(-67.041480430644,12.2352182624232,-15.4502559001017));
#42310=CARTESIAN_POINT('Ctrl Pts',(-67.1033752206594,12.2839359550366,-16.2104420116553));
#42311=CARTESIAN_POINT('Ctrl Pts',(-67.1396331269749,12.3143823159889,-16.7094247054265));
#42312=CARTESIAN_POINT('Ctrl Pts',(-67.1597751406538,12.3367540398636,-17.0744826446256));
#42313=CARTESIAN_POINT('Ctrl Pts',(-67.1710420796526,12.3572346069264,-17.3744609695137));
#42314=CARTESIAN_POINT('Ctrl Pts',(-67.1750081532322,12.3661954177773,-17.5145108019458));
#42315=CARTESIAN_POINT('Ctrl Pts',(-67.1819313592866,12.3810343842226,-17.7811673358964));
#42316=CARTESIAN_POINT('Ctrl Pts',(-67.1872045835245,12.3930034573781,-18.0511067663896));
#42317=CARTESIAN_POINT('Ctrl Pts',(-67.1910471326289,12.4020167829618,-18.3172149975864));
#42318=CARTESIAN_POINT('Ctrl Pts',(-67.1928746823619,12.4065925190783,-18.4835108802885));
#42319=CARTESIAN_POINT('Ctrl Pts',(-67.1940169378708,12.409629318995,-18.6159908563114));
#42320=CARTESIAN_POINT('Ctrl Pts',(-67.1947179035365,12.4116154912796,-18.7152308292935));
#42321=CARTESIAN_POINT('Ctrl Pts',(-67.1951772825936,12.4130321638294,-18.7977648718811));
#42322=CARTESIAN_POINT('Ctrl Pts',(-67.1954721588069,12.4140298350441,-18.8637109791609));
#42323=CARTESIAN_POINT('Ctrl Pts',(-67.1975777453642,12.4217425034244,-19.4237549404876));
#42324=CARTESIAN_POINT('Ctrl Pts',(-67.1891546020952,12.4130338676924,-20.4793867008131));
#42325=CARTESIAN_POINT('Ctrl Pts',(-67.1629544371965,12.3746171685172,-21.9943111510365));
#42326=CARTESIAN_POINT('Ctrl Pts',(-67.1512169371865,12.35790654959,-22.9761797143203));
#42327=CARTESIAN_POINT('Ctrl Pts',(-67.1503428753901,12.3581065561651,-23.5799735642095));
#42328=CARTESIAN_POINT('Ctrl Pts',(-67.1500443571836,12.3582079065643,-23.832139615935));
#42329=CARTESIAN_POINT('Ctrl Pts',(-67.1496270629664,12.3584370651098,-24.3298720223066));
#42330=CARTESIAN_POINT('Ctrl Pts',(-67.1493180411603,12.3589006541,-25.2066041979464));
#42331=CARTESIAN_POINT('Ctrl Pts',(-67.1497943090567,12.359625042183,-26.4611455773589));
#42332=CARTESIAN_POINT('Ctrl Pts',(-67.1509133188839,12.3602460538217,-27.9707230001521));
#42333=CARTESIAN_POINT('Ctrl Pts',(-67.1514200620566,12.3602526285253,-28.9761938345696));
#42334=CARTESIAN_POINT('Ctrl Pts',(-67.1514670086208,12.3600746705999,-29.5408978499594));
#42335=CARTESIAN_POINT('Ctrl Pts',(-67.1514707984293,12.3600288621789,-29.6664071507096));
#42336=CARTESIAN_POINT('Ctrl Pts',(-67.15145485088,12.3599117051442,-29.9174517359273));
#42337=CARTESIAN_POINT('Ctrl Pts',(-67.1513709046654,12.3596452911758,-30.3569094723028));
#42338=CARTESIAN_POINT('Ctrl Pts',(-67.1510286339558,12.3588955981039,-31.2361249633699));
#42339=CARTESIAN_POINT('Ctrl Pts',(-67.1503177795842,12.3574019954836,-32.492341994905));
#42340=CARTESIAN_POINT('Ctrl Pts',(-67.1500578075652,12.3558315772813,-33.7468367107806));
#42341=CARTESIAN_POINT('Ctrl Pts',(-67.1505685996278,12.3548177890257,-34.7481724761365));
#42342=CARTESIAN_POINT('Ctrl Pts',(-67.1511366027792,12.3544470739449,-35.2479443558075));
#42343=CARTESIAN_POINT('Ctrl Pts',(-67.151710177535,12.3542337839783,-35.6233483768898));
#42344=CARTESIAN_POINT('Ctrl Pts',(-67.1521595997931,12.3540805990332,-35.8752264773858));
#42345=CARTESIAN_POINT('Ctrl Pts',(-67.1532881011523,12.3537436882837,-36.37796293713));
#42346=CARTESIAN_POINT('Ctrl Pts',(-67.1557824192001,12.3531236898836,-37.2562620752088));
#42347=CARTESIAN_POINT('Ctrl Pts',(-67.1622143470569,12.3519562497411,-39.0077775913824));
#42348=CARTESIAN_POINT('Ctrl Pts',(-67.1679797364291,12.3520581762157,-40.5075856924395));
#42349=CARTESIAN_POINT('Ctrl Pts',(-67.1704705762212,12.3536956253068,-41.7618662070699));
#42350=CARTESIAN_POINT('Ctrl Pts',(-67.1710199552577,12.3536945457625,-42.1403574085443));
#42351=CARTESIAN_POINT('Ctrl Pts',(-67.1714736601701,12.3531280238148,-42.6426012862483));
#42352=CARTESIAN_POINT('Ctrl Pts',(-67.1717766222623,12.3523303716963,-43.1450763086216));
#42353=CARTESIAN_POINT('Ctrl Pts',(-67.1719403089611,12.35115790606,-43.7722363024753));
#42354=CARTESIAN_POINT('Ctrl Pts',(-67.1720084137478,12.3503043777855,-44.5233188378637));
#42355=CARTESIAN_POINT('Ctrl Pts',(-67.1721388745049,12.3507428083146,-45.147364066605));
#42356=CARTESIAN_POINT('Ctrl Pts',(-67.1723970297961,12.3521845659274,-45.6452843848084));
#42357=CARTESIAN_POINT('Ctrl Pts',(-67.1726945719965,12.3539166793565,-46.0179728583073));
#42358=CARTESIAN_POINT('Ctrl Pts',(-67.1731233944469,12.3564007832012,-46.3898756442327));
#42359=CARTESIAN_POINT('Ctrl Pts',(-67.173907190769,12.3608454915033,-46.8845301952318));
#42360=CARTESIAN_POINT('Ctrl Pts',(-67.1747736668019,12.3656167149972,-47.2542405740443));
#42361=CARTESIAN_POINT('Ctrl Pts',(-67.1758857581577,12.3715408530953,-47.6233441990874));
#42362=CARTESIAN_POINT('Ctrl Pts',(-67.1767001397065,12.376672274449,-47.8575659949926));
#42363=CARTESIAN_POINT('Ctrl Pts',(-67.1784460180514,12.3918218385907,-48.3389264315629));
#42364=CARTESIAN_POINT('Ctrl Pts',(-67.1818261944169,12.4286292243439,-49.1898560942608));
#42365=CARTESIAN_POINT('Ctrl Pts',(-67.1873609124508,12.4984868596341,-50.4439578574161));
#42366=CARTESIAN_POINT('Ctrl Pts',(-67.1951733397397,12.565626926741,-52.0036846004141));
#42367=CARTESIAN_POINT('Ctrl Pts',(-67.2016690783125,12.5663061222207,-53.0814149816948));
#42368=CARTESIAN_POINT('Ctrl Pts',(-67.2064789926283,12.5413177612883,-53.7691211085328));
#42369=CARTESIAN_POINT('Ctrl Pts',(-67.2088116313674,12.5246755553911,-54.0745985103634));
#42370=CARTESIAN_POINT('Ctrl Pts',(-67.2140688628474,12.4743493841427,-54.6530762516019));
#42371=CARTESIAN_POINT('Ctrl Pts',(-67.2242908291814,12.3511593671177,-55.6351736922375));
#42372=CARTESIAN_POINT('Ctrl Pts',(-67.2453866476106,12.0354472455036,-57.4433406611621));
#42373=CARTESIAN_POINT('Ctrl Pts',(-67.2549899284182,11.87386411116,-58.7310581353012));
#42374=CARTESIAN_POINT('Ctrl Pts',(-67.2634764260892,11.9213680452202,-59.4960375627948));
#42375=CARTESIAN_POINT('Ctrl Pts',(-67.2643428975657,11.929020325518,-59.6094025664119));
#42376=CARTESIAN_POINT('Ctrl Pts',(-67.2661229085829,11.9467751815193,-59.8255841341478));
#42377=CARTESIAN_POINT('Ctrl Pts',(-67.2690844957648,11.9861214596594,-60.2117300472603));
#42378=CARTESIAN_POINT('Ctrl Pts',(-67.2745957471064,12.0954359936569,-60.9877494117348));
#42379=CARTESIAN_POINT('Ctrl Pts',(-67.2798403939225,12.2863932650726,-61.8931045719696));
#42380=CARTESIAN_POINT('Ctrl Pts',(-67.2842233506651,12.532479666206,-62.8077863856855));
#42381=CARTESIAN_POINT('Ctrl Pts',(-67.2864382164809,12.6892759716219,-63.3253180861268));
#42382=CARTESIAN_POINT('Ctrl Pts',(-67.2878428582821,12.8004882189023,-63.6709723005203));
#42383=CARTESIAN_POINT('Ctrl Pts',(-67.2887625715289,12.876344402861,-63.9015944753022));
#42384=CARTESIAN_POINT('Ctrl Pts',(-67.2896655043126,12.9546392534038,-64.1323074621358));
#42385=CARTESIAN_POINT('Ctrl Pts',(-67.2904429757562,13.0251364600611,-64.334325166348));
#42386=CARTESIAN_POINT('Ctrl Pts',(-67.2908849974231,13.0659607520918,-64.4497839441229));
#42387=CARTESIAN_POINT('Ctrl Pts',(-67.2915478237582,13.1277135490983,-64.6229601846799));
#42388=CARTESIAN_POINT('Ctrl Pts',(-67.292096048499,13.1802570070354,-64.7673204410586));
#42389=CARTESIAN_POINT('Ctrl Pts',(-67.2930408018807,13.2682857663681,-65.0056649728891));
#42390=CARTESIAN_POINT('Ctrl Pts',(-67.2957192466897,13.3511433890363,-65.2186001383609));
#42391=CARTESIAN_POINT('Ctrl Pts',(-67.2998050326217,13.5404202332849,-65.6685810191878));
#42392=CARTESIAN_POINT('Ctrl Pts',(-67.3065272003076,13.9089172400581,-66.4580761268423));
#42393=CARTESIAN_POINT('Ctrl Pts',(-67.3147653261941,14.7890086193988,-68.0970223218478));
#42394=CARTESIAN_POINT('Ctrl Pts',(-67.3123125064053,15.6870807723725,-69.5915449895342));
#42395=CARTESIAN_POINT('Ctrl Pts',(-67.3068846662169,16.3185728591383,-70.7930072900375));
#42396=CARTESIAN_POINT('Ctrl Pts',(-67.3073607613388,16.4474560716216,-71.0375585891527));
#42397=CARTESIAN_POINT('Ctrl Pts',(-67.307325727314,16.7128021838016,-71.5400729754856));
#42398=CARTESIAN_POINT('Ctrl Pts',(-67.3076469814166,17.0427969476755,-72.1628009962699));
#42399=CARTESIAN_POINT('Ctrl Pts',(-67.3077616390266,17.4418457255338,-72.9134843805435));
#42400=CARTESIAN_POINT('Ctrl Pts',(-67.3080145306994,18.2413498671255,-74.4139694720434));
#42401=CARTESIAN_POINT('Ctrl Pts',(-67.3079779188089,18.9112408709397,-75.6668108364885));
#42402=CARTESIAN_POINT('Ctrl Pts',(-67.3077127272134,19.8829571287319,-77.4942050732508));
#42403=CARTESIAN_POINT('Ctrl Pts',(-67.3078280944553,20.318656508363,-78.3134992775899));
#42404=CARTESIAN_POINT('Ctrl Pts',(-67.3078280944529,20.7551780957521,-79.134476979685));
#42405=CARTESIAN_POINT('Ctrl Pts',(-65.1729327667129,7.18175574164057,24.8300916319504));
#42406=CARTESIAN_POINT('Ctrl Pts',(-65.1731006306621,7.18176547068664,24.781194303211));
#42407=CARTESIAN_POINT('Ctrl Pts',(-65.1732766972058,7.18177566391607,24.7322978687525));
#42408=CARTESIAN_POINT('Ctrl Pts',(-65.1753571165701,7.18189796096853,24.181473259413));
#42409=CARTESIAN_POINT('Ctrl Pts',(-65.176438647727,7.18157806354087,23.1769240129338));
#42410=CARTESIAN_POINT('Ctrl Pts',(-65.1785990533414,7.18054693828407,21.1679996176307));
#42411=CARTESIAN_POINT('Ctrl Pts',(-65.192484643868,7.18138468374927,19.6638715508315));
#42412=CARTESIAN_POINT('Ctrl Pts',(-65.2244936611386,7.18522550993877,18.4129862938216));
#42413=CARTESIAN_POINT('Ctrl Pts',(-65.2395231838244,7.18700742344305,17.9096005950179));
#42414=CARTESIAN_POINT('Ctrl Pts',(-65.2767049565944,7.19137325174919,16.9050968056351));
#42415=CARTESIAN_POINT('Ctrl Pts',(-65.3564962710775,7.20089393748341,15.1508281818811));
#42416=CARTESIAN_POINT('Ctrl Pts',(-65.4366562425691,7.21131561767836,13.6505216649638));
#42417=CARTESIAN_POINT('Ctrl Pts',(-65.4947464921632,7.22052378517439,12.3986048174561));
#42418=CARTESIAN_POINT('Ctrl Pts',(-65.5194228726211,7.22461698459507,11.8988115580567));
#42419=CARTESIAN_POINT('Ctrl Pts',(-65.5726798734756,7.23405319214692,10.898840753164));
#42420=CARTESIAN_POINT('Ctrl Pts',(-65.6430001132168,7.2471190074519,9.64780942493501));
#42421=CARTESIAN_POINT('Ctrl Pts',(-65.7210118147592,7.2622821734432,8.14323182215361));
#42422=CARTESIAN_POINT('Ctrl Pts',(-65.7607837886347,7.26991612109166,7.13698809994421));
#42423=CARTESIAN_POINT('Ctrl Pts',(-65.7791343148924,7.27337759048613,6.50737055322745));
#42424=CARTESIAN_POINT('Ctrl Pts',(-65.7866816659716,7.2744078822174,6.25153810606456));
#42425=CARTESIAN_POINT('Ctrl Pts',(-65.8021713561666,7.27501414102468,5.74396397630533));
#42426=CARTESIAN_POINT('Ctrl Pts',(-65.8293878736281,7.27299490306546,4.85742889524331));
#42427=CARTESIAN_POINT('Ctrl Pts',(-65.8752994724579,7.26213375344673,3.09979743749822));
#42428=CARTESIAN_POINT('Ctrl Pts',(-65.8735048151651,7.25912195022732,1.62896241126073));
#42429=CARTESIAN_POINT('Ctrl Pts',(-65.8322698068349,7.28148808984448,0.604410369730052));
#42430=CARTESIAN_POINT('Ctrl Pts',(-65.8269365106498,7.28382509893192,0.458530192554338));
#42431=CARTESIAN_POINT('Ctrl Pts',(-65.8150539209303,7.28525649887588,0.183890613738274));
#42432=CARTESIAN_POINT('Ctrl Pts',(-65.7909935752901,7.28121908724863,-0.295181368341263));
#42433=CARTESIAN_POINT('Ctrl Pts',(-65.7479654170422,7.2620589119011,-0.950370087138988));
#42434=CARTESIAN_POINT('Ctrl Pts',(-65.6840197828005,7.23415949011369,-1.69777034578746));
#42435=CARTESIAN_POINT('Ctrl Pts',(-65.5854876409769,7.20742295195961,-2.63740705266532));
#42436=CARTESIAN_POINT('Ctrl Pts',(-65.4443779860654,7.22096622634433,-3.70705755910344));
#42437=CARTESIAN_POINT('Ctrl Pts',(-65.345245023354,7.33247226156198,-4.47217890661716));
#42438=CARTESIAN_POINT('Ctrl Pts',(-65.2979157678212,7.45312012683586,-4.93759588484351));
#42439=CARTESIAN_POINT('Ctrl Pts',(-65.2804785126524,7.50112655480425,-5.0995647485744));
#42440=CARTESIAN_POINT('Ctrl Pts',(-65.2395481259881,7.63544794831347,-5.47205399305951));
#42441=CARTESIAN_POINT('Ctrl Pts',(-65.1562506133512,7.95410912208094,-6.18518406530892));
#42442=CARTESIAN_POINT('Ctrl Pts',(-65.0052479173948,8.61964836548844,-7.35890192235289));
#42443=CARTESIAN_POINT('Ctrl Pts',(-64.8395199160683,9.40141111790384,-8.66272049186451));
#42444=CARTESIAN_POINT('Ctrl Pts',(-64.7377773979986,9.91756603305767,-9.65968667108287));
#42445=CARTESIAN_POINT('Ctrl Pts',(-64.6888422500041,10.1892383163194,-10.259520915547));
#42446=CARTESIAN_POINT('Ctrl Pts',(-64.6685015126593,10.3146673064093,-10.571342686021));
#42447=CARTESIAN_POINT('Ctrl Pts',(-64.6554064435216,10.40373887505,-10.8102983290437));
#42448=CARTESIAN_POINT('Ctrl Pts',(-64.6520444913612,10.4533044253585,-10.9405423567448));
#42449=CARTESIAN_POINT('Ctrl Pts',(-64.6458528877893,10.5562636271704,-11.2173755632169));
#42450=CARTESIAN_POINT('Ctrl Pts',(-64.6443003259781,10.729009873209,-11.6917518645855));
#42451=CARTESIAN_POINT('Ctrl Pts',(-64.6692140356061,11.0572039967835,-12.6414406117879));
#42452=CARTESIAN_POINT('Ctrl Pts',(-64.7748437077602,11.4627448290961,-13.9868601108971));
#42453=CARTESIAN_POINT('Ctrl Pts',(-64.9023929031954,11.7353176655387,-15.1977465931819));
#42454=CARTESIAN_POINT('Ctrl Pts',(-64.9730859398394,11.8780561006582,-16.003632893284));
#42455=CARTESIAN_POINT('Ctrl Pts',(-65.0144064204024,11.9637472321134,-16.5408015357675));
#42456=CARTESIAN_POINT('Ctrl Pts',(-65.036810908705,12.0176256541411,-16.9430078212279));
#42457=CARTESIAN_POINT('Ctrl Pts',(-65.0483918994916,12.0576678349292,-17.2778640553446));
#42458=CARTESIAN_POINT('Ctrl Pts',(-65.0524394558381,12.0742199515051,-17.4248988623711));
#42459=CARTESIAN_POINT('Ctrl Pts',(-65.059593815533,12.1019222700238,-17.7087034577803));
#42460=CARTESIAN_POINT('Ctrl Pts',(-65.065115123067,12.1239068138689,-17.9932360279406));
#42461=CARTESIAN_POINT('Ctrl Pts',(-65.0692116335719,12.1403445332771,-18.2735090635166));
#42462=CARTESIAN_POINT('Ctrl Pts',(-65.0711917791365,12.1485863813074,-18.4479829553626));
#42463=CARTESIAN_POINT('Ctrl Pts',(-65.0724518363108,12.1540079468313,-18.5867619236669));
#42464=CARTESIAN_POINT('Ctrl Pts',(-65.0732381579507,12.1575226457074,-18.6905548579323));
#42465=CARTESIAN_POINT('Ctrl Pts',(-65.0737661119046,12.1600040267476,-18.776760678138));
#42466=CARTESIAN_POINT('Ctrl Pts',(-65.0741139960963,12.161734611473,-18.8455631933068));
#42467=CARTESIAN_POINT('Ctrl Pts',(-65.0766615262646,12.1750053272291,-19.4294573932671));
#42468=CARTESIAN_POINT('Ctrl Pts',(-65.0687114676951,12.1567208841226,-20.5166934694074));
#42469=CARTESIAN_POINT('Ctrl Pts',(-65.0420209941393,12.0860740690322,-22.0377659033389));
#42470=CARTESIAN_POINT('Ctrl Pts',(-65.0297090483665,12.0563534656099,-22.9972621820203));
#42471=CARTESIAN_POINT('Ctrl Pts',(-65.0288044687836,12.0559985325857,-23.5792914978727));
#42472=CARTESIAN_POINT('Ctrl Pts',(-65.0284706314498,12.0558629287408,-23.8339510858948));
#42473=CARTESIAN_POINT('Ctrl Pts',(-65.0278976338286,12.0556160776309,-24.3303747538134));
#42474=CARTESIAN_POINT('Ctrl Pts',(-65.0271282891604,12.0552335060199,-25.2079354084859));
#42475=CARTESIAN_POINT('Ctrl Pts',(-65.026601121765,12.0548554597604,-26.4615383680323));
#42476=CARTESIAN_POINT('Ctrl Pts',(-65.0265849159444,12.0546807638577,-27.9706860922064));
#42477=CARTESIAN_POINT('Ctrl Pts',(-65.0267830893282,12.0547572443005,-28.975322605205));
#42478=CARTESIAN_POINT('Ctrl Pts',(-65.0268966462046,12.0548512731844,-29.539530536201));
#42479=CARTESIAN_POINT('Ctrl Pts',(-65.0269197971744,12.0548744982796,-29.6648497847285));
#42480=CARTESIAN_POINT('Ctrl Pts',(-65.0269599296714,12.0549296743612,-29.9155791753429));
#42481=CARTESIAN_POINT('Ctrl Pts',(-65.0270172921303,12.055050139514,-30.3545185075444));
#42482=CARTESIAN_POINT('Ctrl Pts',(-65.027114817731,12.0553729207471,-31.2329193484625));
#42483=CARTESIAN_POINT('Ctrl Pts',(-65.0273850542116,12.0560432368111,-32.4885410674878));
#42484=CARTESIAN_POINT('Ctrl Pts',(-65.0283289325803,12.0568680050243,-33.7431920138229));
#42485=CARTESIAN_POINT('Ctrl Pts',(-65.0297895448079,12.0575451092745,-34.7450603784708));
#42486=CARTESIAN_POINT('Ctrl Pts',(-65.0308017464864,12.0578906286939,-35.2452602875554));
#42487=CARTESIAN_POINT('Ctrl Pts',(-65.0316892610028,12.0581422004777,-35.6210283418864));
#42488=CARTESIAN_POINT('Ctrl Pts',(-65.032356599898,12.0582981071551,-35.8728926831772));
#42489=CARTESIAN_POINT('Ctrl Pts',(-65.0339471095556,12.0585643755601,-36.3757447541211));
#42490=CARTESIAN_POINT('Ctrl Pts',(-65.0373045889605,12.0589701842811,-37.2541885309612));
#42491=CARTESIAN_POINT('Ctrl Pts',(-65.0455921016347,12.0596801196328,-39.0060372985966));
#42492=CARTESIAN_POINT('Ctrl Pts',(-65.0528329561677,12.0610847527648,-40.506167908724));
#42493=CARTESIAN_POINT('Ctrl Pts',(-65.0561230687881,12.0635538952629,-41.7607219271154));
#42494=CARTESIAN_POINT('Ctrl Pts',(-65.0568807869497,12.0637897616258,-42.1392522960393));
#42495=CARTESIAN_POINT('Ctrl Pts',(-65.0575648769863,12.0635101890673,-42.6415769457643));
#42496=CARTESIAN_POINT('Ctrl Pts',(-65.0580703731843,12.0629819805719,-43.1441349944183));
#42497=CARTESIAN_POINT('Ctrl Pts',(-65.0584428191974,12.0621103910298,-43.7714134904261));
#42498=CARTESIAN_POINT('Ctrl Pts',(-65.0587147492222,12.0615562535142,-44.5226577243393));
#42499=CARTESIAN_POINT('Ctrl Pts',(-65.058996497838,12.0621888968184,-45.1468563514877));
#42500=CARTESIAN_POINT('Ctrl Pts',(-65.0593768292321,12.0637490456156,-45.6449060383322));
#42501=CARTESIAN_POINT('Ctrl Pts',(-65.05976957428,12.065551588587,-46.0176971655781));
#42502=CARTESIAN_POINT('Ctrl Pts',(-65.0603002313248,12.0680870066288,-46.3897078745373));
#42503=CARTESIAN_POINT('Ctrl Pts',(-65.0612326202001,12.0725740901228,-46.8845125519888));
#42504=CARTESIAN_POINT('Ctrl Pts',(-65.0622297353678,12.0773464433905,-47.2543460356923));
#42505=CARTESIAN_POINT('Ctrl Pts',(-65.0634913888751,12.0832508706114,-47.6235775922098));
#42506=CARTESIAN_POINT('Ctrl Pts',(-65.0644034048839,12.0883602483909,-47.8579214938423));
#42507=CARTESIAN_POINT('Ctrl Pts',(-65.0663413372696,12.1034236213073,-48.3394840139549));
#42508=CARTESIAN_POINT('Ctrl Pts',(-65.070052685802,12.1399819433414,-49.190730687232));
#42509=CARTESIAN_POINT('Ctrl Pts',(-65.0760796661541,12.2092354674003,-50.4451446520436));
#42510=CARTESIAN_POINT('Ctrl Pts',(-65.0845863352261,12.275437662191,-52.0050245066472));
#42511=CARTESIAN_POINT('Ctrl Pts',(-65.0916544734623,12.275475630366,-53.0826911850069));
#42512=CARTESIAN_POINT('Ctrl Pts',(-65.09686685345,12.2501386925666,-53.7703051293251));
#42513=CARTESIAN_POINT('Ctrl Pts',(-65.0993710942821,12.2333246964283,-54.0758996019516));
#42514=CARTESIAN_POINT('Ctrl Pts',(-65.1050038878201,12.1826499594705,-54.6544835605439));
#42515=CARTESIAN_POINT('Ctrl Pts',(-65.1159591757095,12.0588208329425,-55.6367269241876));
#42516=CARTESIAN_POINT('Ctrl Pts',(-65.1387536951772,11.7418820496672,-57.4448818104869));
#42517=CARTESIAN_POINT('Ctrl Pts',(-65.1497661458798,11.5796938358338,-58.7322284200674));
#42518=CARTESIAN_POINT('Ctrl Pts',(-65.1588520219563,11.6269959572717,-59.4966254801638));
#42519=CARTESIAN_POINT('Ctrl Pts',(-65.1597913711798,11.6346205198146,-59.6099285989042));
#42520=CARTESIAN_POINT('Ctrl Pts',(-65.1617104418904,11.6523304276544,-59.8259887953581));
#42521=CARTESIAN_POINT('Ctrl Pts',(-65.1649009270484,11.691615509919,-60.2119414469383));
#42522=CARTESIAN_POINT('Ctrl Pts',(-65.1708131027259,11.8008814112987,-60.9876425042924));
#42523=CARTESIAN_POINT('Ctrl Pts',(-65.1763985760326,11.9919267773979,-61.8927913471379));
#42524=CARTESIAN_POINT('Ctrl Pts',(-65.1810324756269,12.2381836869314,-62.8074081928519));
#42525=CARTESIAN_POINT('Ctrl Pts',(-65.1833616050184,12.3950912618894,-63.3249534797546));
#42526=CARTESIAN_POINT('Ctrl Pts',(-65.1848342053435,12.5063773919337,-63.6706366796427));
#42527=CARTESIAN_POINT('Ctrl Pts',(-65.1857972679305,12.5822823477447,-63.9012835400789));
#42528=CARTESIAN_POINT('Ctrl Pts',(-65.1867409286383,12.660624217389,-64.1320289060336));
#42529=CARTESIAN_POINT('Ctrl Pts',(-65.1875523445398,12.731160099571,-64.3340819354547));
#42530=CARTESIAN_POINT('Ctrl Pts',(-65.1880133661692,12.7720055701951,-64.4495628783271));
#42531=CARTESIAN_POINT('Ctrl Pts',(-65.1887043345812,12.8337891082829,-64.6227742878501));
#42532=CARTESIAN_POINT('Ctrl Pts',(-65.1892753734552,12.886355873928,-64.7671680924818));
#42533=CARTESIAN_POINT('Ctrl Pts',(-65.1902574334737,12.9744186327503,-65.0055722577058));
#42534=CARTESIAN_POINT('Ctrl Pts',(-65.1929639939196,13.0572795677294,-65.2184944200882));
#42535=CARTESIAN_POINT('Ctrl Pts',(-65.1970899407941,13.2465759472662,-65.6684907956169));
#42536=CARTESIAN_POINT('Ctrl Pts',(-65.2038379111266,13.6150876757719,-66.4579896989852));
#42537=CARTESIAN_POINT('Ctrl Pts',(-65.2120073023104,14.495184046943,-68.0969542174842));
#42538=CARTESIAN_POINT('Ctrl Pts',(-65.2094453005085,15.3932338570684,-69.5914701280964));
#42539=CARTESIAN_POINT('Ctrl Pts',(-65.2040506590276,16.0247361035807,-70.7929256923783));
#42540=CARTESIAN_POINT('Ctrl Pts',(-65.2045249298405,16.1536203661614,-71.0374784533412));
#42541=CARTESIAN_POINT('Ctrl Pts',(-65.2044911734284,16.4189686424828,-71.5399939605228));
#42542=CARTESIAN_POINT('Ctrl Pts',(-65.2048113970372,16.748964735239,-72.1627235728458));
#42543=CARTESIAN_POINT('Ctrl Pts',(-65.2049254398224,17.1480141148444,-72.9134082444139));
#42544=CARTESIAN_POINT('Ctrl Pts',(-65.2051758444602,17.94751750513,-74.4138952011896));
#42545=CARTESIAN_POINT('Ctrl Pts',(-65.2051372831542,18.6174048008469,-75.666735182131));
#42546=CARTESIAN_POINT('Ctrl Pts',(-65.2048737521369,19.589119601252,-77.4941259620686));
#42547=CARTESIAN_POINT('Ctrl Pts',(-65.2049884661457,20.0248191246354,-78.3134208257811));
#42548=CARTESIAN_POINT('Ctrl Pts',(-65.2049884661443,20.4613407120248,-79.1343985278809));
#42549=CARTESIAN_POINT('Ctrl Pts',(-63.7696894174353,6.98565352544322,24.8297715781906));
#42550=CARTESIAN_POINT('Ctrl Pts',(-63.7698754022371,6.98565901678319,24.7808654437697));
#42551=CARTESIAN_POINT('Ctrl Pts',(-63.7700704419802,6.98566484175051,24.7319599955762));
#42552=CARTESIAN_POINT('Ctrl Pts',(-63.7723747362441,6.98573226498455,24.1810332173695));
#42553=CARTESIAN_POINT('Ctrl Pts',(-63.7740759382634,6.98531388885199,23.1764572572281));
#42554=CARTESIAN_POINT('Ctrl Pts',(-63.7779798012375,6.98405340995919,21.1672988065382));
#42555=CARTESIAN_POINT('Ctrl Pts',(-63.7933215085387,6.98451453063052,19.662989697282));
#42556=CARTESIAN_POINT('Ctrl Pts',(-63.8261929975327,6.98782796082582,18.4119278795435));
#42557=CARTESIAN_POINT('Ctrl Pts',(-63.8418447324602,6.98925763853974,17.9076482542059));
#42558=CARTESIAN_POINT('Ctrl Pts',(-63.880926988907,6.99260755998853,16.9025804656894));
#42559=CARTESIAN_POINT('Ctrl Pts',(-63.9647088951749,6.99992394929679,15.1487433991109));
#42560=CARTESIAN_POINT('Ctrl Pts',(-64.0455470805801,7.00949894400017,13.6515218526789));
#42561=CARTESIAN_POINT('Ctrl Pts',(-64.098696702948,7.01997981272938,12.4032514948202));
#42562=CARTESIAN_POINT('Ctrl Pts',(-64.1207157044886,7.02480995950052,11.9049960438307));
#42563=CARTESIAN_POINT('Ctrl Pts',(-64.1665352750066,7.03635887512195,10.9070850335965));
#42564=CARTESIAN_POINT('Ctrl Pts',(-64.2244318158956,7.05318465097466,9.65722545946371));
#42565=CARTESIAN_POINT('Ctrl Pts',(-64.2866992888549,7.0730305690719,8.15210701155296));
#42566=CARTESIAN_POINT('Ctrl Pts',(-64.3177633310595,7.08346918516099,7.14421141822163));
#42567=CARTESIAN_POINT('Ctrl Pts',(-64.3322248208874,7.08827621830881,6.51340849004068));
#42568=CARTESIAN_POINT('Ctrl Pts',(-64.3379036734705,7.09000405968928,6.26145462276259));
#42569=CARTESIAN_POINT('Ctrl Pts',(-64.3488488955487,7.0928476106599,5.75783761392703));
#42570=CARTESIAN_POINT('Ctrl Pts',(-64.3665313656493,7.09644101342747,4.87630620818669));
#42571=CARTESIAN_POINT('Ctrl Pts',(-64.3931775759778,7.09983365583526,3.11473296932821));
#42572=CARTESIAN_POINT('Ctrl Pts',(-64.390706566645,7.10323420609789,1.61707447161998));
#42573=CARTESIAN_POINT('Ctrl Pts',(-64.3656735433867,7.11125149590393,0.566093556418151));
#42574=CARTESIAN_POINT('Ctrl Pts',(-64.3626063731248,7.11154332115744,0.417459700651948));
#42575=CARTESIAN_POINT('Ctrl Pts',(-64.3562519135411,7.10849507332251,0.137579049188044));
#42576=CARTESIAN_POINT('Ctrl Pts',(-64.3444164021131,7.09530783242205,-0.349523687108764));
#42577=CARTESIAN_POINT('Ctrl Pts',(-64.3252031381455,7.05979166709545,-1.01361669019925));
#42578=CARTESIAN_POINT('Ctrl Pts',(-64.2970831645417,7.00916298099789,-1.76931776303998));
#42579=CARTESIAN_POINT('Ctrl Pts',(-64.252057415312,6.95081827755828,-2.71870875872315));
#42580=CARTESIAN_POINT('Ctrl Pts',(-64.1790545778391,6.93153335347633,-3.79916535074235));
#42581=CARTESIAN_POINT('Ctrl Pts',(-64.1044018915843,7.02167392362584,-4.55546854069931));
#42582=CARTESIAN_POINT('Ctrl Pts',(-64.055960785065,7.12358918683067,-5.00983827241397));
#42583=CARTESIAN_POINT('Ctrl Pts',(-64.0352080829805,7.16701362915479,-5.1804555944748));
#42584=CARTESIAN_POINT('Ctrl Pts',(-63.9845619585847,7.2837517387543,-5.55675071672487));
#42585=CARTESIAN_POINT('Ctrl Pts',(-63.8768951076057,7.55749257169478,-6.2706362403536));
#42586=CARTESIAN_POINT('Ctrl Pts',(-63.6860409931831,8.12647345543323,-7.43121625720289));
#42587=CARTESIAN_POINT('Ctrl Pts',(-63.4897568246847,8.81062253157607,-8.71673413747512));
#42588=CARTESIAN_POINT('Ctrl Pts',(-63.3751676902504,9.27810483645933,-9.68542634044361));
#42589=CARTESIAN_POINT('Ctrl Pts',(-63.3215359864303,9.53122238448528,-10.2618406454498));
#42590=CARTESIAN_POINT('Ctrl Pts',(-63.299654584813,9.65124363494989,-10.5588933561495));
#42591=CARTESIAN_POINT('Ctrl Pts',(-63.2856764206741,9.73803276839272,-10.7852775908397));
#42592=CARTESIAN_POINT('Ctrl Pts',(-63.2822813596893,9.78582617521137,-10.9050332690881));
#42593=CARTESIAN_POINT('Ctrl Pts',(-63.275435806406,9.88868110167001,-11.1631131951564));
#42594=CARTESIAN_POINT('Ctrl Pts',(-63.2722147714165,10.0681138616425,-11.6064577992792));
#42595=CARTESIAN_POINT('Ctrl Pts',(-63.2908788132213,10.4351120140857,-12.5043246842074));
#42596=CARTESIAN_POINT('Ctrl Pts',(-63.3792311558901,10.9515206937253,-13.804208650469));
#42597=CARTESIAN_POINT('Ctrl Pts',(-63.4895117642943,11.3514805234501,-15.0210988949459));
#42598=CARTESIAN_POINT('Ctrl Pts',(-63.5517362811958,11.5696710320611,-15.855747929383));
#42599=CARTESIAN_POINT('Ctrl Pts',(-63.5881689262417,11.7012922018101,-16.4186870190564));
#42600=CARTESIAN_POINT('Ctrl Pts',(-63.6079221058119,11.7828702143422,-16.8479091406712));
#42601=CARTESIAN_POINT('Ctrl Pts',(-63.6177306458527,11.8399814853698,-17.209139536956));
#42602=CARTESIAN_POINT('Ctrl Pts',(-63.6212262162933,11.8623333559051,-17.3601464543715));
#42603=CARTESIAN_POINT('Ctrl Pts',(-63.6275625825483,11.9004279682416,-17.6553308721399));
#42604=CARTESIAN_POINT('Ctrl Pts',(-63.6327263352227,11.9305108061342,-17.9493048631528));
#42605=CARTESIAN_POINT('Ctrl Pts',(-63.636814929413,11.9532190071079,-18.2390800966978));
#42606=CARTESIAN_POINT('Ctrl Pts',(-63.6389297014477,11.9646334412043,-18.419027608437));
#42607=CARTESIAN_POINT('Ctrl Pts',(-63.6403699837502,11.9721946874457,-18.5620587376317));
#42608=CARTESIAN_POINT('Ctrl Pts',(-63.6413268066055,11.9771192867651,-18.6689280061842));
#42609=CARTESIAN_POINT('Ctrl Pts',(-63.6420245297228,11.9806217858325,-18.7576224800683));
#42610=CARTESIAN_POINT('Ctrl Pts',(-63.6425237893563,11.9830812331201,-18.8283632041732));
#42611=CARTESIAN_POINT('Ctrl Pts',(-63.6464473787105,12.0020513115575,-19.4284651472464));
#42612=CARTESIAN_POINT('Ctrl Pts',(-63.6437138971256,11.9798821969473,-20.5374478886419));
#42613=CARTESIAN_POINT('Ctrl Pts',(-63.6262506952142,11.8912747104092,-22.0636299507839));
#42614=CARTESIAN_POINT('Ctrl Pts',(-63.6179169859225,11.8553060677419,-23.0089801859288));
#42615=CARTESIAN_POINT('Ctrl Pts',(-63.618118343459,11.8553665692817,-23.5769319212298));
#42616=CARTESIAN_POINT('Ctrl Pts',(-63.6181784988178,11.8553617093484,-23.833611292254));
#42617=CARTESIAN_POINT('Ctrl Pts',(-63.6182267748102,11.855244353337,-24.3297026902985));
#42618=CARTESIAN_POINT('Ctrl Pts',(-63.6181442093241,11.8547963251245,-25.2086594719894));
#42619=CARTESIAN_POINT('Ctrl Pts',(-63.6176784819112,11.8537177944518,-26.4623719266191));
#42620=CARTESIAN_POINT('Ctrl Pts',(-63.6169388654805,11.8525376530228,-27.9714101984933));
#42621=CARTESIAN_POINT('Ctrl Pts',(-63.6166024463615,11.8523626942919,-28.9751301649085));
#42622=CARTESIAN_POINT('Ctrl Pts',(-63.616525609042,11.8525915130598,-29.538673180489));
#42623=CARTESIAN_POINT('Ctrl Pts',(-63.6165016390556,11.8526496677232,-29.663897709431));
#42624=CARTESIAN_POINT('Ctrl Pts',(-63.6164302295526,11.8527912434887,-29.9144197942482));
#42625=CARTESIAN_POINT('Ctrl Pts',(-63.6162516972046,11.8531027923439,-30.3530468480679));
#42626=CARTESIAN_POINT('Ctrl Pts',(-63.6157311073167,11.8539546247715,-31.2309389380913));
#42627=CARTESIAN_POINT('Ctrl Pts',(-63.6148431265873,11.8556795568147,-32.4861989169135));
#42628=CARTESIAN_POINT('Ctrl Pts',(-63.6145935192643,11.8576843350789,-33.7409476810005));
#42629=CARTESIAN_POINT('Ctrl Pts',(-63.6152713142585,11.8592171607395,-34.7431466351753));
#42630=CARTESIAN_POINT('Ctrl Pts',(-63.6159933336223,11.859920622453,-35.2436139868135));
#42631=CARTESIAN_POINT('Ctrl Pts',(-63.6167079047789,11.8604100846371,-35.6196094130991));
#42632=CARTESIAN_POINT('Ctrl Pts',(-63.6172684324702,11.8607237861603,-35.8714646383254));
#42633=CARTESIAN_POINT('Ctrl Pts',(-63.6186752536478,11.861303074395,-36.3743891623664));
#42634=CARTESIAN_POINT('Ctrl Pts',(-63.6217993206522,11.8622275208018,-37.252922343994));
#42635=CARTESIAN_POINT('Ctrl Pts',(-63.6298477047311,11.8639233401363,-39.0049862482332));
#42636=CARTESIAN_POINT('Ctrl Pts',(-63.6371263912388,11.8659636564327,-40.5053058386373));
#42637=CARTESIAN_POINT('Ctrl Pts',(-63.640311572706,11.868849022841,-41.7600215564704));
#42638=CARTESIAN_POINT('Ctrl Pts',(-63.6410215578774,11.8692071894829,-42.1385714134598));
#42639=CARTESIAN_POINT('Ctrl Pts',(-63.6416247968917,11.8690788609008,-42.6409437357382));
#42640=CARTESIAN_POINT('Ctrl Pts',(-63.6420442113358,11.8686913607439,-43.1435505796875));
#42641=CARTESIAN_POINT('Ctrl Pts',(-63.6423057211347,11.8679765546826,-43.7709009231348));
#42642=CARTESIAN_POINT('Ctrl Pts',(-63.642464081799,11.8675775925606,-44.5222452391161));
#42643=CARTESIAN_POINT('Ctrl Pts',(-63.6426880223968,11.8683102916394,-45.1465401450018));
#42644=CARTESIAN_POINT('Ctrl Pts',(-63.6430543735511,11.8699350545023,-45.6446752421376));
#42645=CARTESIAN_POINT('Ctrl Pts',(-63.6434567293027,11.8717768159626,-46.0175343101423));
#42646=CARTESIAN_POINT('Ctrl Pts',(-63.6440198836177,11.8743423734263,-46.3896168324758));
#42647=CARTESIAN_POINT('Ctrl Pts',(-63.6450304489903,11.8788571094554,-46.8845230715641));
#42648=CARTESIAN_POINT('Ctrl Pts',(-63.6461291598736,11.8836364224796,-47.2544375579395));
#42649=CARTESIAN_POINT('Ctrl Pts',(-63.647528478827,11.8895375926054,-47.6237561523055));
#42650=CARTESIAN_POINT('Ctrl Pts',(-63.6485428951208,11.8946411569445,-47.8581835740059));
#42651=CARTESIAN_POINT('Ctrl Pts',(-63.6507219838377,11.9096733665,-48.3398826218171));
#42652=CARTESIAN_POINT('Ctrl Pts',(-63.6549464333906,11.9461278115514,-49.191338394477));
#42653=CARTESIAN_POINT('Ctrl Pts',(-63.6619157754883,12.0151208620817,-50.4459409503195));
#42654=CARTESIAN_POINT('Ctrl Pts',(-63.6717891625091,12.0808794384306,-52.005892033572));
#42655=CARTESIAN_POINT('Ctrl Pts',(-63.6798303075965,12.0806248037229,-53.083496984492));
#42656=CARTESIAN_POINT('Ctrl Pts',(-63.6856537767969,12.0551219416618,-53.7710411485962));
#42657=CARTESIAN_POINT('Ctrl Pts',(-63.6884233195104,12.0382215980599,-54.0767002566206));
#42658=CARTESIAN_POINT('Ctrl Pts',(-63.6946323725045,11.9873734678641,-54.6553408493773));
#42659=CARTESIAN_POINT('Ctrl Pts',(-63.7066933073477,11.8632328948125,-55.6376679014349));
#42660=CARTESIAN_POINT('Ctrl Pts',(-63.7319072425593,11.5456916330798,-57.4458331464746));
#42661=CARTESIAN_POINT('Ctrl Pts',(-63.7447621529028,11.3832837960144,-58.7329792961044));
#42662=CARTESIAN_POINT('Ctrl Pts',(-63.7545613485058,11.4305221025594,-59.4970096797001));
#42663=CARTESIAN_POINT('Ctrl Pts',(-63.7555848923888,11.4381341868878,-59.6102728268609));
#42664=CARTESIAN_POINT('Ctrl Pts',(-63.7576573519843,11.4558255574764,-59.8262552169067));
#42665=CARTESIAN_POINT('Ctrl Pts',(-63.7610798780398,11.4950864058057,-60.2120843422442));
#42666=CARTESIAN_POINT('Ctrl Pts',(-63.7673238661899,11.604340302306,-60.9875841261972));
#42667=CARTESIAN_POINT('Ctrl Pts',(-63.7730478757242,11.7954457433543,-61.8926106059757));
#42668=CARTESIAN_POINT('Ctrl Pts',(-63.7777058427018,12.0418075447461,-62.8071988471768));
#42669=CARTESIAN_POINT('Ctrl Pts',(-63.7800290846894,12.1987823712394,-63.3247601796953));
#42670=CARTESIAN_POINT('Ctrl Pts',(-63.7814988872406,12.3101139836278,-63.6704669069245));
#42671=CARTESIAN_POINT('Ctrl Pts',(-63.7824611602337,12.3860489760023,-63.9011327444094));
#42672=CARTESIAN_POINT('Ctrl Pts',(-63.7834061546104,12.4644205718716,-64.1319021146194));
#42673=CARTESIAN_POINT('Ctrl Pts',(-63.7842226387807,12.534981143384,-64.3339803821948));
#42674=CARTESIAN_POINT('Ctrl Pts',(-63.7846878529151,12.5758403042838,-64.4494769739131));
#42675=CARTESIAN_POINT('Ctrl Pts',(-63.7853865526954,12.6376438717188,-64.6227130283474));
#42676=CARTESIAN_POINT('Ctrl Pts',(-63.7859671043656,12.6902263580769,-64.7671299996233));
#42677=CARTESIAN_POINT('Ctrl Pts',(-63.7869707071906,12.7783127131793,-65.0055749183316));
#42678=CARTESIAN_POINT('Ctrl Pts',(-63.7897023542802,12.8611805287705,-65.2184920273913));
#42679=CARTESIAN_POINT('Ctrl Pts',(-63.7938642659111,13.0504967665102,-65.6685032220532));
#42680=CARTESIAN_POINT('Ctrl Pts',(-63.8006501111802,13.419030367146,-66.4580109154324));
#42681=CARTESIAN_POINT('Ctrl Pts',(-63.8088093151091,14.2991451022795,-68.0969920796353));
#42682=CARTESIAN_POINT('Ctrl Pts',(-63.8061682095631,15.197178338022,-69.5915031348636));
#42683=CARTESIAN_POINT('Ctrl Pts',(-63.8007614617662,15.8286774377953,-70.7929513875053));
#42684=CARTESIAN_POINT('Ctrl Pts',(-63.8012363421957,15.9575632529478,-71.0375054692253));
#42685=CARTESIAN_POINT('Ctrl Pts',(-63.8012020563296,16.2229128823079,-71.5400218089304));
#42686=CARTESIAN_POINT('Ctrl Pts',(-63.8015224371708,16.5529105451709,-72.1627527612785));
#42687=CARTESIAN_POINT('Ctrl Pts',(-63.8016365427922,16.9519606071174,-72.9134384000559));
#42688=CARTESIAN_POINT('Ctrl Pts',(-63.801887531904,17.7514641555769,-74.4139267390471));
#42689=CARTESIAN_POINT('Ctrl Pts',(-63.8018491238696,18.4213494921883,-75.6667656774867));
#42690=CARTESIAN_POINT('Ctrl Pts',(-63.8015849222615,19.3930630603169,-77.4941539578504));
#42691=CARTESIAN_POINT('Ctrl Pts',(-63.8016996598983,19.8287630444859,-78.3134493621658));
#42692=CARTESIAN_POINT('Ctrl Pts',(-63.8016996598979,20.2652846318753,-79.1344270642664));
#42693=CARTESIAN_POINT('Ctrl Pts',(-62.8338151407029,6.8546477540195,24.8297302613622));
#42694=CARTESIAN_POINT('Ctrl Pts',(-62.8340115792225,6.85465323508077,24.7808221078273));
#42695=CARTESIAN_POINT('Ctrl Pts',(-62.8342175601913,6.85465899790165,24.7319145444119));
#42696=CARTESIAN_POINT('Ctrl Pts',(-62.8366511414996,6.85472789486385,24.180965761181));
#42697=CARTESIAN_POINT('Ctrl Pts',(-62.8387162951856,6.85434969833623,23.1764292239802));
#42698=CARTESIAN_POINT('Ctrl Pts',(-62.8436351601958,6.8531811917745,21.1672018319798));
#42699=CARTESIAN_POINT('Ctrl Pts',(-62.8598283586026,6.85366027580704,19.662794087716));
#42700=CARTESIAN_POINT('Ctrl Pts',(-62.8931842631358,6.85683026604056,18.4116172696421));
#42701=CARTESIAN_POINT('Ctrl Pts',(-62.9091943230322,6.85816151222857,17.9069947365679));
#42702=CARTESIAN_POINT('Ctrl Pts',(-62.9493960520515,6.86118423799795,16.9017134160942));
#42703=CARTESIAN_POINT('Ctrl Pts',(-63.0355303640731,6.86776884027254,15.1480772929341));
#42704=CARTESIAN_POINT('Ctrl Pts',(-63.1167830427203,6.87677402886358,13.6519841949253));
#42705=CARTESIAN_POINT('Ctrl Pts',(-63.1668769608044,6.88742580172407,12.4050174992644));
#42706=CARTESIAN_POINT('Ctrl Pts',(-63.1872702187809,6.89236509125422,11.9072337591036));
#42707=CARTESIAN_POINT('Ctrl Pts',(-63.2285708140232,6.90433015335502,10.9099577545617));
#42708=CARTESIAN_POINT('Ctrl Pts',(-63.2791532115687,6.92188623197643,9.66042858869122));
#42709=CARTESIAN_POINT('Ctrl Pts',(-63.3319835707986,6.94309248454624,8.1550995458438));
#42710=CARTESIAN_POINT('Ctrl Pts',(-63.3577200966173,6.95446308247782,7.14685283004719));
#42711=CARTESIAN_POINT('Ctrl Pts',(-63.3695412050602,6.95984072374416,6.5158568507044));
#42712=CARTESIAN_POINT('Ctrl Pts',(-63.3740112364851,6.96194049935772,6.26579931908071));
#42713=CARTESIAN_POINT('Ctrl Pts',(-63.3819402533974,6.96596381357759,5.76417995360215));
#42714=CARTESIAN_POINT('Ctrl Pts',(-63.3931890708294,6.97246277513824,4.88524930960752));
#42715=CARTESIAN_POINT('Ctrl Pts',(-63.4049800456724,6.98320362282675,3.12260412316239));
#42716=CARTESIAN_POINT('Ctrl Pts',(-63.397064949177,6.98692004233924,1.61454048227347));
#42717=CARTESIAN_POINT('Ctrl Pts',(-63.3837705927333,6.98698504325039,0.549557566522543));
#42718=CARTESIAN_POINT('Ctrl Pts',(-63.3823088516265,6.98602192500681,0.400247124524424));
#42719=CARTESIAN_POINT('Ctrl Pts',(-63.379865221235,6.9805549762376,0.11840182408989));
#42720=CARTESIAN_POINT('Ctrl Pts',(-63.376586020454,6.96292688560398,-0.371955668368111));
#42721=CARTESIAN_POINT('Ctrl Pts',(-63.3735372952247,6.92107897807562,-1.04112212290876));
#42722=CARTESIAN_POINT('Ctrl Pts',(-63.3684057548297,6.86309953998232,-1.80275589269775));
#42723=CARTESIAN_POINT('Ctrl Pts',(-63.3552431104083,6.7953694544763,-2.75947712877428));
#42724=CARTESIAN_POINT('Ctrl Pts',(-63.3187759597658,6.76383147787105,-3.8469482611788));
#42725=CARTESIAN_POINT('Ctrl Pts',(-63.2579283717942,6.84104022493431,-4.60512667349721));
#42726=CARTESIAN_POINT('Ctrl Pts',(-63.209633432285,6.93174634857654,-5.05880999706912));
#42727=CARTESIAN_POINT('Ctrl Pts',(-63.1874589389198,6.97222160551015,-5.23775199780588));
#42728=CARTESIAN_POINT('Ctrl Pts',(-63.1324664682631,7.07740834543431,-5.62111870290018));
#42729=CARTESIAN_POINT('Ctrl Pts',(-63.0132710022083,7.32070934558602,-6.34142159100564));
#42730=CARTESIAN_POINT('Ctrl Pts',(-62.8029714049297,7.82089116164816,-7.49528858757482));
#42731=CARTESIAN_POINT('Ctrl Pts',(-62.5937142138828,8.43184828164372,-8.76555145163734));
#42732=CARTESIAN_POINT('Ctrl Pts',(-62.4750153791188,8.86099477492063,-9.71158643825483));
#42733=CARTESIAN_POINT('Ctrl Pts',(-62.4202266875157,9.09858812391573,-10.2697765285665));
#42734=CARTESIAN_POINT('Ctrl Pts',(-62.3980883968512,9.21353757691983,-10.5555636968051));
#42735=CARTESIAN_POINT('Ctrl Pts',(-62.3840055420638,9.29775731001258,-10.772483691087));
#42736=CARTESIAN_POINT('Ctrl Pts',(-62.3807561244255,9.34383584914166,-10.8851100172883));
#42737=CARTESIAN_POINT('Ctrl Pts',(-62.3737895087591,9.44543509673677,-11.1302410859108));
#42738=CARTESIAN_POINT('Ctrl Pts',(-62.3697124507635,9.62728392490675,-11.552595682906));
#42739=CARTESIAN_POINT('Ctrl Pts',(-62.3836776826827,10.0163651883242,-12.4161722919694));
#42740=CARTESIAN_POINT('Ctrl Pts',(-62.4572892794437,10.6025342688307,-13.6872799140626));
#42741=CARTESIAN_POINT('Ctrl Pts',(-62.551144293846,11.0857746927166,-14.9067694176834));
#42742=CARTESIAN_POINT('Ctrl Pts',(-62.6046657741735,11.3546649960417,-15.7588413683948));
#42743=CARTESIAN_POINT('Ctrl Pts',(-62.6360151165037,11.5174995819471,-16.3378357915975));
#42744=CARTESIAN_POINT('Ctrl Pts',(-62.6529197325506,11.6183684103482,-16.7844771132674));
#42745=CARTESIAN_POINT('Ctrl Pts',(-62.661007271049,11.6874564495597,-17.1630785787601));
#42746=CARTESIAN_POINT('Ctrl Pts',(-62.6639773063431,11.7137391607947,-17.3164072826276));
#42747=CARTESIAN_POINT('Ctrl Pts',(-62.6694917572641,11.7590410886046,-17.6187296259618));
#42748=CARTESIAN_POINT('Ctrl Pts',(-62.6742326758448,11.7948232448022,-17.9185801404599));
#42749=CARTESIAN_POINT('Ctrl Pts',(-62.6782132969468,11.8220628977155,-18.214357897131));
#42750=CARTESIAN_POINT('Ctrl Pts',(-62.6803854927335,11.8358204920855,-18.3977662585142));
#42751=CARTESIAN_POINT('Ctrl Pts',(-62.681938094352,11.8449976740084,-18.5434958556949));
#42752=CARTESIAN_POINT('Ctrl Pts',(-62.6830112083581,11.8510066622983,-18.6523195445154));
#42753=CARTESIAN_POINT('Ctrl Pts',(-62.6838310955826,11.8553124749393,-18.7425981540404));
#42754=CARTESIAN_POINT('Ctrl Pts',(-62.6844423537282,11.8583569043954,-18.8145734035056));
#42755=CARTESIAN_POINT('Ctrl Pts',(-62.689399559392,11.8819763640981,-19.4250116413265));
#42756=CARTESIAN_POINT('Ctrl Pts',(-62.6910339248514,11.8589163836346,-20.5480768373031));
#42757=CARTESIAN_POINT('Ctrl Pts',(-62.6815934174645,11.7609615658011,-22.0780145591206));
#42758=CARTESIAN_POINT('Ctrl Pts',(-62.6769185361321,11.721960099837,-23.0149122259586));
#42759=CARTESIAN_POINT('Ctrl Pts',(-62.678123904909,11.7226307795498,-23.5742749277269));
#42760=CARTESIAN_POINT('Ctrl Pts',(-62.6785373306137,11.7228653133253,-23.8323956434533));
#42761=CARTESIAN_POINT('Ctrl Pts',(-62.6791628363596,11.723061351535,-24.328550779212));
#42762=CARTESIAN_POINT('Ctrl Pts',(-62.6797649486642,11.7228301746731,-25.208812019077));
#42763=CARTESIAN_POINT('Ctrl Pts',(-62.6795180509527,11.721354647077,-26.4629723137077));
#42764=CARTESIAN_POINT('Ctrl Pts',(-62.6783663162937,11.719331824033,-27.9721402328826));
#42765=CARTESIAN_POINT('Ctrl Pts',(-62.6776431536264,11.7188561776346,-28.9752162355559));
#42766=CARTESIAN_POINT('Ctrl Pts',(-62.6774118773276,11.7191185710211,-29.5382640782203));
#42767=CARTESIAN_POINT('Ctrl Pts',(-62.6773491361315,11.7191843518876,-29.6634734726559));
#42768=CARTESIAN_POINT('Ctrl Pts',(-62.6771832973685,11.7193464575595,-29.9139158292759));
#42769=CARTESIAN_POINT('Ctrl Pts',(-62.6767974667868,11.7197081187366,-30.3524427022208));
#42770=CARTESIAN_POINT('Ctrl Pts',(-62.6757161266157,11.7207035080354,-31.2301571714372));
#42771=CARTESIAN_POINT('Ctrl Pts',(-62.6737284539109,11.7227420343164,-32.4853003188504));
#42772=CARTESIAN_POINT('Ctrl Pts',(-62.6723076625688,11.7250992605578,-33.7400848304719));
#42773=CARTESIAN_POINT('Ctrl Pts',(-62.6722045970334,11.7268711920779,-34.7423990436705));
#42774=CARTESIAN_POINT('Ctrl Pts',(-62.6726198912039,11.7276862042832,-35.2429609730206));
#42775=CARTESIAN_POINT('Ctrl Pts',(-62.6731482121727,11.7282453287308,-35.6190353193089));
#42776=CARTESIAN_POINT('Ctrl Pts',(-62.6735901991154,11.7286061377335,-35.8708877515963));
#42777=CARTESIAN_POINT('Ctrl Pts',(-62.6747833042721,11.7292760920224,-36.3738371005951));
#42778=CARTESIAN_POINT('Ctrl Pts',(-62.6775891060468,11.7303765850017,-37.252408178439));
#42779=CARTESIAN_POINT('Ctrl Pts',(-62.6851873348145,11.7323848629711,-39.0045498356469));
#42780=CARTESIAN_POINT('Ctrl Pts',(-62.692265882017,11.7347119494115,-40.5049667535654));
#42781=CARTESIAN_POINT('Ctrl Pts',(-62.695239949014,11.7377580254097,-41.7597505042597));
#42782=CARTESIAN_POINT('Ctrl Pts',(-62.6958792593676,11.738157075941,-42.1383079782095));
#42783=CARTESIAN_POINT('Ctrl Pts',(-62.6963815746102,11.7380731186388,-42.6406963780333));
#42784=CARTESIAN_POINT('Ctrl Pts',(-62.6966985552679,11.737727586151,-43.1433206750748));
#42785=CARTESIAN_POINT('Ctrl Pts',(-62.6968346575229,11.7370587036778,-43.770697111739));
#42786=CARTESIAN_POINT('Ctrl Pts',(-62.6968644079167,11.7367064246829,-44.522079902509));
#42787=CARTESIAN_POINT('Ctrl Pts',(-62.6970141184905,11.7374722068428,-45.1464142818122));
#42788=CARTESIAN_POINT('Ctrl Pts',(-62.6973494393679,11.7391167215345,-45.6445807164024));
#42789=CARTESIAN_POINT('Ctrl Pts',(-62.6977450145172,11.7409717862853,-46.0174655577079));
#42790=CARTESIAN_POINT('Ctrl Pts',(-62.6983200753203,11.7435488056649,-46.3895757692737));
#42791=CARTESIAN_POINT('Ctrl Pts',(-62.6993742294946,11.748076964468,-46.884520150013));
#42792=CARTESIAN_POINT('Ctrl Pts',(-62.7005405475063,11.7528632367589,-47.2544690340029));
#42793=CARTESIAN_POINT('Ctrl Pts',(-62.7020348968166,11.7587711374807,-47.6238212726955));
#42794=CARTESIAN_POINT('Ctrl Pts',(-62.7031217210978,11.763879089902,-47.8582798567994));
#42795=CARTESIAN_POINT('Ctrl Pts',(-62.7054764654297,11.7789149464117,-48.3400298774589));
#42796=CARTESIAN_POINT('Ctrl Pts',(-62.7100833225575,11.8153679604299,-49.1915642344275));
#42797=CARTESIAN_POINT('Ctrl Pts',(-62.717777994255,11.8843157202965,-50.4462399295271));
#42798=CARTESIAN_POINT('Ctrl Pts',(-62.7286999205461,11.9500069460353,-52.0062161071989));
#42799=CARTESIAN_POINT('Ctrl Pts',(-62.7374959362373,11.949687036557,-53.0838008351293));
#42800=CARTESIAN_POINT('Ctrl Pts',(-62.7437884983338,11.9241594855834,-53.7713208691149));
#42801=CARTESIAN_POINT('Ctrl Pts',(-62.7467611187832,11.907245159,-54.0769991327927));
#42802=CARTESIAN_POINT('Ctrl Pts',(-62.7534137736499,11.8563715973007,-54.6556565089427));
#42803=CARTESIAN_POINT('Ctrl Pts',(-62.7663322934056,11.7321812678653,-55.6380099133699));
#42804=CARTESIAN_POINT('Ctrl Pts',(-62.7934235036687,11.4145596951018,-57.4461871903748));
#42805=CARTESIAN_POINT('Ctrl Pts',(-62.8077245409834,11.2521219439642,-58.7332604275265));
#42806=CARTESIAN_POINT('Ctrl Pts',(-62.8180691335882,11.2993626248574,-59.4971603992213));
#42807=CARTESIAN_POINT('Ctrl Pts',(-62.8191556956144,11.3069755572714,-59.6104097894527));
#42808=CARTESIAN_POINT('Ctrl Pts',(-62.8213424963917,11.3246688368783,-59.8263651893896));
#42809=CARTESIAN_POINT('Ctrl Pts',(-62.8249355674505,11.3639328404393,-60.2121510219349));
#42810=CARTESIAN_POINT('Ctrl Pts',(-62.8314136747293,11.473195673799,-60.987579835687));
#42811=CARTESIAN_POINT('Ctrl Pts',(-62.8372132869808,11.6643200165725,-61.8925621015889));
#42812=CARTESIAN_POINT('Ctrl Pts',(-62.8418592680993,11.9107132299678,-62.8071417167703));
#42813=CARTESIAN_POINT('Ctrl Pts',(-62.8441621771561,12.067709855702,-63.3247106649581));
#42814=CARTESIAN_POINT('Ctrl Pts',(-62.8456207194592,12.1790564938607,-63.6704269131557));
#42815=CARTESIAN_POINT('Ctrl Pts',(-62.8465765977845,12.2550018209773,-63.9011003893636));
#42816=CARTESIAN_POINT('Ctrl Pts',(-62.8475177340291,12.3333834338942,-64.1318789040432));
#42817=CARTESIAN_POINT('Ctrl Pts',(-62.8483343466319,12.4039529527749,-64.3339667523024));
#42818=CARTESIAN_POINT('Ctrl Pts',(-62.8488008391134,12.4448171722134,-64.4494692201393));
#42819=CARTESIAN_POINT('Ctrl Pts',(-62.8495027592879,12.5066282910488,-64.6227144879154));
#42820=CARTESIAN_POINT('Ctrl Pts',(-62.8500889237322,12.5592167888116,-64.7671399538787));
#42821=CARTESIAN_POINT('Ctrl Pts',(-62.8511068271889,12.6473128402298,-65.0055997389676));
#42822=CARTESIAN_POINT('Ctrl Pts',(-62.8538567398629,12.7301855205883,-65.2185162513763));
#42823=CARTESIAN_POINT('Ctrl Pts',(-62.8580451703127,12.9195124929881,-65.6685342521179));
#42824=CARTESIAN_POINT('Ctrl Pts',(-62.8648618849641,13.2880586636127,-66.4580471169517));
#42825=CARTESIAN_POINT('Ctrl Pts',(-62.8730236038173,14.1681833963552,-68.0970356539531));
#42826=CARTESIAN_POINT('Ctrl Pts',(-62.8703297670018,15.0662044172692,-69.5915446237086));
#42827=CARTESIAN_POINT('Ctrl Pts',(-62.8649073183664,15.6976981063461,-70.7929892612915));
#42828=CARTESIAN_POINT('Ctrl Pts',(-62.8653830676195,15.8265847643315,-71.0375439352764));
#42829=CARTESIAN_POINT('Ctrl Pts',(-62.8653481645824,16.0919347801547,-71.5400606036235));
#42830=CARTESIAN_POINT('Ctrl Pts',(-62.8656690400584,16.4219330456641,-72.1627921270539));
#42831=CARTESIAN_POINT('Ctrl Pts',(-62.8657833950704,16.8209833597187,-72.9134781492287));
#42832=CARTESIAN_POINT('Ctrl Pts',(-62.8660354724408,17.620487045096,-74.4139670314268));
#42833=CARTESIAN_POINT('Ctrl Pts',(-62.8659980621607,18.2903711348304,-75.6668055103832));
#42834=CARTESIAN_POINT('Ctrl Pts',(-62.8657332857691,19.2620837088665,-77.494192794518));
#42835=CARTESIAN_POINT('Ctrl Pts',(-62.8658483368064,19.697783753344,-78.3134884153658));
#42836=CARTESIAN_POINT('Ctrl Pts',(-62.8658483368066,20.1343053407335,-79.1344661174665));
#42837=CARTESIAN_POINT('Ctrl Pts',(-61.1951504763405,6.62458514109144,24.8301509583975));
#42838=CARTESIAN_POINT('Ctrl Pts',(-61.1953568465687,6.62460289413373,24.7812567470511));
#42839=CARTESIAN_POINT('Ctrl Pts',(-61.1955732470009,6.62462155064825,24.7323633371));
#42840=CARTESIAN_POINT('Ctrl Pts',(-61.1981287247375,6.62484065059862,24.1815793110815));
#42841=CARTESIAN_POINT('Ctrl Pts',(-61.2005612044126,6.62486564311747,23.1773121540749));
#42842=CARTESIAN_POINT('Ctrl Pts',(-61.2065292919888,6.624845624491,21.1683493771042));
#42843=CARTESIAN_POINT('Ctrl Pts',(-61.2235178549665,6.62630144191226,19.6639204589936));
#42844=CARTESIAN_POINT('Ctrl Pts',(-61.2571829939099,6.63009485789897,18.4126497901983));
#42845=CARTESIAN_POINT('Ctrl Pts',(-61.2735182517976,6.63178904822752,17.9085919333625));
#42846=CARTESIAN_POINT('Ctrl Pts',(-61.3148582396206,6.63582087133403,16.9037625251246));
#42847=CARTESIAN_POINT('Ctrl Pts',(-61.4034039595603,6.64442515136615,15.1503355737336));
#42848=CARTESIAN_POINT('Ctrl Pts',(-61.4846424691607,6.65419630033967,13.6525696721531));
#42849=CARTESIAN_POINT('Ctrl Pts',(-61.5303696538949,6.66322521494574,12.4030927090508));
#42850=CARTESIAN_POINT('Ctrl Pts',(-61.5484916289262,6.66723912559534,11.9041681631621));
#42851=CARTESIAN_POINT('Ctrl Pts',(-61.5835940410652,6.6764350674265,10.9051885064317));
#42852=CARTESIAN_POINT('Ctrl Pts',(-61.6242295358563,6.68936722404817,9.65433962806701));
#42853=CARTESIAN_POINT('Ctrl Pts',(-61.6643034346199,6.70437569936267,8.14919086030427));
#42854=CARTESIAN_POINT('Ctrl Pts',(-61.6828526508977,6.71238820862013,7.14227280148821));
#42855=CARTESIAN_POINT('Ctrl Pts',(-61.691153893495,6.71622150470251,6.5125725955013));
#42856=CARTESIAN_POINT('Ctrl Pts',(-61.693975656162,6.71774731565301,6.26365110309824));
#42857=CARTESIAN_POINT('Ctrl Pts',(-61.6979000775793,6.72081792898549,5.76357738792179));
#42858=CARTESIAN_POINT('Ctrl Pts',(-61.7007460307582,6.72610541865317,4.88660297529398));
#42859=CARTESIAN_POINT('Ctrl Pts',(-61.6943584373772,6.73552427919849,3.12430421344482));
#42860=CARTESIAN_POINT('Ctrl Pts',(-61.6817135425056,6.73863874741957,1.60931204378402));
#42861=CARTESIAN_POINT('Ctrl Pts',(-61.6813928422738,6.73535180835137,0.537771163006079));
#42862=CARTESIAN_POINT('Ctrl Pts',(-61.6816981518373,6.73411327655994,0.3912714579851));
#42863=CARTESIAN_POINT('Ctrl Pts',(-61.68350649646,6.72869968547698,0.112541836839732));
#42864=CARTESIAN_POINT('Ctrl Pts',(-61.6894870030561,6.71240579224838,-0.372452970662816));
#42865=CARTESIAN_POINT('Ctrl Pts',(-61.7040975329937,6.67465326445107,-1.03804543785192));
#42866=CARTESIAN_POINT('Ctrl Pts',(-61.7253695647143,6.62146645629319,-1.80065539383669));
#42867=CARTESIAN_POINT('Ctrl Pts',(-61.7512793681603,6.55718283441924,-2.76679751972595));
#42868=CARTESIAN_POINT('Ctrl Pts',(-61.7656676096798,6.52083721095943,-3.88195177421976));
#42869=CARTESIAN_POINT('Ctrl Pts',(-61.7289403580524,6.58491345336716,-4.67530859774312));
#42870=CARTESIAN_POINT('Ctrl Pts',(-61.6838248946664,6.66300030427892,-5.14929721479892));
#42871=CARTESIAN_POINT('Ctrl Pts',(-61.6616341867744,6.70028622946335,-5.35061029919009));
#42872=CARTESIAN_POINT('Ctrl Pts',(-61.6045172022772,6.7892304110016,-5.7591672929034));
#42873=CARTESIAN_POINT('Ctrl Pts',(-61.4763898493465,6.98344413109923,-6.50509413113006));
#42874=CARTESIAN_POINT('Ctrl Pts',(-61.2473833659582,7.35409788266046,-7.64876931607059));
#42875=CARTESIAN_POINT('Ctrl Pts',(-61.0314320905569,7.81239046287047,-8.88225427570305));
#42876=CARTESIAN_POINT('Ctrl Pts',(-60.9163069811461,8.15953579844562,-9.77881172773552));
#42877=CARTESIAN_POINT('Ctrl Pts',(-60.8648618014957,8.3625242399895,-10.2991416545444));
#42878=CARTESIAN_POINT('Ctrl Pts',(-60.8446197878516,8.46523082053907,-10.5621314670901));
#42879=CARTESIAN_POINT('Ctrl Pts',(-60.8319172356274,8.54249578079412,-10.7601506448152));
#42880=CARTESIAN_POINT('Ctrl Pts',(-60.8294089355775,8.58445045011968,-10.8601835508611));
#42881=CARTESIAN_POINT('Ctrl Pts',(-60.8233475986099,8.68113721341898,-11.0821155945678));
#42882=CARTESIAN_POINT('Ctrl Pts',(-60.8191264510034,8.8622819506804,-11.4681317840093));
#42883=CARTESIAN_POINT('Ctrl Pts',(-60.825787087303,9.27900712280218,-12.2749049213649));
#42884=CARTESIAN_POINT('Ctrl Pts',(-60.8669206700503,9.97125551368284,-13.500531742468));
#42885=CARTESIAN_POINT('Ctrl Pts',(-60.9181470813914,10.5940713881071,-14.718901355251));
#42886=CARTESIAN_POINT('Ctrl Pts',(-60.9479815065831,10.9531558728833,-15.5960065118785));
#42887=CARTESIAN_POINT('Ctrl Pts',(-60.9654189278638,11.1726665720368,-16.1996779621415));
#42888=CARTESIAN_POINT('Ctrl Pts',(-60.9746669874423,11.3096398470889,-16.6748462364098));
#42889=CARTESIAN_POINT('Ctrl Pts',(-60.9784506935739,11.4013262488943,-17.0829887398642));
#42890=CARTESIAN_POINT('Ctrl Pts',(-60.9801153713349,11.4346064335128,-17.2394831842584));
#42891=CARTESIAN_POINT('Ctrl Pts',(-60.9835406317571,11.493183293384,-17.5530226881813));
#42892=CARTESIAN_POINT('Ctrl Pts',(-60.987154044757,11.5395859846949,-17.8619590869959));
#42893=CARTESIAN_POINT('Ctrl Pts',(-60.9907599742485,11.57555857648,-18.1673057259696));
#42894=CARTESIAN_POINT('Ctrl Pts',(-60.9930021503445,11.5939322244607,-18.3562342522241));
#42895=CARTESIAN_POINT('Ctrl Pts',(-60.9947717812819,11.6063715025536,-18.506301898915));
#42896=CARTESIAN_POINT('Ctrl Pts',(-60.996086104167,11.6146094490627,-18.6182731242901));
#42897=CARTESIAN_POINT('Ctrl Pts',(-60.9971686866792,11.6206033299365,-18.7111110077954));
#42898=CARTESIAN_POINT('Ctrl Pts',(-60.9980252446697,11.6249001658783,-18.7850844415051));
#42899=CARTESIAN_POINT('Ctrl Pts',(-61.0052655975391,11.658615375535,-19.4122754252571));
#42900=CARTESIAN_POINT('Ctrl Pts',(-61.0171580558027,11.6384378193482,-20.5586059913791));
#42901=CARTESIAN_POINT('Ctrl Pts',(-61.0268905636031,11.5302210404426,-22.0960107426974));
#42902=CARTESIAN_POINT('Ctrl Pts',(-61.0308003746837,11.4889047680634,-23.0205296925236));
#42903=CARTESIAN_POINT('Ctrl Pts',(-61.034268841733,11.4915868109434,-23.5669959069628));
#42904=CARTESIAN_POINT('Ctrl Pts',(-61.0354944060958,11.4926254194423,-23.8278637947768));
#42905=CARTESIAN_POINT('Ctrl Pts',(-61.0374774564534,11.4939939440805,-24.3248640057824));
#42906=CARTESIAN_POINT('Ctrl Pts',(-61.0397977550119,11.4949749112046,-25.2083710153304));
#42907=CARTESIAN_POINT('Ctrl Pts',(-61.0404249912444,11.4932218000262,-26.4644076265833));
#42908=CARTESIAN_POINT('Ctrl Pts',(-61.0387164910498,11.4895162222653,-27.9742630599744));
#42909=CARTESIAN_POINT('Ctrl Pts',(-61.0372248727665,11.4881938993359,-28.9760342398299));
#42910=CARTESIAN_POINT('Ctrl Pts',(-61.0366487955333,11.4884173372713,-29.537966544389));
#42911=CARTESIAN_POINT('Ctrl Pts',(-61.0364980446522,11.4884760063778,-29.6632426016537));
#42912=CARTESIAN_POINT('Ctrl Pts',(-61.0361127406127,11.4886160154417,-29.9136400903341));
#42913=CARTESIAN_POINT('Ctrl Pts',(-61.0352348851594,11.4889209698375,-30.3521843141996));
#42914=CARTESIAN_POINT('Ctrl Pts',(-61.0327943604326,11.4897472430984,-31.2298741115997));
#42915=CARTESIAN_POINT('Ctrl Pts',(-61.0280955236478,11.4914170504487,-32.4850496433206));
#42916=CARTESIAN_POINT('Ctrl Pts',(-61.0237560037054,11.4933884105369,-33.7398705006316));
#42917=CARTESIAN_POINT('Ctrl Pts',(-61.0216795012927,11.494928498429,-34.7422088794976));
#42918=CARTESIAN_POINT('Ctrl Pts',(-61.0213039587799,11.4956447572322,-35.2427959475687));
#42919=CARTESIAN_POINT('Ctrl Pts',(-61.0213443437813,11.4961496164705,-35.6188862471038));
#42920=CARTESIAN_POINT('Ctrl Pts',(-61.0214713523777,11.4964756971778,-35.8707395448149));
#42921=CARTESIAN_POINT('Ctrl Pts',(-61.0220817752789,11.4970873720578,-36.3736956800009));
#42922=CARTESIAN_POINT('Ctrl Pts',(-61.0239730980735,11.4980814232848,-37.2522838368669));
#42923=CARTESIAN_POINT('Ctrl Pts',(-61.0301360530368,11.49996694904,-39.0044607649581));
#42924=CARTESIAN_POINT('Ctrl Pts',(-61.0363929751217,11.5021747951859,-40.5049056867621));
#42925=CARTESIAN_POINT('Ctrl Pts',(-61.038688280218,11.5051403709043,-41.7597005904433));
#42926=CARTESIAN_POINT('Ctrl Pts',(-61.0391158413235,11.5055189117883,-42.1382542681091));
#42927=CARTESIAN_POINT('Ctrl Pts',(-61.0393328711263,11.5054108475311,-42.6406427225632));
#42928=CARTESIAN_POINT('Ctrl Pts',(-61.0393667119375,11.5050396412129,-43.143267376347));
#42929=CARTESIAN_POINT('Ctrl Pts',(-61.0391643540375,11.5043394908254,-43.7706474579098));
#42930=CARTESIAN_POINT('Ctrl Pts',(-61.0388463115252,11.5039544201184,-44.522038933998));
#42931=CARTESIAN_POINT('Ctrl Pts',(-61.0387830075111,11.5047001916358,-45.1463845156248));
#42932=CARTESIAN_POINT('Ctrl Pts',(-61.0390122327925,11.5063391844499,-45.6445644550148));
#42933=CARTESIAN_POINT('Ctrl Pts',(-61.0393640958474,11.5081942047304,-46.0174606131328));
#42934=CARTESIAN_POINT('Ctrl Pts',(-61.039935717522,11.5107763740768,-46.389583419531));
#42935=CARTESIAN_POINT('Ctrl Pts',(-61.0410444943961,11.5153183312048,-46.8845472445286));
#42936=CARTESIAN_POINT('Ctrl Pts',(-61.0423253344689,11.5201259784132,-47.2545104306091));
#42937=CARTESIAN_POINT('Ctrl Pts',(-61.0439915921777,11.5260610428822,-47.6238803016604));
#42938=CARTESIAN_POINT('Ctrl Pts',(-61.0452133055278,11.5311901476113,-47.8583558760436));
#42939=CARTESIAN_POINT('Ctrl Pts',(-61.0479070618055,11.5462780632115,-48.3401315118095));
#42940=CARTESIAN_POINT('Ctrl Pts',(-61.0532747093371,11.5828405598515,-49.191698673183));
#42941=CARTESIAN_POINT('Ctrl Pts',(-61.0624582839014,11.6520091930191,-50.4463827362363));
#42942=CARTESIAN_POINT('Ctrl Pts',(-61.0755553226412,11.7179771546967,-52.0063311577792));
#42943=CARTESIAN_POINT('Ctrl Pts',(-61.0859180795864,11.7178710496722,-53.0838827351573));
#42944=CARTESIAN_POINT('Ctrl Pts',(-61.0931759356651,11.6924606284119,-53.7713808569349));
#42945=CARTESIAN_POINT('Ctrl Pts',(-61.0965679740002,11.6755941460017,-54.0770527297992));
#42946=CARTESIAN_POINT('Ctrl Pts',(-61.1041373840954,11.6248246767352,-54.6557013892285));
#42947=CARTESIAN_POINT('Ctrl Pts',(-61.1188310121637,11.5008416036265,-55.6380514548762));
#42948=CARTESIAN_POINT('Ctrl Pts',(-61.1497851147588,11.1836495777128,-57.4462530429054));
#42949=CARTESIAN_POINT('Ctrl Pts',(-61.1670666897246,11.0216150152346,-58.7333503102741));
#42950=CARTESIAN_POINT('Ctrl Pts',(-61.1785196927827,11.0690156598972,-59.4972166156187));
#42951=CARTESIAN_POINT('Ctrl Pts',(-61.1797324035572,11.0766436804769,-59.610460938086));
#42952=CARTESIAN_POINT('Ctrl Pts',(-61.1821470349915,11.0943661075029,-59.826407298789));
#42953=CARTESIAN_POINT('Ctrl Pts',(-61.1860750911724,11.1336747416495,-60.2121792687574));
#42954=CARTESIAN_POINT('Ctrl Pts',(-61.1929940783206,11.2430043968676,-60.9875884813146));
#42955=CARTESIAN_POINT('Ctrl Pts',(-61.1988897348787,11.434166518421,-61.8925697160505));
#42956=CARTESIAN_POINT('Ctrl Pts',(-61.203454845895,11.6805800342668,-62.8071635715259));
#42957=CARTESIAN_POINT('Ctrl Pts',(-61.2056875777563,11.8375844710509,-63.3247444139147));
#42958=CARTESIAN_POINT('Ctrl Pts',(-61.207106559886,11.9489372873714,-63.6704701734733));
#42959=CARTESIAN_POINT('Ctrl Pts',(-61.2080390043346,12.0248867410563,-63.9011501929878));
#42960=CARTESIAN_POINT('Ctrl Pts',(-61.2089631312672,12.1032736056746,-64.1319359786747));
#42961=CARTESIAN_POINT('Ctrl Pts',(-61.2097731523333,12.1738481359528,-64.3340303511605));
#42962=CARTESIAN_POINT('Ctrl Pts',(-61.2102387008837,12.2147154843522,-64.4495366347599));
#42963=CARTESIAN_POINT('Ctrl Pts',(-61.2109422345935,12.2765315348749,-64.6227876819708));
#42964=CARTESIAN_POINT('Ctrl Pts',(-61.2115365416596,12.3291249368404,-64.7672181703169));
#42965=CARTESIAN_POINT('Ctrl Pts',(-61.2125793523105,12.4172299066177,-65.0056862298864));
#42966=CARTESIAN_POINT('Ctrl Pts',(-61.2153652508937,12.5001132674356,-65.218606727214));
#42967=CARTESIAN_POINT('Ctrl Pts',(-61.2196064879568,12.689457605908,-65.6686332701946));
#42968=CARTESIAN_POINT('Ctrl Pts',(-61.2264901285657,13.0580281190058,-66.4581561128385));
#42969=CARTESIAN_POINT('Ctrl Pts',(-61.2346767188754,13.9381728298099,-68.0971536023905));
#42970=CARTESIAN_POINT('Ctrl Pts',(-61.2318869813096,14.8361779057614,-69.5916616377109));
#42971=CARTESIAN_POINT('Ctrl Pts',(-61.2264190170371,15.4676581624523,-70.7931013307634));
#42972=CARTESIAN_POINT('Ctrl Pts',(-61.226897358886,15.5965462230223,-71.0376566986305));
#42973=CARTESIAN_POINT('Ctrl Pts',(-61.2268607544551,15.8618963803404,-71.540173633185));
#42974=CARTESIAN_POINT('Ctrl Pts',(-61.2271831423561,16.191895854752,-72.1629057961627));
#42975=CARTESIAN_POINT('Ctrl Pts',(-61.2272982744814,16.5909466691714,-72.9135921473858));
#42976=CARTESIAN_POINT('Ctrl Pts',(-61.2275535433326,17.3904512539708,-74.414081485479));
#42977=CARTESIAN_POINT('Ctrl Pts',(-61.2275189123817,18.0603357245619,-75.6669197390852));
#42978=CARTESIAN_POINT('Ctrl Pts',(-61.2272523446541,19.0320477916089,-77.4943063972569));
#42979=CARTESIAN_POINT('Ctrl Pts',(-61.2273683371954,19.4677484205143,-78.3136022825405));
#42980=CARTESIAN_POINT('Ctrl Pts',(-61.2273683371965,19.9042700079039,-79.1345799846401));
#42981=CARTESIAN_POINT('Ctrl Pts',(-58.8531122166346,6.29125272644766,24.8311203649996));
#42982=CARTESIAN_POINT('Ctrl Pts',(-58.8532961937455,6.29129086286412,24.7822564017764));
#42983=CARTESIAN_POINT('Ctrl Pts',(-58.8534891349777,6.29133083864146,24.7333938104296));
#42984=CARTESIAN_POINT('Ctrl Pts',(-58.8557674938895,6.29180286160571,24.1829644323862));
#42985=CARTESIAN_POINT('Ctrl Pts',(-58.8576561439393,6.29245164919413,23.1790663946222));
#42986=CARTESIAN_POINT('Ctrl Pts',(-58.8621437037072,6.29414891037338,21.1707766206951));
#42987=CARTESIAN_POINT('Ctrl Pts',(-58.8773005334509,6.29727974088763,19.6666102910973));
#42988=CARTESIAN_POINT('Ctrl Pts',(-58.9087343097988,6.30248678381129,18.4155063967086));
#42989=CARTESIAN_POINT('Ctrl Pts',(-58.9239208629026,6.30506753822643,17.9134491475579));
#42990=CARTESIAN_POINT('Ctrl Pts',(-58.9622603778399,6.31167889478455,16.9100151317855));
#42991=CARTESIAN_POINT('Ctrl Pts',(-59.0445014771969,6.32575615580128,15.156267729807));
#42992=CARTESIAN_POINT('Ctrl Pts',(-59.121227022368,6.33770163219755,13.6520274439723));
#42993=CARTESIAN_POINT('Ctrl Pts',(-59.1666781482765,6.34266844612933,12.3942057487324));
#42994=CARTESIAN_POINT('Ctrl Pts',(-59.1849569030176,6.34440140556946,11.8918622480249));
#42995=CARTESIAN_POINT('Ctrl Pts',(-59.2212603198012,6.34698803383082,10.887944920771));
#42996=CARTESIAN_POINT('Ctrl Pts',(-59.264744899169,6.34880576241689,9.63375633357624));
#42997=CARTESIAN_POINT('Ctrl Pts',(-59.309280904769,6.34943935722079,8.1292838841226));
#42998=CARTESIAN_POINT('Ctrl Pts',(-59.33080531134,6.3492938089834,7.12580691947219));
#42999=CARTESIAN_POINT('Ctrl Pts',(-59.3407250943735,6.34917190545594,6.49905229246299));
#43000=CARTESIAN_POINT('Ctrl Pts',(-59.344257855347,6.34902412143873,6.24814730896979));
#43001=CARTESIAN_POINT('Ctrl Pts',(-59.3497871505297,6.34837358937043,5.74656716465428));
#43002=CARTESIAN_POINT('Ctrl Pts',(-59.3558335964775,6.34644962358975,4.86753800339333));
#43003=CARTESIAN_POINT('Ctrl Pts',(-59.3564368234274,6.3407682801717,3.10841465155978));
#43004=CARTESIAN_POINT('Ctrl Pts',(-59.3481217387933,6.33680373878316,1.6064410335573));
#43005=CARTESIAN_POINT('Ctrl Pts',(-59.3485867412118,6.33898133936188,0.550249730022763));
#43006=CARTESIAN_POINT('Ctrl Pts',(-59.3488632899375,6.3388493940282,0.412544918647314));
#43007=CARTESIAN_POINT('Ctrl Pts',(-59.3502551323157,6.33706032033583,0.146038796302226));
#43008=CARTESIAN_POINT('Ctrl Pts',(-59.354636133616,6.33045187856548,-0.318799356198402));
#43009=CARTESIAN_POINT('Ctrl Pts',(-59.365101533094,6.31366265886565,-0.966398103144115));
#43010=CARTESIAN_POINT('Ctrl Pts',(-59.3800454526428,6.28976423518019,-1.72136052089009));
#43011=CARTESIAN_POINT('Ctrl Pts',(-59.3975400810526,6.26260085226075,-2.69704581639326));
#43012=CARTESIAN_POINT('Ctrl Pts',(-59.40450084396,6.2551724004228,-3.86020427199859));
#43013=CARTESIAN_POINT('Ctrl Pts',(-59.3732913183919,6.3105225319854,-4.7330162397558));
#43014=CARTESIAN_POINT('Ctrl Pts',(-59.3363236294509,6.3728634900837,-5.26471278144059));
#43015=CARTESIAN_POINT('Ctrl Pts',(-59.3183051330271,6.40277469599597,-5.50590057745168));
#43016=CARTESIAN_POINT('Ctrl Pts',(-59.2730143834109,6.46462282018107,-5.97073531772149));
#43017=CARTESIAN_POINT('Ctrl Pts',(-59.1724437406644,6.58512407701506,-6.78935181889418));
#43018=CARTESIAN_POINT('Ctrl Pts',(-58.9912299422981,6.78668033438211,-7.94607044258143));
#43019=CARTESIAN_POINT('Ctrl Pts',(-58.8223505883216,7.04768916551194,-9.1021062641336));
#43020=CARTESIAN_POINT('Ctrl Pts',(-58.7357216700054,7.28298798145105,-9.90635334776788));
#43021=CARTESIAN_POINT('Ctrl Pts',(-58.6977514493031,7.43538440915907,-10.3634137229407));
#43022=CARTESIAN_POINT('Ctrl Pts',(-58.6830441212754,7.51808105230493,-10.5911200580965));
#43023=CARTESIAN_POINT('Ctrl Pts',(-58.6738673485026,7.58258871876441,-10.7612008946215));
#43024=CARTESIAN_POINT('Ctrl Pts',(-58.6723385105303,7.61730140285522,-10.8454011907547));
#43025=CARTESIAN_POINT('Ctrl Pts',(-58.6676698986058,7.70231098946049,-11.0380112045874));
#43026=CARTESIAN_POINT('Ctrl Pts',(-58.6622822535284,7.87155800820933,-11.3815799766734));
#43027=CARTESIAN_POINT('Ctrl Pts',(-58.6531466112637,8.29798633581786,-12.130872232531));
#43028=CARTESIAN_POINT('Ctrl Pts',(-58.6342749136415,9.08897227873553,-13.3224838570275));
#43029=CARTESIAN_POINT('Ctrl Pts',(-58.6087950344317,9.85805749859873,-14.533148519742));
#43030=CARTESIAN_POINT('Ctrl Pts',(-58.5920541257189,10.3189466513491,-15.4242509616649));
#43031=CARTESIAN_POINT('Ctrl Pts',(-58.5811013201179,10.605186759511,-16.0451898751326));
#43032=CARTESIAN_POINT('Ctrl Pts',(-58.573432142254,10.7884568267168,-16.5447992998918));
#43033=CARTESIAN_POINT('Ctrl Pts',(-58.5676883080846,10.9110470070739,-16.9819084772538));
#43034=CARTESIAN_POINT('Ctrl Pts',(-58.5665924615939,10.9530157283704,-17.1389394785022));
#43035=CARTESIAN_POINT('Ctrl Pts',(-58.565186039239,11.0297212299339,-17.4603156750021));
#43036=CARTESIAN_POINT('Ctrl Pts',(-58.5657292503271,11.0918059668326,-17.775045312381));
#43037=CARTESIAN_POINT('Ctrl Pts',(-58.567631299581,11.1421440428145,-18.0875252669167));
#43038=CARTESIAN_POINT('Ctrl Pts',(-58.5693893143105,11.1687320979712,-18.2806147809453));
#43039=CARTESIAN_POINT('Ctrl Pts',(-58.5710784518379,11.1873827163689,-18.4340835752316));
#43040=CARTESIAN_POINT('Ctrl Pts',(-58.5724843464094,11.200079791777,-18.5485545419872));
#43041=CARTESIAN_POINT('Ctrl Pts',(-58.5737628074572,11.209637864024,-18.6434639623201));
#43042=CARTESIAN_POINT('Ctrl Pts',(-58.5748447036218,11.2166942132934,-18.7190720981452));
#43043=CARTESIAN_POINT('Ctrl Pts',(-58.5843889835097,11.2733702537564,-19.3600989807476));
#43044=CARTESIAN_POINT('Ctrl Pts',(-58.6122679980678,11.2811842135818,-20.5287343569894));
#43045=CARTESIAN_POINT('Ctrl Pts',(-58.6549092938124,11.1939846227444,-22.0800671830156));
#43046=CARTESIAN_POINT('Ctrl Pts',(-58.6746892880707,11.1633058977298,-23.002056987914));
#43047=CARTESIAN_POINT('Ctrl Pts',(-58.6822095587603,11.1727610649111,-23.5434804899239));
#43048=CARTESIAN_POINT('Ctrl Pts',(-58.684825910602,11.1767772453322,-23.8089158323289));
#43049=CARTESIAN_POINT('Ctrl Pts',(-58.68921806134,11.1825691191453,-24.3107277047849));
#43050=CARTESIAN_POINT('Ctrl Pts',(-58.6946743015338,11.1886601066525,-25.2031527090417));
#43051=CARTESIAN_POINT('Ctrl Pts',(-58.6972904418314,11.1878390504411,-26.4667907242899));
#43052=CARTESIAN_POINT('Ctrl Pts',(-58.695550935967,11.1802721927887,-27.9803331897321));
#43053=CARTESIAN_POINT('Ctrl Pts',(-58.6934375254854,11.1762187286891,-28.9803097901365));
#43054=CARTESIAN_POINT('Ctrl Pts',(-58.6926044024015,11.1757358086309,-29.5402059986131));
#43055=CARTESIAN_POINT('Ctrl Pts',(-58.6923786527866,11.175608118668,-29.6661970306196));
#43056=CARTESIAN_POINT('Ctrl Pts',(-58.691777738781,11.1752918400781,-29.9173102175387));
#43057=CARTESIAN_POINT('Ctrl Pts',(-58.6903597777594,11.1745838716585,-30.3573160737653));
#43058=CARTESIAN_POINT('Ctrl Pts',(-58.6862628275566,11.1726237782499,-31.2371633439593));
#43059=CARTESIAN_POINT('Ctrl Pts',(-58.6779893478998,11.1687102067029,-32.4941329293564));
#43060=CARTESIAN_POINT('Ctrl Pts',(-58.6696472868024,11.1644713794661,-33.7487245447044));
#43061=CARTESIAN_POINT('Ctrl Pts',(-58.6648294286161,11.1616084609084,-34.7497194105669));
#43062=CARTESIAN_POINT('Ctrl Pts',(-58.6633592706326,11.1604912904934,-35.2492446389077));
#43063=CARTESIAN_POINT('Ctrl Pts',(-58.6627234813872,11.1598108101496,-35.6244021496755));
#43064=CARTESIAN_POINT('Ctrl Pts',(-58.6624116018931,11.1593550428197,-35.876299419224));
#43065=CARTESIAN_POINT('Ctrl Pts',(-58.6621968791146,11.1584502265351,-36.3789602469091));
#43066=CARTESIAN_POINT('Ctrl Pts',(-58.6627792456753,11.1569364021083,-37.2572338064125));
#43067=CARTESIAN_POINT('Ctrl Pts',(-58.666775291758,11.1543027159659,-39.0085851302233));
#43068=CARTESIAN_POINT('Ctrl Pts',(-58.6717281129795,11.1535635448823,-40.5083721509013));
#43069=CARTESIAN_POINT('Ctrl Pts',(-58.6729665323629,11.1545275425125,-41.7625315481145));
#43070=CARTESIAN_POINT('Ctrl Pts',(-58.6730633843322,11.1543158533502,-42.1409928886693));
#43071=CARTESIAN_POINT('Ctrl Pts',(-58.6728300965074,11.1534692046473,-42.6431728214892));
#43072=CARTESIAN_POINT('Ctrl Pts',(-58.672416217241,11.152397036243,-43.145586346829));
#43073=CARTESIAN_POINT('Ctrl Pts',(-58.6716732984394,11.1509008480668,-43.7726642904261));
#43074=CARTESIAN_POINT('Ctrl Pts',(-58.6707842528653,11.1497187299375,-44.5236476183902));
#43075=CARTESIAN_POINT('Ctrl Pts',(-58.6703490091193,11.1499572785657,-45.1476122395524));
#43076=CARTESIAN_POINT('Ctrl Pts',(-58.6703668830272,11.1512972489388,-45.6454579126515));
#43077=CARTESIAN_POINT('Ctrl Pts',(-58.6706090718571,11.1529859202588,-46.0180910572761));
#43078=CARTESIAN_POINT('Ctrl Pts',(-58.6711257361361,11.1554629271224,-46.3899382025871));
#43079=CARTESIAN_POINT('Ctrl Pts',(-58.6722425500054,11.1599519212778,-46.8845154608703));
#43080=CARTESIAN_POINT('Ctrl Pts',(-58.6736282575498,11.1648205689537,-47.2541720644948));
#43081=CARTESIAN_POINT('Ctrl Pts',(-58.6754793287284,11.1708942736337,-47.6232145606296));
#43082=CARTESIAN_POINT('Ctrl Pts',(-58.6768511114755,11.1761435241196,-47.8573713658892));
#43083=CARTESIAN_POINT('Ctrl Pts',(-58.6799285636696,11.1915943224041,-48.3386218652533));
#43084=CARTESIAN_POINT('Ctrl Pts',(-58.6861752653204,11.2290893717988,-49.1893687745462));
#43085=CARTESIAN_POINT('Ctrl Pts',(-58.697103456101,11.3002976745431,-50.4432603072607));
#43086=CARTESIAN_POINT('Ctrl Pts',(-58.7128525538229,11.3694293772098,-52.0028309595));
#43087=CARTESIAN_POINT('Ctrl Pts',(-58.7252359840649,11.3714960879605,-53.0805742291338));
#43088=CARTESIAN_POINT('Ctrl Pts',(-58.7338122345408,11.3473454802483,-53.7683279890051));
#43089=CARTESIAN_POINT('Ctrl Pts',(-58.7377772621395,11.3310806389284,-54.0736961880198));
#43090=CARTESIAN_POINT('Ctrl Pts',(-58.7466365080233,11.2815592954844,-54.6520733062992));
#43091=CARTESIAN_POINT('Ctrl Pts',(-58.7638898698218,11.1598900367289,-55.6340505101549));
#43092=CARTESIAN_POINT('Ctrl Pts',(-58.8006108123127,10.8473623013647,-57.4422974072245));
#43093=CARTESIAN_POINT('Ctrl Pts',(-58.8224914382479,10.6879749092258,-58.7303365344381));
#43094=CARTESIAN_POINT('Ctrl Pts',(-58.835594620721,10.7363280185413,-59.4957081676448));
#43095=CARTESIAN_POINT('Ctrl Pts',(-58.836993637099,10.74408270014,-59.6091141407841));
#43096=CARTESIAN_POINT('Ctrl Pts',(-58.8397436281837,10.7620211453917,-59.8253766905018));
#43097=CARTESIAN_POINT('Ctrl Pts',(-58.8441588137794,10.8016412372195,-60.211651793111));
#43098=CARTESIAN_POINT('Ctrl Pts',(-58.8516989619916,10.9113266438308,-60.9878888234346));
#43099=CARTESIAN_POINT('Ctrl Pts',(-58.857685494782,11.1023842020238,-61.8934033624564));
#43100=CARTESIAN_POINT('Ctrl Pts',(-58.8620921377479,11.3484146029664,-62.8081655158882));
#43101=CARTESIAN_POINT('Ctrl Pts',(-58.864207460578,11.5051532444805,-63.3257123652384));
#43102=CARTESIAN_POINT('Ctrl Pts',(-58.8655630123144,11.6163287818732,-63.6713635074078));
#43103=CARTESIAN_POINT('Ctrl Pts',(-58.8664588288894,11.6921620009195,-63.9019800687117));
#43104=CARTESIAN_POINT('Ctrl Pts',(-58.8673574433335,11.7704370207402,-64.132681988696));
#43105=CARTESIAN_POINT('Ctrl Pts',(-58.8681593124706,11.8409222518968,-64.3346849727148));
#43106=CARTESIAN_POINT('Ctrl Pts',(-58.8686248863825,11.8817415053248,-64.4501338510522));
#43107=CARTESIAN_POINT('Ctrl Pts',(-58.8693334710135,11.9434887627976,-64.6232937862657));
#43108=CARTESIAN_POINT('Ctrl Pts',(-58.8699430590789,11.9960318969489,-64.7676371916027));
#43109=CARTESIAN_POINT('Ctrl Pts',(-58.871029597124,12.0840685274892,-65.0059504080628));
#43110=CARTESIAN_POINT('Ctrl Pts',(-58.8738720353503,12.1669625240645,-65.2189057880762));
#43111=CARTESIAN_POINT('Ctrl Pts',(-58.8782013908965,12.3562848247715,-65.6688933557686));
#43112=CARTESIAN_POINT('Ctrl Pts',(-58.8852010805029,12.7248446653879,-66.4584080929237));
#43113=CARTESIAN_POINT('Ctrl Pts',(-58.8934536686832,13.6049626308997,-68.0973591656563));
#43114=CARTESIAN_POINT('Ctrl Pts',(-58.890514373704,14.5029599787097,-69.5918846190804));
#43115=CARTESIAN_POINT('Ctrl Pts',(-58.8849533524291,15.1344094051463,-70.7933411325163));
#43116=CARTESIAN_POINT('Ctrl Pts',(-58.8854371813811,15.2632950509403,-71.0378928237048));
#43117=CARTESIAN_POINT('Ctrl Pts',(-58.8853973597922,15.5286395211488,-71.5404069143742));
#43118=CARTESIAN_POINT('Ctrl Pts',(-58.8857230037312,15.8586354644087,-72.1631350728754));
#43119=CARTESIAN_POINT('Ctrl Pts',(-58.885839920841,16.2576846620882,-72.9138181502591));
#43120=CARTESIAN_POINT('Ctrl Pts',(-58.8861019161312,17.0571910976897,-74.4143027371218));
#43121=CARTESIAN_POINT('Ctrl Pts',(-58.88607217105,17.727083913447,-75.667144537146));
#43122=CARTESIAN_POINT('Ctrl Pts',(-58.8858010083843,18.6987988142781,-77.4945400537225));
#43123=CARTESIAN_POINT('Ctrl Pts',(-58.8859188984952,19.1344987773697,-78.3138342787722));
#43124=CARTESIAN_POINT('Ctrl Pts',(-58.8859188984958,19.5710203647592,-79.1348119808692));
#43125=CARTESIAN_POINT('Ctrl Pts',(-56.0538590718158,5.89164146497962,24.8309570990425));
#43126=CARTESIAN_POINT('Ctrl Pts',(-56.0540143435333,5.89167115080391,24.7820881194473));
#43127=CARTESIAN_POINT('Ctrl Pts',(-56.0541771996283,5.89170228701854,24.7332204878178));
#43128=CARTESIAN_POINT('Ctrl Pts',(-56.0561007201811,5.89206946163348,24.1827303638316));
#43129=CARTESIAN_POINT('Ctrl Pts',(-56.0573372933614,5.89246395895494,23.1786704198053));
#43130=CARTESIAN_POINT('Ctrl Pts',(-56.0600560331059,5.89346177619444,21.170311115581));
#43131=CARTESIAN_POINT('Ctrl Pts',(-56.0728696004135,5.89589831524976,19.6662389302259));
#43132=CARTESIAN_POINT('Ctrl Pts',(-56.1012331131985,5.9004995024897,18.4152736671248));
#43133=CARTESIAN_POINT('Ctrl Pts',(-56.1147456695187,5.90278092892602,17.91322278237));
#43134=CARTESIAN_POINT('Ctrl Pts',(-56.1485274863742,5.90865048676361,16.909741050075));
#43135=CARTESIAN_POINT('Ctrl Pts',(-56.2210518374978,5.92123437931685,15.1557159402556));
#43136=CARTESIAN_POINT('Ctrl Pts',(-56.291361507408,5.93222838507849,13.6513443862109));
#43137=CARTESIAN_POINT('Ctrl Pts',(-56.3379466536074,5.93725400977883,12.3936626189808));
#43138=CARTESIAN_POINT('Ctrl Pts',(-56.3572553596225,5.93910149189236,11.8914224813623));
#43139=CARTESIAN_POINT('Ctrl Pts',(-56.397483859715,5.94219627272114,10.8877548182249));
#43140=CARTESIAN_POINT('Ctrl Pts',(-56.4485258936853,5.94505574783066,9.63391126524183));
#43141=CARTESIAN_POINT('Ctrl Pts',(-56.5037743046481,5.94707303303974,8.12966173762822));
#43142=CARTESIAN_POINT('Ctrl Pts',(-56.5317925643883,5.94767327443603,7.1260044365657));
#43143=CARTESIAN_POINT('Ctrl Pts',(-56.5450396626367,5.94786054042254,6.49901900310903));
#43144=CARTESIAN_POINT('Ctrl Pts',(-56.5500709620272,5.94782861036557,6.24784413173467));
#43145=CARTESIAN_POINT('Ctrl Pts',(-56.5591807391264,5.94742917467341,5.74591614945796));
#43146=CARTESIAN_POINT('Ctrl Pts',(-56.5726632237092,5.94597989349818,4.86635060028145));
#43147=CARTESIAN_POINT('Ctrl Pts',(-56.5901175188842,5.94129391697758,3.10695664261026));
#43148=CARTESIAN_POINT('Ctrl Pts',(-56.5898844598564,5.93815909136145,1.6053077669838));
#43149=CARTESIAN_POINT('Ctrl Pts',(-56.5833252757848,5.94003526968791,0.551394948598051));
#43150=CARTESIAN_POINT('Ctrl Pts',(-56.5825457545805,5.94003663591684,0.41880487008954));
#43151=CARTESIAN_POINT('Ctrl Pts',(-56.580982321595,5.93914199528337,0.158963928055661));
#43152=CARTESIAN_POINT('Ctrl Pts',(-56.5781752073396,5.93553475454912,-0.294696734365856));
#43153=CARTESIAN_POINT('Ctrl Pts',(-56.5736488125126,5.92602527432297,-0.932811606764838));
#43154=CARTESIAN_POINT('Ctrl Pts',(-56.5663733399661,5.91247012088004,-1.68504842023479));
#43155=CARTESIAN_POINT('Ctrl Pts',(-56.5529361709947,5.89741962355672,-2.67010185783887));
#43156=CARTESIAN_POINT('Ctrl Pts',(-56.5267030388217,5.89541906210424,-3.86922662353056));
#43157=CARTESIAN_POINT('Ctrl Pts',(-56.4904512572469,5.93200810912679,-4.7959249042925));
#43158=CARTESIAN_POINT('Ctrl Pts',(-56.4616453953466,5.97256296933579,-5.36841310784015));
#43159=CARTESIAN_POINT('Ctrl Pts',(-56.448551598945,5.99074380499537,-5.63975167835125));
#43160=CARTESIAN_POINT('Ctrl Pts',(-56.4190493601774,6.02058827887102,-6.14839873414667));
#43161=CARTESIAN_POINT('Ctrl Pts',(-56.3591263483878,6.06667792792076,-7.0278626699762));
#43162=CARTESIAN_POINT('Ctrl Pts',(-56.2580117170356,6.13756571361465,-8.20757162092261));
#43163=CARTESIAN_POINT('Ctrl Pts',(-56.1585687663277,6.27717431418544,-9.30115919905004));
#43164=CARTESIAN_POINT('Ctrl Pts',(-56.1031354938693,6.44040154776427,-10.0253960678308));
#43165=CARTESIAN_POINT('Ctrl Pts',(-56.0771896455893,6.55680114801948,-10.4300530054078));
#43166=CARTESIAN_POINT('Ctrl Pts',(-56.0663161167364,6.62353155550022,-10.6298104366514));
#43167=CARTESIAN_POINT('Ctrl Pts',(-56.0590770993462,6.67697368336153,-10.778573282487));
#43168=CARTESIAN_POINT('Ctrl Pts',(-56.0571992136534,6.70559636921108,-10.8520132861725));
#43169=CARTESIAN_POINT('Ctrl Pts',(-56.0515005149677,6.77917284717286,-11.0244204407004));
#43170=CARTESIAN_POINT('Ctrl Pts',(-56.0411345716577,6.93305537747737,-11.340343791566));
#43171=CARTESIAN_POINT('Ctrl Pts',(-56.011914768945,7.34958690420016,-12.0562955055699));
#43172=CARTESIAN_POINT('Ctrl Pts',(-55.9424747216657,8.1862460486787,-13.2319041224142));
#43173=CARTESIAN_POINT('Ctrl Pts',(-55.8608597038884,9.03453486786773,-14.4337444050702));
#43174=CARTESIAN_POINT('Ctrl Pts',(-55.8079568363992,9.55318525252669,-15.3235500042448));
#43175=CARTESIAN_POINT('Ctrl Pts',(-55.7740504317906,9.87883708879492,-15.9463018801817));
#43176=CARTESIAN_POINT('Ctrl Pts',(-55.7512662410359,10.0920056554103,-16.4518960126066));
#43177=CARTESIAN_POINT('Ctrl Pts',(-55.7359220297285,10.2374525790615,-16.8987888302202));
#43178=CARTESIAN_POINT('Ctrl Pts',(-55.7320689232897,10.2852545852319,-17.0517748945108));
#43179=CARTESIAN_POINT('Ctrl Pts',(-55.7251193981875,10.3761163494362,-17.3701681813707));
#43180=CARTESIAN_POINT('Ctrl Pts',(-55.7210961407007,10.4523015685782,-17.6808831787287));
#43181=CARTESIAN_POINT('Ctrl Pts',(-55.7191029346574,10.5175678738284,-17.9910276878221));
#43182=CARTESIAN_POINT('Ctrl Pts',(-55.7187684585226,10.5535306604547,-18.182771202428));
#43183=CARTESIAN_POINT('Ctrl Pts',(-55.7189610221274,10.5797643459227,-18.3354326496423));
#43184=CARTESIAN_POINT('Ctrl Pts',(-55.7193386864896,10.5981575542272,-18.4493730759027));
#43185=CARTESIAN_POINT('Ctrl Pts',(-55.719834105721,10.6124749611974,-18.5439261461873));
#43186=CARTESIAN_POINT('Ctrl Pts',(-55.7203345737224,10.6233387493865,-18.6192936042957));
#43187=CARTESIAN_POINT('Ctrl Pts',(-55.7251713925168,10.7123963481415,-19.2585240944519));
#43188=CARTESIAN_POINT('Ctrl Pts',(-55.7520250218645,10.7813072911956,-20.4319694878879));
#43189=CARTESIAN_POINT('Ctrl Pts',(-55.8032254818595,10.7625487878085,-22.0034771657111));
#43190=CARTESIAN_POINT('Ctrl Pts',(-55.8263661739389,10.7595625294605,-22.9457268569596));
#43191=CARTESIAN_POINT('Ctrl Pts',(-55.8329419755844,10.7812272868954,-23.5027977642127));
#43192=CARTESIAN_POINT('Ctrl Pts',(-55.8350007170921,10.7905800865703,-23.7745956206071));
#43193=CARTESIAN_POINT('Ctrl Pts',(-55.838224518375,10.8040442653164,-24.2876942535255));
#43194=CARTESIAN_POINT('Ctrl Pts',(-55.8413588798641,10.8183584472778,-25.1969624136924));
#43195=CARTESIAN_POINT('Ctrl Pts',(-55.8404949232791,10.8167877909337,-26.4759728986782));
#43196=CARTESIAN_POINT('Ctrl Pts',(-55.8360405173551,10.7998738602452,-27.9942653201028));
#43197=CARTESIAN_POINT('Ctrl Pts',(-55.8344655777984,10.7909493984571,-28.9881204599642));
#43198=CARTESIAN_POINT('Ctrl Pts',(-55.8350322006705,10.7900532279127,-29.5421574820583));
#43199=CARTESIAN_POINT('Ctrl Pts',(-55.8351543195557,10.7898179947142,-29.66907839006));
#43200=CARTESIAN_POINT('Ctrl Pts',(-55.8353793832605,10.7892186923991,-29.9207420642163));
#43201=CARTESIAN_POINT('Ctrl Pts',(-55.8357305677563,10.7878514107045,-30.3622249830816));
#43202=CARTESIAN_POINT('Ctrl Pts',(-55.8363226938693,10.7839957883729,-31.2440641162283));
#43203=CARTESIAN_POINT('Ctrl Pts',(-55.8371669269615,10.7762250372598,-32.502826336033));
#43204=CARTESIAN_POINT('Ctrl Pts',(-55.8388591106586,10.7678234114254,-33.7572186189596));
#43205=CARTESIAN_POINT('Ctrl Pts',(-55.841226804019,10.7620937741947,-34.7569628628096));
#43206=CARTESIAN_POINT('Ctrl Pts',(-55.8428227877759,10.7598001050066,-35.2554687285961));
#43207=CARTESIAN_POINT('Ctrl Pts',(-55.8442140874073,10.7583625563017,-35.6297323528476));
#43208=CARTESIAN_POINT('Ctrl Pts',(-55.8452512129642,10.7574031974616,-35.8816814900035));
#43209=CARTESIAN_POINT('Ctrl Pts',(-55.8476911991255,10.7555251923315,-36.3840681381157));
#43210=CARTESIAN_POINT('Ctrl Pts',(-55.8527753048416,10.7524095571393,-37.2620392783869));
#43211=CARTESIAN_POINT('Ctrl Pts',(-55.8651535433563,10.7468967612603,-39.012576118021));
#43212=CARTESIAN_POINT('Ctrl Pts',(-55.8758018000701,10.7443314436968,-40.5116970211463));
#43213=CARTESIAN_POINT('Ctrl Pts',(-55.8805818189657,10.7440559669415,-41.7652700730797));
#43214=CARTESIAN_POINT('Ctrl Pts',(-55.8816707004699,10.7434755783443,-42.1436749828539));
#43215=CARTESIAN_POINT('Ctrl Pts',(-55.8826253981071,10.742166861845,-42.6456815044681));
#43216=CARTESIAN_POINT('Ctrl Pts',(-55.883307740908,10.7406566540061,-43.1479163674791));
#43217=CARTESIAN_POINT('Ctrl Pts',(-55.8837622543073,10.7386623652207,-43.7747218600627));
#43218=CARTESIAN_POINT('Ctrl Pts',(-55.8840300940209,10.736978965313,-44.5253121513578));
#43219=CARTESIAN_POINT('Ctrl Pts',(-55.8843226463286,10.7368944092536,-45.1488873604603));
#43220=CARTESIAN_POINT('Ctrl Pts',(-55.8847786975065,10.7380347093961,-45.6463822046966));
#43221=CARTESIAN_POINT('Ctrl Pts',(-55.8852774009959,10.7396076611498,-46.0187333172631));
#43222=CARTESIAN_POINT('Ctrl Pts',(-55.8859781309581,10.742004341543,-46.3902795861577));
#43223=CARTESIAN_POINT('Ctrl Pts',(-55.8872418727823,10.7464351107409,-46.8844296309421));
#43224=CARTESIAN_POINT('Ctrl Pts',(-55.8886304800328,10.7513204207975,-47.2537390824915));
#43225=CARTESIAN_POINT('Ctrl Pts',(-55.8904071186326,10.7574518725442,-47.6224112719319));
#43226=CARTESIAN_POINT('Ctrl Pts',(-55.8916719305651,10.7627479026435,-47.8562235296186));
#43227=CARTESIAN_POINT('Ctrl Pts',(-55.8943472510965,10.7783554968543,-48.3369101694879));
#43228=CARTESIAN_POINT('Ctrl Pts',(-55.8994494045695,10.8162811003826,-49.1868020971753));
#43229=CARTESIAN_POINT('Ctrl Pts',(-55.9078479682809,10.8885388182956,-50.4399472811988));
#43230=CARTESIAN_POINT('Ctrl Pts',(-55.9200980636677,10.9594740604823,-51.999272177031));
#43231=CARTESIAN_POINT('Ctrl Pts',(-55.930488576419,10.9629006319631,-53.0772758084486));
#43232=CARTESIAN_POINT('Ctrl Pts',(-55.9381073316661,10.9395748779739,-53.7653056101449));
#43233=CARTESIAN_POINT('Ctrl Pts',(-55.9416528001124,10.9237215733015,-54.0704359512858));
#43234=CARTESIAN_POINT('Ctrl Pts',(-55.9496601025327,10.8750549527632,-54.6486009070764));
#43235=CARTESIAN_POINT('Ctrl Pts',(-55.9654123447332,10.7549969018306,-55.6302504324446));
#43236=CARTESIAN_POINT('Ctrl Pts',(-55.9994587470345,10.4458388026915,-57.4383823406074));
#43237=CARTESIAN_POINT('Ctrl Pts',(-56.0199533839382,10.2883173198432,-58.7272209294824));
#43238=CARTESIAN_POINT('Ctrl Pts',(-56.0326694572419,10.337296984968,-59.4940973816812));
#43239=CARTESIAN_POINT('Ctrl Pts',(-56.0340287334952,10.345141303396,-59.6076641521854));
#43240=CARTESIAN_POINT('Ctrl Pts',(-56.036730510265,10.3632314626706,-59.8242413083678));
#43241=CARTESIAN_POINT('Ctrl Pts',(-56.0411386361281,10.403075772758,-60.2110159317316));
#43242=CARTESIAN_POINT('Ctrl Pts',(-56.0489389363496,10.5130299230923,-60.9880655794156));
#43243=CARTESIAN_POINT('Ctrl Pts',(-56.0556792290518,10.7040268545881,-61.894066021176));
#43244=CARTESIAN_POINT('Ctrl Pts',(-56.0609547177322,10.9497591159132,-62.808920765965));
#43245=CARTESIAN_POINT('Ctrl Pts',(-56.0635408677761,11.106278666547,-63.326385277232));
#43246=CARTESIAN_POINT('Ctrl Pts',(-56.0651787688794,11.2173018142146,-63.6719298736204));
#43247=CARTESIAN_POINT('Ctrl Pts',(-56.0662527809051,11.2930332503178,-63.9024618429909));
#43248=CARTESIAN_POINT('Ctrl Pts',(-56.0673122919143,11.3712072941945,-64.133059681309));
#43249=CARTESIAN_POINT('Ctrl Pts',(-56.0682356952383,11.4416085466937,-64.3349546075141));
#43250=CARTESIAN_POINT('Ctrl Pts',(-56.0687646661073,11.4823814423657,-64.450336977776));
#43251=CARTESIAN_POINT('Ctrl Pts',(-56.0695619617873,11.544061119532,-64.6233925849231));
#43252=CARTESIAN_POINT('Ctrl Pts',(-56.0702317582838,11.5965520161077,-64.7676389886702));
#43253=CARTESIAN_POINT('Ctrl Pts',(-56.07139569208,11.6845120204599,-65.0057825717699));
#43254=CARTESIAN_POINT('Ctrl Pts',(-56.074264515776,11.767387288938,-65.2187502867463));
#43255=CARTESIAN_POINT('Ctrl Pts',(-56.0786397783873,11.9566422124607,-65.6686664407302));
#43256=CARTESIAN_POINT('Ctrl Pts',(-56.0856374180506,12.3251133559867,-66.4581304223345));
#43257=CARTESIAN_POINT('Ctrl Pts',(-56.09372093771,13.2051032634938,-68.0970024151852));
#43258=CARTESIAN_POINT('Ctrl Pts',(-56.0906321351764,14.1031093673489,-69.5915486423818));
#43259=CARTESIAN_POINT('Ctrl Pts',(-56.0851957454358,14.7345963774996,-70.7930412663358));
#43260=CARTESIAN_POINT('Ctrl Pts',(-56.0856737258281,14.8634736923075,-71.037586644955));
#43261=CARTESIAN_POINT('Ctrl Pts',(-56.0856398440421,15.1288129436771,-71.5400969655525));
#43262=CARTESIAN_POINT('Ctrl Pts',(-56.0859627501435,15.4588011640861,-72.1628188095271));
#43263=CARTESIAN_POINT('Ctrl Pts',(-56.0860780358828,15.8578470167035,-72.9134975508988));
#43264=CARTESIAN_POINT('Ctrl Pts',(-56.0863311102607,16.6573513988515,-74.413976018313));
#43265=CARTESIAN_POINT('Ctrl Pts',(-56.0862924185878,17.3272522841457,-75.6668224616729));
#43266=CARTESIAN_POINT('Ctrl Pts',(-56.0860259166991,18.2989737931892,-77.4942288644924));
#43267=CARTESIAN_POINT('Ctrl Pts',(-56.0861417091234,18.7346714090501,-78.3135205636837));
#43268=CARTESIAN_POINT('Ctrl Pts',(-56.0861417091228,19.1711929964396,-79.1344982657809));
#43269=CARTESIAN_POINT('Ctrl Pts',(-53.2695191090026,5.51412391624868,24.8304298636229));
#43270=CARTESIAN_POINT('Ctrl Pts',(-53.2696729804314,5.51413893918573,24.781544104745));
#43271=CARTESIAN_POINT('Ctrl Pts',(-53.2698343600099,5.51415470785899,24.7326593874112));
#43272=CARTESIAN_POINT('Ctrl Pts',(-53.2717402620553,5.51434076369697,24.1819722349007));
#43273=CARTESIAN_POINT('Ctrl Pts',(-53.2731264290575,5.51435894341818,23.1776970740902));
#43274=CARTESIAN_POINT('Ctrl Pts',(-53.2763014396343,5.51432310337358,21.1689687233707));
#43275=CARTESIAN_POINT('Ctrl Pts',(-53.2889904683357,5.51556557258312,19.6647568302414));
#43276=CARTESIAN_POINT('Ctrl Pts',(-53.3162754315305,5.518818802787,18.4137075492479));
#43277=CARTESIAN_POINT('Ctrl Pts',(-53.3293106107319,5.52034451434612,17.9105627879296));
#43278=CARTESIAN_POINT('Ctrl Pts',(-53.3619539357177,5.52412101015913,16.9063102282351));
#43279=CARTESIAN_POINT('Ctrl Pts',(-53.4319747813724,5.53225803755914,15.152428522052));
#43280=CARTESIAN_POINT('Ctrl Pts',(-53.4991679604305,5.54059971155965,13.6515466504369));
#43281=CARTESIAN_POINT('Ctrl Pts',(-53.5425107860897,5.54690481688883,12.3984165575284));
#43282=CARTESIAN_POINT('Ctrl Pts',(-53.5603706376019,5.54960764105437,11.8980142668053));
#43283=CARTESIAN_POINT('Ctrl Pts',(-53.5972312288389,5.55551650862214,10.8970295658701));
#43284=CARTESIAN_POINT('Ctrl Pts',(-53.6434679491633,5.56341564867434,9.64501806028444));
#43285=CARTESIAN_POINT('Ctrl Pts',(-53.6928486983768,5.57229632593769,8.14044610826101));
#43286=CARTESIAN_POINT('Ctrl Pts',(-53.7174705237535,5.57688272688435,7.13495869916707));
#43287=CARTESIAN_POINT('Ctrl Pts',(-53.7289266788192,5.57903837763239,6.50641411021376));
#43288=CARTESIAN_POINT('Ctrl Pts',(-53.7332088253681,5.57988413685081,6.25651562184119));
#43289=CARTESIAN_POINT('Ctrl Pts',(-53.7407031707429,5.58150267609513,5.75562639093175));
#43290=CARTESIAN_POINT('Ctrl Pts',(-53.7511456644898,5.58410243092635,4.87741752009759));
#43291=CARTESIAN_POINT('Ctrl Pts',(-53.7623560903057,5.58814369853549,3.11632311933031));
#43292=CARTESIAN_POINT('Ctrl Pts',(-53.7590470244509,5.58856175398403,1.6064679537484));
#43293=CARTESIAN_POINT('Ctrl Pts',(-53.7540980002488,5.58677338992612,0.543397417953566));
#43294=CARTESIAN_POINT('Ctrl Pts',(-53.753513348334,5.58635411736398,0.412074377092105));
#43295=CARTESIAN_POINT('Ctrl Pts',(-53.752352226417,5.58478397945459,0.153131956078355));
#43296=CARTESIAN_POINT('Ctrl Pts',(-53.7502960394157,5.58030638502699,-0.298962418503893));
#43297=CARTESIAN_POINT('Ctrl Pts',(-53.747041298155,5.57006430941205,-0.937293506954136));
#43298=CARTESIAN_POINT('Ctrl Pts',(-53.7418125431459,5.5551497800351,-1.69263172943391));
#43299=CARTESIAN_POINT('Ctrl Pts',(-53.7320405695537,5.536106807732,-2.68608904075444));
#43300=CARTESIAN_POINT('Ctrl Pts',(-53.7126486696442,5.52214075949863,-3.90323953145756));
#43301=CARTESIAN_POINT('Ctrl Pts',(-53.6857217408105,5.53762914818405,-4.85284196928096));
#43302=CARTESIAN_POINT('Ctrl Pts',(-53.6642023602138,5.56056015472782,-5.44207547801918));
#43303=CARTESIAN_POINT('Ctrl Pts',(-53.6548329760197,5.56915151054791,-5.72862142582819));
#43304=CARTESIAN_POINT('Ctrl Pts',(-53.6345397295929,5.57623641436791,-6.25851002643969));
#43305=CARTESIAN_POINT('Ctrl Pts',(-53.5946255286048,5.57365819050158,-7.16755236124054));
#43306=CARTESIAN_POINT('Ctrl Pts',(-53.5267824369403,5.56513849529919,-8.35954499643954));
#43307=CARTESIAN_POINT('Ctrl Pts',(-53.4528358806497,5.63531466714391,-9.42459253171312));
#43308=CARTESIAN_POINT('Ctrl Pts',(-53.4063569805158,5.75703994750273,-10.1070730340725));
#43309=CARTESIAN_POINT('Ctrl Pts',(-53.3826169629337,5.8516342288584,-10.4838875321135));
#43310=CARTESIAN_POINT('Ctrl Pts',(-53.3718033621994,5.9082272881835,-10.6687549503979));
#43311=CARTESIAN_POINT('Ctrl Pts',(-53.3641622492917,5.95443181047735,-10.806250048848));
#43312=CARTESIAN_POINT('Ctrl Pts',(-53.3609764178454,5.97942695957719,-10.8749681752605));
#43313=CARTESIAN_POINT('Ctrl Pts',(-53.3526198015811,6.04532819060391,-11.0376782273807));
#43314=CARTESIAN_POINT('Ctrl Pts',(-53.3361006816262,6.18733006109969,-11.3402774953735));
#43315=CARTESIAN_POINT('Ctrl Pts',(-53.2907959702171,6.58731155192089,-12.0388473668935));
#43316=CARTESIAN_POINT('Ctrl Pts',(-53.1924783584682,7.42521315073151,-13.2043467596497));
#43317=CARTESIAN_POINT('Ctrl Pts',(-53.0842900264596,8.29440822558255,-14.3989188175356));
#43318=CARTESIAN_POINT('Ctrl Pts',(-53.015262415626,8.83233778190795,-15.2828268594339));
#43319=CARTESIAN_POINT('Ctrl Pts',(-52.9712767444326,9.1723889427504,-15.9015569257269));
#43320=CARTESIAN_POINT('Ctrl Pts',(-52.941883462723,9.39814693567254,-16.404340394339));
#43321=CARTESIAN_POINT('Ctrl Pts',(-52.9221524344923,9.55495080979618,-16.8496642085187));
#43322=CARTESIAN_POINT('Ctrl Pts',(-52.9171702213878,9.60532703150434,-16.9974857947432));
#43323=CARTESIAN_POINT('Ctrl Pts',(-52.9077925126434,9.70384045488972,-17.3085378437202));
#43324=CARTESIAN_POINT('Ctrl Pts',(-52.9017119486451,9.7888502139978,-17.611479209509));
#43325=CARTESIAN_POINT('Ctrl Pts',(-52.8978643914528,9.86457371739576,-17.9151182244612));
#43326=CARTESIAN_POINT('Ctrl Pts',(-52.8964966777581,9.90752297295601,-18.1030131264597));
#43327=CARTESIAN_POINT('Ctrl Pts',(-52.8959255353737,9.93963575717371,-18.2528564737207));
#43328=CARTESIAN_POINT('Ctrl Pts',(-52.8957656598868,9.96255665128214,-18.3647826827941));
#43329=CARTESIAN_POINT('Ctrl Pts',(-52.8958406345935,9.98074558923007,-18.4577554651167));
#43330=CARTESIAN_POINT('Ctrl Pts',(-52.8960220828767,9.99475780550526,-18.5319159564531));
#43331=CARTESIAN_POINT('Ctrl Pts',(-52.8982398755439,10.1108798618789,-19.161197415467));
#43332=CARTESIAN_POINT('Ctrl Pts',(-52.9230826162276,10.2397643749445,-20.3264110372225));
#43333=CARTESIAN_POINT('Ctrl Pts',(-52.9776760452522,10.3009424686941,-21.9157318243612));
#43334=CARTESIAN_POINT('Ctrl Pts',(-53.0026397326956,10.3306613219927,-22.8884250543864));
#43335=CARTESIAN_POINT('Ctrl Pts',(-53.0078332433723,10.3640352479388,-23.4697077997478));
#43336=CARTESIAN_POINT('Ctrl Pts',(-53.0090207928301,10.3779232234325,-23.7492065296354));
#43337=CARTESIAN_POINT('Ctrl Pts',(-53.0101422632217,10.3965999748253,-24.2767246640981));
#43338=CARTESIAN_POINT('Ctrl Pts',(-53.0084606712719,10.4126262654147,-25.2060431411203));
#43339=CARTESIAN_POINT('Ctrl Pts',(-52.9989783339964,10.398230606303,-26.5002884694706));
#43340=CARTESIAN_POINT('Ctrl Pts',(-52.9857517356138,10.3609028968362,-28.0156324090607));
#43341=CARTESIAN_POINT('Ctrl Pts',(-52.9821696124883,10.3463072684496,-28.9935516511673));
#43342=CARTESIAN_POINT('Ctrl Pts',(-52.9834192251574,10.3472723357311,-29.5347726580737));
#43343=CARTESIAN_POINT('Ctrl Pts',(-52.9837372616693,10.3475112658483,-29.6609741299702));
#43344=CARTESIAN_POINT('Ctrl Pts',(-52.9845353643974,10.3481161356179,-29.9101521285755));
#43345=CARTESIAN_POINT('Ctrl Pts',(-52.986340876066,10.349480494944,-30.3482200575802));
#43346=CARTESIAN_POINT('Ctrl Pts',(-52.9914277859591,10.3532806040434,-31.2241592854396));
#43347=CARTESIAN_POINT('Ctrl Pts',(-53.0020924987196,10.3609199025555,-32.4786454126478));
#43348=CARTESIAN_POINT('Ctrl Pts',(-53.015062011775,10.3692826159378,-33.7336959612824));
#43349=CARTESIAN_POINT('Ctrl Pts',(-53.0254914065946,10.3752013019634,-34.7370311416471));
#43350=CARTESIAN_POINT('Ctrl Pts',(-53.0305261145087,10.3777432817774,-35.2383457278596));
#43351=CARTESIAN_POINT('Ctrl Pts',(-53.0341499042062,10.3794217654475,-35.6150639393877));
#43352=CARTESIAN_POINT('Ctrl Pts',(-53.0366808553066,10.3805297298129,-35.8668994441295));
#43353=CARTESIAN_POINT('Ctrl Pts',(-53.0420881296609,10.3826532259823,-36.3700528992668));
#43354=CARTESIAN_POINT('Ctrl Pts',(-53.0523371587987,10.386195572391,-37.2488687853845));
#43355=CARTESIAN_POINT('Ctrl Pts',(-53.0745845450279,10.3926516914606,-39.0015260691109));
#43356=CARTESIAN_POINT('Ctrl Pts',(-53.0924719215915,10.3979267436415,-40.5024720108467));
#43357=CARTESIAN_POINT('Ctrl Pts',(-53.1018001444244,10.4028349641943,-41.7577669805917));
#43358=CARTESIAN_POINT('Ctrl Pts',(-53.1041676838787,10.4037624619664,-42.136430142011));
#43359=CARTESIAN_POINT('Ctrl Pts',(-53.1066815827788,10.4043145535304,-42.6389847981761));
#43360=CARTESIAN_POINT('Ctrl Pts',(-53.1088301638818,10.4045597059282,-43.1417757799241));
#43361=CARTESIAN_POINT('Ctrl Pts',(-53.110939299965,10.4045416070056,-43.7693696339286));
#43362=CARTESIAN_POINT('Ctrl Pts',(-53.1129027891297,10.4048250580523,-44.5210196499416));
#43363=CARTESIAN_POINT('Ctrl Pts',(-53.1143623411914,10.4059949502891,-45.1455823564742));
#43364=CARTESIAN_POINT('Ctrl Pts',(-53.1155986256389,10.407885674506,-45.6439270779171));
#43365=CARTESIAN_POINT('Ctrl Pts',(-53.1166060629224,10.4098856947673,-46.0169470561475));
#43366=CARTESIAN_POINT('Ctrl Pts',(-53.1177377013386,10.4125673568949,-46.3891933597327));
#43367=CARTESIAN_POINT('Ctrl Pts',(-53.1194730531813,10.4171804267262,-46.8843198176108));
#43368=CARTESIAN_POINT('Ctrl Pts',(-53.1210917554422,10.4219674360715,-47.254411337671));
#43369=CARTESIAN_POINT('Ctrl Pts',(-53.1230216141993,10.4278328510612,-47.6239090432503));
#43370=CARTESIAN_POINT('Ctrl Pts',(-53.1243337754983,10.4328860199948,-47.8585325572095));
#43371=CARTESIAN_POINT('Ctrl Pts',(-53.1269381890424,10.4477144863777,-48.3405539590965));
#43372=CARTESIAN_POINT('Ctrl Pts',(-53.1315208014342,10.4835733437767,-49.1925394235593));
#43373=CARTESIAN_POINT('Ctrl Pts',(-53.1382805406101,10.5511535870157,-50.4477259469352));
#43374=CARTESIAN_POINT('Ctrl Pts',(-53.1478839894708,10.6148347212714,-52.0080606162247));
#43375=CARTESIAN_POINT('Ctrl Pts',(-53.1563545836586,10.6132655386803,-53.0856319446143));
#43376=CARTESIAN_POINT('Ctrl Pts',(-53.1628474808204,10.5871080946179,-53.7730506798432));
#43377=CARTESIAN_POINT('Ctrl Pts',(-53.1658809440165,10.5698873205239,-54.078978194353));
#43378=CARTESIAN_POINT('Ctrl Pts',(-53.172718225336,10.5184020731151,-54.6578777376874));
#43379=CARTESIAN_POINT('Ctrl Pts',(-53.186128484262,10.3931280910598,-55.6405469499418));
#43380=CARTESIAN_POINT('Ctrl Pts',(-53.2152647300223,10.073597963779,-57.4486599529017));
#43381=CARTESIAN_POINT('Ctrl Pts',(-53.2322648244722,9.91038299977115,-58.7349749671413));
#43382=CARTESIAN_POINT('Ctrl Pts',(-53.2438575714141,9.95727375411102,-59.497859872132));
#43383=CARTESIAN_POINT('Ctrl Pts',(-53.2451145053797,9.96484293104403,-59.6110104688653));
#43384=CARTESIAN_POINT('Ctrl Pts',(-53.2476494794711,9.98246534722492,-59.8267651893542));
#43385=CARTESIAN_POINT('Ctrl Pts',(-53.2518916147946,10.0216393104554,-60.2122308274534));
#43386=CARTESIAN_POINT('Ctrl Pts',(-53.2597849475336,10.1308552935276,-60.9871127641917));
#43387=CARTESIAN_POINT('Ctrl Pts',(-53.2673306041421,10.322172678003,-61.891687150218));
#43388=CARTESIAN_POINT('Ctrl Pts',(-53.2735732107563,10.5688715421272,-62.8060550616252));
#43389=CARTESIAN_POINT('Ctrl Pts',(-53.2766749767257,10.7260538805703,-63.3235783249706));
#43390=CARTESIAN_POINT('Ctrl Pts',(-53.2786068180125,10.8375187332017,-63.6692949698584));
#43391=CARTESIAN_POINT('Ctrl Pts',(-53.2798618887772,10.9135406655232,-63.8999771283551));
#43392=CARTESIAN_POINT('Ctrl Pts',(-53.2810746824334,10.9919940234548,-64.1307767366773));
#43393=CARTESIAN_POINT('Ctrl Pts',(-53.2821036920121,11.0626205110791,-64.3328945957961));
#43394=CARTESIAN_POINT('Ctrl Pts',(-53.2826838151074,11.1035153020404,-64.4484175619505));
#43395=CARTESIAN_POINT('Ctrl Pts',(-53.283548221091,11.1653700926799,-64.6216968474611));
#43396=CARTESIAN_POINT('Ctrl Pts',(-53.284252795929,11.2179902945138,-64.7661579752883));
#43397=CARTESIAN_POINT('Ctrl Pts',(-53.2854405442884,11.3061294590031,-65.0046841289595));
#43398=CARTESIAN_POINT('Ctrl Pts',(-53.2882199013159,11.3889600472922,-65.2175420671513));
#43399=CARTESIAN_POINT('Ctrl Pts',(-53.292448406723,11.5782434117156,-65.6675288390924));
#43400=CARTESIAN_POINT('Ctrl Pts',(-53.2991156029898,11.9466785795384,-66.4569755997879));
#43401=CARTESIAN_POINT('Ctrl Pts',(-53.3065839328934,12.8266158262504,-68.0959375031218));
#43402=CARTESIAN_POINT('Ctrl Pts',(-53.3034527100005,13.7246014984242,-69.5904403556736));
#43403=CARTESIAN_POINT('Ctrl Pts',(-53.298461024074,14.3562308772955,-70.7919116954683));
#43404=CARTESIAN_POINT('Ctrl Pts',(-53.2989079885199,14.4851082685386,-71.0364643141845));
#43405=CARTESIAN_POINT('Ctrl Pts',(-53.298884851345,14.7504619528231,-71.538981752293));
#43406=CARTESIAN_POINT('Ctrl Pts',(-53.299187908537,15.0804546178337,-72.1617121321261));
#43407=CARTESIAN_POINT('Ctrl Pts',(-53.2992942658897,15.4795028987994,-72.9123984874085));
#43408=CARTESIAN_POINT('Ctrl Pts',(-53.2995192454489,16.2789992759831,-74.4128876795658));
#43409=CARTESIAN_POINT('Ctrl Pts',(-53.2994656403349,16.9488786459547,-75.6657250237291));
#43410=CARTESIAN_POINT('Ctrl Pts',(-53.2992200346635,17.9205956470159,-77.4931101939678));
#43411=CARTESIAN_POINT('Ctrl Pts',(-53.2993262462524,18.356293084259,-78.3124054144669));
#43412=CARTESIAN_POINT('Ctrl Pts',(-53.2993262462519,18.7928146716484,-79.133383116566));
#43413=CARTESIAN_POINT('Ctrl Pts',(-50.4917882253004,5.17566710371987,24.8304874162273));
#43414=CARTESIAN_POINT('Ctrl Pts',(-50.4919422879461,5.17568106144213,24.7816034400889));
#43415=CARTESIAN_POINT('Ctrl Pts',(-50.4921038555884,5.17569570639061,24.732720517874));
#43416=CARTESIAN_POINT('Ctrl Pts',(-50.4940119203857,5.17586856599346,24.1820548339752));
#43417=CARTESIAN_POINT('Ctrl Pts',(-50.4955724909529,5.17593860157383,23.1778361008006));
#43418=CARTESIAN_POINT('Ctrl Pts',(-50.4992667335108,5.17606267776333,21.1691322613434));
#43419=CARTESIAN_POINT('Ctrl Pts',(-50.5119607466055,5.17721416687989,19.6648867929363));
#43420=CARTESIAN_POINT('Ctrl Pts',(-50.5383956361274,5.17996827678101,18.4137882022575));
#43421=CARTESIAN_POINT('Ctrl Pts',(-50.5511098675465,5.18125500287494,17.9106295924923));
#43422=CARTESIAN_POINT('Ctrl Pts',(-50.5830956060071,5.18442656664954,16.9063864387148));
#43423=CARTESIAN_POINT('Ctrl Pts',(-50.6516776928239,5.19123763326873,15.1526081475984));
#43424=CARTESIAN_POINT('Ctrl Pts',(-50.7162583676642,5.19817828286658,13.6518058482652));
#43425=CARTESIAN_POINT('Ctrl Pts',(-50.7557353079412,5.20339071244593,12.3986742928636));
#43426=CARTESIAN_POINT('Ctrl Pts',(-50.7717676670402,5.20561905708811,11.8982650828353));
#43427=CARTESIAN_POINT('Ctrl Pts',(-50.8041080415491,5.21047533733246,10.8972213333765));
#43428=CARTESIAN_POINT('Ctrl Pts',(-50.8435506882696,5.21694325198105,9.64509183781364));
#43429=CARTESIAN_POINT('Ctrl Pts',(-50.8845928089285,5.22422283738103,8.14041002755545));
#43430=CARTESIAN_POINT('Ctrl Pts',(-50.9045815330377,5.22799726787858,7.13494612707244));
#43431=CARTESIAN_POINT('Ctrl Pts',(-50.9137804798122,5.22978749172542,6.50645248630553));
#43432=CARTESIAN_POINT('Ctrl Pts',(-50.9171207652802,5.23048874545483,6.25663725309473));
#43433=CARTESIAN_POINT('Ctrl Pts',(-50.9226055832772,5.23184374261148,5.75586011385058));
#43434=CARTESIAN_POINT('Ctrl Pts',(-50.9293192198983,5.2340482166052,4.8778075754179));
#43435=CARTESIAN_POINT('Ctrl Pts',(-50.9332230963537,5.23757919640148,3.11687270565004));
#43436=CARTESIAN_POINT('Ctrl Pts',(-50.9271940666093,5.23816338383166,1.6066003813206));
#43437=CARTESIAN_POINT('Ctrl Pts',(-50.924944151531,5.23660003134025,0.543423623103098));
#43438=CARTESIAN_POINT('Ctrl Pts',(-50.9247138303533,5.2363056290163,0.414339096126991));
#43439=CARTESIAN_POINT('Ctrl Pts',(-50.9243864185811,5.23530944223134,0.158224698787665));
#43440=CARTESIAN_POINT('Ctrl Pts',(-50.9241068848092,5.23260255432325,-0.2891299684906));
#43441=CARTESIAN_POINT('Ctrl Pts',(-50.9242445619944,5.22653553940069,-0.923639989145307));
#43442=CARTESIAN_POINT('Ctrl Pts',(-50.9242394642031,5.2175972786583,-1.67831756883862));
#43443=CARTESIAN_POINT('Ctrl Pts',(-50.9227165665054,5.20579796768503,-2.67664338433093));
#43444=CARTESIAN_POINT('Ctrl Pts',(-50.9154444941589,5.19587448445967,-3.91038768968163));
#43445=CARTESIAN_POINT('Ctrl Pts',(-50.8985483027333,5.20214371572755,-4.88421643440741));
#43446=CARTESIAN_POINT('Ctrl Pts',(-50.8828450232104,5.21332010223727,-5.49185544560995));
#43447=CARTESIAN_POINT('Ctrl Pts',(-50.8764257048549,5.2150483326915,-5.78760510738548));
#43448=CARTESIAN_POINT('Ctrl Pts',(-50.8633447034513,5.20613721753072,-6.33252108952286));
#43449=CARTESIAN_POINT('Ctrl Pts',(-50.8389414588566,5.16930113279147,-7.26308501721412));
#43450=CARTESIAN_POINT('Ctrl Pts',(-50.7964756300872,5.10494006098571,-8.4711418915596));
#43451=CARTESIAN_POINT('Ctrl Pts',(-50.737747222281,5.12507030419363,-9.529298817259));
#43452=CARTESIAN_POINT('Ctrl Pts',(-50.6902034234311,5.21378862573971,-10.1917268936));
#43453=CARTESIAN_POINT('Ctrl Pts',(-50.6621507433786,5.28919873023719,-10.5537179772744));
#43454=CARTESIAN_POINT('Ctrl Pts',(-50.6479227661616,5.33605027741116,-10.7302607132582));
#43455=CARTESIAN_POINT('Ctrl Pts',(-50.6372113533515,5.37493309748007,-10.8614628809451));
#43456=CARTESIAN_POINT('Ctrl Pts',(-50.6307408610024,5.39714223544244,-10.9310589148788));
#43457=CARTESIAN_POINT('Ctrl Pts',(-50.615457868595,5.45499085945406,-11.0920476345774));
#43458=CARTESIAN_POINT('Ctrl Pts',(-50.5847067920761,5.5809826822393,-11.3922056187527));
#43459=CARTESIAN_POINT('Ctrl Pts',(-50.5066841896989,5.9405065242805,-12.0837419858941));
#43460=CARTESIAN_POINT('Ctrl Pts',(-50.3581920745141,6.71333282334061,-13.24143272121));
#43461=CARTESIAN_POINT('Ctrl Pts',(-50.2070844063659,7.53254968807352,-14.4264283964002));
#43462=CARTESIAN_POINT('Ctrl Pts',(-50.1143745831895,8.04622175930128,-15.2954922329237));
#43463=CARTESIAN_POINT('Ctrl Pts',(-50.0567907074399,8.37352615381154,-15.9005955895759));
#43464=CARTESIAN_POINT('Ctrl Pts',(-50.0203542727671,8.59476626467718,-16.3877449176251));
#43465=CARTESIAN_POINT('Ctrl Pts',(-49.9979142754099,8.75369398499996,-16.8155401572584));
#43466=CARTESIAN_POINT('Ctrl Pts',(-49.9932937554699,8.80427540492771,-16.9532446535472));
#43467=CARTESIAN_POINT('Ctrl Pts',(-49.9850391776131,8.90725677558605,-17.2463051810055));
#43468=CARTESIAN_POINT('Ctrl Pts',(-49.9818900096223,9.00097130090873,-17.5313844372905));
#43469=CARTESIAN_POINT('Ctrl Pts',(-49.9822865499116,9.08953544821376,-17.8187950252249));
#43470=CARTESIAN_POINT('Ctrl Pts',(-49.9841806466715,9.14198168186362,-17.997075773544));
#43471=CARTESIAN_POINT('Ctrl Pts',(-49.9865389808682,9.18252740910799,-18.1396657873466));
#43472=CARTESIAN_POINT('Ctrl Pts',(-49.9887415658394,9.21215644005256,-18.246358287446));
#43473=CARTESIAN_POINT('Ctrl Pts',(-49.9909150035896,9.23623998981229,-18.3351553365422));
#43474=CARTESIAN_POINT('Ctrl Pts',(-49.9928534025731,9.25513922998495,-18.4060925378598));
#43475=CARTESIAN_POINT('Ctrl Pts',(-50.0104080099896,9.41372406993346,-19.0085655115853));
#43476=CARTESIAN_POINT('Ctrl Pts',(-50.0785835779704,9.65166925678319,-20.1448867246259));
#43477=CARTESIAN_POINT('Ctrl Pts',(-50.2094455136225,9.86360570203751,-21.7593394035839));
#43478=CARTESIAN_POINT('Ctrl Pts',(-50.2695728798328,9.95364845399459,-22.7883530169235));
#43479=CARTESIAN_POINT('Ctrl Pts',(-50.2853974619132,10.0086808237604,-23.4174394581283));
#43480=CARTESIAN_POINT('Ctrl Pts',(-50.2905491917215,10.0307168845544,-23.7072050842054));
#43481=CARTESIAN_POINT('Ctrl Pts',(-50.2982535121411,10.059985098277,-24.2572722652478));
#43482=CARTESIAN_POINT('Ctrl Pts',(-50.3049354504982,10.0831641537804,-25.2170434829339));
#43483=CARTESIAN_POINT('Ctrl Pts',(-50.299090492575,10.0554482373577,-26.5365348741012));
#43484=CARTESIAN_POINT('Ctrl Pts',(-50.2804361269476,9.99211926516758,-28.0501492024477));
#43485=CARTESIAN_POINT('Ctrl Pts',(-50.2699104858743,9.96837189047219,-29.005969213032));
#43486=CARTESIAN_POINT('Ctrl Pts',(-50.2675102217974,9.96983147071442,-29.5291008868419));
#43487=CARTESIAN_POINT('Ctrl Pts',(-50.2669406729928,9.9702759020367,-29.6548785372973));
#43488=CARTESIAN_POINT('Ctrl Pts',(-50.2656765811437,9.97141249672459,-29.9013334019936));
#43489=CARTESIAN_POINT('Ctrl Pts',(-50.2631539222159,9.97412106283928,-30.3359632918983));
#43490=CARTESIAN_POINT('Ctrl Pts',(-50.2570939411495,9.98199525595261,-31.2055924825988));
#43491=CARTESIAN_POINT('Ctrl Pts',(-50.2467310549431,9.99874366664344,-32.4553294381363));
#43492=CARTESIAN_POINT('Ctrl Pts',(-50.2372638556452,10.0180406299146,-33.7105948576416));
#43493=CARTESIAN_POINT('Ctrl Pts',(-50.2321054601144,10.0318670608778,-34.7174137538182));
#43494=CARTESIAN_POINT('Ctrl Pts',(-50.2306260626996,10.037800648482,-35.2215261148078));
#43495=CARTESIAN_POINT('Ctrl Pts',(-50.23005283174,10.0416318474723,-35.6007176993595));
#43496=CARTESIAN_POINT('Ctrl Pts',(-50.2298354684155,10.0441425631425,-35.8523882463753));
#43497=CARTESIAN_POINT('Ctrl Pts',(-50.2299882230626,10.0490093971083,-36.3562680642938));
#43498=CARTESIAN_POINT('Ctrl Pts',(-50.2316173278082,10.0573057462866,-37.2358952215116));
#43499=CARTESIAN_POINT('Ctrl Pts',(-50.2389254191521,10.0723990884057,-38.9907229977759));
#43500=CARTESIAN_POINT('Ctrl Pts',(-50.2473114970814,10.0841162826904,-40.4935920088638));
#43501=CARTESIAN_POINT('Ctrl Pts',(-50.2501140904947,10.0932039565461,-41.7505062234857));
#43502=CARTESIAN_POINT('Ctrl Pts',(-50.2505809071243,10.0953249979928,-42.1293419423953));
#43503=CARTESIAN_POINT('Ctrl Pts',(-50.2507131066099,10.0973339515644,-42.632366127817));
#43504=CARTESIAN_POINT('Ctrl Pts',(-50.2505992437383,10.0989722141392,-43.1356438106316));
#43505=CARTESIAN_POINT('Ctrl Pts',(-50.2501451161471,10.100540748878,-43.7639698516428));
#43506=CARTESIAN_POINT('Ctrl Pts',(-50.2495854290043,10.102441873018,-44.5166707004118));
#43507=CARTESIAN_POINT('Ctrl Pts',(-50.2495106314317,10.1046844156364,-45.1422732594455));
#43508=CARTESIAN_POINT('Ctrl Pts',(-50.2499203773133,10.1072148812516,-45.6415285781111));
#43509=CARTESIAN_POINT('Ctrl Pts',(-50.2505268590744,10.1095939362813,-46.0152816765834));
#43510=CARTESIAN_POINT('Ctrl Pts',(-50.2514927039908,10.1125449059654,-46.3883095356268));
#43511=CARTESIAN_POINT('Ctrl Pts',(-50.2533375408547,10.1173643015842,-46.8845367359995));
#43512=CARTESIAN_POINT('Ctrl Pts',(-50.2554489682574,10.1221245401292,-47.2555408653554));
#43513=CARTESIAN_POINT('Ctrl Pts',(-50.2581634178688,10.1278349914596,-47.6259921783748));
#43514=CARTESIAN_POINT('Ctrl Pts',(-50.2601382453279,10.1327494655044,-47.8614537741923));
#43515=CARTESIAN_POINT('Ctrl Pts',(-50.2645669531397,10.1470848162755,-48.3448779496376));
#43516=CARTESIAN_POINT('Ctrl Pts',(-50.2735228646179,10.181589460592,-49.1990209944655));
#43517=CARTESIAN_POINT('Ctrl Pts',(-50.2892411015512,10.2458256924249,-50.4562472205667));
#43518=CARTESIAN_POINT('Ctrl Pts',(-50.3115704218278,10.3041487355604,-52.0175019206382));
#43519=CARTESIAN_POINT('Ctrl Pts',(-50.3283744489858,10.2985694370559,-53.0946911955599));
#43520=CARTESIAN_POINT('Ctrl Pts',(-50.3394854329771,10.2700744321005,-53.7815927083882));
#43521=CARTESIAN_POINT('Ctrl Pts',(-50.3444777023812,10.2516813158405,-54.0883431032896));
#43522=CARTESIAN_POINT('Ctrl Pts',(-50.3554547454227,10.1977742066435,-54.6680452815916));
#43523=CARTESIAN_POINT('Ctrl Pts',(-50.3766307896317,10.06795271147,-55.6518561088696));
#43524=CARTESIAN_POINT('Ctrl Pts',(-50.4220100454917,9.73932917875835,-57.4602542456734));
#43525=CARTESIAN_POINT('Ctrl Pts',(-50.4517174235069,9.5716293558584,-58.7437695560338));
#43526=CARTESIAN_POINT('Ctrl Pts',(-50.4672683941523,9.616802212515,-59.501807302348));
#43527=CARTESIAN_POINT('Ctrl Pts',(-50.4689891228026,9.62414747583199,-59.6144877527924));
#43528=CARTESIAN_POINT('Ctrl Pts',(-50.472309048858,9.64137944175633,-59.8292913302342));
#43529=CARTESIAN_POINT('Ctrl Pts',(-50.477602282877,9.67996605567735,-60.2132517968072));
#43530=CARTESIAN_POINT('Ctrl Pts',(-50.4864151011654,9.78843142638471,-60.9856425795006));
#43531=CARTESIAN_POINT('Ctrl Pts',(-50.4929757612956,9.97978760295941,-61.888626609612));
#43532=CARTESIAN_POINT('Ctrl Pts',(-50.4974662177313,10.2271615291421,-62.8025169538524));
#43533=CARTESIAN_POINT('Ctrl Pts',(-50.4995193297966,10.3848718063098,-63.3201554766683));
#43534=CARTESIAN_POINT('Ctrl Pts',(-50.5008191348443,10.4967073652988,-63.6660944985812));
#43535=CARTESIAN_POINT('Ctrl Pts',(-50.501676136481,10.5729794099748,-63.8969640514493));
#43536=CARTESIAN_POINT('Ctrl Pts',(-50.5025358148872,10.6516782376813,-64.1280050630122));
#43537=CARTESIAN_POINT('Ctrl Pts',(-50.5033099106476,10.7225113373282,-64.3303833066746));
#43538=CARTESIAN_POINT('Ctrl Pts',(-50.5037621554921,10.7635201092562,-64.4460686102444));
#43539=CARTESIAN_POINT('Ctrl Pts',(-50.5044534077156,10.8255411352936,-64.6196044834109));
#43540=CARTESIAN_POINT('Ctrl Pts',(-50.5050557817371,10.8782882713032,-64.7643078741904));
#43541=CARTESIAN_POINT('Ctrl Pts',(-50.5061377180057,10.9666119413916,-65.003260922051));
#43542=CARTESIAN_POINT('Ctrl Pts',(-50.508638492893,11.0493697468618,-65.2160015584756));
#43543=CARTESIAN_POINT('Ctrl Pts',(-50.5124241402302,11.2386522834735,-65.6660749449834));
#43544=CARTESIAN_POINT('Ctrl Pts',(-50.5183391803283,11.6070025105966,-66.4555156665412));
#43545=CARTESIAN_POINT('Ctrl Pts',(-50.5247662875685,12.4868488647233,-68.0945928971807));
#43546=CARTESIAN_POINT('Ctrl Pts',(-50.5217297342562,13.3848211445789,-69.5890408902695));
#43547=CARTESIAN_POINT('Ctrl Pts',(-50.5172962706906,14.0166187274579,-70.7904911454533));
#43548=CARTESIAN_POINT('Ctrl Pts',(-50.5176848766757,14.1454945205256,-71.0350535179694));
#43549=CARTESIAN_POINT('Ctrl Pts',(-50.517655798034,14.410863768523,-71.5375810908797));
#43550=CARTESIAN_POINT('Ctrl Pts',(-50.517917673406,14.7408594614161,-72.1603229363731));
#43551=CARTESIAN_POINT('Ctrl Pts',(-50.518010611717,15.1399102004369,-72.9110189371167));
#43552=CARTESIAN_POINT('Ctrl Pts',(-50.5182159283882,15.9393977459531,-74.4115205735121));
#43553=CARTESIAN_POINT('Ctrl Pts',(-50.5181862633849,16.6092508749019,-75.6643443595441));
#43554=CARTESIAN_POINT('Ctrl Pts',(-50.5179716192911,17.5809598952617,-77.4917029993533));
#43555=CARTESIAN_POINT('Ctrl Pts',(-50.5180655120236,18.0166559625962,-78.3110026508708));
#43556=CARTESIAN_POINT('Ctrl Pts',(-50.518065512024,18.4531775499857,-79.1319803529701));
#43557=CARTESIAN_POINT('Ctrl Pts',(-47.7140625860263,4.8827673795561,24.83071473666));
#43558=CARTESIAN_POINT('Ctrl Pts',(-47.7142056270501,4.88278315123272,24.7818380104655));
#43559=CARTESIAN_POINT('Ctrl Pts',(-47.7143556438381,4.88279969683197,24.7329624584372));
#43560=CARTESIAN_POINT('Ctrl Pts',(-47.7161271346974,4.88299471720164,24.1823823057849));
#43561=CARTESIAN_POINT('Ctrl Pts',(-47.7175219397781,4.88318692485811,23.1782622657522));
#43562=CARTESIAN_POINT('Ctrl Pts',(-47.7207922725251,4.88366739337577,21.1697171422517));
#43563=CARTESIAN_POINT('Ctrl Pts',(-47.7325810415589,4.8849613002945,19.6655362846526));
#43564=CARTESIAN_POINT('Ctrl Pts',(-47.7573975348289,4.88749005855023,18.4144717200027));
#43565=CARTESIAN_POINT('Ctrl Pts',(-47.769321527011,4.88871561455663,17.9117751017612));
#43566=CARTESIAN_POINT('Ctrl Pts',(-47.7993052830692,4.89181262920139,16.9078592146539));
#43567=CARTESIAN_POINT('Ctrl Pts',(-47.8636134358962,4.89843749421352,15.1540238664033));
#43568=CARTESIAN_POINT('Ctrl Pts',(-47.9244214182784,4.9045205544751,13.6517668992275));
#43569=CARTESIAN_POINT('Ctrl Pts',(-47.9619817440457,4.90795714804035,12.3967188770755));
#43570=CARTESIAN_POINT('Ctrl Pts',(-47.9772718407815,4.90931808413415,11.8955283110643));
#43571=CARTESIAN_POINT('Ctrl Pts',(-48.0082364270896,4.91195046187805,10.8933425971299));
#43572=CARTESIAN_POINT('Ctrl Pts',(-48.0462304403728,4.91499931755227,9.64044727576877));
#43573=CARTESIAN_POINT('Ctrl Pts',(-48.0860237179557,4.91801032724594,8.13590746288963));
#43574=CARTESIAN_POINT('Ctrl Pts',(-48.1056048462851,4.91941894175397,7.13125448252537));
#43575=CARTESIAN_POINT('Ctrl Pts',(-48.114686641634,4.92006091807443,6.50343758513863));
#43576=CARTESIAN_POINT('Ctrl Pts',(-48.1180230915424,4.92028147784815,6.25307816982595));
#43577=CARTESIAN_POINT('Ctrl Pts',(-48.1236516608096,4.92059287275183,5.75186189897002));
#43578=CARTESIAN_POINT('Ctrl Pts',(-48.1309515307269,4.92082784154472,4.87323677530985));
#43579=CARTESIAN_POINT('Ctrl Pts',(-48.1368414760995,4.92039644109217,3.11312011492933));
#43580=CARTESIAN_POINT('Ctrl Pts',(-48.1321571924445,4.91941407371968,1.60646228368251));
#43581=CARTESIAN_POINT('Ctrl Pts',(-48.129156544069,4.91953163485657,0.547584962884119));
#43582=CARTESIAN_POINT('Ctrl Pts',(-48.1287924961985,4.91952801215846,0.420815421233139));
#43583=CARTESIAN_POINT('Ctrl Pts',(-48.1280361619762,4.91943902897318,0.167950253877022));
#43584=CARTESIAN_POINT('Ctrl Pts',(-48.1266207283341,4.91909880758473,-0.274020854476047));
#43585=CARTESIAN_POINT('Ctrl Pts',(-48.1242402329894,4.91818580446943,-0.903549531841198));
#43586=CARTESIAN_POINT('Ctrl Pts',(-48.1205054012334,4.91686798226099,-1.65599660187086));
#43587=CARTESIAN_POINT('Ctrl Pts',(-48.1139402652433,4.91526753761711,-2.65656601275255));
#43588=CARTESIAN_POINT('Ctrl Pts',(-48.1020107258878,4.91468314017721,-3.90276616773367));
#43589=CARTESIAN_POINT('Ctrl Pts',(-48.0869522803996,4.91787671070461,-4.89718018300294));
#43590=CARTESIAN_POINT('Ctrl Pts',(-48.0753265931897,4.92184490707251,-5.52057074281727));
#43591=CARTESIAN_POINT('Ctrl Pts',(-48.071358629886,4.91998443516637,-5.81518912269095));
#43592=CARTESIAN_POINT('Ctrl Pts',(-48.065598030688,4.90444031378955,-6.36312258883095));
#43593=CARTESIAN_POINT('Ctrl Pts',(-48.0593098149811,4.8554734950931,-7.29936993447058));
#43594=CARTESIAN_POINT('Ctrl Pts',(-48.0512760304793,4.76954410211827,-8.52468295486078));
#43595=CARTESIAN_POINT('Ctrl Pts',(-48.0199706320373,4.75930038017222,-9.61057795434388));
#43596=CARTESIAN_POINT('Ctrl Pts',(-47.9753301070093,4.82177048553547,-10.2929213114712));
#43597=CARTESIAN_POINT('Ctrl Pts',(-47.9425518598432,4.87982047166548,-10.6643681872605));
#43598=CARTESIAN_POINT('Ctrl Pts',(-47.9236879911956,4.91686516645017,-10.8446063286549));
#43599=CARTESIAN_POINT('Ctrl Pts',(-47.9085602268087,4.94794884722439,-10.9784757588702));
#43600=CARTESIAN_POINT('Ctrl Pts',(-47.8977045764268,4.96879134742631,-11.0611503257524));
#43601=CARTESIAN_POINT('Ctrl Pts',(-47.8728032300964,5.01813210065941,-11.237347059156));
#43602=CARTESIAN_POINT('Ctrl Pts',(-47.8219732147258,5.12165285259022,-11.5584670494563));
#43603=CARTESIAN_POINT('Ctrl Pts',(-47.696862002376,5.39770009893267,-12.2615093154998));
#43604=CARTESIAN_POINT('Ctrl Pts',(-47.4801637820874,5.97029461539933,-13.409392442977));
#43605=CARTESIAN_POINT('Ctrl Pts',(-47.2858376380383,6.59337864600068,-14.5727985195787));
#43606=CARTESIAN_POINT('Ctrl Pts',(-47.1768883689351,7.00109873332153,-15.4001667508105));
#43607=CARTESIAN_POINT('Ctrl Pts',(-47.1119587725962,7.2675736093193,-15.9664123979976));
#43608=CARTESIAN_POINT('Ctrl Pts',(-47.0739610162134,7.45762098996782,-16.408466282203));
#43609=CARTESIAN_POINT('Ctrl Pts',(-47.0518262734791,7.60559604349496,-16.7855990350013));
#43610=CARTESIAN_POINT('Ctrl Pts',(-47.0491042389521,7.65322588539756,-16.9019857164455));
#43611=CARTESIAN_POINT('Ctrl Pts',(-47.0437189541059,7.75708675336488,-17.1545293646334));
#43612=CARTESIAN_POINT('Ctrl Pts',(-47.0439331697809,7.86091063353106,-17.4007379070685));
#43613=CARTESIAN_POINT('Ctrl Pts',(-47.0476351836161,7.96778846203953,-17.6519066560223));
#43614=CARTESIAN_POINT('Ctrl Pts',(-47.0517168740913,8.0348517437553,-17.8085785791225));
#43615=CARTESIAN_POINT('Ctrl Pts',(-47.0558659103499,8.08885825268645,-17.9346102696999));
#43616=CARTESIAN_POINT('Ctrl Pts',(-47.0594481061716,8.12943201619854,-18.0292450533832));
#43617=CARTESIAN_POINT('Ctrl Pts',(-47.0627989499055,8.16331558501532,-18.1083105118728));
#43618=CARTESIAN_POINT('Ctrl Pts',(-47.065699715029,8.19044455332856,-18.1716594129134));
#43619=CARTESIAN_POINT('Ctrl Pts',(-47.0915481899381,8.42112550168468,-18.7107584271862));
#43620=CARTESIAN_POINT('Ctrl Pts',(-47.1795150098835,8.86475935936997,-19.7614149232649));
#43621=CARTESIAN_POINT('Ctrl Pts',(-47.3620548986719,9.42469340784848,-21.4020513833473));
#43622=CARTESIAN_POINT('Ctrl Pts',(-47.4583992990562,9.68081121232479,-22.554207420914));
#43623=CARTESIAN_POINT('Ctrl Pts',(-47.4898086194942,9.79586248166539,-23.2865755238212));
#43624=CARTESIAN_POINT('Ctrl Pts',(-47.501349742819,9.83847812537408,-23.5883713749792));
#43625=CARTESIAN_POINT('Ctrl Pts',(-47.5222830062559,9.899624865415,-24.1758236534797));
#43626=CARTESIAN_POINT('Ctrl Pts',(-47.5525794688505,9.95672557240012,-25.1849747235455));
#43627=CARTESIAN_POINT('Ctrl Pts',(-47.5791316427958,9.93345826502849,-26.554952963881));
#43628=CARTESIAN_POINT('Ctrl Pts',(-47.5910145312468,9.84915846139396,-28.0887083936959));
#43629=CARTESIAN_POINT('Ctrl Pts',(-47.590154490986,9.81302209147109,-29.0338517263358));
#43630=CARTESIAN_POINT('Ctrl Pts',(-47.5885328811147,9.81147315537453,-29.5440203080735));
#43631=CARTESIAN_POINT('Ctrl Pts',(-47.5879832531315,9.81101342556759,-29.6742051600839));
#43632=CARTESIAN_POINT('Ctrl Pts',(-47.586159408563,9.80992869543475,-29.9250303861287));
#43633=CARTESIAN_POINT('Ctrl Pts',(-47.5811779859765,9.8074963975209,-30.3685920642081));
#43634=CARTESIAN_POINT('Ctrl Pts',(-47.5649066278992,9.80080875659515,-31.2513375375534));
#43635=CARTESIAN_POINT('Ctrl Pts',(-47.5285387694553,9.78697953291634,-32.5117857886755));
#43636=CARTESIAN_POINT('Ctrl Pts',(-47.487944364367,9.77080234221746,-33.7653306238441));
#43637=CARTESIAN_POINT('Ctrl Pts',(-47.4609716571189,9.75914312276783,-34.7638900742689));
#43638=CARTESIAN_POINT('Ctrl Pts',(-47.4506615003537,9.75421317547709,-35.2614394808298));
#43639=CARTESIAN_POINT('Ctrl Pts',(-47.4446011455489,9.75108103893098,-35.6349289491052));
#43640=CARTESIAN_POINT('Ctrl Pts',(-47.4407392943142,9.74903357004824,-35.886860521582));
#43641=CARTESIAN_POINT('Ctrl Pts',(-47.4337743681483,9.74501554106365,-36.3889623730522));
#43642=CARTESIAN_POINT('Ctrl Pts',(-47.4234052858481,9.73817027186817,-37.2665896791131));
#43643=CARTESIAN_POINT('Ctrl Pts',(-47.4086833908215,9.72585364518767,-39.016506618311));
#43644=CARTESIAN_POINT('Ctrl Pts',(-47.4018934869779,9.71812680820316,-40.5149077728951));
#43645=CARTESIAN_POINT('Ctrl Pts',(-47.3945431296122,9.71450015756152,-41.7677065187014));
#43646=CARTESIAN_POINT('Ctrl Pts',(-47.3920533546265,9.71297629043158,-42.1459383835886));
#43647=CARTESIAN_POINT('Ctrl Pts',(-47.3884471775193,9.7105222723979,-42.6476858082887));
#43648=CARTESIAN_POINT('Ctrl Pts',(-47.3847526214039,9.70792387566558,-43.1496599707732));
#43649=CARTESIAN_POINT('Ctrl Pts',(-47.380166200749,9.70470411107148,-43.7761346809352));
#43650=CARTESIAN_POINT('Ctrl Pts',(-47.3753391603478,9.70180347230122,-44.5263353855605));
#43651=CARTESIAN_POINT('Ctrl Pts',(-47.3724027140093,9.70095069186048,-45.1495947593217));
#43652=CARTESIAN_POINT('Ctrl Pts',(-47.3710255206844,9.70166790288393,-45.6468710869082));
#43653=CARTESIAN_POINT('Ctrl Pts',(-47.3705541460537,9.7030148028798,-46.0190618603836));
#43654=CARTESIAN_POINT('Ctrl Pts',(-47.3707232711661,9.70528492627313,-46.3904531500575));
#43655=CARTESIAN_POINT('Ctrl Pts',(-47.3719099595908,9.70968313810096,-46.8844091999811));
#43656=CARTESIAN_POINT('Ctrl Pts',(-47.3739920794671,9.71471544780657,-47.2535610007287));
#43657=CARTESIAN_POINT('Ctrl Pts',(-47.377042747569,9.72110569989881,-47.6220828227915));
#43658=CARTESIAN_POINT('Ctrl Pts',(-47.379394710066,9.72663118277781,-47.8555473010797));
#43659=CARTESIAN_POINT('Ctrl Pts',(-47.3850814028465,9.74293475389079,-48.3357425678953));
#43660=CARTESIAN_POINT('Ctrl Pts',(-47.3974607951798,9.78260342253114,-49.1848346622388));
#43661=CARTESIAN_POINT('Ctrl Pts',(-47.420861741289,9.85863948788479,-50.4372610284887));
#43662=CARTESIAN_POINT('Ctrl Pts',(-47.4551721471118,9.93471239285828,-51.9965477521186));
#43663=CARTESIAN_POINT('Ctrl Pts',(-47.4807755546611,9.94130590937094,-53.0752907530237));
#43664=CARTESIAN_POINT('Ctrl Pts',(-47.4973496509146,9.91947610813647,-53.7640655738369));
#43665=CARTESIAN_POINT('Ctrl Pts',(-47.504696395322,9.90424908173486,-54.0693324798308));
#43666=CARTESIAN_POINT('Ctrl Pts',(-47.5209704879564,9.85681016982776,-54.6478353651674));
#43667=CARTESIAN_POINT('Ctrl Pts',(-47.5527040090638,9.7389428317153,-55.6299312386107));
#43668=CARTESIAN_POINT('Ctrl Pts',(-47.6218994130365,9.43391335290437,-57.4385708087684));
#43669=CARTESIAN_POINT('Ctrl Pts',(-47.6718410018616,9.27979124975618,-58.7266178134533));
#43670=CARTESIAN_POINT('Ctrl Pts',(-47.6932325704654,9.32938585408278,-59.4923571602097));
#43671=CARTESIAN_POINT('Ctrl Pts',(-47.6956163076311,9.33731312674235,-59.6059273236726));
#43672=CARTESIAN_POINT('Ctrl Pts',(-47.7000531835202,9.35552167504649,-59.8224323611747));
#43673=CARTESIAN_POINT('Ctrl Pts',(-47.7067957930165,9.39549614861372,-60.2091251275057));
#43674=CARTESIAN_POINT('Ctrl Pts',(-47.7166992431684,9.50539796378372,-60.9859887116099));
#43675=CARTESIAN_POINT('Ctrl Pts',(-47.7214561246767,9.69581790910098,-61.8918098640388));
#43676=CARTESIAN_POINT('Ctrl Pts',(-47.7231340239658,9.94076524943754,-62.8064520549017));
#43677=CARTESIAN_POINT('Ctrl Pts',(-47.7235728164878,10.0968205414922,-63.3237784091988));
#43678=CARTESIAN_POINT('Ctrl Pts',(-47.7239244868068,10.2075530885451,-63.6692185723788));
#43679=CARTESIAN_POINT('Ctrl Pts',(-47.7241919849669,10.2830958246665,-63.8996767464525));
#43680=CARTESIAN_POINT('Ctrl Pts',(-47.7245395261178,10.3610953015556,-64.1301952062868));
#43681=CARTESIAN_POINT('Ctrl Pts',(-47.7249565011536,10.4313567498936,-64.3320134772627));
#43682=CARTESIAN_POINT('Ctrl Pts',(-47.725233940366,10.4720545332634,-64.4473499295881));
#43683=CARTESIAN_POINT('Ctrl Pts',(-47.7256936092775,10.533626264635,-64.6203343662188));
#43684=CARTESIAN_POINT('Ctrl Pts',(-47.7261710234038,10.5860392702119,-64.764516585462));
#43685=CARTESIAN_POINT('Ctrl Pts',(-47.7271481468912,10.6738842217373,-65.0025456548103));
#43686=CARTESIAN_POINT('Ctrl Pts',(-47.7292868500511,10.7565109011004,-65.2153884779408));
#43687=CARTESIAN_POINT('Ctrl Pts',(-47.7325281998836,10.9453778085396,-65.6651144802906));
#43688=CARTESIAN_POINT('Ctrl Pts',(-47.7375242496738,11.3132330337332,-66.4543442202597));
#43689=CARTESIAN_POINT('Ctrl Pts',(-47.742720043608,12.1924933283291,-68.093045861499));
#43690=CARTESIAN_POINT('Ctrl Pts',(-47.7397424623433,13.0906786878871,-69.5876056501862));
#43691=CARTESIAN_POINT('Ctrl Pts',(-47.7358676365723,13.7226372510541,-70.7892450656705));
#43692=CARTESIAN_POINT('Ctrl Pts',(-47.7361872582796,13.8514717103097,-71.0337783640329));
#43693=CARTESIAN_POINT('Ctrl Pts',(-47.7361421067603,14.1168124493924,-71.5362905071052));
#43694=CARTESIAN_POINT('Ctrl Pts',(-47.7363536649938,14.4467722109897,-72.1590041429464));
#43695=CARTESIAN_POINT('Ctrl Pts',(-47.7364328182178,14.8458083399649,-72.9096798690549));
#43696=CARTESIAN_POINT('Ctrl Pts',(-47.7366285550249,15.6452929518777,-74.4101506961281));
#43697=CARTESIAN_POINT('Ctrl Pts',(-47.7366429623231,16.3152035488193,-75.6629949469208));
#43698=CARTESIAN_POINT('Ctrl Pts',(-47.736456510601,17.286950025154,-77.4904073841466));
#43699=CARTESIAN_POINT('Ctrl Pts',(-47.7365375132694,17.7226385361246,-78.309695710462));
#43700=CARTESIAN_POINT('Ctrl Pts',(-47.7365375132698,18.1591601235141,-79.1306734125598));
#43701=CARTESIAN_POINT('Ctrl Pts',(-45.3967918070423,4.67699963232774,24.8307058930071));
#43702=CARTESIAN_POINT('Ctrl Pts',(-45.3969247453239,4.67701242909821,24.7818288627054));
#43703=CARTESIAN_POINT('Ctrl Pts',(-45.397064167043,4.67702585109274,24.7329529910232));
#43704=CARTESIAN_POINT('Ctrl Pts',(-45.3987107511635,4.67718419498956,24.1823696429735));
#43705=CARTESIAN_POINT('Ctrl Pts',(-45.399943482568,4.67733496035957,23.1782399075204));
#43706=CARTESIAN_POINT('Ctrl Pts',(-45.4027913014562,4.67770710281781,21.169693024752));
#43707=CARTESIAN_POINT('Ctrl Pts',(-45.4137513655735,4.67875883292481,19.6655344501099));
#43708=CARTESIAN_POINT('Ctrl Pts',(-45.4371439178203,4.68084188217039,18.4144909972096));
#43709=CARTESIAN_POINT('Ctrl Pts',(-45.4483529927258,4.68185556026981,17.9118184479246));
#43710=CARTESIAN_POINT('Ctrl Pts',(-45.4764839784317,4.6844273467736,16.9079162604237));
#43711=CARTESIAN_POINT('Ctrl Pts',(-45.5368339980899,4.68993785502906,15.1540506288512));
#43712=CARTESIAN_POINT('Ctrl Pts',(-45.5943262619857,4.69496910524554,13.651732361177));
#43713=CARTESIAN_POINT('Ctrl Pts',(-45.6306532223048,4.69773716630875,12.3966160910634));
#43714=CARTESIAN_POINT('Ctrl Pts',(-45.645533067266,4.69882553265937,11.8954011378803));
#43715=CARTESIAN_POINT('Ctrl Pts',(-45.6759652827717,4.70090494360455,10.8931907311465));
#43716=CARTESIAN_POINT('Ctrl Pts',(-45.7137310016318,4.70327483834507,9.64032794844271));
#43717=CARTESIAN_POINT('Ctrl Pts',(-45.7537367904843,4.70557261803631,8.13584025276354));
#43718=CARTESIAN_POINT('Ctrl Pts',(-45.7736012586385,4.70662765532891,7.13125052478055));
#43719=CARTESIAN_POINT('Ctrl Pts',(-45.7828654989878,4.70710029618373,6.50345235752316));
#43720=CARTESIAN_POINT('Ctrl Pts',(-45.786317932379,4.70725494412154,6.25304043598331));
#43721=CARTESIAN_POINT('Ctrl Pts',(-45.79232155606,4.70744926658238,5.75176951392184));
#43722=CARTESIAN_POINT('Ctrl Pts',(-45.8005821236953,4.70752015725955,4.87308667096534));
#43723=CARTESIAN_POINT('Ctrl Pts',(-45.8090583297727,4.70690178131339,3.11300099992041));
#43724=CARTESIAN_POINT('Ctrl Pts',(-45.8057997026327,4.70604569953201,1.60676663184952));
#43725=CARTESIAN_POINT('Ctrl Pts',(-45.801541792903,4.70626009274662,0.548402311047068));
#43726=CARTESIAN_POINT('Ctrl Pts',(-45.800987058998,4.70628635093447,0.422265412886293));
#43727=CARTESIAN_POINT('Ctrl Pts',(-45.7996982292011,4.70633332612108,0.170242135982571));
#43728=CARTESIAN_POINT('Ctrl Pts',(-45.7969864778771,4.70640749724397,-0.270319621179316));
#43729=CARTESIAN_POINT('Ctrl Pts',(-45.7919117308241,4.70649545803417,-0.898565940448079));
#43730=CARTESIAN_POINT('Ctrl Pts',(-45.7841763362845,4.70665066661472,-1.65059668736111));
#43731=CARTESIAN_POINT('Ctrl Pts',(-45.7720979368721,4.70695598006177,-2.65209326123843));
#43732=CARTESIAN_POINT('Ctrl Pts',(-45.7544067252159,4.70769649167174,-3.90228908918057));
#43733=CARTESIAN_POINT('Ctrl Pts',(-45.7390897014505,4.70882200721035,-4.90310426061235));
#43734=CARTESIAN_POINT('Ctrl Pts',(-45.7296261817282,4.70977477222109,-5.53090732296519));
#43735=CARTESIAN_POINT('Ctrl Pts',(-45.7268366532521,4.70748289314281,-5.8148845586905));
#43736=CARTESIAN_POINT('Ctrl Pts',(-45.7244657734331,4.69424688991172,-6.35268126287957));
#43737=CARTESIAN_POINT('Ctrl Pts',(-45.7265689277227,4.6545344809692,-7.27701819244823));
#43738=CARTESIAN_POINT('Ctrl Pts',(-45.7354526397734,4.58310519728748,-8.51387914878369));
#43739=CARTESIAN_POINT('Ctrl Pts',(-45.7212919559776,4.56554752860145,-9.64670319162602));
#43740=CARTESIAN_POINT('Ctrl Pts',(-45.6837627054695,4.60905344849388,-10.3800545643896));
#43741=CARTESIAN_POINT('Ctrl Pts',(-45.6525098638216,4.65242437433776,-10.7834717441486));
#43742=CARTESIAN_POINT('Ctrl Pts',(-45.6333676049592,4.68066429919607,-10.9800027379942));
#43743=CARTESIAN_POINT('Ctrl Pts',(-45.6175442952074,4.7045672444496,-11.1264413626487));
#43744=CARTESIAN_POINT('Ctrl Pts',(-45.6058880023824,4.72274561546546,-11.2308040278533));
#43745=CARTESIAN_POINT('Ctrl Pts',(-45.5793699186064,4.76188153157013,-11.4380718933958));
#43746=CARTESIAN_POINT('Ctrl Pts',(-45.5250898332709,4.83937214468783,-11.8069446789524));
#43747=CARTESIAN_POINT('Ctrl Pts',(-45.3906594720488,5.0258697792546,-12.5625029020933));
#43748=CARTESIAN_POINT('Ctrl Pts',(-45.158745326719,5.36769124802376,-13.7059503803668));
#43749=CARTESIAN_POINT('Ctrl Pts',(-44.969591291523,5.74461147330062,-14.8067575155667));
#43750=CARTESIAN_POINT('Ctrl Pts',(-44.8704275478205,6.01905615197813,-15.5628579938208));
#43751=CARTESIAN_POINT('Ctrl Pts',(-44.8123138665661,6.20768107447676,-16.0721633411231));
#43752=CARTESIAN_POINT('Ctrl Pts',(-44.7788699687686,6.35515843082492,-16.4599600676233));
#43753=CARTESIAN_POINT('Ctrl Pts',(-44.7583146261796,6.47997019558751,-16.7835552998439));
#43754=CARTESIAN_POINT('Ctrl Pts',(-44.7557554874463,6.52050151786484,-16.8810245148453));
#43755=CARTESIAN_POINT('Ctrl Pts',(-44.7489789344751,6.61425689484792,-17.0979643074361));
#43756=CARTESIAN_POINT('Ctrl Pts',(-44.7451500186526,6.71482824858523,-17.3131211918334));
#43757=CARTESIAN_POINT('Ctrl Pts',(-44.7421629759046,6.82454748409996,-17.536656251571));
#43758=CARTESIAN_POINT('Ctrl Pts',(-44.7409682498287,6.89588792145546,-17.6774709268476));
#43759=CARTESIAN_POINT('Ctrl Pts',(-44.7402504896582,6.95474132705015,-17.7915647827595));
#43760=CARTESIAN_POINT('Ctrl Pts',(-44.7398618658818,6.9996531379746,-17.8776153760358));
#43761=CARTESIAN_POINT('Ctrl Pts',(-44.7396424466105,7.03772449674589,-17.9498189774081));
#43762=CARTESIAN_POINT('Ctrl Pts',(-44.7395285895074,7.06853977631745,-18.0078479715581));
#43763=CARTESIAN_POINT('Ctrl Pts',(-44.738940858362,7.33248078330128,-18.5026887600909));
#43764=CARTESIAN_POINT('Ctrl Pts',(-44.7475478523009,7.89770799509759,-19.4959453393272));
#43765=CARTESIAN_POINT('Ctrl Pts',(-44.77859896707,8.75275826442582,-21.1108797897797));
#43766=CARTESIAN_POINT('Ctrl Pts',(-44.8079240027748,9.21771067855626,-22.3235170660312));
#43767=CARTESIAN_POINT('Ctrl Pts',(-44.822182301373,9.42261513598022,-23.1341165708057));
#43768=CARTESIAN_POINT('Ctrl Pts',(-44.8295413571494,9.49226918962049,-23.4355351762691));
#43769=CARTESIAN_POINT('Ctrl Pts',(-44.8486440692701,9.60622383888513,-24.0416682028876));
#43770=CARTESIAN_POINT('Ctrl Pts',(-44.8919587890394,9.73932723050289,-25.0765185835468));
#43771=CARTESIAN_POINT('Ctrl Pts',(-44.9691138795149,9.78755568820071,-26.4855691463327));
#43772=CARTESIAN_POINT('Ctrl Pts',(-45.0569316107679,9.74764456518795,-28.0488624674195));
#43773=CARTESIAN_POINT('Ctrl Pts',(-45.0988599204631,9.72631169784832,-29.0068894234387));
#43774=CARTESIAN_POINT('Ctrl Pts',(-45.1140632449712,9.73093911688483,-29.5227854550886));
#43775=CARTESIAN_POINT('Ctrl Pts',(-45.117241485544,9.73183657866296,-29.6591174681343));
#43776=CARTESIAN_POINT('Ctrl Pts',(-45.1228617630355,9.7323434200145,-29.9189198025019));
#43777=CARTESIAN_POINT('Ctrl Pts',(-45.1308676185089,9.73035583683325,-30.3782608199284));
#43778=CARTESIAN_POINT('Ctrl Pts',(-45.140335332486,9.71607778341234,-31.2861753032791));
#43779=CARTESIAN_POINT('Ctrl Pts',(-45.1397869098246,9.67435802849875,-32.5682626669705));
#43780=CARTESIAN_POINT('Ctrl Pts',(-45.1324405558967,9.62395212007861,-33.8230375358978));
#43781=CARTESIAN_POINT('Ctrl Pts',(-45.1295733860487,9.58976473289804,-34.8105640708621));
#43782=CARTESIAN_POINT('Ctrl Pts',(-45.130384517476,9.57657466323373,-35.2983868395446));
#43783=CARTESIAN_POINT('Ctrl Pts',(-45.1322694980909,9.56878906202912,-35.6631965396283));
#43784=CARTESIAN_POINT('Ctrl Pts',(-45.1336556288892,9.56343674678396,-35.9164128013516));
#43785=CARTESIAN_POINT('Ctrl Pts',(-45.1367645565076,9.55304305372151,-36.4169831933688));
#43786=CARTESIAN_POINT('Ctrl Pts',(-45.1430480250175,9.53547359998068,-37.2937852133888));
#43787=CARTESIAN_POINT('Ctrl Pts',(-45.1574629516336,9.50320056041596,-39.0397848560149));
#43788=CARTESIAN_POINT('Ctrl Pts',(-45.1692248551232,9.48228635093581,-40.5346106375694));
#43789=CARTESIAN_POINT('Ctrl Pts',(-45.1740013159767,9.47012749911255,-41.7837555766233));
#43790=CARTESIAN_POINT('Ctrl Pts',(-45.1749544288447,9.46608915424261,-42.1616592520973));
#43791=CARTESIAN_POINT('Ctrl Pts',(-45.1755256992377,9.46052268500198,-42.6624065251111));
#43792=CARTESIAN_POINT('Ctrl Pts',(-45.1757255102865,9.454990384937,-43.1633834694535));
#43793=CARTESIAN_POINT('Ctrl Pts',(-45.1754206775425,9.4484490105667,-43.7883710672532));
#43794=CARTESIAN_POINT('Ctrl Pts',(-45.1746548077921,9.44216516589298,-44.5364876519143));
#43795=CARTESIAN_POINT('Ctrl Pts',(-45.1740879321796,9.43903630354368,-45.1577233309101));
#43796=CARTESIAN_POINT('Ctrl Pts',(-45.1739047017952,9.43825076570018,-45.6531846096039));
#43797=CARTESIAN_POINT('Ctrl Pts',(-45.173970432579,9.43864791268071,-46.0239274066856));
#43798=CARTESIAN_POINT('Ctrl Pts',(-45.1742986039458,9.44014687421711,-46.393783701766));
#43799=CARTESIAN_POINT('Ctrl Pts',(-45.1751670329734,9.44376679547408,-46.8855678935479));
#43800=CARTESIAN_POINT('Ctrl Pts',(-45.1763968106901,9.44848910792274,-47.2529795752224));
#43801=CARTESIAN_POINT('Ctrl Pts',(-45.1781381234655,9.4547797656765,-47.6196453890339));
#43802=CARTESIAN_POINT('Ctrl Pts',(-45.1793506736816,9.46029382162677,-47.8514512849776));
#43803=CARTESIAN_POINT('Ctrl Pts',(-45.1818745708335,9.47688635047598,-48.3288845642534));
#43804=CARTESIAN_POINT('Ctrl Pts',(-45.1866624941977,9.51787745918839,-49.1737568330917));
#43805=CARTESIAN_POINT('Ctrl Pts',(-45.1948598210357,9.59793065018163,-50.4223165193547));
#43806=CARTESIAN_POINT('Ctrl Pts',(-45.2085164273352,9.68189629520511,-51.9798747925369));
#43807=CARTESIAN_POINT('Ctrl Pts',(-45.2214687681134,9.69459317093489,-53.0593760433816));
#43808=CARTESIAN_POINT('Ctrl Pts',(-45.231365032527,9.6765817016563,-53.7491408978133));
#43809=CARTESIAN_POINT('Ctrl Pts',(-45.235844382703,9.66329571846373,-54.0529210224869));
#43810=CARTESIAN_POINT('Ctrl Pts',(-45.2461663565889,9.61995793369472,-54.6299665971305));
#43811=CARTESIAN_POINT('Ctrl Pts',(-45.2670530690536,9.50987452788591,-55.6099392070727));
#43812=CARTESIAN_POINT('Ctrl Pts',(-45.3151012174976,9.22120407775639,-57.4179601559676));
#43813=CARTESIAN_POINT('Ctrl Pts',(-45.3510003949752,9.07568722001837,-58.7106356831304));
#43814=CARTESIAN_POINT('Ctrl Pts',(-45.3673316143288,9.12817116247798,-59.484360913267));
#43815=CARTESIAN_POINT('Ctrl Pts',(-45.3691636132104,9.13652638436252,-59.5987350105386));
#43816=CARTESIAN_POINT('Ctrl Pts',(-45.3726709599828,9.15544384876885,-59.8168408868926));
#43817=CARTESIAN_POINT('Ctrl Pts',(-45.3782408371613,9.1964363465885,-60.206054760062));
#43818=CARTESIAN_POINT('Ctrl Pts',(-45.3874159203442,9.30742768779234,-60.9870282365347));
#43819=CARTESIAN_POINT('Ctrl Pts',(-45.3941164500462,9.49720122186125,-61.8953425943457));
#43820=CARTESIAN_POINT('Ctrl Pts',(-45.3986858966782,9.74037100393175,-62.810549390693));
#43821=CARTESIAN_POINT('Ctrl Pts',(-45.4007811970171,9.89520149739856,-63.3275246686143));
#43822=CARTESIAN_POINT('Ctrl Pts',(-45.4021139182939,10.0050961863,-63.672469087878));
#43823=CARTESIAN_POINT('Ctrl Pts',(-45.4029951100338,10.0800837113633,-63.902528470281));
#43824=CARTESIAN_POINT('Ctrl Pts',(-45.4038793121767,10.1575337164629,-64.1325474137763));
#43825=CARTESIAN_POINT('Ctrl Pts',(-45.4046791309213,10.2273415532064,-64.3338420419547));
#43826=CARTESIAN_POINT('Ctrl Pts',(-45.4051469880807,10.2677891911925,-64.4488546655427));
#43827=CARTESIAN_POINT('Ctrl Pts',(-45.4058623292339,10.3289966359398,-64.6213298159851));
#43828=CARTESIAN_POINT('Ctrl Pts',(-45.40648665549,10.3811273464558,-64.7650352495097));
#43829=CARTESIAN_POINT('Ctrl Pts',(-45.4075997403387,10.4685582900223,-65.0022279615426));
#43830=CARTESIAN_POINT('Ctrl Pts',(-45.4096705636337,10.5510978670919,-65.2151667368062));
#43831=CARTESIAN_POINT('Ctrl Pts',(-45.4128271094035,10.7396355313408,-65.6645805689296));
#43832=CARTESIAN_POINT('Ctrl Pts',(-45.4175108483084,11.1070949519467,-66.4536193008161));
#43833=CARTESIAN_POINT('Ctrl Pts',(-45.4219924228712,11.9858538302058,-68.0919758206631));
#43834=CARTESIAN_POINT('Ctrl Pts',(-45.4188767922422,12.8841409741353,-69.5866322626632));
#43835=CARTESIAN_POINT('Ctrl Pts',(-45.415583326104,13.516191818909,-70.7884170998586));
#43836=CARTESIAN_POINT('Ctrl Pts',(-45.4158701096126,13.6449908510542,-71.0329220887169));
#43837=CARTESIAN_POINT('Ctrl Pts',(-45.415847067481,13.910302727703,-71.5354152219409));
#43838=CARTESIAN_POINT('Ctrl Pts',(-45.4160399532874,14.2402265724916,-72.1580992078819));
#43839=CARTESIAN_POINT('Ctrl Pts',(-45.4161097683259,14.6392468323838,-72.9087535210569));
#43840=CARTESIAN_POINT('Ctrl Pts',(-45.416265759434,15.4387251486653,-74.4091941654481));
#43841=CARTESIAN_POINT('Ctrl Pts',(-45.4162454052114,16.1086751496886,-75.6620602523283));
#43842=CARTESIAN_POINT('Ctrl Pts',(-45.4160811373678,17.0804492222374,-77.4895263141691));
#43843=CARTESIAN_POINT('Ctrl Pts',(-45.4161506449042,17.5161264810383,-78.3088023967617));
#43844=CARTESIAN_POINT('Ctrl Pts',(-45.416150644904,17.9526480684277,-79.1297800988595));
#43845=CARTESIAN_POINT('Ctrl Pts',(-43.5414773952673,4.53448753146326,24.8306508196532));
#43846=CARTESIAN_POINT('Ctrl Pts',(-43.5416047669445,4.53449721364328,24.7817720471109));
#43847=CARTESIAN_POINT('Ctrl Pts',(-43.5417383544304,4.53450737193678,24.7328943885228));
#43848=CARTESIAN_POINT('Ctrl Pts',(-43.543315880609,4.53462714710031,24.1822910231318));
#43849=CARTESIAN_POINT('Ctrl Pts',(-43.5444934277257,4.53472020364173,23.1781405139521));
#43850=CARTESIAN_POINT('Ctrl Pts',(-43.547213232334,4.5349402426484,21.1695567924396));
#43851=CARTESIAN_POINT('Ctrl Pts',(-43.5577141297553,4.53573626681342,19.665396739518));
#43852=CARTESIAN_POINT('Ctrl Pts',(-43.580141872167,4.53741690684206,18.4143536264076));
#43853=CARTESIAN_POINT('Ctrl Pts',(-43.5908845213517,4.53822766910346,17.9115809741758));
#43854=CARTESIAN_POINT('Ctrl Pts',(-43.6178388001956,4.54027275181146,16.9076098476224));
#43855=CARTESIAN_POINT('Ctrl Pts',(-43.6756604074524,4.54466059694902,15.1537552531732));
#43856=CARTESIAN_POINT('Ctrl Pts',(-43.7308046180445,4.54878265955304,13.6517813104176));
#43857=CARTESIAN_POINT('Ctrl Pts',(-43.7657324230018,4.55126962212829,12.3970993819365));
#43858=CARTESIAN_POINT('Ctrl Pts',(-43.7800502239518,4.55227609946025,11.8960613948514));
#43859=CARTESIAN_POINT('Ctrl Pts',(-43.8093651510474,4.55429402046486,10.8941089443398));
#43860=CARTESIAN_POINT('Ctrl Pts',(-43.845806874139,4.55674166000825,9.64145045637587));
#43861=CARTESIAN_POINT('Ctrl Pts',(-43.8844367131125,4.55926806744004,8.1369499361624));
#43862=CARTESIAN_POINT('Ctrl Pts',(-43.9036277914651,4.56049111790417,7.13221967877992));
#43863=CARTESIAN_POINT('Ctrl Pts',(-43.9125642966023,4.56105117356098,6.5042781166866));
#43864=CARTESIAN_POINT('Ctrl Pts',(-43.9158997499813,4.56125301868147,6.25398521843682));
#43865=CARTESIAN_POINT('Ctrl Pts',(-43.9217210164265,4.56157889868081,5.75280983079089));
#43866=CARTESIAN_POINT('Ctrl Pts',(-43.9297820679564,4.56195876363265,4.87427062012176));
#43867=CARTESIAN_POINT('Ctrl Pts',(-43.938205566208,4.56211186615648,3.11402949048081));
#43868=CARTESIAN_POINT('Ctrl Pts',(-43.9350456348124,4.56163244268552,1.60721235589409));
#43869=CARTESIAN_POINT('Ctrl Pts',(-43.9305449025619,4.56149728983932,0.548044744225739));
#43870=CARTESIAN_POINT('Ctrl Pts',(-43.92995163912,4.56148146887285,0.421924264229309));
#43871=CARTESIAN_POINT('Ctrl Pts',(-43.9285495522382,4.56144306894868,0.169861106284108));
#43872=CARTESIAN_POINT('Ctrl Pts',(-43.9255547920404,4.56136199309973,-0.270760078205373));
#43873=CARTESIAN_POINT('Ctrl Pts',(-43.9198775066915,4.56119887486765,-0.899129331533509));
#43874=CARTESIAN_POINT('Ctrl Pts',(-43.911291515231,4.56096508359156,-1.65145592914514));
#43875=CARTESIAN_POINT('Ctrl Pts',(-43.8981044383047,4.56057963339869,-2.65340542950447));
#43876=CARTESIAN_POINT('Ctrl Pts',(-43.8795254386815,4.56002921357857,-3.90436111785173));
#43877=CARTESIAN_POINT('Ctrl Pts',(-43.8649534269833,4.55953271096634,-4.90614818740102));
#43878=CARTESIAN_POINT('Ctrl Pts',(-43.8567126149039,4.55926409820865,-5.5342146452382));
#43879=CARTESIAN_POINT('Ctrl Pts',(-43.8543503288117,4.55733097510175,-5.80798547657267));
#43880=CARTESIAN_POINT('Ctrl Pts',(-43.8526460470249,4.5476465780853,-6.33496129077482));
#43881=CARTESIAN_POINT('Ctrl Pts',(-43.8556772819808,4.51933786023616,-7.24583280436193));
#43882=CARTESIAN_POINT('Ctrl Pts',(-43.8664394386739,4.46763897095714,-8.48976964485138));
#43883=CARTESIAN_POINT('Ctrl Pts',(-43.8575645087604,4.45187518229086,-9.66162616485918));
#43884=CARTESIAN_POINT('Ctrl Pts',(-43.8264841504034,4.4812317939519,-10.439780141466));
#43885=CARTESIAN_POINT('Ctrl Pts',(-43.7996564267498,4.51183958327011,-10.8729601445167));
#43886=CARTESIAN_POINT('Ctrl Pts',(-43.7829273783394,4.53207292227548,-11.0855147011133));
#43887=CARTESIAN_POINT('Ctrl Pts',(-43.7689707331577,4.54933119378543,-11.2445899642726));
#43888=CARTESIAN_POINT('Ctrl Pts',(-43.7588133500233,4.56283159515784,-11.3649302891771));
#43889=CARTESIAN_POINT('Ctrl Pts',(-43.7361617811776,4.59013029690435,-11.5975385803844));
#43890=CARTESIAN_POINT('Ctrl Pts',(-43.6905885533692,4.64136130536106,-12.0073322160453));
#43891=CARTESIAN_POINT('Ctrl Pts',(-43.5793977696364,4.75541578831326,-12.8203071653748));
#43892=CARTESIAN_POINT('Ctrl Pts',(-43.3841981059185,4.9490682713273,-13.9775243432551));
#43893=CARTESIAN_POINT('Ctrl Pts',(-43.2172359706947,5.17142115793501,-15.0210579656182));
#43894=CARTESIAN_POINT('Ctrl Pts',(-43.1255566330017,5.35275489925325,-15.7202982956007));
#43895=CARTESIAN_POINT('Ctrl Pts',(-43.0701105163936,5.48340085420829,-16.187028048169));
#43896=CARTESIAN_POINT('Ctrl Pts',(-43.0357728430286,5.59339004773325,-16.5380745918997));
#43897=CARTESIAN_POINT('Ctrl Pts',(-43.0120736898623,5.69205831004088,-16.828969321626));
#43898=CARTESIAN_POINT('Ctrl Pts',(-43.0064495536189,5.72452332379515,-16.9184974593357));
#43899=CARTESIAN_POINT('Ctrl Pts',(-42.9929620042525,5.80202720051158,-17.1189555795941));
#43900=CARTESIAN_POINT('Ctrl Pts',(-42.9800430618435,5.88864111055256,-17.3213604480838));
#43901=CARTESIAN_POINT('Ctrl Pts',(-42.9661972175604,5.98623251149259,-17.5339384305494));
#43902=CARTESIAN_POINT('Ctrl Pts',(-42.9574124453944,6.05092529343878,-17.6688699894998));
#43903=CARTESIAN_POINT('Ctrl Pts',(-42.9501947049534,6.10496966356968,-17.7786718266522));
#43904=CARTESIAN_POINT('Ctrl Pts',(-42.944713353776,6.14654508271073,-17.861727557838));
#43905=CARTESIAN_POINT('Ctrl Pts',(-42.9400770881554,6.18205237853153,-17.9315973336786));
#43906=CARTESIAN_POINT('Ctrl Pts',(-42.9363275774573,6.21094945034024,-17.987854648448));
#43907=CARTESIAN_POINT('Ctrl Pts',(-42.9042578360259,6.45927552362335,-18.4681475521462));
#43908=CARTESIAN_POINT('Ctrl Pts',(-42.8354204510704,7.01884438328396,-19.4483385870696));
#43909=CARTESIAN_POINT('Ctrl Pts',(-42.7235818122568,7.91026567127129,-21.0487658406634));
#43910=CARTESIAN_POINT('Ctrl Pts',(-42.6615545965536,8.4235782780184,-22.2516132514597));
#43911=CARTESIAN_POINT('Ctrl Pts',(-42.6397937596963,8.66346632602533,-23.0651674066825));
#43912=CARTESIAN_POINT('Ctrl Pts',(-42.6373184823834,8.74403332351748,-23.3530168149133));
#43913=CARTESIAN_POINT('Ctrl Pts',(-42.6400465652739,8.88929551511328,-23.9425206307659));
#43914=CARTESIAN_POINT('Ctrl Pts',(-42.6686855051693,9.09087494114976,-24.9504735243279));
#43915=CARTESIAN_POINT('Ctrl Pts',(-42.7586291051712,9.26186522797534,-26.3468890062045));
#43916=CARTESIAN_POINT('Ctrl Pts',(-42.8930054067009,9.35687651394788,-27.9245675859953));
#43917=CARTESIAN_POINT('Ctrl Pts',(-42.9668170921629,9.39917625537599,-28.9088150521134));
#43918=CARTESIAN_POINT('Ctrl Pts',(-42.9956359053881,9.43022741933181,-29.443973003435));
#43919=CARTESIAN_POINT('Ctrl Pts',(-43.0017926813387,9.43761783172049,-29.5826600934523));
#43920=CARTESIAN_POINT('Ctrl Pts',(-43.0138136196532,9.4499284676199,-29.8480333340984));
#43921=CARTESIAN_POINT('Ctrl Pts',(-43.0338459223275,9.46699420480363,-30.3160542990129));
#43922=CARTESIAN_POINT('Ctrl Pts',(-43.0703214349251,9.48410743700334,-31.2394572305364));
#43923=CARTESIAN_POINT('Ctrl Pts',(-43.1136297167087,9.47282905295429,-32.5365077571059));
#43924=CARTESIAN_POINT('Ctrl Pts',(-43.1505483501123,9.4437724363275,-33.7968559783388));
#43925=CARTESIAN_POINT('Ctrl Pts',(-43.179756915703,9.42602709605934,-34.7830704643692));
#43926=CARTESIAN_POINT('Ctrl Pts',(-43.1948523344428,9.42133520497665,-35.268262685831));
#43927=CARTESIAN_POINT('Ctrl Pts',(-43.2066091516522,9.42030918799427,-35.6304498875428));
#43928=CARTESIAN_POINT('Ctrl Pts',(-43.2145227328819,9.41945632756122,-35.8853449854496));
#43929=CARTESIAN_POINT('Ctrl Pts',(-43.2304076818416,9.41760776333118,-36.3872449299346));
#43930=CARTESIAN_POINT('Ctrl Pts',(-43.2581874912136,9.41378261879008,-37.2671370953687));
#43931=CARTESIAN_POINT('Ctrl Pts',(-43.3123675870467,9.40523996947063,-39.0179770168176));
#43932=CARTESIAN_POINT('Ctrl Pts',(-43.3516470087399,9.3984466337369,-40.5163790979968));
#43933=CARTESIAN_POINT('Ctrl Pts',(-43.3751017626546,9.39620560352966,-41.7682292525567));
#43934=CARTESIAN_POINT('Ctrl Pts',(-43.3814199683655,9.39507916206091,-42.1468284953897));
#43935=CARTESIAN_POINT('Ctrl Pts',(-43.3886805914299,9.39311251970767,-42.648723821498));
#43936=CARTESIAN_POINT('Ctrl Pts',(-43.3952225192057,9.39095754326053,-43.1509067571471));
#43937=CARTESIAN_POINT('Ctrl Pts',(-43.4021768476301,9.3881987826084,-43.7775575981803));
#43938=CARTESIAN_POINT('Ctrl Pts',(-43.4089425171841,9.38565114231246,-44.5278758127687));
#43939=CARTESIAN_POINT('Ctrl Pts',(-43.4135801355141,9.38488373368826,-45.1511124442861));
#43940=CARTESIAN_POINT('Ctrl Pts',(-43.4168965709671,9.38552163166002,-45.6482817329203));
#43941=CARTESIAN_POINT('Ctrl Pts',(-43.4192263128526,9.38672700188353,-46.0203539813832));
#43942=CARTESIAN_POINT('Ctrl Pts',(-43.4214469215391,9.38876730446991,-46.3915879436735));
#43943=CARTESIAN_POINT('Ctrl Pts',(-43.4243304847402,9.39273174188816,-46.8852820141213));
#43944=CARTESIAN_POINT('Ctrl Pts',(-43.4264592644717,9.39728689787286,-47.2541897357405));
#43945=CARTESIAN_POINT('Ctrl Pts',(-43.4286836829519,9.40308146710722,-47.6224425609724));
#43946=CARTESIAN_POINT('Ctrl Pts',(-43.429990352853,9.40814613749297,-47.8560422350782));
#43947=CARTESIAN_POINT('Ctrl Pts',(-43.4319672217862,9.42328710943704,-48.3363028422295));
#43948=CARTESIAN_POINT('Ctrl Pts',(-43.4339862099306,9.46037407270681,-49.1855495348585));
#43949=CARTESIAN_POINT('Ctrl Pts',(-43.4341047106985,9.53162435862161,-50.4380086570674));
#43950=CARTESIAN_POINT('Ctrl Pts',(-43.4341668879683,9.60155648143506,-51.9969456558317));
#43951=CARTESIAN_POINT('Ctrl Pts',(-43.4371547465252,9.60478703772803,-53.0749378134565));
#43952=CARTESIAN_POINT('Ctrl Pts',(-43.4410236568199,9.5814192426866,-53.763015054666));
#43953=CARTESIAN_POINT('Ctrl Pts',(-43.4428228358991,9.56558565266787,-54.0680510784552));
#43954=CARTESIAN_POINT('Ctrl Pts',(-43.4470784464119,9.51700097357967,-54.646136857561));
#43955=CARTESIAN_POINT('Ctrl Pts',(-43.4558884498313,9.39728206386044,-55.6276963317156));
#43956=CARTESIAN_POINT('Ctrl Pts',(-43.4773355348517,9.08917547582348,-57.435843844612));
#43957=CARTESIAN_POINT('Ctrl Pts',(-43.4929180935316,8.93280683980113,-58.7247135338309));
#43958=CARTESIAN_POINT('Ctrl Pts',(-43.502951944175,8.98141711200675,-59.4917463672902));
#43959=CARTESIAN_POINT('Ctrl Pts',(-43.5040887115791,8.98923400294946,-59.6053713579836));
#43960=CARTESIAN_POINT('Ctrl Pts',(-43.5064241734618,9.00724889639743,-59.822026795714));
#43961=CARTESIAN_POINT('Ctrl Pts',(-43.5105090660535,9.04695435480541,-60.208917902705));
#43962=CARTESIAN_POINT('Ctrl Pts',(-43.5187094594682,9.15655669920001,-60.9860555524913));
#43963=CARTESIAN_POINT('Ctrl Pts',(-43.5276864039261,9.34700515261771,-61.8918809221699));
#43964=CARTESIAN_POINT('Ctrl Pts',(-43.5356257866396,9.59205287880273,-62.8063113263271));
#43965=CARTESIAN_POINT('Ctrl Pts',(-43.5396263340133,9.74814896875034,-63.3234516794069));
#43966=CARTESIAN_POINT('Ctrl Pts',(-43.5420730449082,9.85888623633741,-63.668749484404));
#43967=CARTESIAN_POINT('Ctrl Pts',(-43.543644714704,9.93442527720585,-63.8991082023449));
#43968=CARTESIAN_POINT('Ctrl Pts',(-43.5451267245491,10.0124096431432,-64.1295221636211));
#43969=CARTESIAN_POINT('Ctrl Pts',(-43.5463409253479,10.0826455753854,-64.3312457131275));
#43970=CARTESIAN_POINT('Ctrl Pts',(-43.5470109321769,10.1233250296039,-64.4465274780185));
#43971=CARTESIAN_POINT('Ctrl Pts',(-43.5479928422882,10.184865352795,-64.6194294836793));
#43972=CARTESIAN_POINT('Ctrl Pts',(-43.5487597636013,10.2372439185951,-64.7635425338402));
#43973=CARTESIAN_POINT('Ctrl Pts',(-43.5499804671287,10.325018907116,-65.001458961203));
#43974=CARTESIAN_POINT('Ctrl Pts',(-43.5520500501327,10.4075489819384,-65.2142421704268));
#43975=CARTESIAN_POINT('Ctrl Pts',(-43.555204266958,10.5962475318124,-65.6638448096376));
#43976=CARTESIAN_POINT('Ctrl Pts',(-43.5597525060502,10.9638366542822,-66.4529293315174));
#43977=CARTESIAN_POINT('Ctrl Pts',(-43.5638198409699,11.8427641573275,-68.0914988092095));
#43978=CARTESIAN_POINT('Ctrl Pts',(-43.5606853444821,12.7410165411229,-69.5860763169363));
#43979=CARTESIAN_POINT('Ctrl Pts',(-43.5579024385739,13.37315894584,-70.7877805666056));
#43980=CARTESIAN_POINT('Ctrl Pts',(-43.5581710713026,13.5019721513977,-71.0323018745553));
#43981=CARTESIAN_POINT('Ctrl Pts',(-43.5581777217519,13.767308255904,-71.5348068904238));
#43982=CARTESIAN_POINT('Ctrl Pts',(-43.558363918352,14.0972510551101,-72.1575083352297));
#43983=CARTESIAN_POINT('Ctrl Pts',(-43.5584264256019,14.4962797472263,-72.908176648061));
#43984=CARTESIAN_POINT('Ctrl Pts',(-43.5585385417129,15.2957534471709,-74.4086378087151));
#43985=CARTESIAN_POINT('Ctrl Pts',(-43.558469611058,15.9656725151421,-75.6614891722437));
#43986=CARTESIAN_POINT('Ctrl Pts',(-43.5583278325102,16.9374352319471,-77.4889175968542));
#43987=CARTESIAN_POINT('Ctrl Pts',(-43.5583885600327,17.3731177442317,-78.3082009283048));
#43988=CARTESIAN_POINT('Ctrl Pts',(-43.5583885600325,17.8096393316212,-79.1291786304031));
#43989=CARTESIAN_POINT('Ctrl Pts',(-41.6855749463137,4.40659539398005,24.8306029215866));
#43990=CARTESIAN_POINT('Ctrl Pts',(-41.685697662467,4.40660227643802,24.7817226223589));
#43991=CARTESIAN_POINT('Ctrl Pts',(-41.6858263644354,4.40660949804129,24.7328433953815));
#43992=CARTESIAN_POINT('Ctrl Pts',(-41.687346263331,4.40669468880106,24.1822225641872));
#43993=CARTESIAN_POINT('Ctrl Pts',(-41.6884979401384,4.40673956543124,23.1780567543321));
#43994=CARTESIAN_POINT('Ctrl Pts',(-41.691168825236,4.40683205281526,21.1694396153191));
#43995=CARTESIAN_POINT('Ctrl Pts',(-41.7012849291027,4.40739933760772,19.6652749989752));
#43996=CARTESIAN_POINT('Ctrl Pts',(-41.7228065880957,4.4087035664667,18.4142278522954));
#43997=CARTESIAN_POINT('Ctrl Pts',(-41.7331204592441,4.40932365972109,17.9113569622441));
#43998=CARTESIAN_POINT('Ctrl Pts',(-41.7590060536787,4.41087272201821,16.907319682426));
#43999=CARTESIAN_POINT('Ctrl Pts',(-41.8145312035812,4.414201634924,15.1534845454099));
#44000=CARTESIAN_POINT('Ctrl Pts',(-41.8673890990281,4.41746314725499,13.651850155213));
#44001=CARTESIAN_POINT('Ctrl Pts',(-41.9007195299706,4.4196756879196,12.3975888332274));
#44002=CARTESIAN_POINT('Ctrl Pts',(-41.9143680521242,4.42060006605874,11.8967219557013));
#44003=CARTESIAN_POINT('Ctrl Pts',(-41.9422657521244,4.4225475988363,10.8950145380524));
#44004=CARTESIAN_POINT('Ctrl Pts',(-41.9768607225259,4.4250514613291,9.6425418442172));
#44005=CARTESIAN_POINT('Ctrl Pts',(-42.0134492212083,4.42777879406171,8.13801797377742));
#44006=CARTESIAN_POINT('Ctrl Pts',(-42.031566864206,4.42915768851939,7.13314986501666));
#44007=CARTESIAN_POINT('Ctrl Pts',(-42.0399866776811,4.4298009317554,6.50507269877867));
#44008=CARTESIAN_POINT('Ctrl Pts',(-42.0431248666837,4.43004717070963,6.25491000507619));
#44009=CARTESIAN_POINT('Ctrl Pts',(-42.0485825634162,4.43050090764894,5.75384465386732));
#44010=CARTESIAN_POINT('Ctrl Pts',(-42.0560865636054,4.43118750202483,4.87546769899893));
#44011=CARTESIAN_POINT('Ctrl Pts',(-42.063708946106,4.43212033692018,3.11507335553097));
#44012=CARTESIAN_POINT('Ctrl Pts',(-42.0603647805318,4.43205410986387,1.60759953127178));
#44013=CARTESIAN_POINT('Ctrl Pts',(-42.0559272801265,4.43154123524431,0.547546226208736));
#44014=CARTESIAN_POINT('Ctrl Pts',(-42.0553411834889,4.43147526155733,0.421316876104222));
#44015=CARTESIAN_POINT('Ctrl Pts',(-42.0539523129837,4.43131874832274,0.169050265537001));
#44016=CARTESIAN_POINT('Ctrl Pts',(-42.0509798249934,4.43098586061686,-0.271900904983259));
#44017=CARTESIAN_POINT('Ctrl Pts',(-42.0453476764959,4.43035149565878,-0.900620055919381));
#44018=CARTESIAN_POINT('Ctrl Pts',(-42.0368686096194,4.42941053987935,-1.65330233669832));
#44019=CARTESIAN_POINT('Ctrl Pts',(-42.0239588406089,4.42796549860846,-2.65549737470179));
#44020=CARTESIAN_POINT('Ctrl Pts',(-42.0060682271433,4.42597160743345,-3.90642587730085));
#44021=CARTESIAN_POINT('Ctrl Pts',(-41.9926014280487,4.4244184970362,-4.90790089596296));
#44022=CARTESIAN_POINT('Ctrl Pts',(-41.9852842444455,4.42356328852968,-5.53526790519391));
#44023=CARTESIAN_POINT('Ctrl Pts',(-41.9830897219956,4.42221824706501,-5.79917433259166));
#44024=CARTESIAN_POINT('Ctrl Pts',(-41.9810825063314,4.41633986280381,-6.315422455717));
#44025=CARTESIAN_POINT('Ctrl Pts',(-41.9823681306211,4.39969099804006,-7.21277145484061));
#44026=CARTESIAN_POINT('Ctrl Pts',(-41.9896449906298,4.36892455429229,-8.46250372528066));
#44027=CARTESIAN_POINT('Ctrl Pts',(-41.9821520153673,4.35789994862493,-9.67049901943245));
#44028=CARTESIAN_POINT('Ctrl Pts',(-41.9576210819876,4.3745848449589,-10.4909114220271));
#44029=CARTESIAN_POINT('Ctrl Pts',(-41.9364549378075,4.39279740316707,-10.9526158538038));
#44030=CARTESIAN_POINT('Ctrl Pts',(-41.9232258854634,4.40503170868416,-11.1807898585064));
#44031=CARTESIAN_POINT('Ctrl Pts',(-41.9121637037425,4.41554754816524,-11.3522122103185));
#44032=CARTESIAN_POINT('Ctrl Pts',(-41.9043363905,4.42361119608237,-11.4848721190377));
#44033=CARTESIAN_POINT('Ctrl Pts',(-41.8875072833387,4.4384065006293,-11.7382331079967));
#44034=CARTESIAN_POINT('Ctrl Pts',(-41.8549592713017,4.46324441376506,-12.1817395961442));
#44035=CARTESIAN_POINT('Ctrl Pts',(-41.7787962092932,4.50967578248564,-13.0456684600629));
#44036=CARTESIAN_POINT('Ctrl Pts',(-41.644491098764,4.58263430774086,-14.2285222813806));
#44037=CARTESIAN_POINT('Ctrl Pts',(-41.5123917809733,4.68998798291981,-15.2366382479619));
#44038=CARTESIAN_POINT('Ctrl Pts',(-41.4287824925274,4.79553689828114,-15.8936194208614));
#44039=CARTESIAN_POINT('Ctrl Pts',(-41.3747256809767,4.87640790074795,-16.3280864374078));
#44040=CARTESIAN_POINT('Ctrl Pts',(-41.3366524575088,4.95035921181498,-16.6510048310789));
#44041=CARTESIAN_POINT('Ctrl Pts',(-41.306835620299,5.02081124413835,-16.9176146481003));
#44042=CARTESIAN_POINT('Ctrl Pts',(-41.29636387782,5.04509520112619,-17.0047436605908));
#44043=CARTESIAN_POINT('Ctrl Pts',(-41.2730346722212,5.10353261298984,-17.196868830241));
#44044=CARTESIAN_POINT('Ctrl Pts',(-41.2480790791988,5.17084493684142,-17.3934626491004));
#44045=CARTESIAN_POINT('Ctrl Pts',(-41.221105495172,5.24831389192612,-17.6003988774604));
#44046=CARTESIAN_POINT('Ctrl Pts',(-41.2035751962912,5.30040427107532,-17.7323825235609));
#44047=CARTESIAN_POINT('Ctrl Pts',(-41.1891277198281,5.34431580294902,-17.8399805850786));
#44048=CARTESIAN_POINT('Ctrl Pts',(-41.1781000088454,5.37829931059263,-17.9215089454721));
#44049=CARTESIAN_POINT('Ctrl Pts',(-41.1687506376316,5.40748252995808,-17.9901864120133));
#44050=CARTESIAN_POINT('Ctrl Pts',(-41.1611793212934,5.43133205518555,-18.0455404137636));
#44051=CARTESIAN_POINT('Ctrl Pts',(-41.0963218209191,5.63677452637474,-18.5184584440352));
#44052=CARTESIAN_POINT('Ctrl Pts',(-40.9564136843565,6.11712912367197,-19.4926969375005));
#44053=CARTESIAN_POINT('Ctrl Pts',(-40.7364366289171,6.9157475288387,-21.0886818032411));
#44054=CARTESIAN_POINT('Ctrl Pts',(-40.6149000229783,7.38772813226633,-22.2673531899013));
#44055=CARTESIAN_POINT('Ctrl Pts',(-40.5669825701007,7.62255736913357,-23.0490607398952));
#44056=CARTESIAN_POINT('Ctrl Pts',(-40.556831256611,7.70335393494949,-23.3180003280109));
#44057=CARTESIAN_POINT('Ctrl Pts',(-40.5433299693075,7.86078183394624,-23.8747078218839));
#44058=CARTESIAN_POINT('Ctrl Pts',(-40.5459948282985,8.11005511183186,-24.8289667580384));
#44059=CARTESIAN_POINT('Ctrl Pts',(-40.6076287795505,8.40807181386579,-26.1759437191406));
#44060=CARTESIAN_POINT('Ctrl Pts',(-40.7347495145975,8.68290591483088,-27.7493495807299));
#44061=CARTESIAN_POINT('Ctrl Pts',(-40.8164187078509,8.82327999821301,-28.7669616509389));
#44062=CARTESIAN_POINT('Ctrl Pts',(-40.8492236913612,8.89606935974853,-29.3296269754071));
#44063=CARTESIAN_POINT('Ctrl Pts',(-40.8559901601149,8.91325409450142,-29.4678481197618));
#44064=CARTESIAN_POINT('Ctrl Pts',(-40.8700356227369,8.94447667853886,-29.73607891955));
#44065=CARTESIAN_POINT('Ctrl Pts',(-40.8949093233339,8.99390826626215,-30.2073921688695));
#44066=CARTESIAN_POINT('Ctrl Pts',(-40.9461990154241,9.0718486267278,-31.1392426571425));
#44067=CARTESIAN_POINT('Ctrl Pts',(-41.0213279503794,9.13631858149522,-32.4475458748229));
#44068=CARTESIAN_POINT('Ctrl Pts',(-41.0947609597759,9.16910478169614,-33.7171654407122));
#44069=CARTESIAN_POINT('Ctrl Pts',(-41.1509081769705,9.19432417390162,-34.7085603115485));
#44070=CARTESIAN_POINT('Ctrl Pts',(-41.1779978329913,9.20935303612885,-35.1956042420512));
#44071=CARTESIAN_POINT('Ctrl Pts',(-41.1979259101171,9.22261206042192,-35.5589384775174));
#44072=CARTESIAN_POINT('Ctrl Pts',(-41.211274985297,9.23163148260346,-35.815843256208));
#44073=CARTESIAN_POINT('Ctrl Pts',(-41.2379556572264,9.24831886907607,-36.3209572959123));
#44074=CARTESIAN_POINT('Ctrl Pts',(-41.2843674816221,9.2749306091751,-37.206592034575));
#44075=CARTESIAN_POINT('Ctrl Pts',(-41.374064639626,9.31856056441366,-38.9678356583997));
#44076=CARTESIAN_POINT('Ctrl Pts',(-41.4394366532432,9.34455345009808,-40.4743298755513));
#44077=CARTESIAN_POINT('Ctrl Pts',(-41.4804556071417,9.36439928361108,-41.7326381762914));
#44078=CARTESIAN_POINT('Ctrl Pts',(-41.4917681728629,9.36962188655343,-42.1126309299343));
#44079=CARTESIAN_POINT('Ctrl Pts',(-41.5052363141583,9.37537120989589,-42.6169053118342));
#44080=CARTESIAN_POINT('Ctrl Pts',(-41.5177026046486,9.38048383318957,-43.1215402313297));
#44081=CARTESIAN_POINT('Ctrl Pts',(-41.5315381423871,9.385893671131,-43.7515528341479));
#44082=CARTESIAN_POINT('Ctrl Pts',(-41.5457753993936,9.39159865784897,-44.5062999306404));
#44083=CARTESIAN_POINT('Ctrl Pts',(-41.5560294813494,9.39633244195201,-45.1335791991821));
#44084=CARTESIAN_POINT('Ctrl Pts',(-41.5634795732993,9.40047075649581,-45.6341556731554));
#44085=CARTESIAN_POINT('Ctrl Pts',(-41.5687465317506,9.40384986790816,-46.0088895953954));
#44086=CARTESIAN_POINT('Ctrl Pts',(-41.5737465074904,9.40759620424152,-46.3828880382925));
#44087=CARTESIAN_POINT('Ctrl Pts',(-41.5801306758304,9.41319667576749,-46.88040080413));
#44088=CARTESIAN_POINT('Ctrl Pts',(-41.5846779335584,9.41823077142094,-47.2523538003496));
#44089=CARTESIAN_POINT('Ctrl Pts',(-41.5891880026032,9.42398765962361,-47.6237819174283));
#44090=CARTESIAN_POINT('Ctrl Pts',(-41.5919840811149,9.42881699202896,-47.8606476760656));
#44091=CARTESIAN_POINT('Ctrl Pts',(-41.5967687945331,9.4425848061764,-48.3462104845544));
#44092=CARTESIAN_POINT('Ctrl Pts',(-41.6032500935833,9.47507599431753,-49.2037625717664));
#44093=CARTESIAN_POINT('Ctrl Pts',(-41.6083296045376,9.53401971082211,-50.4641957400867));
#44094=CARTESIAN_POINT('Ctrl Pts',(-41.6115416025726,9.58327908023829,-52.0270286219866));
#44095=CARTESIAN_POINT('Ctrl Pts',(-41.6142570143924,9.57141240308287,-53.1035174134462));
#44096=CARTESIAN_POINT('Ctrl Pts',(-41.6170842694937,9.53940035558117,-53.7894131631721));
#44097=CARTESIAN_POINT('Ctrl Pts',(-41.6181932184546,9.51929615382017,-54.097309136534));
#44098=CARTESIAN_POINT('Ctrl Pts',(-41.6204158196274,9.46175833377061,-54.6781916945254));
#44099=CARTESIAN_POINT('Ctrl Pts',(-41.6241355094009,9.32499922588705,-55.6639665235512));
#44100=CARTESIAN_POINT('Ctrl Pts',(-41.6321391320519,8.98141565581387,-57.4737578573867));
#44101=CARTESIAN_POINT('Ctrl Pts',(-41.6352564780507,8.80416763399032,-58.7542741719814));
#44102=CARTESIAN_POINT('Ctrl Pts',(-41.6419319708265,8.84554828365744,-59.5066281603445));
#44103=CARTESIAN_POINT('Ctrl Pts',(-41.6427197098762,8.85240436315506,-59.6187556373831));
#44104=CARTESIAN_POINT('Ctrl Pts',(-41.6444588222317,8.86878566359322,-59.8324321931772));
#44105=CARTESIAN_POINT('Ctrl Pts',(-41.6477959507849,8.906130579617,-60.2145958717469));
#44106=CARTESIAN_POINT('Ctrl Pts',(-41.6555290946326,9.01309581026938,-60.9839390616392));
#44107=CARTESIAN_POINT('Ctrl Pts',(-41.6656789092045,9.2046257784976,-61.884804523698));
#44108=CARTESIAN_POINT('Ctrl Pts',(-41.6752684815886,9.45314319759352,-62.7978123507762));
#44109=CARTESIAN_POINT('Ctrl Pts',(-41.6801807428335,9.61165849753839,-63.3153935693162));
#44110=CARTESIAN_POINT('Ctrl Pts',(-41.6831468915368,9.72402519255565,-63.661473322807));
#44111=CARTESIAN_POINT('Ctrl Pts',(-41.6850374865527,9.80064280446529,-63.8924835916954));
#44112=CARTESIAN_POINT('Ctrl Pts',(-41.6867870113969,9.87966992968769,-64.1237362136409));
#44113=CARTESIAN_POINT('Ctrl Pts',(-41.6881799527362,9.95075883245909,-64.3263615763983));
#44114=CARTESIAN_POINT('Ctrl Pts',(-41.688934145285,9.9919032359808,-64.4422061061361));
#44115=CARTESIAN_POINT('Ctrl Pts',(-41.6900235328282,10.054115637533,-64.6159981699555));
#44116=CARTESIAN_POINT('Ctrl Pts',(-41.6908383052638,10.1069972284883,-64.7609540810492));
#44117=CARTESIAN_POINT('Ctrl Pts',(-41.6920728116426,10.195489344907,-65.0003621966698));
#44118=CARTESIAN_POINT('Ctrl Pts',(-41.6940697097662,10.2780415895599,-65.2128739119397));
#44119=CARTESIAN_POINT('Ctrl Pts',(-41.6971009990176,10.467137609276,-65.6629225402255));
#44120=CARTESIAN_POINT('Ctrl Pts',(-41.7013784550244,10.835093913543,-66.4521842042188));
#44121=CARTESIAN_POINT('Ctrl Pts',(-41.7049787078459,11.7144976447062,-68.0912567734202));
#44122=CARTESIAN_POINT('Ctrl Pts',(-41.7019352411704,12.6125834775925,-69.585655539249));
#44123=CARTESIAN_POINT('Ctrl Pts',(-41.6996350389558,13.2448030238341,-70.7871589920456));
#44124=CARTESIAN_POINT('Ctrl Pts',(-41.6998795464537,13.3736551022578,-71.0317206123756));
#44125=CARTESIAN_POINT('Ctrl Pts',(-41.6999072801692,13.6390412747428,-71.5342543097902));
#44126=CARTESIAN_POINT('Ctrl Pts',(-41.7000799865726,13.9690255241614,-72.1569980731772));
#44127=CARTESIAN_POINT('Ctrl Pts',(-41.7001336613318,14.36807282733,-72.9076991264268));
#44128=CARTESIAN_POINT('Ctrl Pts',(-41.7002071861,15.1675386808873,-74.4082071762659));
#44129=CARTESIAN_POINT('Ctrl Pts',(-41.7001019708216,15.837371218953,-75.6610214368742));
#44130=CARTESIAN_POINT('Ctrl Pts',(-41.6999820122622,16.809089882623,-77.4883620781338));
#44131=CARTESIAN_POINT('Ctrl Pts',(-41.7000326001874,17.2447800067055,-78.3076624344991));
#44132=CARTESIAN_POINT('Ctrl Pts',(-41.7000326001874,17.681301594095,-79.1286401365976));
#44133=CARTESIAN_POINT('Ctrl Pts',(-39.8297931480168,4.30089380366595,24.830602047834));
#44134=CARTESIAN_POINT('Ctrl Pts',(-39.8299114630833,4.3008990929334,24.78172171557));
#44135=CARTESIAN_POINT('Ctrl Pts',(-39.8300355500048,4.30090464320175,24.7328424414219));
#44136=CARTESIAN_POINT('Ctrl Pts',(-39.8315008348087,4.30097010912121,24.1822216618942));
#44137=CARTESIAN_POINT('Ctrl Pts',(-39.8326341752565,4.30100217254688,23.1780621652815));
#44138=CARTESIAN_POINT('Ctrl Pts',(-39.8352790867674,4.30106615227246,21.1694431088377));
#44139=CARTESIAN_POINT('Ctrl Pts',(-39.8450305426849,4.30150215534326,19.6652809261295));
#44140=CARTESIAN_POINT('Ctrl Pts',(-39.8656602898903,4.30251651664904,18.4142310178032));
#44141=CARTESIAN_POINT('Ctrl Pts',(-39.8755574820151,4.30299596277146,17.9113461412146));
#44142=CARTESIAN_POINT('Ctrl Pts',(-39.9004164841773,4.30418812240353,16.9073028735776));
#44143=CARTESIAN_POINT('Ctrl Pts',(-39.9537335816,4.30674885227799,15.1534825452192));
#44144=CARTESIAN_POINT('Ctrl Pts',(-40.0043389427622,4.3092914420343,13.6519164127763));
#44145=CARTESIAN_POINT('Ctrl Pts',(-40.0359637219453,4.31108023983322,12.3977176469952));
#44146=CARTESIAN_POINT('Ctrl Pts',(-40.0488823383933,4.31183394637067,11.8968749770987));
#44147=CARTESIAN_POINT('Ctrl Pts',(-40.0751861247578,4.31344186128328,10.8951953012143));
#44148=CARTESIAN_POINT('Ctrl Pts',(-40.1076610674584,4.31553762482537,9.64275117357418));
#44149=CARTESIAN_POINT('Ctrl Pts',(-40.1418550022536,4.31784800138233,8.13821998910642));
#44150=CARTESIAN_POINT('Ctrl Pts',(-40.1587271976532,4.31902826059171,7.13335908880077));
#44151=CARTESIAN_POINT('Ctrl Pts',(-40.1665508599929,4.31958193706928,6.50527516075616));
#44152=CARTESIAN_POINT('Ctrl Pts',(-40.1694560805316,4.31979833457379,6.25515470745086));
#44153=CARTESIAN_POINT('Ctrl Pts',(-40.1744696474126,4.32021173111455,5.7541330082611));
#44154=CARTESIAN_POINT('Ctrl Pts',(-40.1812597490853,4.32087297286246,4.87583060632696));
#44155=CARTESIAN_POINT('Ctrl Pts',(-40.1877615170938,4.32187781283288,3.11542901410488));
#44156=CARTESIAN_POINT('Ctrl Pts',(-40.1841517730371,4.3219093923555,1.60788699549147));
#44157=CARTESIAN_POINT('Ctrl Pts',(-40.1800414129611,4.32131088132128,0.547597544998743));
#44158=CARTESIAN_POINT('Ctrl Pts',(-40.1795013359313,4.32123244923683,0.421302512279844));
#44159=CARTESIAN_POINT('Ctrl Pts',(-40.1782294712075,4.32104491163839,0.168935192359385));
#44160=CARTESIAN_POINT('Ctrl Pts',(-40.175524627641,4.32064205722609,-0.27218276183076));
#44161=CARTESIAN_POINT('Ctrl Pts',(-40.1704276659856,4.31987394138445,-0.901034338282424));
#44162=CARTESIAN_POINT('Ctrl Pts',(-40.1627832733404,4.31873536139517,-1.65383635728535));
#44163=CARTESIAN_POINT('Ctrl Pts',(-40.1511337820403,4.31702074322043,-2.65598405249863));
#44164=CARTESIAN_POINT('Ctrl Pts',(-40.1349501757378,4.31472508907572,-3.90657868690618));
#44165=CARTESIAN_POINT('Ctrl Pts',(-40.1226251363579,4.3131393526332,-4.90749312754089));
#44166=CARTESIAN_POINT('Ctrl Pts',(-40.1158543990754,4.31237494775209,-5.53413996057266));
#44167=CARTESIAN_POINT('Ctrl Pts',(-40.1135869601886,4.31165753439819,-5.79060421533873));
#44168=CARTESIAN_POINT('Ctrl Pts',(-40.1104842025132,4.30889665464121,-6.29867272758451));
#44169=CARTESIAN_POINT('Ctrl Pts',(-40.1079320500244,4.30140928720403,-7.18557117664585));
#44170=CARTESIAN_POINT('Ctrl Pts',(-40.1075002949748,4.28773211170499,-8.43919536745521));
#44171=CARTESIAN_POINT('Ctrl Pts',(-40.0979431800538,4.28250603011998,-9.6737737294806));
#44172=CARTESIAN_POINT('Ctrl Pts',(-40.0794180589679,4.2896159913547,-10.5256234324252));
#44173=CARTESIAN_POINT('Ctrl Pts',(-40.0644505017986,4.29757952688169,-11.0088597276714));
#44174=CARTESIAN_POINT('Ctrl Pts',(-40.0553407674673,4.30298489891383,-11.2490523951628));
#44175=CARTESIAN_POINT('Ctrl Pts',(-40.0478046614143,4.30765034982014,-11.4299264392524));
#44176=CARTESIAN_POINT('Ctrl Pts',(-40.0427004166551,4.31074429421119,-11.5669600302684));
#44177=CARTESIAN_POINT('Ctrl Pts',(-40.0323767708002,4.31529495958614,-11.8298741459896));
#44178=CARTESIAN_POINT('Ctrl Pts',(-40.0138927680509,4.32018324612044,-12.288832822566));
#44179=CARTESIAN_POINT('Ctrl Pts',(-39.9745792624865,4.3211634986152,-13.1809544205443));
#44180=CARTESIAN_POINT('Ctrl Pts',(-39.9075100857676,4.32116438958334,-14.3942739237789));
#44181=CARTESIAN_POINT('Ctrl Pts',(-39.8243636709521,4.36339195578311,-15.4141826122897));
#44182=CARTESIAN_POINT('Ctrl Pts',(-39.7568993275666,4.42274128845835,-16.0696027064544));
#44183=CARTESIAN_POINT('Ctrl Pts',(-39.7088063807627,4.47133204515602,-16.5006483077442));
#44184=CARTESIAN_POINT('Ctrl Pts',(-39.6692619585097,4.51884981766233,-16.8181705647147));
#44185=CARTESIAN_POINT('Ctrl Pts',(-39.6346316045092,4.5655688528116,-17.0796880689598));
#44186=CARTESIAN_POINT('Ctrl Pts',(-39.6204120795866,4.58382912268261,-17.175690740393));
#44187=CARTESIAN_POINT('Ctrl Pts',(-39.5894669012688,4.62516231987957,-17.3766146318054));
#44188=CARTESIAN_POINT('Ctrl Pts',(-39.5553158916272,4.67215116259866,-17.5815260242127));
#44189=CARTESIAN_POINT('Ctrl Pts',(-39.5185800153218,4.72485428291418,-17.7931822188726));
#44190=CARTESIAN_POINT('Ctrl Pts',(-39.4946952607774,4.75998745770387,-17.9275952541007));
#44191=CARTESIAN_POINT('Ctrl Pts',(-39.4751042176496,4.78938719031116,-18.0366034819522));
#44192=CARTESIAN_POINT('Ctrl Pts',(-39.4601907595611,4.81205896222492,-18.1190253381994));
#44193=CARTESIAN_POINT('Ctrl Pts',(-39.4475935447712,4.83146010520306,-18.1882840561084));
#44194=CARTESIAN_POINT('Ctrl Pts',(-39.4374244274026,4.8472792986152,-18.244027993542));
#44195=CARTESIAN_POINT('Ctrl Pts',(-39.3504688559995,4.98336628900204,-18.719720209416));
#44196=CARTESIAN_POINT('Ctrl Pts',(-39.1701471321289,5.29569390328575,-19.6878533559967));
#44197=CARTESIAN_POINT('Ctrl Pts',(-38.9242229480404,5.82689686466538,-21.2532366026309));
#44198=CARTESIAN_POINT('Ctrl Pts',(-38.8059077773893,6.16859330004726,-22.3670328740001));
#44199=CARTESIAN_POINT('Ctrl Pts',(-38.7570216643074,6.36015803481956,-23.0814111966791));
#44200=CARTESIAN_POINT('Ctrl Pts',(-38.7447800238885,6.42923735981035,-23.328423449339));
#44201=CARTESIAN_POINT('Ctrl Pts',(-38.723820624919,6.57429412002019,-23.8426500143035));
#44202=CARTESIAN_POINT('Ctrl Pts',(-38.7039991705238,6.83111560382248,-24.7331385960951));
#44203=CARTESIAN_POINT('Ctrl Pts',(-38.7099306974958,7.20325016995822,-26.0161853728573));
#44204=CARTESIAN_POINT('Ctrl Pts',(-38.7505792606654,7.62202264051377,-27.5675741391084));
#44205=CARTESIAN_POINT('Ctrl Pts',(-38.7797668023837,7.86054302302213,-28.6152446982086));
#44206=CARTESIAN_POINT('Ctrl Pts',(-38.7892658775211,7.97746624359547,-29.2076491505204));
#44207=CARTESIAN_POINT('Ctrl Pts',(-38.7911525363579,8.00347609994022,-29.3415640528822));
#44208=CARTESIAN_POINT('Ctrl Pts',(-38.795568900938,8.05340115514498,-29.6075879530807));
#44209=CARTESIAN_POINT('Ctrl Pts',(-38.8043527904606,8.13629703152824,-30.0725680034506));
#44210=CARTESIAN_POINT('Ctrl Pts',(-38.8263682508179,8.28492022380721,-30.9967695748171));
#44211=CARTESIAN_POINT('Ctrl Pts',(-38.8686709923634,8.45617305599503,-32.3008431646847));
#44212=CARTESIAN_POINT('Ctrl Pts',(-38.9203939555227,8.59310886872018,-33.5776947955661));
#44213=CARTESIAN_POINT('Ctrl Pts',(-38.9637989885803,8.69480564673521,-34.5803683821298));
#44214=CARTESIAN_POINT('Ctrl Pts',(-38.9855148236409,8.74510155541343,-35.0749037451322));
#44215=CARTESIAN_POINT('Ctrl Pts',(-39.0016350899177,8.78356692726934,-35.4444375768675));
#44216=CARTESIAN_POINT('Ctrl Pts',(-39.0123957027471,8.80985696054819,-35.7026593968134));
#44217=CARTESIAN_POINT('Ctrl Pts',(-39.0349110126382,8.85998494195932,-36.2120466346827));
#44218=CARTESIAN_POINT('Ctrl Pts',(-39.0759897514108,8.94313733967483,-37.104355852086));
#44219=CARTESIAN_POINT('Ctrl Pts',(-39.1626367000569,9.09070470507714,-38.8797197070461));
#44220=CARTESIAN_POINT('Ctrl Pts',(-39.2343498384004,9.1889654345898,-40.3979241974921));
#44221=CARTESIAN_POINT('Ctrl Pts',(-39.2818954499488,9.25877965806356,-41.6660339213601));
#44222=CARTESIAN_POINT('Ctrl Pts',(-39.2950638878413,9.27834154057425,-42.0486116434629));
#44223=CARTESIAN_POINT('Ctrl Pts',(-39.3110379056122,9.3017834411066,-42.5567161560632));
#44224=CARTESIAN_POINT('Ctrl Pts',(-39.326088661976,9.32368226929647,-43.0652356268463));
#44225=CARTESIAN_POINT('Ctrl Pts',(-39.3434458658797,9.34832447909361,-43.7003231605712));
#44226=CARTESIAN_POINT('Ctrl Pts',(-39.362809408335,9.37425457532264,-44.4614473516942));
#44227=CARTESIAN_POINT('Ctrl Pts',(-39.3784480905642,9.39339504305688,-45.0942864763365));
#44228=CARTESIAN_POINT('Ctrl Pts',(-39.3910942576435,9.4075375084826,-45.5994493536755));
#44229=CARTESIAN_POINT('Ctrl Pts',(-39.4007552007379,9.41765522041657,-45.9776910996982));
#44230=CARTESIAN_POINT('Ctrl Pts',(-39.4107012674894,9.42736606118332,-46.3552617040635));
#44231=CARTESIAN_POINT('Ctrl Pts',(-39.4244828041639,9.43987014279348,-46.8576199079467));
#44232=CARTESIAN_POINT('Ctrl Pts',(-39.4355796726667,9.44891064666244,-47.2332959012991));
#44233=CARTESIAN_POINT('Ctrl Pts',(-39.4474131679077,9.45786884799196,-47.608522670452));
#44234=CARTESIAN_POINT('Ctrl Pts',(-39.4555075039778,9.46441277966897,-47.8486933692234));
#44235=CARTESIAN_POINT('Ctrl Pts',(-39.4722691301041,9.48038854409172,-48.3400075043167));
#44236=CARTESIAN_POINT('Ctrl Pts',(-39.5028365388771,9.51357355094779,-49.2068771604531));
#44237=CARTESIAN_POINT('Ctrl Pts',(-39.5486702333604,9.56588051029713,-50.4776982592062));
#44238=CARTESIAN_POINT('Ctrl Pts',(-39.6027707836672,9.59908376373866,-52.0484437744134));
#44239=CARTESIAN_POINT('Ctrl Pts',(-39.6355429012624,9.57401187231233,-53.1270087990632));
#44240=CARTESIAN_POINT('Ctrl Pts',(-39.6540971477978,9.53365496047467,-53.8133957215356));
#44241=CARTESIAN_POINT('Ctrl Pts',(-39.6616800978402,9.50902042983665,-54.1258915107586));
#44242=CARTESIAN_POINT('Ctrl Pts',(-39.6767805853012,9.44146978560207,-54.7119512819459));
#44243=CARTESIAN_POINT('Ctrl Pts',(-39.7028304779311,9.28487457519746,-55.7048841033207));
#44244=CARTESIAN_POINT('Ctrl Pts',(-39.7523611380775,8.89899646706934,-57.5182886098759));
#44245=CARTESIAN_POINT('Ctrl Pts',(-39.7831463768863,8.70030675270623,-58.7896356166503));
#44246=CARTESIAN_POINT('Ctrl Pts',(-39.7997801411076,8.73508473009655,-59.5229656801026));
#44247=CARTESIAN_POINT('Ctrl Pts',(-39.8016896555854,8.741017361795,-59.6336104409786));
#44248=CARTESIAN_POINT('Ctrl Pts',(-39.8052901413032,8.75581682568381,-59.8440440927058));
#44249=CARTESIAN_POINT('Ctrl Pts',(-39.8109597621908,8.79080107943052,-60.2212073384165));
#44250=CARTESIAN_POINT('Ctrl Pts',(-39.8200282135911,8.89479056849624,-60.9822394237097));
#44251=CARTESIAN_POINT('Ctrl Pts',(-39.8260360532955,9.0865192287289,-61.8779760087666));
#44252=CARTESIAN_POINT('Ctrl Pts',(-39.8295731896413,9.33765559955061,-62.7895320369173));
#44253=CARTESIAN_POINT('Ctrl Pts',(-39.8310212942597,9.49817191638174,-63.3075735756629));
#44254=CARTESIAN_POINT('Ctrl Pts',(-39.8319255508167,9.61193685091784,-63.6544547583156));
#44255=CARTESIAN_POINT('Ctrl Pts',(-39.8325232750647,9.68948855333687,-63.8861306959977));
#44256=CARTESIAN_POINT('Ctrl Pts',(-39.8331318185583,9.76943793851357,-64.1182399850882));
#44257=CARTESIAN_POINT('Ctrl Pts',(-39.8337018758477,9.84128825163668,-64.3217838167787));
#44258=CARTESIAN_POINT('Ctrl Pts',(-39.8340427347527,9.88285030071759,-64.4382012244413));
#44259=CARTESIAN_POINT('Ctrl Pts',(-39.8345719320016,9.9456683768302,-64.6128988734076));
#44260=CARTESIAN_POINT('Ctrl Pts',(-39.8350523314316,9.99900995718296,-64.7587123480466));
#44261=CARTESIAN_POINT('Ctrl Pts',(-39.8359396646288,10.0881584837466,-64.9996352209183));
#44262=CARTESIAN_POINT('Ctrl Pts',(-39.8374902700331,10.1706399387457,-65.2117876939817));
#44263=CARTESIAN_POINT('Ctrl Pts',(-39.8398170196311,10.3600045172887,-65.6621891819383));
#44264=CARTESIAN_POINT('Ctrl Pts',(-39.843131858082,10.7281843839988,-66.4514728099116));
#44265=CARTESIAN_POINT('Ctrl Pts',(-39.845876871811,11.6080767952086,-68.0909065229435));
#44266=CARTESIAN_POINT('Ctrl Pts',(-39.843327687577,12.5062924443932,-69.5851576688017));
#44267=CARTESIAN_POINT('Ctrl Pts',(-39.8413504014661,13.1386697797965,-70.7866057521726));
#44268=CARTESIAN_POINT('Ctrl Pts',(-39.8415361597441,13.2675599635809,-71.0312033519439));
#44269=CARTESIAN_POINT('Ctrl Pts',(-39.8415353492584,13.5330038135489,-71.5337768994219));
#44270=CARTESIAN_POINT('Ctrl Pts',(-39.8416622329038,13.8630346117925,-72.1565663160765));
#44271=CARTESIAN_POINT('Ctrl Pts',(-39.8417041928247,14.2621049670467,-72.907306052374));
#44272=CARTESIAN_POINT('Ctrl Pts',(-39.8417838427976,15.0615664520001,-74.4078651633378));
#44273=CARTESIAN_POINT('Ctrl Pts',(-39.8417435694573,15.7313146331549,-75.6606366493089));
#44274=CARTESIAN_POINT('Ctrl Pts',(-39.841647950285,16.7029874268988,-77.4878785996119));
#44275=CARTESIAN_POINT('Ctrl Pts',(-39.8416897698438,17.1386891158188,-78.307198653046));
#44276=CARTESIAN_POINT('Ctrl Pts',(-39.8416897698439,17.5752107032083,-79.1281763551445));
#44277=CARTESIAN_POINT('Ctrl Pts',(-37.9743804869919,4.21861863427918,24.8306265576595));
#44278=CARTESIAN_POINT('Ctrl Pts',(-37.9744933412749,4.21862296368332,24.781747004875));
#44279=CARTESIAN_POINT('Ctrl Pts',(-37.9746116996787,4.21862750610694,24.7328685159225));
#44280=CARTESIAN_POINT('Ctrl Pts',(-37.9760093878018,4.21868107839185,24.1822571666999));
#44281=CARTESIAN_POINT('Ctrl Pts',(-37.9770928025108,4.21871687976674,23.1781116141306));
#44282=CARTESIAN_POINT('Ctrl Pts',(-37.9796222523406,4.21879772051816,21.1695091063699));
#44283=CARTESIAN_POINT('Ctrl Pts',(-37.988923418268,4.21915417447705,19.6653556871867));
#44284=CARTESIAN_POINT('Ctrl Pts',(-38.0085896781781,4.21993578500939,18.4143085580057));
#44285=CARTESIAN_POINT('Ctrl Pts',(-38.0180265439753,4.2203080448418,17.9114693439527));
#44286=CARTESIAN_POINT('Ctrl Pts',(-38.0417320316029,4.22123855332113,16.9074600931303));
#44287=CARTESIAN_POINT('Ctrl Pts',(-38.092576449602,4.22323443097777,15.1536393156253));
#44288=CARTESIAN_POINT('Ctrl Pts',(-38.1408051880377,4.22516989518677,13.6519419426153));
#44289=CARTESIAN_POINT('Ctrl Pts',(-38.170903396427,4.22644947705509,12.3975570868814));
#44290=CARTESIAN_POINT('Ctrl Pts',(-38.1831929699881,4.22698018707274,11.8966377111797));
#44291=CARTESIAN_POINT('Ctrl Pts',(-38.2081999459129,4.22808605464995,10.8948432547909));
#44292=CARTESIAN_POINT('Ctrl Pts',(-38.2390434108757,4.2294918983112,9.64232897953741));
#44293=CARTESIAN_POINT('Ctrl Pts',(-38.2715056140244,4.23100759531148,8.13781350830912));
#44294=CARTESIAN_POINT('Ctrl Pts',(-38.2875179676639,4.2317702569467,7.13304930191504));
#44295=CARTESIAN_POINT('Ctrl Pts',(-38.2949489018608,4.23212573179239,6.50503800955867));
#44296=CARTESIAN_POINT('Ctrl Pts',(-38.2977099300648,4.23226189994421,6.25485919894676));
#44297=CARTESIAN_POINT('Ctrl Pts',(-38.3024790164624,4.23251304482732,5.75379011111632));
#44298=CARTESIAN_POINT('Ctrl Pts',(-38.3089479453886,4.23289290544923,4.8754362249382));
#44299=CARTESIAN_POINT('Ctrl Pts',(-38.3151739057549,4.23340331481503,3.11513220656035));
#44300=CARTESIAN_POINT('Ctrl Pts',(-38.3117375096816,4.23332952842037,1.60807604480747));
#44301=CARTESIAN_POINT('Ctrl Pts',(-38.3077338232431,4.23299020488926,0.548264881323011));
#44302=CARTESIAN_POINT('Ctrl Pts',(-38.3072081561105,4.23294628726474,0.422037778870473));
#44303=CARTESIAN_POINT('Ctrl Pts',(-38.3059713749947,4.23284144102519,0.169792824938136));
#44304=CARTESIAN_POINT('Ctrl Pts',(-38.3033435895393,4.23261728659212,-0.271125465382427));
#44305=CARTESIAN_POINT('Ctrl Pts',(-38.2983999561383,4.23218967685735,-0.899719883146217));
#44306=CARTESIAN_POINT('Ctrl Pts',(-38.2909903793428,4.23156156894473,-1.6523352386966));
#44307=CARTESIAN_POINT('Ctrl Pts',(-38.2797133192693,4.23061375891271,-2.65430127585317));
#44308=CARTESIAN_POINT('Ctrl Pts',(-38.2640680641888,4.22935135029831,-3.90488850894447));
#44309=CARTESIAN_POINT('Ctrl Pts',(-38.2521812332404,4.22846831850042,-4.90598421604601));
#44310=CARTESIAN_POINT('Ctrl Pts',(-38.245662932773,4.22803832190949,-5.53266413366317));
#44311=CARTESIAN_POINT('Ctrl Pts',(-38.2432660770742,4.22776094337687,-5.7850702330293));
#44312=CARTESIAN_POINT('Ctrl Pts',(-38.239157279881,4.22686154318823,-6.28877538383063));
#44313=CARTESIAN_POINT('Ctrl Pts',(-38.2333400682135,4.22459584850577,-7.1701007369905));
#44314=CARTESIAN_POINT('Ctrl Pts',(-38.2265369799843,4.22056807197913,-8.42604530220827));
#44315=CARTESIAN_POINT('Ctrl Pts',(-38.2152635068069,4.21879488566088,-9.67537062573929));
#44316=CARTESIAN_POINT('Ctrl Pts',(-38.2016123736228,4.22048906463511,-10.5446281636035));
#44317=CARTESIAN_POINT('Ctrl Pts',(-38.1916770114935,4.22252872692914,-11.0397205111789));
#44318=CARTESIAN_POINT('Ctrl Pts',(-38.1859173687779,4.22393808368096,-11.2865534428756));
#44319=CARTESIAN_POINT('Ctrl Pts',(-38.1812503236375,4.22516215592496,-11.4725327889825));
#44320=CARTESIAN_POINT('Ctrl Pts',(-38.1782132664989,4.22569598471026,-11.6083006574023));
#44321=CARTESIAN_POINT('Ctrl Pts',(-38.1724963236154,4.22539253894241,-11.8717389184555));
#44322=CARTESIAN_POINT('Ctrl Pts',(-38.1632652605988,4.22184588540865,-12.3312268093402));
#44323=CARTESIAN_POINT('Ctrl Pts',(-38.146644928951,4.2057839670911,-13.2294108148301));
#44324=CARTESIAN_POINT('Ctrl Pts',(-38.1209532574981,4.17591208670593,-14.462707710516));
#44325=CARTESIAN_POINT('Ctrl Pts',(-38.078515050113,4.17918427375947,-15.5158363917128));
#44326=CARTESIAN_POINT('Ctrl Pts',(-38.0352829832334,4.20693258492168,-16.1977362964252));
#44327=CARTESIAN_POINT('Ctrl Pts',(-38.0020608049623,4.23285504278592,-16.6472440721846));
#44328=CARTESIAN_POINT('Ctrl Pts',(-37.9717172227133,4.2613947474326,-16.9790036420799));
#44329=CARTESIAN_POINT('Ctrl Pts',(-37.9430624290585,4.29089588194445,-17.2524972836078));
#44330=CARTESIAN_POINT('Ctrl Pts',(-37.9310944384756,4.30340318167128,-17.3624838714222));
#44331=CARTESIAN_POINT('Ctrl Pts',(-37.9049516670918,4.33043376104169,-17.5832900565561));
#44332=CARTESIAN_POINT('Ctrl Pts',(-37.8757206533561,4.36056488940581,-17.8067425951866));
#44333=CARTESIAN_POINT('Ctrl Pts',(-37.8439229501231,4.39335377727898,-18.0324728092801));
#44334=CARTESIAN_POINT('Ctrl Pts',(-37.8230876353914,4.41489277682979,-18.1745891414915));
#44335=CARTESIAN_POINT('Ctrl Pts',(-37.8059091120036,4.43270415477703,-18.288878512028));
#44336=CARTESIAN_POINT('Ctrl Pts',(-37.7927864478151,4.4463428369108,-18.3749011727451));
#44337=CARTESIAN_POINT('Ctrl Pts',(-37.7816662610051,4.4579337525335,-18.4468361470788));
#44338=CARTESIAN_POINT('Ctrl Pts',(-37.7726670462702,4.46733538452826,-18.5045381817367));
#44339=CARTESIAN_POINT('Ctrl Pts',(-37.6956240797217,4.5479987181198,-18.9958335683562));
#44340=CARTESIAN_POINT('Ctrl Pts',(-37.531578810134,4.72380138407194,-19.9617965245065));
#44341=CARTESIAN_POINT('Ctrl Pts',(-37.3071222493637,5.01839492298006,-21.4593889396249));
#44342=CARTESIAN_POINT('Ctrl Pts',(-37.1979292243293,5.23114314143361,-22.492559477754));
#44343=CARTESIAN_POINT('Ctrl Pts',(-37.1477785057481,5.3663840162175,-23.143767430772));
#44344=CARTESIAN_POINT('Ctrl Pts',(-37.1317756722386,5.41682183827126,-23.374560641058));
#44345=CARTESIAN_POINT('Ctrl Pts',(-37.1010420548658,5.52904087143839,-23.8568415378094));
#44346=CARTESIAN_POINT('Ctrl Pts',(-37.0546893039173,5.74296592891402,-24.7049493973709));
#44347=CARTESIAN_POINT('Ctrl Pts',(-37.0012049893423,6.08801716179193,-25.9535934320049));
#44348=CARTESIAN_POINT('Ctrl Pts',(-36.9470279644122,6.51018306820065,-27.4977922697091));
#44349=CARTESIAN_POINT('Ctrl Pts',(-36.9130693803763,6.76162478093457,-28.5617199323548));
#44350=CARTESIAN_POINT('Ctrl Pts',(-36.8938132746591,6.8835366097984,-29.1698009783583));
#44351=CARTESIAN_POINT('Ctrl Pts',(-36.8900864116145,6.90952801988863,-29.3003038722774));
#44352=CARTESIAN_POINT('Ctrl Pts',(-36.8827560528828,6.96066199356787,-29.5634991228843));
#44353=CARTESIAN_POINT('Ctrl Pts',(-36.8710543183909,7.0467001782728,-30.0218644761164));
#44354=CARTESIAN_POINT('Ctrl Pts',(-36.851341532771,7.20700354283504,-30.9356587905047));
#44355=CARTESIAN_POINT('Ctrl Pts',(-36.8333810382757,7.40736751552731,-32.2288073399679));
#44356=CARTESIAN_POINT('Ctrl Pts',(-36.826924086164,7.58396623130391,-33.5044465690719));
#44357=CARTESIAN_POINT('Ctrl Pts',(-36.8272877347697,7.71909430657529,-34.5127169328848));
#44358=CARTESIAN_POINT('Ctrl Pts',(-36.8291349703753,7.78592356887283,-35.0124871732846));
#44359=CARTESIAN_POINT('Ctrl Pts',(-36.8309931623893,7.83642439587603,-35.3867717541854));
#44360=CARTESIAN_POINT('Ctrl Pts',(-36.832274469254,7.87064395520631,-35.6443002734807));
#44361=CARTESIAN_POINT('Ctrl Pts',(-36.8366281141019,7.93732800623012,-36.1545335368831));
#44362=CARTESIAN_POINT('Ctrl Pts',(-36.8480097321712,8.05060401090947,-37.0473268414636));
#44363=CARTESIAN_POINT('Ctrl Pts',(-36.8830256946237,8.26262751388984,-38.8247059011497));
#44364=CARTESIAN_POINT('Ctrl Pts',(-36.9240274059898,8.4190591370404,-40.3445738849485));
#44365=CARTESIAN_POINT('Ctrl Pts',(-36.9521838192205,8.53490390652826,-41.6142113403113));
#44366=CARTESIAN_POINT('Ctrl Pts',(-36.9595866936516,8.56769269468203,-41.9993803748625));
#44367=CARTESIAN_POINT('Ctrl Pts',(-36.9686014748246,8.60762379522345,-42.5092105260691));
#44368=CARTESIAN_POINT('Ctrl Pts',(-36.9772121426193,8.64550080422054,-43.0193369830249));
#44369=CARTESIAN_POINT('Ctrl Pts',(-36.987702670631,8.68941259692222,-43.6555519495176));
#44370=CARTESIAN_POINT('Ctrl Pts',(-37.0012727711582,8.73833577638218,-44.4168683480898));
#44371=CARTESIAN_POINT('Ctrl Pts',(-37.0146294238036,8.77731233846491,-45.048789040518));
#44372=CARTESIAN_POINT('Ctrl Pts',(-37.0272992448317,8.80823108976467,-45.5525785506231));
#44373=CARTESIAN_POINT('Ctrl Pts',(-37.0379798249283,8.83147635912366,-45.9294512079208));
#44374=CARTESIAN_POINT('Ctrl Pts',(-37.0500287686793,8.85497269830543,-46.3053079102783));
#44375=CARTESIAN_POINT('Ctrl Pts',(-37.0681863270722,8.88687733082516,-46.8049009793023));
#44376=CARTESIAN_POINT('Ctrl Pts',(-37.0844161301337,8.91174571627579,-47.1779366605091));
#44377=CARTESIAN_POINT('Ctrl Pts',(-37.102864789622,8.93761822369083,-47.5500895309825));
#44378=CARTESIAN_POINT('Ctrl Pts',(-37.1161923388764,8.95566301568517,-47.787728821962));
#44379=CARTESIAN_POINT('Ctrl Pts',(-37.1455454527048,8.99655532667588,-48.2747802767314));
#44380=CARTESIAN_POINT('Ctrl Pts',(-37.2034973491576,9.07697651567799,-49.1353231676698));
#44381=CARTESIAN_POINT('Ctrl Pts',(-37.3001167446471,9.20299194423899,-50.4014516292164));
#44382=CARTESIAN_POINT('Ctrl Pts',(-37.424112639288,9.32146046985706,-51.9759769909471));
#44383=CARTESIAN_POINT('Ctrl Pts',(-37.5026213956257,9.34328952661308,-53.0650482694175));
#44384=CARTESIAN_POINT('Ctrl Pts',(-37.5476337506195,9.32683669469911,-53.7605884615843));
#44385=CARTESIAN_POINT('Ctrl Pts',(-37.5665661126474,9.31272464671798,-54.0738284532984));
#44386=CARTESIAN_POINT('Ctrl Pts',(-37.6057031913977,9.26414962921768,-54.663337487995));
#44387=CARTESIAN_POINT('Ctrl Pts',(-37.6764662088264,9.13742110622336,-55.6615785587876));
#44388=CARTESIAN_POINT('Ctrl Pts',(-37.8164949562745,8.79806780322109,-57.4845265225189));
#44389=CARTESIAN_POINT('Ctrl Pts',(-37.9141915114532,8.61952768235194,-58.761476841605));
#44390=CARTESIAN_POINT('Ctrl Pts',(-37.9541952896336,8.66244269536972,-59.5035309748523));
#44391=CARTESIAN_POINT('Ctrl Pts',(-37.9587592236704,8.66957094444295,-59.6163026306148));
#44392=CARTESIAN_POINT('Ctrl Pts',(-37.9669276688694,8.68634443524689,-59.8301967046942));
#44393=CARTESIAN_POINT('Ctrl Pts',(-37.9787510920646,8.72419183715132,-60.2132581371599));
#44394=CARTESIAN_POINT('Ctrl Pts',(-37.9935384811198,8.83135451601754,-60.9838245730438));
#44395=CARTESIAN_POINT('Ctrl Pts',(-37.9948051042161,9.02173398324445,-61.885731569312));
#44396=CARTESIAN_POINT('Ctrl Pts',(-37.989617077741,9.26845024412025,-62.7989711447217));
#44397=CARTESIAN_POINT('Ctrl Pts',(-37.9859198864002,9.42587180626457,-63.3164647629597));
#44398=CARTESIAN_POINT('Ctrl Pts',(-37.9838015485123,9.53754686050424,-63.6623771036356));
#44399=CARTESIAN_POINT('Ctrl Pts',(-37.9825249382728,9.61371634326418,-63.8932483834881));
#44400=CARTESIAN_POINT('Ctrl Pts',(-37.9815185946865,9.69232843708823,-64.1243218214184));
#44401=CARTESIAN_POINT('Ctrl Pts',(-37.9809875763424,9.76308889151633,-64.3267502887585));
#44402=CARTESIAN_POINT('Ctrl Pts',(-37.9808002426337,9.80405805079477,-64.4424707032604));
#44403=CARTESIAN_POINT('Ctrl Pts',(-37.9806439053292,9.86602059892453,-64.6160649186278));
#44404=CARTESIAN_POINT('Ctrl Pts',(-37.9807887081246,9.91872513061641,-64.760831311268));
#44405=CARTESIAN_POINT('Ctrl Pts',(-37.9814928352743,10.0069714773366,-64.9998936835609));
#44406=CARTESIAN_POINT('Ctrl Pts',(-37.9826490650251,10.0893718431465,-65.2123548953848));
#44407=CARTESIAN_POINT('Ctrl Pts',(-37.9843492455442,10.2781728978025,-65.6621712721371));
#44408=CARTESIAN_POINT('Ctrl Pts',(-37.9866286590482,10.645795689941,-66.4512015386042));
#44409=CARTESIAN_POINT('Ctrl Pts',(-37.9879000851148,11.5250521960472,-68.0900185972829));
#44410=CARTESIAN_POINT('Ctrl Pts',(-37.9850730271635,12.423642682094,-69.5845303134357));
#44411=CARTESIAN_POINT('Ctrl Pts',(-37.9833124268618,13.0561024586398,-70.7862856454141));
#44412=CARTESIAN_POINT('Ctrl Pts',(-37.9834167705123,13.1849450671358,-71.0308400933947));
#44413=CARTESIAN_POINT('Ctrl Pts',(-37.9833552700991,13.4503457396783,-71.5333931190796));
#44414=CARTESIAN_POINT('Ctrl Pts',(-37.9834148605826,13.7803328254118,-72.1561449947392));
#44415=CARTESIAN_POINT('Ctrl Pts',(-37.9834441005009,14.1793852288138,-72.9068571737646));
#44416=CARTESIAN_POINT('Ctrl Pts',(-37.9835609738141,14.9788505997464,-74.4073744667933));
#44417=CARTESIAN_POINT('Ctrl Pts',(-37.9836479048135,15.6486830122308,-75.6601882148424));
#44418=CARTESIAN_POINT('Ctrl Pts',(-37.9835718534664,16.6204025035737,-77.4875159095769));
#44419=CARTESIAN_POINT('Ctrl Pts',(-37.9836050954401,17.0560964081388,-78.3068234984452));
#44420=CARTESIAN_POINT('Ctrl Pts',(-37.9836050954401,17.4926179955282,-79.1278012005436));
#44421=CARTESIAN_POINT('Ctrl Pts',(-36.8145414704191,4.17706810938354,24.8306393376479));
#44422=CARTESIAN_POINT('Ctrl Pts',(-36.8146506950273,4.17707182564265,24.7817601788696));
#44423=CARTESIAN_POINT('Ctrl Pts',(-36.8147652478949,4.17707572405304,24.7328820877382));
#44424=CARTESIAN_POINT('Ctrl Pts',(-36.8161179581993,4.17712171263977,24.182275474903));
#44425=CARTESIAN_POINT('Ctrl Pts',(-36.8171627107515,4.17715798726589,23.1781363569847));
#44426=CARTESIAN_POINT('Ctrl Pts',(-36.8195998551861,4.17724371941347,21.1695423782853));
#44427=CARTESIAN_POINT('Ctrl Pts',(-36.8286020356479,4.17754948633292,19.66539321355));
#44428=CARTESIAN_POINT('Ctrl Pts',(-36.8476544376428,4.17819248391852,18.4143478831888));
#44429=CARTESIAN_POINT('Ctrl Pts',(-36.8567956666284,4.17850085887141,17.9115338606246));
#44430=CARTESIAN_POINT('Ctrl Pts',(-36.8797573378532,4.17927517531058,16.9075428284866));
#44431=CARTESIAN_POINT('Ctrl Pts',(-36.9290069124392,4.18093483608638,15.1537199901826));
#44432=CARTESIAN_POINT('Ctrl Pts',(-36.9757452497305,4.18251067564459,13.6519464718781));
#44433=CARTESIAN_POINT('Ctrl Pts',(-37.0049439033556,4.18349506199556,12.3974580494044));
#44434=CARTESIAN_POINT('Ctrl Pts',(-37.0168690655117,4.18389716709014,11.896496347134));
#44435=CARTESIAN_POINT('Ctrl Pts',(-37.0411436577337,4.18471547900478,10.8946396040635));
#44436=CARTESIAN_POINT('Ctrl Pts',(-37.0711039027786,4.18572677788779,9.64208784240444));
#44437=CARTESIAN_POINT('Ctrl Pts',(-37.1026535454665,4.18679000665914,8.13758235446264));
#44438=CARTESIAN_POINT('Ctrl Pts',(-37.1182314109417,4.18731418915677,7.13287015374521));
#44439=CARTESIAN_POINT('Ctrl Pts',(-37.1254642281502,4.1875565209857,6.50489713067809));
#44440=CARTESIAN_POINT('Ctrl Pts',(-37.128155112656,4.18764613376774,6.25467125009352));
#44441=CARTESIAN_POINT('Ctrl Pts',(-37.1328167164426,4.18779971642136,5.75355956197867));
#44442=CARTESIAN_POINT('Ctrl Pts',(-37.1391750727683,4.18800414638075,4.87515574383194));
#44443=CARTESIAN_POINT('Ctrl Pts',(-37.1454177456287,4.18819017072339,3.11491456727999));
#44444=CARTESIAN_POINT('Ctrl Pts',(-37.1421588108841,4.18806139037958,1.60821253231155));
#44445=CARTESIAN_POINT('Ctrl Pts',(-37.1381315205537,4.18794334293428,0.548768836768961));
#44446=CARTESIAN_POINT('Ctrl Pts',(-37.1376027122731,4.18792827716166,0.422597518332732));
#44447=CARTESIAN_POINT('Ctrl Pts',(-37.1363583452212,4.18789230873776,0.170450774630366));
#44448=CARTESIAN_POINT('Ctrl Pts',(-37.1337143965635,4.18781547475265,-0.270307417104572));
#44449=CARTESIAN_POINT('Ctrl Pts',(-37.128739477224,4.18766826957105,-0.898708045971484));
#44450=CARTESIAN_POINT('Ctrl Pts',(-37.1212908405087,4.18744931772557,-1.65117956824175));
#44451=CARTESIAN_POINT('Ctrl Pts',(-37.1099619032053,4.1871129344279,-2.65302799518834));
#44452=CARTESIAN_POINT('Ctrl Pts',(-37.09427463321,4.1866465079283,-3.90365427999558));
#44453=CARTESIAN_POINT('Ctrl Pts',(-37.0824128175559,4.18629030821057,-4.90495429670346));
#44454=CARTESIAN_POINT('Ctrl Pts',(-37.0759419900389,4.18609948224038,-5.53177471628879));
#44455=CARTESIAN_POINT('Ctrl Pts',(-37.0734490733729,4.18601901608428,-5.78278322973631));
#44456=CARTESIAN_POINT('Ctrl Pts',(-37.068774466851,4.18584253793842,-6.28501209766204));
#44457=CARTESIAN_POINT('Ctrl Pts',(-37.0612153049882,4.18550176203556,-7.16444418145535));
#44458=CARTESIAN_POINT('Ctrl Pts',(-37.051088171976,4.18497049210318,-8.42122512102502));
#44459=CARTESIAN_POINT('Ctrl Pts',(-37.038885514991,4.18453356806039,-9.67567405245044));
#44460=CARTESIAN_POINT('Ctrl Pts',(-37.0276914499488,4.18435986985205,-10.5509869279345));
#44461=CARTESIAN_POINT('Ctrl Pts',(-37.0203151196171,4.18430562699315,-11.0502134500236));
#44462=CARTESIAN_POINT('Ctrl Pts',(-37.0162634821171,4.18429470100516,-11.2993853814344));
#44463=CARTESIAN_POINT('Ctrl Pts',(-37.0130611661426,4.18429260457632,-11.4871271373884));
#44464=CARTESIAN_POINT('Ctrl Pts',(-37.0110448690885,4.18398173723689,-11.6210508779523));
#44465=CARTESIAN_POINT('Ctrl Pts',(-37.0074948447866,4.18227085814457,-11.8829086291118));
#44466=CARTESIAN_POINT('Ctrl Pts',(-37.0023895368805,4.1767444699889,-12.3396792789109));
#44467=CARTESIAN_POINT('Ctrl Pts',(-36.9953355747988,4.15807514016592,-13.2368410977104));
#44468=CARTESIAN_POINT('Ctrl Pts',(-36.98692719984,4.1239517633785,-14.4787967330387));
#44469=CARTESIAN_POINT('Ctrl Pts',(-36.9639435464291,4.11490441611126,-15.552347252464));
#44470=CARTESIAN_POINT('Ctrl Pts',(-36.9350271873072,4.12865937629905,-16.252631627403));
#44471=CARTESIAN_POINT('Ctrl Pts',(-36.9116737747744,4.14363804540266,-16.7156276685256));
#44472=CARTESIAN_POINT('Ctrl Pts',(-36.8890848383236,4.16207307191748,-17.0587999422591));
#44473=CARTESIAN_POINT('Ctrl Pts',(-36.8669552974436,4.18202463484443,-17.3424822046825));
#44474=CARTESIAN_POINT('Ctrl Pts',(-36.8577331954662,4.19063519194624,-17.4597987335548));
#44475=CARTESIAN_POINT('Ctrl Pts',(-36.837750631618,4.20884846416802,-17.6922569789042));
#44476=CARTESIAN_POINT('Ctrl Pts',(-36.8155634200376,4.22888625981175,-17.9267206097568));
#44477=CARTESIAN_POINT('Ctrl Pts',(-36.7914693697599,4.25044510162083,-18.1616254051611));
#44478=CARTESIAN_POINT('Ctrl Pts',(-36.7756778369371,4.26454517607042,-18.308973522781));
#44479=CARTESIAN_POINT('Ctrl Pts',(-36.7626422312317,4.27617033658842,-18.4270538895154));
#44480=CARTESIAN_POINT('Ctrl Pts',(-36.7526738439219,4.28505922055653,-18.5157491412756));
#44481=CARTESIAN_POINT('Ctrl Pts',(-36.7442156277307,4.29260330675946,-18.5897585461262));
#44482=CARTESIAN_POINT('Ctrl Pts',(-36.7373621096969,4.29871796800706,-18.6490303045467));
#44483=CARTESIAN_POINT('Ctrl Pts',(-36.6786435611264,4.35114684308371,-19.1531722422004));
#44484=CARTESIAN_POINT('Ctrl Pts',(-36.5517941291924,4.4648025218755,-20.1274966208569));
#44485=CARTESIAN_POINT('Ctrl Pts',(-36.3629902843748,4.65825546096279,-21.5949066389794));
#44486=CARTESIAN_POINT('Ctrl Pts',(-36.258482687298,4.80650647098656,-22.5868678297255));
#44487=CARTESIAN_POINT('Ctrl Pts',(-36.2041312424173,4.90714442404014,-23.2071548394697));
#44488=CARTESIAN_POINT('Ctrl Pts',(-36.1842954084408,4.94560004507131,-23.4322288054636));
#44489=CARTESIAN_POINT('Ctrl Pts',(-36.1439879759796,5.03312209851521,-23.901369364868));
#44490=CARTESIAN_POINT('Ctrl Pts',(-36.0745253032527,5.20540870627714,-24.7326154565184));
#44491=CARTESIAN_POINT('Ctrl Pts',(-35.9763792540907,5.4960732899547,-25.967198555433));
#44492=CARTESIAN_POINT('Ctrl Pts',(-35.8638730883827,5.86559758195893,-27.5074586456592));
#44493=CARTESIAN_POINT('Ctrl Pts',(-35.7970238913048,6.08933924924599,-28.5741940065593));
#44494=CARTESIAN_POINT('Ctrl Pts',(-35.7639743896009,6.19771303571068,-29.1848272516722));
#44495=CARTESIAN_POINT('Ctrl Pts',(-35.7573496776361,6.22054498842897,-29.3138091203023));
#44496=CARTESIAN_POINT('Ctrl Pts',(-35.744157507517,6.26582226975952,-29.5752104980963));
#44497=CARTESIAN_POINT('Ctrl Pts',(-35.7222727087314,6.34236043846015,-30.0300178405691));
#44498=CARTESIAN_POINT('Ctrl Pts',(-35.6823716163915,6.48680121409233,-30.9378995013247));
#44499=CARTESIAN_POINT('Ctrl Pts',(-35.6360682369693,6.67203034121833,-32.2246917237026));
#44500=CARTESIAN_POINT('Ctrl Pts',(-35.602424279164,6.84043243075705,-33.4980677505866));
#44501=CARTESIAN_POINT('Ctrl Pts',(-35.5825233522388,6.97146434574046,-34.5073233082595));
#44502=CARTESIAN_POINT('Ctrl Pts',(-35.5747656005365,7.03676380952808,-35.0086292126765));
#44503=CARTESIAN_POINT('Ctrl Pts',(-35.5697386951994,7.08620366384295,-35.3844250261613));
#44504=CARTESIAN_POINT('Ctrl Pts',(-35.5665433265602,7.11965891412784,-35.6410715501154));
#44505=CARTESIAN_POINT('Ctrl Pts',(-35.562152378891,7.18553225339312,-36.150621600417));
#44506=CARTESIAN_POINT('Ctrl Pts',(-35.5587186405156,7.29894277838356,-37.0416973417176));
#44507=CARTESIAN_POINT('Ctrl Pts',(-35.5663553325028,7.51681414684123,-38.8159662755505));
#44508=CARTESIAN_POINT('Ctrl Pts',(-35.5869256269565,7.6868654242813,-40.3327515990101));
#44509=CARTESIAN_POINT('Ctrl Pts',(-35.600071936512,7.81648886757626,-41.5997097363398));
#44510=CARTESIAN_POINT('Ctrl Pts',(-35.6029973034266,7.85315812159936,-41.9863157305565));
#44511=CARTESIAN_POINT('Ctrl Pts',(-35.6065402637938,7.89782342059797,-42.4960833951206));
#44512=CARTESIAN_POINT('Ctrl Pts',(-35.6099161058435,7.94043513506824,-43.0059427141509));
#44513=CARTESIAN_POINT('Ctrl Pts',(-35.6143750775419,7.99051271915899,-43.6407347128252));
#44514=CARTESIAN_POINT('Ctrl Pts',(-35.6215523453426,8.04830994811261,-44.398876931035));
#44515=CARTESIAN_POINT('Ctrl Pts',(-35.6303514970611,8.09677619833867,-45.0268145521791));
#44516=CARTESIAN_POINT('Ctrl Pts',(-35.6398718628481,8.13700691506071,-45.5266306469361));
#44517=CARTESIAN_POINT('Ctrl Pts',(-35.648468541391,8.1682473135573,-45.9001070187702));
#44518=CARTESIAN_POINT('Ctrl Pts',(-35.6587338366661,8.2008710525493,-46.2721457927705));
#44519=CARTESIAN_POINT('Ctrl Pts',(-35.6749387045069,8.24660419070035,-46.7660688678912));
#44520=CARTESIAN_POINT('Ctrl Pts',(-35.6902809195264,8.28392755781832,-47.1341623966199));
#44521=CARTESIAN_POINT('Ctrl Pts',(-35.7082692818551,8.32385161219814,-47.500860791251));
#44522=CARTESIAN_POINT('Ctrl Pts',(-35.7216788552181,8.35174113882669,-47.7342227588538));
#44523=CARTESIAN_POINT('Ctrl Pts',(-35.7515901662072,8.41505553960775,-48.2137123367135));
#44524=CARTESIAN_POINT('Ctrl Pts',(-35.8120627570416,8.54067956461536,-49.0623306215748));
#44525=CARTESIAN_POINT('Ctrl Pts',(-35.9170717556947,8.74428194334892,-50.3163275049105));
#44526=CARTESIAN_POINT('Ctrl Pts',(-36.0593740981134,8.96238047461758,-51.8872068047178));
#44527=CARTESIAN_POINT('Ctrl Pts',(-36.1553810000668,9.04507524266935,-52.9838173650416));
#44528=CARTESIAN_POINT('Ctrl Pts',(-36.2124020013169,9.06172995327984,-53.6873700494853));
#44529=CARTESIAN_POINT('Ctrl Pts',(-36.2364593892998,9.06239337045504,-53.9978055411204));
#44530=CARTESIAN_POINT('Ctrl Pts',(-36.2877503511432,9.04237784569512,-54.5868399174417));
#44531=CARTESIAN_POINT('Ctrl Pts',(-36.3835699740437,8.9640044494523,-55.5855825795852));
#44532=CARTESIAN_POINT('Ctrl Pts',(-36.5813073250735,8.70846064059012,-57.4175989887824));
#44533=CARTESIAN_POINT('Ctrl Pts',(-36.7259019766856,8.56770686894578,-58.7072698807721));
#44534=CARTESIAN_POINT('Ctrl Pts',(-36.782338123889,8.62482634667821,-59.4707756675742));
#44535=CARTESIAN_POINT('Ctrl Pts',(-36.7887634890227,8.63400662213569,-59.5865773895651));
#44536=CARTESIAN_POINT('Ctrl Pts',(-36.8002731557661,8.65423114517781,-59.8059753328883));
#44537=CARTESIAN_POINT('Ctrl Pts',(-36.8169541787248,8.69719905574384,-60.1980565910176));
#44538=CARTESIAN_POINT('Ctrl Pts',(-36.8379285804888,8.81069057980454,-60.983438205225));
#44539=CARTESIAN_POINT('Ctrl Pts',(-36.8400324690854,9.0008653106084,-61.895075215011));
#44540=CARTESIAN_POINT('Ctrl Pts',(-36.833025237701,9.2428331962055,-62.8113508141628));
#44541=CARTESIAN_POINT('Ctrl Pts',(-36.8279560631062,9.39662372468876,-63.3282484325131));
#44542=CARTESIAN_POINT('Ctrl Pts',(-36.8250506657004,9.50579153322136,-63.6728480522941));
#44543=CARTESIAN_POINT('Ctrl Pts',(-36.8232987567908,9.58029320294315,-63.9026020207381));
#44544=CARTESIAN_POINT('Ctrl Pts',(-36.8219207850234,9.65727402391867,-64.1322082227681));
#44545=CARTESIAN_POINT('Ctrl Pts',(-36.8211968688644,9.72670407409752,-64.3330399111182));
#44546=CARTESIAN_POINT('Ctrl Pts',(-36.8209436600969,9.76694921258375,-64.4477593319922));
#44547=CARTESIAN_POINT('Ctrl Pts',(-36.8207356143094,9.827867991798,-64.6197666251074));
#44548=CARTESIAN_POINT('Ctrl Pts',(-36.820943020463,9.87979354233477,-64.7630215620431));
#44549=CARTESIAN_POINT('Ctrl Pts',(-36.8219192494767,9.96695386528716,-64.9994059056064));
#44550=CARTESIAN_POINT('Ctrl Pts',(-36.8231725041911,10.0495336392164,-65.2126160893504));
#44551=CARTESIAN_POINT('Ctrl Pts',(-36.82499495272,10.2379636953157,-65.6619525374483));
#44552=CARTESIAN_POINT('Ctrl Pts',(-36.8271181992213,10.6053251831302,-66.4511851584012));
#44553=CARTESIAN_POINT('Ctrl Pts',(-36.8272923782176,11.4838409823459,-68.0896332538814));
#44554=CARTESIAN_POINT('Ctrl Pts',(-36.8234065807366,12.3821608378723,-69.5844108199255));
#44555=CARTESIAN_POINT('Ctrl Pts',(-36.8218354649019,13.0144506626477,-70.786159996006));
#44556=CARTESIAN_POINT('Ctrl Pts',(-36.8218980779087,13.1432412485324,-71.0306777115429));
#44557=CARTESIAN_POINT('Ctrl Pts',(-36.8218129450693,13.4085677772461,-71.5331812361234));
#44558=CARTESIAN_POINT('Ctrl Pts',(-36.8218398088373,13.7384930297767,-72.1558847530838));
#44559=CARTESIAN_POINT('Ctrl Pts',(-36.8218623967062,14.137515020371,-72.9065507501415));
#44560=CARTESIAN_POINT('Ctrl Pts',(-36.8219908398845,14.936984438163,-74.4070081525254));
#44561=CARTESIAN_POINT('Ctrl Pts',(-36.8221312065847,15.6069267144729,-75.6598871290026));
#44562=CARTESIAN_POINT('Ctrl Pts',(-36.8220673386195,16.5787078435202,-77.4873463549366));
#44563=CARTESIAN_POINT('Ctrl Pts',(-36.8220955884565,17.0143863943048,-78.3066347591213));
#44564=CARTESIAN_POINT('Ctrl Pts',(-36.8220955884566,17.4509079816942,-79.1276124612196));
#44565=CARTESIAN_POINT('Ctrl Pts',(-35.8862883815749,4.14964241231811,24.8306453611339));
#44566=CARTESIAN_POINT('Ctrl Pts',(-35.8863946402816,4.14964559583046,24.781766398004));
#44567=CARTESIAN_POINT('Ctrl Pts',(-35.8865060824592,4.14964893562382,24.7328885041874));
#44568=CARTESIAN_POINT('Ctrl Pts',(-35.8878220796098,4.14968831258694,24.182284251377));
#44569=CARTESIAN_POINT('Ctrl Pts',(-35.8888338622136,4.1497223590721,23.1781482479736));
#44570=CARTESIAN_POINT('Ctrl Pts',(-35.8911909796499,4.14980495718219,21.1695585828577));
#44571=CARTESIAN_POINT('Ctrl Pts',(-35.8999488466652,4.15006655052355,19.6654120350873));
#44572=CARTESIAN_POINT('Ctrl Pts',(-35.918507596782,4.1506015914958,18.4143681228999));
#44573=CARTESIAN_POINT('Ctrl Pts',(-35.9274101115364,4.15085968205004,17.9115681746897));
#44574=CARTESIAN_POINT('Ctrl Pts',(-35.9497686326789,4.15151040993799,16.907587303699));
#44575=CARTESIAN_POINT('Ctrl Pts',(-35.9977262208149,4.15290448218856,15.1537628190788));
#44576=CARTESIAN_POINT('Ctrl Pts',(-36.0432641073147,4.1542076681852,13.651948151249));
#44577=CARTESIAN_POINT('Ctrl Pts',(-36.0717655121545,4.15498251426331,12.3974030081685));
#44578=CARTESIAN_POINT('Ctrl Pts',(-36.0834116029276,4.15529458500124,11.8964181254143));
#44579=CARTESIAN_POINT('Ctrl Pts',(-36.1071370294188,4.15591534395308,10.8945279252343));
#44580=CARTESIAN_POINT('Ctrl Pts',(-36.136444163004,4.1566621270959,9.6419569332076));
#44581=CARTESIAN_POINT('Ctrl Pts',(-36.1673368895585,4.15742625530908,8.13745839911925));
#44582=CARTESIAN_POINT('Ctrl Pts',(-36.1826020917766,4.1577946577808,7.13277408159323));
#44583=CARTESIAN_POINT('Ctrl Pts',(-36.1896949520552,4.15796306023695,6.50482106525867));
#44584=CARTESIAN_POINT('Ctrl Pts',(-36.1923388683203,4.15802189763918,6.25455986045041));
#44585=CARTESIAN_POINT('Ctrl Pts',(-36.1969369263861,4.1581106296951,5.75341435659549));
#44586=CARTESIAN_POINT('Ctrl Pts',(-36.2032535362139,4.15819691448695,4.87496918784217));
#44587=CARTESIAN_POINT('Ctrl Pts',(-36.2096128412279,4.15816654078512,3.11476734483232));
#44588=CARTESIAN_POINT('Ctrl Pts',(-36.2065231000555,4.15800477907593,1.60830836530141));
#44589=CARTESIAN_POINT('Ctrl Pts',(-36.2023901977377,4.15805498954621,0.549132646374202));
#44590=CARTESIAN_POINT('Ctrl Pts',(-36.2018474091026,4.15806236256343,0.423005400853475));
#44591=CARTESIAN_POINT('Ctrl Pts',(-36.2005696253334,4.15807930101949,0.170934716825099));
#44592=CARTESIAN_POINT('Ctrl Pts',(-36.1978539375442,4.15811533846752,-0.269699105975777));
#44593=CARTESIAN_POINT('Ctrl Pts',(-36.1927454283527,4.15817800690684,-0.897953119275321));
#44594=CARTESIAN_POINT('Ctrl Pts',(-36.185103668902,4.15827024278405,-1.65031602714938));
#44595=CARTESIAN_POINT('Ctrl Pts',(-36.1735015690339,4.15838989116868,-2.6520843755158));
#44596=CARTESIAN_POINT('Ctrl Pts',(-36.1574887428905,4.15852036661871,-3.90276838449031));
#44597=CARTESIAN_POINT('Ctrl Pts',(-36.1454832904363,4.15853186877887,-4.90425270890406));
#44598=CARTESIAN_POINT('Ctrl Pts',(-36.1389903705117,4.15849989683032,-5.53122578067775));
#44599=CARTESIAN_POINT('Ctrl Pts',(-36.1364213474791,4.15852132331837,-5.78169150779713));
#44600=CARTESIAN_POINT('Ctrl Pts',(-36.1313777044444,4.15867155979321,-6.28336956168771));
#44601=CARTESIAN_POINT('Ctrl Pts',(-36.122741714016,4.15914649121972,-7.16209558041097));
#44602=CARTESIAN_POINT('Ctrl Pts',(-36.11062700423,4.16002563108501,-8.41924559593771));
#44603=CARTESIAN_POINT('Ctrl Pts',(-36.0979378721441,4.16011467591934,-9.67574382559009));
#44604=CARTESIAN_POINT('Ctrl Pts',(-36.0882951212805,4.15920632450633,-10.5534752798069));
#44605=CARTESIAN_POINT('Ctrl Pts',(-36.0825016438357,4.1583296753329,-11.0543357491708));
#44606=CARTESIAN_POINT('Ctrl Pts',(-36.0794997434348,4.15775737267943,-11.3044371099148));
#44607=CARTESIAN_POINT('Ctrl Pts',(-36.0771950437572,4.15727094088865,-11.4928473165457));
#44608=CARTESIAN_POINT('Ctrl Pts',(-36.0757841290909,4.15669504852568,-11.6250424614838));
#44609=CARTESIAN_POINT('Ctrl Pts',(-36.0734605672477,4.1546897995167,-11.8849898120977));
#44610=CARTESIAN_POINT('Ctrl Pts',(-36.0705582594424,4.1491611106547,-12.338529623164));
#44611=CARTESIAN_POINT('Ctrl Pts',(-36.0682616272298,4.13188215694291,-13.232714440791));
#44612=CARTESIAN_POINT('Ctrl Pts',(-36.0684238134283,4.09998213405072,-14.4789694954568));
#44613=CARTESIAN_POINT('Ctrl Pts',(-36.0570757827599,4.08628902253444,-15.5672532812383));
#44614=CARTESIAN_POINT('Ctrl Pts',(-36.0381982641581,4.09230382197452,-16.2816087198696));
#44615=CARTESIAN_POINT('Ctrl Pts',(-36.0221580751819,4.10083040385787,-16.7550758926505));
#44616=CARTESIAN_POINT('Ctrl Pts',(-36.0057514960225,4.11285987052124,-17.1072248415648));
#44617=CARTESIAN_POINT('Ctrl Pts',(-35.9891607297069,4.12653843794509,-17.3989493347664));
#44618=CARTESIAN_POINT('Ctrl Pts',(-35.9823198969599,4.13242701942715,-17.5205098832969));
#44619=CARTESIAN_POINT('Ctrl Pts',(-35.9676474843925,4.1447016794492,-17.7602658762473));
#44620=CARTESIAN_POINT('Ctrl Pts',(-35.9515412202045,4.15801546224031,-18.001525451086));
#44621=CARTESIAN_POINT('Ctrl Pts',(-35.9341397743477,4.17221689876555,-18.2423215927065));
#44622=CARTESIAN_POINT('Ctrl Pts',(-35.9227524102192,4.18147118565899,-18.3930619490067));
#44623=CARTESIAN_POINT('Ctrl Pts',(-35.9133537783526,4.18908839335587,-18.513651392042));
#44624=CARTESIAN_POINT('Ctrl Pts',(-35.9061647785332,4.19490847302005,-18.6041351482638));
#44625=CARTESIAN_POINT('Ctrl Pts',(-35.9000612943855,4.19984592113213,-18.6795538907485));
#44626=CARTESIAN_POINT('Ctrl Pts',(-35.8951128771809,4.20384764031546,-18.7399050267767));
#44627=CARTESIAN_POINT('Ctrl Pts',(-35.8526921669526,4.2381583887282,-19.2529529861667));
#44628=CARTESIAN_POINT('Ctrl Pts',(-35.760254812392,4.31271623368857,-20.2358611422357));
#44629=CARTESIAN_POINT('Ctrl Pts',(-35.6112529180016,4.44665882940044,-21.6930146193082));
#44630=CARTESIAN_POINT('Ctrl Pts',(-35.5154493742871,4.55651940675062,-22.6659175228438));
#44631=CARTESIAN_POINT('Ctrl Pts',(-35.4592812336553,4.63398076469743,-23.2716923919344));
#44632=CARTESIAN_POINT('Ctrl Pts',(-35.4372505995826,4.66424453213448,-23.4962824133311));
#44633=CARTESIAN_POINT('Ctrl Pts',(-35.3907531102402,4.73347007409692,-23.9615642265644));
#44634=CARTESIAN_POINT('Ctrl Pts',(-35.305277650528,4.87131590316984,-24.7878810585807));
#44635=CARTESIAN_POINT('Ctrl Pts',(-35.1758847760366,5.10698704564035,-26.0159825559886));
#44636=CARTESIAN_POINT('Ctrl Pts',(-35.0251617842373,5.40948230024783,-27.5504638123744));
#44637=CARTESIAN_POINT('Ctrl Pts',(-34.9390560374465,5.59420259744437,-28.6124002756524));
#44638=CARTESIAN_POINT('Ctrl Pts',(-34.8983911824391,5.68406100232119,-29.2195884874086));
#44639=CARTESIAN_POINT('Ctrl Pts',(-34.8900265532928,5.70288570916111,-29.3476037983399));
#44640=CARTESIAN_POINT('Ctrl Pts',(-34.8734077068156,5.74036969201598,-29.6072368148802));
#44641=CARTESIAN_POINT('Ctrl Pts',(-34.845590131241,5.80393710757317,-30.0590182597113));
#44642=CARTESIAN_POINT('Ctrl Pts',(-34.7940841644091,5.92489230913247,-30.9614069392673));
#44643=CARTESIAN_POINT('Ctrl Pts',(-34.7319608996809,6.08300768791716,-32.2419080216104));
#44644=CARTESIAN_POINT('Ctrl Pts',(-34.6836000442781,6.2310247072079,-33.5114953241617));
#44645=CARTESIAN_POINT('Ctrl Pts',(-34.6527570741318,6.34855643808978,-34.5193896260131));
#44646=CARTESIAN_POINT('Ctrl Pts',(-34.6399400714304,6.40788861012915,-35.0206377216183));
#44647=CARTESIAN_POINT('Ctrl Pts',(-34.6312477397019,6.45304449511186,-35.3965836686083));
#44648=CARTESIAN_POINT('Ctrl Pts',(-34.6256995318638,6.48363888487945,-35.6521654141448));
#44649=CARTESIAN_POINT('Ctrl Pts',(-34.6166756023149,6.54450478408635,-36.1602930070773));
#44650=CARTESIAN_POINT('Ctrl Pts',(-34.6054976367161,6.65064325450614,-37.0486813865334));
#44651=CARTESIAN_POINT('Ctrl Pts',(-34.5985929019923,6.85999883007196,-38.8181150574146));
#44652=CARTESIAN_POINT('Ctrl Pts',(-34.6079843194644,7.03094019656917,-40.3310612298055));
#44653=CARTESIAN_POINT('Ctrl Pts',(-34.6122469819752,7.16449148557296,-41.5949163129102));
#44654=CARTESIAN_POINT('Ctrl Pts',(-34.6124779151437,7.20222495561867,-41.9827092555688));
#44655=CARTESIAN_POINT('Ctrl Pts',(-34.6127388112367,7.24813890723205,-42.4921260116324));
#44656=CARTESIAN_POINT('Ctrl Pts',(-34.6129391610133,7.29206616231259,-43.001417825639));
#44657=CARTESIAN_POINT('Ctrl Pts',(-34.6136397961648,7.34415615870572,-43.6344264110089));
#44658=CARTESIAN_POINT('Ctrl Pts',(-34.6164895533612,7.40579628834921,-44.388988882819));
#44659=CARTESIAN_POINT('Ctrl Pts',(-34.6217374437153,7.45932871493727,-45.0126410170983));
#44660=CARTESIAN_POINT('Ctrl Pts',(-34.6284138968991,7.50518355301202,-45.5082695504738));
#44661=CARTESIAN_POINT('Ctrl Pts',(-34.6348593583171,7.54150340913437,-45.8782017769925));
#44662=CARTESIAN_POINT('Ctrl Pts',(-34.642947844707,7.58017136010169,-46.2462884260783));
#44663=CARTESIAN_POINT('Ctrl Pts',(-34.65622333736,7.63538868340226,-46.7343837912956));
#44664=CARTESIAN_POINT('Ctrl Pts',(-34.6693039888815,7.68154214126522,-47.0974376750828));
#44665=CARTESIAN_POINT('Ctrl Pts',(-34.68504086039,7.7316813158421,-47.4586081772142));
#44666=CARTESIAN_POINT('Ctrl Pts',(-34.6971135255681,7.76674535176387,-47.6876879712688));
#44667=CARTESIAN_POINT('Ctrl Pts',(-34.7238675511503,7.84665764000097,-48.1596138295459));
#44668=CARTESIAN_POINT('Ctrl Pts',(-34.7781729950287,8.00639497600336,-48.9963097167226));
#44669=CARTESIAN_POINT('Ctrl Pts',(-34.8731749732318,8.27109386541086,-50.2376278605034));
#44670=CARTESIAN_POINT('Ctrl Pts',(-35.0063319813504,8.57410681218887,-51.8015718655458));
#44671=CARTESIAN_POINT('Ctrl Pts',(-35.1015618374688,8.71420329995202,-52.9017018699587));
#44672=CARTESIAN_POINT('Ctrl Pts',(-35.160871970943,8.76411916709648,-53.6106120097621));
#44673=CARTESIAN_POINT('Ctrl Pts',(-35.1860374687326,8.77929721972541,-53.9163395189235));
#44674=CARTESIAN_POINT('Ctrl Pts',(-35.2413576732862,8.78877244981892,-54.5018843049029));
#44675=CARTESIAN_POINT('Ctrl Pts',(-35.3480660504264,8.76265769681329,-55.4966936433364));
#44676=CARTESIAN_POINT('Ctrl Pts',(-35.5794804576178,8.6047778550797,-57.3345419063183));
#44677=CARTESIAN_POINT('Ctrl Pts',(-35.7570859886107,8.51263157414461,-58.6417003743386));
#44678=CARTESIAN_POINT('Ctrl Pts',(-35.8255593211804,8.58858922534792,-59.4316201891843));
#44679=CARTESIAN_POINT('Ctrl Pts',(-35.8333837380864,8.60041583723261,-59.550567178602));
#44680=CARTESIAN_POINT('Ctrl Pts',(-35.8475295837383,8.62516120799974,-59.7759386231754));
#44681=CARTESIAN_POINT('Ctrl Pts',(-35.8683787863595,8.67492305574173,-60.1776568829463));
#44682=CARTESIAN_POINT('Ctrl Pts',(-35.8961044631683,8.79731615480497,-60.9790075033711));
#44683=CARTESIAN_POINT('Ctrl Pts',(-35.9029595858914,8.98912101592088,-61.9014292473522));
#44684=CARTESIAN_POINT('Ctrl Pts',(-35.8990024346742,9.2278237708258,-62.8215390008787));
#44685=CARTESIAN_POINT('Ctrl Pts',(-35.895251208417,9.37872568359486,-63.3381346355321));
#44686=CARTESIAN_POINT('Ctrl Pts',(-35.8931550250171,9.48585299121616,-63.6815553093281));
#44687=CARTESIAN_POINT('Ctrl Pts',(-35.8919311575114,9.55898789419036,-63.9102650053807));
#44688=CARTESIAN_POINT('Ctrl Pts',(-35.891071831239,9.63462927284979,-64.138454184385));
#44689=CARTESIAN_POINT('Ctrl Pts',(-35.8908108483524,9.70296866963137,-64.337716001437));
#44690=CARTESIAN_POINT('Ctrl Pts',(-35.8908267513662,9.74262284984297,-64.4514456344633));
#44691=CARTESIAN_POINT('Ctrl Pts',(-35.8910279680724,9.8026931488241,-64.6218793627845));
#44692=CARTESIAN_POINT('Ctrl Pts',(-35.8915904528576,9.85399574762302,-64.7636268710383));
#44693=CARTESIAN_POINT('Ctrl Pts',(-35.8931818333317,9.94031508235885,-64.9973428837816));
#44694=CARTESIAN_POINT('Ctrl Pts',(-35.8948850335373,10.0234095492546,-65.2116626864872));
#44695=CARTESIAN_POINT('Ctrl Pts',(-35.8973657395788,10.2119700047034,-65.6609565696931));
#44696=CARTESIAN_POINT('Ctrl Pts',(-35.8999362720341,10.5797136472901,-66.4510848059395));
#44697=CARTESIAN_POINT('Ctrl Pts',(-35.8991950183312,11.4577636528938,-68.0898218646214));
#44698=CARTESIAN_POINT('Ctrl Pts',(-35.8936551391635,12.3550480594595,-69.5847771214724));
#44699=CARTESIAN_POINT('Ctrl Pts',(-35.8923188051878,12.9869272447527,-70.786025649498));
#44700=CARTESIAN_POINT('Ctrl Pts',(-35.8923642823853,13.1156897729242,-71.0305436169681));
#44701=CARTESIAN_POINT('Ctrl Pts',(-35.8922843116259,13.3809422470354,-71.5329860629288));
#44702=CARTESIAN_POINT('Ctrl Pts',(-35.8923005572825,13.7108226122191,-72.1556622624769));
#44703=CARTESIAN_POINT('Ctrl Pts',(-35.8923192925645,14.1098170297801,-72.9062849496283));
#44704=CARTESIAN_POINT('Ctrl Pts',(-35.8924355644065,14.9092943937856,-74.4066960770161));
#44705=CARTESIAN_POINT('Ctrl Pts',(-35.8925703043616,15.5793453086214,-75.6596486297005));
#44706=CARTESIAN_POINT('Ctrl Pts',(-35.8925151429371,16.5511896341262,-77.4872367171815));
#44707=CARTESIAN_POINT('Ctrl Pts',(-35.8925387824741,16.9868585707651,-78.3065132863522));
#44708=CARTESIAN_POINT('Ctrl Pts',(-35.8925387824741,17.4233801581546,-79.1274909884505));
#44709=CARTESIAN_POINT('Ctrl Pts',(-34.9576691493447,4.12599202383782,24.8306481986048));
#44710=CARTESIAN_POINT('Ctrl Pts',(-34.9577724821763,4.12599463491672,24.7817693216754));
#44711=CARTESIAN_POINT('Ctrl Pts',(-34.9578808561587,4.12599737399079,24.7328915142085));
#44712=CARTESIAN_POINT('Ctrl Pts',(-34.959160618967,4.12602966925197,24.1822883198965));
#44713=CARTESIAN_POINT('Ctrl Pts',(-34.9601402896146,4.12605960361354,23.1781538414392));
#44714=CARTESIAN_POINT('Ctrl Pts',(-34.9624198041354,4.12613330893548,21.1695660953823));
#44715=CARTESIAN_POINT('Ctrl Pts',(-34.9709368942797,4.12634777941475,19.6654208634938));
#44716=CARTESIAN_POINT('Ctrl Pts',(-34.9890064171506,4.12677640976453,18.4143777378113));
#44717=CARTESIAN_POINT('Ctrl Pts',(-34.9976724232657,4.12698427523286,17.9115850253704));
#44718=CARTESIAN_POINT('Ctrl Pts',(-35.0194340808931,4.12751030302748,16.9076093890702));
#44719=CARTESIAN_POINT('Ctrl Pts',(-35.0661121179879,4.12863692295904,15.1537840479596));
#44720=CARTESIAN_POINT('Ctrl Pts',(-35.1104636563205,4.12967484246056,13.6519484369461));
#44721=CARTESIAN_POINT('Ctrl Pts',(-35.1382705165157,4.13026347554627,12.3973742129691));
#44722=CARTESIAN_POINT('Ctrl Pts',(-35.1496380098962,4.1304972005787,11.8963776288467));
#44723=CARTESIAN_POINT('Ctrl Pts',(-35.1728125176182,4.13095111489406,10.8944707442092));
#44724=CARTESIAN_POINT('Ctrl Pts',(-35.2014663540684,4.13148068919542,9.64189165468456));
#44725=CARTESIAN_POINT('Ctrl Pts',(-35.231695669004,4.1320053583098,8.13739771584359));
#44726=CARTESIAN_POINT('Ctrl Pts',(-35.2466465556333,4.13225112713584,7.13272917219859));
#44727=CARTESIAN_POINT('Ctrl Pts',(-35.2535960572394,4.13236173488828,6.50478605588964));
#44728=CARTESIAN_POINT('Ctrl Pts',(-35.2561917324509,4.13239682594394,6.25449834718108));
#44729=CARTESIAN_POINT('Ctrl Pts',(-35.2607250047413,4.13243619754277,5.75332634083619));
#44730=CARTESIAN_POINT('Ctrl Pts',(-35.2670008280034,4.13243489544792,4.87484930711644));
#44731=CARTESIAN_POINT('Ctrl Pts',(-35.2734810059904,4.13224916658778,3.11467453054322));
#44732=CARTESIAN_POINT('Ctrl Pts',(-35.2705451432604,4.13208318410456,1.60840138381734));
#44733=CARTESIAN_POINT('Ctrl Pts',(-35.2662635206709,4.13227417673443,0.549427262601267));
#44734=CARTESIAN_POINT('Ctrl Pts',(-35.2657011781966,4.13229985044802,0.423333021829396));
#44735=CARTESIAN_POINT('Ctrl Pts',(-35.2643776199116,4.13235997560226,0.171319319719332));
#44736=CARTESIAN_POINT('Ctrl Pts',(-35.2615655281153,4.13248745582765,-0.269221346405241));
#44737=CARTESIAN_POINT('Ctrl Pts',(-35.256279454833,4.13272155600912,-0.897365165415799));
#44738=CARTESIAN_POINT('Ctrl Pts',(-35.2483844930824,4.1330622803331,-1.64964663634109));
#44739=CARTESIAN_POINT('Ctrl Pts',(-35.2364204078958,4.13354951665574,-2.65135422488508));
#44740=CARTESIAN_POINT('Ctrl Pts',(-35.2199669650849,4.13415426865972,-3.90208166627547));
#44741=CARTESIAN_POINT('Ctrl Pts',(-35.2077434624494,4.13446721075594,-4.90370529466454));
#44742=CARTESIAN_POINT('Ctrl Pts',(-35.2011938313991,4.1345652959299,-5.53080166020367));
#44743=CARTESIAN_POINT('Ctrl Pts',(-35.1985491560877,4.13465597637713,-5.78100351140501));
#44744=CARTESIAN_POINT('Ctrl Pts',(-35.193184404245,4.13500168172685,-6.28242334417115));
#44745=CARTESIAN_POINT('Ctrl Pts',(-35.1836501601607,4.13592996924364,-7.16081498294365));
#44746=CARTESIAN_POINT('Ctrl Pts',(-35.1699203342702,4.1375650349294,-8.41814973146324));
#44747=CARTESIAN_POINT('Ctrl Pts',(-35.1568489763635,4.13796350444972,-9.67565452057935));
#44748=CARTESIAN_POINT('Ctrl Pts',(-35.1484688577657,4.13672010875848,-10.5545861827495));
#44749=CARTESIAN_POINT('Ctrl Pts',(-35.1439609354925,4.13544997937989,-11.0562588986197));
#44750=CARTESIAN_POINT('Ctrl Pts',(-35.141810878656,4.13460750086697,-11.306833411016));
#44751=CARTESIAN_POINT('Ctrl Pts',(-35.1402343761306,4.13388694757193,-11.4955612126141));
#44752=CARTESIAN_POINT('Ctrl Pts',(-35.1393081495296,4.13321410289795,-11.6260501035739));
#44753=CARTESIAN_POINT('Ctrl Pts',(-35.1379408867715,4.13125114945088,-11.8839744204317));
#44754=CARTESIAN_POINT('Ctrl Pts',(-35.1366985116337,4.12632895965004,-12.3341277104814));
#44755=CARTESIAN_POINT('Ctrl Pts',(-35.1378308936329,4.11182271700753,-13.2248318815983));
#44756=CARTESIAN_POINT('Ctrl Pts',(-35.1441065414938,4.08496712983523,-14.4741394283709));
#44757=CARTESIAN_POINT('Ctrl Pts',(-35.1418197055586,4.07014756164377,-15.5751678386826));
#44758=CARTESIAN_POINT('Ctrl Pts',(-35.1313495071724,4.07073710575434,-16.3019891761704));
#44759=CARTESIAN_POINT('Ctrl Pts',(-35.121608184413,4.07430272641184,-16.7848166575302));
#44760=CARTESIAN_POINT('Ctrl Pts',(-35.1107864857476,4.08097893857506,-17.1451542089021));
#44761=CARTESIAN_POINT('Ctrl Pts',(-35.0993698341385,4.08919513124322,-17.444274461113));
#44762=CARTESIAN_POINT('Ctrl Pts',(-35.0947277707573,4.09267256341334,-17.5688300168412));
#44763=CARTESIAN_POINT('Ctrl Pts',(-35.0849897417642,4.09975826024745,-17.8141846015044));
#44764=CARTESIAN_POINT('Ctrl Pts',(-35.0745689837778,4.10725125569426,-18.0606167367435));
#44765=CARTESIAN_POINT('Ctrl Pts',(-35.0634683762102,4.11514971682738,-18.3060977674861));
#44766=CARTESIAN_POINT('Ctrl Pts',(-35.0562489157122,4.12027724003972,-18.4595759289252));
#44767=CARTESIAN_POINT('Ctrl Pts',(-35.0503046554234,4.12449618803505,-18.5822356495345));
#44768=CARTESIAN_POINT('Ctrl Pts',(-35.0457624107642,4.12772149878551,-18.6742136748583));
#44769=CARTESIAN_POINT('Ctrl Pts',(-35.0419073345998,4.13046087627797,-18.7508285633372));
#44770=CARTESIAN_POINT('Ctrl Pts',(-35.0387813322475,4.13268440455978,-18.8121067243344));
#44771=CARTESIAN_POINT('Ctrl Pts',(-35.0119742796186,4.15176585766008,-19.3328704769047));
#44772=CARTESIAN_POINT('Ctrl Pts',(-34.9532535258076,4.19404968236951,-20.3253393265434));
#44773=CARTESIAN_POINT('Ctrl Pts',(-34.8461218146786,4.27942771662531,-21.7816710285928));
#44774=CARTESIAN_POINT('Ctrl Pts',(-34.7622578092432,4.35679604434441,-22.7453677417508));
#44775=CARTESIAN_POINT('Ctrl Pts',(-34.706406162113,4.41359504135659,-23.3433389942894));
#44776=CARTESIAN_POINT('Ctrl Pts',(-34.6833510241288,4.43645887396516,-23.569994506372));
#44777=CARTESIAN_POINT('Ctrl Pts',(-34.6330016880252,4.4885780630418,-24.0356330706474));
#44778=CARTESIAN_POINT('Ctrl Pts',(-34.5360070120987,4.59281761600238,-24.8623897228399));
#44779=CARTESIAN_POINT('Ctrl Pts',(-34.3820291507108,4.77043318206014,-26.0866615025097));
#44780=CARTESIAN_POINT('Ctrl Pts',(-34.2022501573895,4.99816048642765,-27.6132729740688));
#44781=CARTESIAN_POINT('Ctrl Pts',(-34.1027071534334,5.1379235449416,-28.6661517966464));
#44782=CARTESIAN_POINT('Ctrl Pts',(-34.0571678319435,5.20670175305063,-29.2667089999963));
#44783=CARTESIAN_POINT('Ctrl Pts',(-34.0475707497204,5.22111959663242,-29.3938797417371));
#44784=CARTESIAN_POINT('Ctrl Pts',(-34.028604724881,5.24989871176608,-29.6515276224334));
#44785=CARTESIAN_POINT('Ctrl Pts',(-33.9966956201125,5.29886863680857,-30.1001465639621));
#44786=CARTESIAN_POINT('Ctrl Pts',(-33.9373100165154,5.39282960398277,-30.9966143632554));
#44787=CARTESIAN_POINT('Ctrl Pts',(-33.8645874739112,5.51821529383873,-32.2702458590929));
#44788=CARTESIAN_POINT('Ctrl Pts',(-33.8064510099774,5.63971813877035,-33.5349589050601));
#44789=CARTESIAN_POINT('Ctrl Pts',(-33.7683455906899,5.7389447926161,-34.5402288448051));
#44790=CARTESIAN_POINT('Ctrl Pts',(-33.7520623330603,5.7898959112938,-35.0406188720943));
#44791=CARTESIAN_POINT('Ctrl Pts',(-33.7408550265922,5.82900185369701,-35.4160583242001));
#44792=CARTESIAN_POINT('Ctrl Pts',(-33.7337120782534,5.85558598327124,-35.6703707812536));
#44793=CARTESIAN_POINT('Ctrl Pts',(-33.7214975953452,5.90909851202696,-36.1765585679139));
#44794=CARTESIAN_POINT('Ctrl Pts',(-33.7048437401063,6.00391340131153,-37.0614840895988));
#44795=CARTESIAN_POINT('Ctrl Pts',(-33.6871930062667,6.19640568017478,-38.8247048152405));
#44796=CARTESIAN_POINT('Ctrl Pts',(-33.6875279344711,6.36198945552724,-40.3331023868815));
#44797=CARTESIAN_POINT('Ctrl Pts',(-33.6841924063127,6.49458121699268,-41.5934174987506));
#44798=CARTESIAN_POINT('Ctrl Pts',(-33.6821137715501,6.53196170930422,-41.9824794946003));
#44799=CARTESIAN_POINT('Ctrl Pts',(-33.679556733124,6.5772536395265,-42.4914256240316));
#44800=CARTESIAN_POINT('Ctrl Pts',(-33.6770099690003,6.620695310972,-43.0000005480967));
#44801=CARTESIAN_POINT('Ctrl Pts',(-33.6743938165608,6.67262545242617,-43.6309140576139));
#44802=CARTESIAN_POINT('Ctrl Pts',(-33.6732482990849,6.73562411321624,-44.3813762849106));
#44803=CARTESIAN_POINT('Ctrl Pts',(-33.6750148369926,6.79223088432819,-45.0001966598899));
#44804=CARTESIAN_POINT('Ctrl Pts',(-33.6787189503938,6.84204581217287,-45.4911432491135));
#44805=CARTESIAN_POINT('Ctrl Pts',(-33.6828304981533,6.88220169762101,-45.8571387897004));
#44806=CARTESIAN_POINT('Ctrl Pts',(-33.6884615838597,6.92566096901639,-46.2208631850937));
#44807=CARTESIAN_POINT('Ctrl Pts',(-33.6982732935283,6.98864642005644,-46.7025690396419));
#44808=CARTESIAN_POINT('Ctrl Pts',(-33.7085346202646,7.04235764800512,-47.0601519723601));
#44809=CARTESIAN_POINT('Ctrl Pts',(-33.7212722467874,7.10134745665142,-47.4153765739217));
#44810=CARTESIAN_POINT('Ctrl Pts',(-33.7314208231614,7.14258540636038,-47.6399758670332));
#44811=CARTESIAN_POINT('Ctrl Pts',(-33.7534691984642,7.23698283658163,-48.1040531003266));
#44812=CARTESIAN_POINT('Ctrl Pts',(-33.7979240267016,7.42695396238463,-48.92862246813));
#44813=CARTESIAN_POINT('Ctrl Pts',(-33.8750212652659,7.74746631799993,-50.1571729190925));
#44814=CARTESIAN_POINT('Ctrl Pts',(-33.9860074859701,8.13149946354455,-51.7127427401713));
#44815=CARTESIAN_POINT('Ctrl Pts',(-34.0713501839444,8.32979075078484,-52.8140558450433));
#44816=CARTESIAN_POINT('Ctrl Pts',(-34.1279026169198,8.41488069409226,-53.5266584439897));
#44817=CARTESIAN_POINT('Ctrl Pts',(-34.1521464533961,8.44513849395254,-53.8262267687612));
#44818=CARTESIAN_POINT('Ctrl Pts',(-34.207293150626,8.48620986701366,-54.4060453279635));
#44819=CARTESIAN_POINT('Ctrl Pts',(-34.3175688808009,8.51763639437878,-55.3935232737951));
#44820=CARTESIAN_POINT('Ctrl Pts',(-34.5699847343345,8.47249989383399,-57.2344911268215));
#44821=CARTESIAN_POINT('Ctrl Pts',(-34.7746778991959,8.44131811526072,-58.5633838426194));
#44822=CARTESIAN_POINT('Ctrl Pts',(-34.8537635343935,8.54158719923408,-59.3846211416249));
#44823=CARTESIAN_POINT('Ctrl Pts',(-34.8628060411605,8.55674888349594,-59.5069065816396));
#44824=CARTESIAN_POINT('Ctrl Pts',(-34.8793880214111,8.58728052614665,-59.7388357980033));
#44825=CARTESIAN_POINT('Ctrl Pts',(-34.9043889070503,8.64584732171681,-60.1510438483319));
#44826=CARTESIAN_POINT('Ctrl Pts',(-34.9400432330761,8.78036742190039,-60.9699513878294));
#44827=CARTESIAN_POINT('Ctrl Pts',(-34.9549177016221,8.9761062550776,-61.9045297714664));
#44828=CARTESIAN_POINT('Ctrl Pts',(-34.9577338936852,9.21318808548523,-62.8293999036441));
#44829=CARTESIAN_POINT('Ctrl Pts',(-34.9573014231098,9.36195520020049,-63.346014853301));
#44830=CARTESIAN_POINT('Ctrl Pts',(-34.9572064571472,9.46749706221942,-63.6883948443447));
#44831=CARTESIAN_POINT('Ctrl Pts',(-34.9572605397201,9.53955730596001,-63.9161318348065));
#44832=CARTESIAN_POINT('Ctrl Pts',(-34.9575908470543,9.61413235727968,-64.1429475604759));
#44833=CARTESIAN_POINT('Ctrl Pts',(-34.9582951148639,9.68160942583985,-64.3406542831807));
#44834=CARTESIAN_POINT('Ctrl Pts',(-34.9588401780772,9.72079980598956,-64.4533965094004));
#44835=CARTESIAN_POINT('Ctrl Pts',(-34.9598126220336,9.78020955611649,-64.6222548455309));
#44836=CARTESIAN_POINT('Ctrl Pts',(-34.9609690699538,9.83103756829643,-64.7624807874525));
#44837=CARTESIAN_POINT('Ctrl Pts',(-34.9634776811836,9.91675954430774,-64.9935028616406));
#44838=CARTESIAN_POINT('Ctrl Pts',(-34.96591894868,10.0007393764809,-65.2093463422365));
#44839=CARTESIAN_POINT('Ctrl Pts',(-34.9694931577729,10.1899720025443,-65.6590816875894));
#44840=CARTESIAN_POINT('Ctrl Pts',(-34.9729628294964,10.5587860036188,-66.4508818038113));
#44841=CARTESIAN_POINT('Ctrl Pts',(-34.9713192854846,11.4366459032312,-68.0906323997746));
#44842=CARTESIAN_POINT('Ctrl Pts',(-34.9635298547312,12.3319946487882,-69.5856482008091));
#44843=CARTESIAN_POINT('Ctrl Pts',(-34.9624949509692,12.963182570155,-70.7858400367887));
#44844=CARTESIAN_POINT('Ctrl Pts',(-34.9625378096041,13.0919432799083,-71.0304000935673));
#44845=CARTESIAN_POINT('Ctrl Pts',(-34.9624838804023,13.3571207722334,-71.5327690442754));
#44846=CARTESIAN_POINT('Ctrl Pts',(-34.9625019627237,13.6869700850091,-72.1554406364071));
#44847=CARTESIAN_POINT('Ctrl Pts',(-34.9625174690599,14.0859380620031,-72.9060232117717));
#44848=CARTESIAN_POINT('Ctrl Pts',(-34.9626013152313,14.8854237837734,-74.4064026651871));
#44849=CARTESIAN_POINT('Ctrl Pts',(-34.9626837410002,15.5555645254436,-75.6594313764821));
#44850=CARTESIAN_POINT('Ctrl Pts',(-34.9626343711923,16.5274626633202,-77.4871400248605));
#44851=CARTESIAN_POINT('Ctrl Pts',(-34.962651678487,16.9631231181656,-78.3064115555001));
#44852=CARTESIAN_POINT('Ctrl Pts',(-34.9626516784869,17.399644705555,-79.1273892575985));
#44853=CARTESIAN_POINT('Ctrl Pts',(-33.6411326911163,4.10026185094264,24.8306459276114));
#44854=CARTESIAN_POINT('Ctrl Pts',(-33.6412319642584,4.10026360106523,24.7817669795734));
#44855=CARTESIAN_POINT('Ctrl Pts',(-33.6413360808126,4.10026543744567,24.7328890984256));
#44856=CARTESIAN_POINT('Ctrl Pts',(-33.6425655719406,4.10028706581328,24.1822851100102));
#44857=CARTESIAN_POINT('Ctrl Pts',(-33.6435016984766,4.10030759411697,23.1781500341781));
#44858=CARTESIAN_POINT('Ctrl Pts',(-33.6456766501809,4.10035873990036,21.1695607665509));
#44859=CARTESIAN_POINT('Ctrl Pts',(-33.6538592406256,4.10050219788364,19.6654154519402));
#44860=CARTESIAN_POINT('Ctrl Pts',(-33.6712444936077,4.10078633831224,18.4143725466167));
#44861=CARTESIAN_POINT('Ctrl Pts',(-33.6795800814252,4.10092488279933,17.9115781933392));
#44862=CARTESIAN_POINT('Ctrl Pts',(-33.7005079290768,4.10127689066396,16.9076016065011));
#44863=CARTESIAN_POINT('Ctrl Pts',(-33.7453987627603,4.10203095679594,15.1537767319238));
#44864=CARTESIAN_POINT('Ctrl Pts',(-33.7880838027813,4.10271762577904,13.6519492833216));
#44865=CARTESIAN_POINT('Ctrl Pts',(-33.8149066064565,4.10309050489671,12.3973832444834));
#44866=CARTESIAN_POINT('Ctrl Pts',(-33.8258787168521,4.1032365923497,11.8963903279294));
#44867=CARTESIAN_POINT('Ctrl Pts',(-33.8482694459468,4.10351371263629,10.894489599616));
#44868=CARTESIAN_POINT('Ctrl Pts',(-33.8759851887753,4.10382707692016,9.64191824077783));
#44869=CARTESIAN_POINT('Ctrl Pts',(-33.9052571194612,4.10412628544038,8.13742690599753));
#44870=CARTESIAN_POINT('Ctrl Pts',(-33.9197457328913,4.10426097418009,7.13275747992258));
#44871=CARTESIAN_POINT('Ctrl Pts',(-33.9264832272774,4.10432008724947,6.5048104286386));
#44872=CARTESIAN_POINT('Ctrl Pts',(-33.9290082793269,4.10433492266779,6.25450674375847));
#44873=CARTESIAN_POINT('Ctrl Pts',(-33.9334483969372,4.10433539753158,5.75331657478791));
#44874=CARTESIAN_POINT('Ctrl Pts',(-33.9396696168259,4.10427149430696,4.87481780318893));
#44875=CARTESIAN_POINT('Ctrl Pts',(-33.9463360604202,4.10399671666449,3.11465231775271));
#44876=CARTESIAN_POINT('Ctrl Pts',(-33.9435846569382,4.10385606244802,1.60848592985718));
#44877=CARTESIAN_POINT('Ctrl Pts',(-33.9389933726073,4.10415579520968,0.549631462269671));
#44878=CARTESIAN_POINT('Ctrl Pts',(-33.9383908140295,4.10419580157567,0.42355837231207));
#44879=CARTESIAN_POINT('Ctrl Pts',(-33.9369740111061,4.10428919894098,0.171580645918622));
#44880=CARTESIAN_POINT('Ctrl Pts',(-33.9339675769833,4.10448653180307,-0.26890088168996));
#44881=CARTESIAN_POINT('Ctrl Pts',(-33.9283281005373,4.10484830380246,-0.896973413154935));
#44882=CARTESIAN_POINT('Ctrl Pts',(-33.9199306318175,4.10537599982153,-1.6492033384174));
#44883=CARTESIAN_POINT('Ctrl Pts',(-33.9072484325072,4.10613579640971,-2.65086985568805));
#44884=CARTESIAN_POINT('Ctrl Pts',(-33.8899141021628,4.10709449182581,-3.9016334018584));
#44885=CARTESIAN_POINT('Ctrl Pts',(-33.8772276156682,4.10762512106839,-4.90334621637353));
#44886=CARTESIAN_POINT('Ctrl Pts',(-33.870536464046,4.10781629048305,-5.53054386391947));
#44887=CARTESIAN_POINT('Ctrl Pts',(-33.8677938414917,4.10793359346624,-5.78086565463426));
#44888=CARTESIAN_POINT('Ctrl Pts',(-33.8621020242897,4.10829656757102,-6.28243488902562));
#44889=CARTESIAN_POINT('Ctrl Pts',(-33.8517440194913,4.10917896514089,-7.16101104825188));
#44890=CARTESIAN_POINT('Ctrl Pts',(-33.8366414601763,4.11063653194915,-8.41828561880177));
#44891=CARTESIAN_POINT('Ctrl Pts',(-33.8233433932831,4.11099976811112,-9.67537954825846));
#44892=CARTESIAN_POINT('Ctrl Pts',(-33.8161444164405,4.10996469475177,-10.5538587598376));
#44893=CARTESIAN_POINT('Ctrl Pts',(-33.8127994565897,4.10890199074922,-11.0552106007861));
#44894=CARTESIAN_POINT('Ctrl Pts',(-33.8114108089721,4.10819573101564,-11.3056275282183));
#44895=CARTESIAN_POINT('Ctrl Pts',(-33.8104823372999,4.10759167960374,-11.4941670743556));
#44896=CARTESIAN_POINT('Ctrl Pts',(-33.8099681540024,4.10709912694592,-11.6224051077876));
#44897=CARTESIAN_POINT('Ctrl Pts',(-33.8093466060482,4.10580528279857,-11.8773977646603));
#44898=CARTESIAN_POINT('Ctrl Pts',(-33.8092393917502,4.10279420483067,-12.3226678483256));
#44899=CARTESIAN_POINT('Ctrl Pts',(-33.8122458515501,4.09433979998904,-13.2075524799972));
#44900=CARTESIAN_POINT('Ctrl Pts',(-33.8217592897651,4.07845534668309,-14.4585286523619));
#44901=CARTESIAN_POINT('Ctrl Pts',(-33.826957607454,4.06742061966935,-15.5735444655491));
#44902=CARTESIAN_POINT('Ctrl Pts',(-33.8249946539307,4.06478942374908,-16.3146866760876));
#44903=CARTESIAN_POINT('Ctrl Pts',(-33.8219696167977,4.06451266184445,-16.8083714860037));
#44904=CARTESIAN_POINT('Ctrl Pts',(-33.8174632618617,4.06620198770372,-17.1783068288034));
#44905=CARTESIAN_POINT('Ctrl Pts',(-33.8121471833676,4.06891067784961,-17.4860839934021));
#44906=CARTESIAN_POINT('Ctrl Pts',(-33.8100849824204,4.06996587647673,-17.6124840694276));
#44907=CARTESIAN_POINT('Ctrl Pts',(-33.806081214047,4.0719464040068,-17.8623067622636));
#44908=CARTESIAN_POINT('Ctrl Pts',(-33.8022014354793,4.07380820348422,-18.1126804113533));
#44909=CARTESIAN_POINT('Ctrl Pts',(-33.7983301480892,4.07565030346945,-18.362086011253));
#44910=CARTESIAN_POINT('Ctrl Pts',(-33.7958893750828,4.07681658210632,-18.5178991825193));
#44911=CARTESIAN_POINT('Ctrl Pts',(-33.7939097121451,4.07777090382214,-18.6423949041297));
#44912=CARTESIAN_POINT('Ctrl Pts',(-33.7924076996464,4.07850068069895,-18.7357232360661));
#44913=CARTESIAN_POINT('Ctrl Pts',(-33.7911385497741,4.0791231282861,-18.8134464020888));
#44914=CARTESIAN_POINT('Ctrl Pts',(-33.7901110297683,4.07963123050946,-18.8755990867573));
#44915=CARTESIAN_POINT('Ctrl Pts',(-33.7813013508289,4.08401178691256,-19.4037380359828));
#44916=CARTESIAN_POINT('Ctrl Pts',(-33.7619344413257,4.0945523600764,-20.4085240838739));
#44917=CARTESIAN_POINT('Ctrl Pts',(-33.7108942174128,4.12835178280623,-21.8787507168737));
#44918=CARTESIAN_POINT('Ctrl Pts',(-33.6512903133875,4.1694546614518,-22.8494396287991));
#44919=CARTESIAN_POINT('Ctrl Pts',(-33.6029153793199,4.20211921413237,-23.4511320389435));
#44920=CARTESIAN_POINT('Ctrl Pts',(-33.5820342108033,4.21590135193268,-23.6858582587801));
#44921=CARTESIAN_POINT('Ctrl Pts',(-33.5341979212337,4.2467529824973,-24.1612926439125));
#44922=CARTESIAN_POINT('Ctrl Pts',(-33.4367464051988,4.30772793100384,-25.0014216097737));
#44923=CARTESIAN_POINT('Ctrl Pts',(-33.2713525856663,4.40626964399774,-26.2283412604594));
#44924=CARTESIAN_POINT('Ctrl Pts',(-33.0732000001619,4.52288389107786,-27.7394229849092));
#44925=CARTESIAN_POINT('Ctrl Pts',(-32.966153269682,4.59294847833412,-28.7702324944338));
#44926=CARTESIAN_POINT('Ctrl Pts',(-32.9185127843775,4.62901401097156,-29.3551201315721));
#44927=CARTESIAN_POINT('Ctrl Pts',(-32.9081220344998,4.63671765787494,-29.4812765337408));
#44928=CARTESIAN_POINT('Ctrl Pts',(-32.8877533460928,4.65204508403021,-29.7355888702512));
#44929=CARTESIAN_POINT('Ctrl Pts',(-32.8533178540442,4.67828853827645,-30.1792586022513));
#44930=CARTESIAN_POINT('Ctrl Pts',(-32.7890377277273,4.72927355630562,-31.0660416354241));
#44931=CARTESIAN_POINT('Ctrl Pts',(-32.7096945706555,4.80034467398294,-32.3281471555683));
#44932=CARTESIAN_POINT('Ctrl Pts',(-32.645543075087,4.87557053433749,-33.5835486060134));
#44933=CARTESIAN_POINT('Ctrl Pts',(-32.6028255393445,4.94170126882913,-34.5827075325046));
#44934=CARTESIAN_POINT('Ctrl Pts',(-32.5843091448841,4.9773109596408,-35.0804869953707));
#44935=CARTESIAN_POINT('Ctrl Pts',(-32.5714311729237,5.00524972267996,-35.4540879938655));
#44936=CARTESIAN_POINT('Ctrl Pts',(-32.5632505675272,5.0244507512656,-35.7062386614517));
#44937=CARTESIAN_POINT('Ctrl Pts',(-32.5488818356357,5.06409381237342,-36.2088033664596));
#44938=CARTESIAN_POINT('Ctrl Pts',(-32.5283727865902,5.13675175346187,-37.0875504480415));
#44939=CARTESIAN_POINT('Ctrl Pts',(-32.5024985675524,5.29328057889031,-38.8399712834976));
#44940=CARTESIAN_POINT('Ctrl Pts',(-32.4943551753827,5.44071029761429,-40.3411442865328));
#44941=CARTESIAN_POINT('Ctrl Pts',(-32.4830885255742,5.56383169955982,-41.5961824692435));
#44942=CARTESIAN_POINT('Ctrl Pts',(-32.4785943977942,5.5983872109969,-41.987177810346));
#44943=CARTESIAN_POINT('Ctrl Pts',(-32.4730549529468,5.63986342477469,-42.4954123978076));
#44944=CARTESIAN_POINT('Ctrl Pts',(-32.4675331943491,5.67971433766435,-43.0028939982844));
#44945=CARTESIAN_POINT('Ctrl Pts',(-32.4611691477671,5.72785009583342,-43.6306186242469));
#44946=CARTESIAN_POINT('Ctrl Pts',(-32.4551335658941,5.78839748470127,-44.3748615626198));
#44947=CARTESIAN_POINT('Ctrl Pts',(-32.4522485725628,5.84546817355414,-44.9863862996825));
#44948=CARTESIAN_POINT('Ctrl Pts',(-32.4517460422648,5.89764344956478,-45.4703023591762));
#44949=CARTESIAN_POINT('Ctrl Pts',(-32.4524203330941,5.94064103534309,-45.8304087771301));
#44950=CARTESIAN_POINT('Ctrl Pts',(-32.4542962913942,5.98811752979867,-46.1876370266157));
#44951=CARTESIAN_POINT('Ctrl Pts',(-32.4586341263884,6.05816853842575,-46.6598808527028));
#44952=CARTESIAN_POINT('Ctrl Pts',(-32.4642005198337,6.11918888790148,-47.009441058689));
#44953=CARTESIAN_POINT('Ctrl Pts',(-32.4717830091301,6.18707038495651,-47.3560463636611));
#44954=CARTESIAN_POINT('Ctrl Pts',(-32.4784343104161,6.23444778201298,-47.5746165913903));
#44955=CARTESIAN_POINT('Ctrl Pts',(-32.491738375135,6.34340193121187,-48.0281241302287));
#44956=CARTESIAN_POINT('Ctrl Pts',(-32.5171296125407,6.56412915175324,-48.8368831289162));
#44957=CARTESIAN_POINT('Ctrl Pts',(-32.5571918409076,6.94345938666132,-50.0494377073212));
#44958=CARTESIAN_POINT('Ctrl Pts',(-32.6163517692873,7.419793013619,-51.5919017767001));
#44959=CARTESIAN_POINT('Ctrl Pts',(-32.671173221184,7.69197796679143,-52.6890339309171));
#44960=CARTESIAN_POINT('Ctrl Pts',(-32.7140153006268,7.82566351500892,-53.4017620163245));
#44961=CARTESIAN_POINT('Ctrl Pts',(-32.7331936544609,7.87607349739887,-53.6899524232844));
#44962=CARTESIAN_POINT('Ctrl Pts',(-32.7796961693441,7.96173857270317,-54.2566674391624));
#44963=CARTESIAN_POINT('Ctrl Pts',(-32.8792227654141,8.07816823912663,-55.2254883969868));
#44964=CARTESIAN_POINT('Ctrl Pts',(-33.1306365058374,8.21417318520405,-57.061460046734));
#44965=CARTESIAN_POINT('Ctrl Pts',(-33.3578423373758,8.29468476161207,-58.4293603073941));
#44966=CARTESIAN_POINT('Ctrl Pts',(-33.4479574718128,8.44121786586595,-59.3029834712513));
#44967=CARTESIAN_POINT('Ctrl Pts',(-33.4582700939901,8.46254072077173,-59.4299480885089));
#44968=CARTESIAN_POINT('Ctrl Pts',(-33.4777130686063,8.50398485229622,-59.6716354324499));
#44969=CARTESIAN_POINT('Ctrl Pts',(-33.5082643182909,8.57944022538127,-60.0992251957493));
#44970=CARTESIAN_POINT('Ctrl Pts',(-33.5569795000898,8.7387053594895,-60.9443011477612));
#44971=CARTESIAN_POINT('Ctrl Pts',(-33.5894256340183,8.94660383900336,-61.8977200611756));
#44972=CARTESIAN_POINT('Ctrl Pts',(-33.6092077650122,9.18702922879557,-62.8311702464978));
#44973=CARTESIAN_POINT('Ctrl Pts',(-33.6175011214833,9.33564698997536,-63.348830090218));
#44974=CARTESIAN_POINT('Ctrl Pts',(-33.6226392855976,9.44073841860971,-63.6904094221816));
#44975=CARTESIAN_POINT('Ctrl Pts',(-33.6260111407969,9.51243779257545,-63.9172154175434));
#44976=CARTESIAN_POINT('Ctrl Pts',(-33.6293782288212,9.58661034444336,-64.1425323012807));
#44977=CARTESIAN_POINT('Ctrl Pts',(-33.6324528341531,9.65378130604465,-64.3384287527984));
#44978=CARTESIAN_POINT('Ctrl Pts',(-33.6342644595799,9.69282161070932,-64.4499981222251));
#44979=CARTESIAN_POINT('Ctrl Pts',(-33.6370457909584,9.75203945725312,-64.6169660163557));
#44980=CARTESIAN_POINT('Ctrl Pts',(-33.6395144700785,9.80277974980643,-64.7553260994723));
#44981=CARTESIAN_POINT('Ctrl Pts',(-33.643901811797,9.88857364994285,-64.9830350846743));
#44982=CARTESIAN_POINT('Ctrl Pts',(-33.64795082258,9.97481551633586,-65.2020234088409));
#44983=CARTESIAN_POINT('Ctrl Pts',(-33.6539259758458,10.1666026322723,-65.6538302753117));
#44984=CARTESIAN_POINT('Ctrl Pts',(-33.6595924304936,10.5389370692624,-66.450124424042));
#44985=CARTESIAN_POINT('Ctrl Pts',(-33.6568032203678,11.4174925225938,-68.0934461183711));
#44986=CARTESIAN_POINT('Ctrl Pts',(-33.6448003690798,12.3077449575316,-69.5882021446881));
#44987=CARTESIAN_POINT('Ctrl Pts',(-33.6443502923429,12.9372441435451,-70.78536641954));
#44988=CARTESIAN_POINT('Ctrl Pts',(-33.644421177294,13.0660882833516,-71.0301126250275));
#44989=CARTESIAN_POINT('Ctrl Pts',(-33.6444502761828,13.3311776194155,-71.5323573056357));
#44990=CARTESIAN_POINT('Ctrl Pts',(-33.6445039851306,13.6610432733458,-72.1551025215315));
#44991=CARTESIAN_POINT('Ctrl Pts',(-33.6445190387081,14.0599875174264,-72.905650919379));
#44992=CARTESIAN_POINT('Ctrl Pts',(-33.6445189626518,14.8594904448648,-74.4060444270055));
#44993=CARTESIAN_POINT('Ctrl Pts',(-33.6444474180559,15.5296998311147,-75.6591844317331));
#44994=CARTESIAN_POINT('Ctrl Pts',(-33.6444118288596,16.5016455819358,-77.4870156479218));
#44995=CARTESIAN_POINT('Ctrl Pts',(-33.6444226998529,16.937307679145,-78.3063082760182));
#44996=CARTESIAN_POINT('Ctrl Pts',(-33.6444226998529,17.3738292665345,-79.1272859781166));
#44997=CARTESIAN_POINT('Ctrl Pts',(-31.9345162052867,4.08110750609352,24.8306358879163));
#44998=CARTESIAN_POINT('Ctrl Pts',(-31.9346105672387,4.08110819548476,24.7817566190947));
#44999=CARTESIAN_POINT('Ctrl Pts',(-31.9347095334598,4.08110891921601,24.7328784098582));
#45000=CARTESIAN_POINT('Ctrl Pts',(-31.9358781874058,4.08111743380434,24.1822706987579));
#45001=CARTESIAN_POINT('Ctrl Pts',(-31.9367672433101,4.08112326086448,23.1781322117713));
#45002=CARTESIAN_POINT('Ctrl Pts',(-31.9388326194472,4.08113679606785,21.1695357424094));
#45003=CARTESIAN_POINT('Ctrl Pts',(-31.946610252159,4.08119335240847,19.6653873712976));
#45004=CARTESIAN_POINT('Ctrl Pts',(-31.9631386790618,4.08131650188692,18.4143428073606));
#45005=CARTESIAN_POINT('Ctrl Pts',(-31.9710628413259,4.08137603223171,17.9115301783847));
#45006=CARTESIAN_POINT('Ctrl Pts',(-31.9909565725438,4.08152662960907,16.9075412729775));
#45007=CARTESIAN_POINT('Ctrl Pts',(-32.0336289154702,4.08185001958378,15.1537208236703));
#45008=CARTESIAN_POINT('Ctrl Pts',(-32.0742120066795,4.08215507985313,13.6519552942647));
#45009=CARTESIAN_POINT('Ctrl Pts',(-32.0997282221007,4.08233864079097,12.3974657568081));
#45010=CARTESIAN_POINT('Ctrl Pts',(-32.110167841507,4.0824130160868,11.8965046392989));
#45011=CARTESIAN_POINT('Ctrl Pts',(-32.1314779092244,4.08256217926155,10.894650705752));
#45012=CARTESIAN_POINT('Ctrl Pts',(-32.1578644090397,4.08274427283381,9.64211396348586));
#45013=CARTESIAN_POINT('Ctrl Pts',(-32.185737655173,4.08293120790136,8.13761947351068));
#45014=CARTESIAN_POINT('Ctrl Pts',(-32.1995331755596,4.08302108192031,7.13291957650245));
#45015=CARTESIAN_POINT('Ctrl Pts',(-32.2059464348698,4.08306126353903,6.50494606817195));
#45016=CARTESIAN_POINT('Ctrl Pts',(-32.2083604990054,4.08307323060974,6.25468682633457));
#45017=CARTESIAN_POINT('Ctrl Pts',(-32.2126422905571,4.0830836800604,5.75353858246067));
#45018=CARTESIAN_POINT('Ctrl Pts',(-32.2187298472004,4.08307184393253,4.87509428458592));
#45019=CARTESIAN_POINT('Ctrl Pts',(-32.2255176385181,4.08297792425966,3.11487633929514));
#45020=CARTESIAN_POINT('Ctrl Pts',(-32.2228927810643,4.0829308868657,1.6084311816116));
#45021=CARTESIAN_POINT('Ctrl Pts',(-32.217800225808,4.08307339977907,0.549250313299977));
#45022=CARTESIAN_POINT('Ctrl Pts',(-32.2171333159763,4.08309239505471,0.423122664200472));
#45023=CARTESIAN_POINT('Ctrl Pts',(-32.2155698373408,4.08313646376419,0.171051744769676));
#45024=CARTESIAN_POINT('Ctrl Pts',(-32.2122631461247,4.0832289645913,-0.269581450850985));
#45025=CARTESIAN_POINT('Ctrl Pts',(-32.2060878540656,4.08339696087033,-0.897818447216643));
#45026=CARTESIAN_POINT('Ctrl Pts',(-32.1969399867877,4.08363936646349,-1.65017409988339));
#45027=CARTESIAN_POINT('Ctrl Pts',(-32.183190880734,4.08398461266246,-2.65190200041652));
#45028=CARTESIAN_POINT('Ctrl Pts',(-32.1645543960765,4.08441089388571,-3.90256933832878));
#45029=CARTESIAN_POINT('Ctrl Pts',(-32.1511779928535,4.08463278729394,-4.90399868829054));
#45030=CARTESIAN_POINT('Ctrl Pts',(-32.1442675643117,4.08470349532937,-5.5310003029722));
#45031=CARTESIAN_POINT('Ctrl Pts',(-32.141443450968,4.08473411273331,-5.78184669019702));
#45032=CARTESIAN_POINT('Ctrl Pts',(-32.1356144713648,4.08479989308598,-6.28393036002289));
#45033=CARTESIAN_POINT('Ctrl Pts',(-32.1250866926104,4.08491789176519,-7.16315027258674));
#45034=CARTESIAN_POINT('Ctrl Pts',(-32.1099595557051,4.08504477551121,-8.41994436870759));
#45035=CARTESIAN_POINT('Ctrl Pts',(-32.0969731510966,4.08498556154858,-9.67493422699999));
#45036=CARTESIAN_POINT('Ctrl Pts',(-32.0901934533112,4.08477864334628,-10.5510367326364));
#45037=CARTESIAN_POINT('Ctrl Pts',(-32.0871489980332,4.08460301614872,-11.0507722276167));
#45038=CARTESIAN_POINT('Ctrl Pts',(-32.0859314968414,4.08449419906031,-11.300307995852));
#45039=CARTESIAN_POINT('Ctrl Pts',(-32.0851400403632,4.08440378635289,-11.4881079878802));
#45040=CARTESIAN_POINT('Ctrl Pts',(-32.084676479878,4.08433773003485,-11.6143548417818));
#45041=CARTESIAN_POINT('Ctrl Pts',(-32.0840061718684,4.08418441062924,-11.8665103449061));
#45042=CARTESIAN_POINT('Ctrl Pts',(-32.0834632744573,4.08386376022149,-12.3070815468493));
#45043=CARTESIAN_POINT('Ctrl Pts',(-32.0845437962985,4.08303573650382,-13.1857153042442));
#45044=CARTESIAN_POINT('Ctrl Pts',(-32.0902649196552,4.08146129759508,-14.4359144556652));
#45045=CARTESIAN_POINT('Ctrl Pts',(-32.0955399985264,4.07998696870516,-15.5604071811699));
#45046=CARTESIAN_POINT('Ctrl Pts',(-32.0970593246399,4.07920603201527,-16.3119948403646));
#45047=CARTESIAN_POINT('Ctrl Pts',(-32.0974049409017,4.07875737974352,-16.8137204991877));
#45048=CARTESIAN_POINT('Ctrl Pts',(-32.0967612035114,4.07851820934122,-17.1909384303492));
#45049=CARTESIAN_POINT('Ctrl Pts',(-32.0955591458867,4.0783944756999,-17.5052480643049));
#45050=CARTESIAN_POINT('Ctrl Pts',(-32.0951785331263,4.07830893422186,-17.6307678456597));
#45051=CARTESIAN_POINT('Ctrl Pts',(-32.0947611684075,4.07802153391888,-17.8811283588127));
#45052=CARTESIAN_POINT('Ctrl Pts',(-32.0947914435315,4.07757715679901,-18.1316402221286));
#45053=CARTESIAN_POINT('Ctrl Pts',(-32.0951376483372,4.07701687846767,-18.3819470814422));
#45054=CARTESIAN_POINT('Ctrl Pts',(-32.0954576236565,4.07662708311104,-18.5383852023367));
#45055=CARTESIAN_POINT('Ctrl Pts',(-32.0957593633384,4.07629641603794,-18.6635057855418));
#45056=CARTESIAN_POINT('Ctrl Pts',(-32.096004322397,4.0760403347023,-18.757339774025));
#45057=CARTESIAN_POINT('Ctrl Pts',(-32.0962205631789,4.07582129407088,-18.8355262789798));
#45058=CARTESIAN_POINT('Ctrl Pts',(-32.0963987625299,4.07564322482876,-18.898071110931));
#45059=CARTESIAN_POINT('Ctrl Pts',(-32.0979374503577,4.07411618025336,-19.4296779691492));
#45060=CARTESIAN_POINT('Ctrl Pts',(-32.1014062968753,4.07083947111897,-20.4453275036986));
#45061=CARTESIAN_POINT('Ctrl Pts',(-32.091375535163,4.07003834507895,-21.9437487586712));
#45062=CARTESIAN_POINT('Ctrl Pts',(-32.0634510847159,4.07541445937402,-22.9421936934073));
#45063=CARTESIAN_POINT('Ctrl Pts',(-32.0357377032757,4.08123731860324,-23.5642997091225));
#45064=CARTESIAN_POINT('Ctrl Pts',(-32.0234900765614,4.08369712503767,-23.8126150139849));
#45065=CARTESIAN_POINT('Ctrl Pts',(-31.9943240335294,4.08879366254401,-24.3087785223559));
#45066=CARTESIAN_POINT('Ctrl Pts',(-31.932439911088,4.09805349845175,-25.1792554912224));
#45067=CARTESIAN_POINT('Ctrl Pts',(-31.8208573144408,4.11046809917765,-26.4257905384195));
#45068=CARTESIAN_POINT('Ctrl Pts',(-31.6775527195453,4.12193231169977,-27.9237041412625));
#45069=CARTESIAN_POINT('Ctrl Pts',(-31.595374453496,4.13049764031296,-28.9218954202539));
#45070=CARTESIAN_POINT('Ctrl Pts',(-31.5582386843568,4.13771925254717,-29.4826943506793));
#45071=CARTESIAN_POINT('Ctrl Pts',(-31.5500189555754,4.13942333750784,-29.6081027205929));
#45072=CARTESIAN_POINT('Ctrl Pts',(-31.5338402768096,4.14276647064553,-29.8583896078162));
#45073=CARTESIAN_POINT('Ctrl Pts',(-31.5061516712207,4.14866697415491,-30.2964630238362));
#45074=CARTESIAN_POINT('Ctrl Pts',(-31.4533147605832,4.16085422920267,-31.1716237260119));
#45075=CARTESIAN_POINT('Ctrl Pts',(-31.3849763731538,4.18120722630591,-32.4191800851958));
#45076=CARTESIAN_POINT('Ctrl Pts',(-31.3259998043518,4.20990488447638,-33.6612396502691));
#45077=CARTESIAN_POINT('Ctrl Pts',(-31.2843934817152,4.2403661598899,-34.6505294036576));
#45078=CARTESIAN_POINT('Ctrl Pts',(-31.2654290237822,4.25847727968631,-35.1436267850304));
#45079=CARTESIAN_POINT('Ctrl Pts',(-31.2518693088976,4.2733344706328,-35.5137598748512));
#45080=CARTESIAN_POINT('Ctrl Pts',(-31.2431724656845,4.2837527640997,-35.7627596706265));
#45081=CARTESIAN_POINT('Ctrl Pts',(-31.2272701574211,4.30616475121193,-36.2597407094396));
#45082=CARTESIAN_POINT('Ctrl Pts',(-31.2029776219995,4.34943726527796,-37.1291764656129));
#45083=CARTESIAN_POINT('Ctrl Pts',(-31.165823696557,4.45072053840333,-38.8655146397168));
#45084=CARTESIAN_POINT('Ctrl Pts',(-31.1438789037403,4.55812564531563,-40.3573310700045));
#45085=CARTESIAN_POINT('Ctrl Pts',(-31.120153611262,4.65319699374158,-41.6062548905775));
#45086=CARTESIAN_POINT('Ctrl Pts',(-31.1120757642504,4.67970788253575,-42.0003677896081));
#45087=CARTESIAN_POINT('Ctrl Pts',(-31.1018334345682,4.71029481371404,-42.5080905849168));
#45088=CARTESIAN_POINT('Ctrl Pts',(-31.0915812944133,4.73947823418146,-43.0145361140732));
#45089=CARTESIAN_POINT('Ctrl Pts',(-31.0791134656114,4.77477568815216,-43.6384222354851));
#45090=CARTESIAN_POINT('Ctrl Pts',(-31.0650476942155,4.82135939840442,-44.3748291118715));
#45091=CARTESIAN_POINT('Ctrl Pts',(-31.0545718522228,4.86839730274684,-44.9770961573069));
#45092=CARTESIAN_POINT('Ctrl Pts',(-31.0472371746296,4.91371893662283,-45.4521586633428));
#45093=CARTESIAN_POINT('Ctrl Pts',(-31.0423675599914,4.95221094591703,-45.8049431946864));
#45094=CARTESIAN_POINT('Ctrl Pts',(-31.0382216264648,4.9958618067405,-46.1542263022132));
#45095=CARTESIAN_POINT('Ctrl Pts',(-31.0337940880935,5.06177203847355,-46.6151421119406));
#45096=CARTESIAN_POINT('Ctrl Pts',(-31.0318867398553,5.12083678396936,-46.955470509921));
#45097=CARTESIAN_POINT('Ctrl Pts',(-31.0311517246586,5.18760011055548,-47.2926014112459));
#45098=CARTESIAN_POINT('Ctrl Pts',(-31.0314818945205,5.23383985222584,-47.506807402411));
#45099=CARTESIAN_POINT('Ctrl Pts',(-31.0296295308109,5.34123088284672,-47.9522952786476));
#45100=CARTESIAN_POINT('Ctrl Pts',(-31.0223479986209,5.56141891612971,-48.7510880924636));
#45101=CARTESIAN_POINT('Ctrl Pts',(-31.0016701388276,5.95147806528555,-49.9552708220521));
#45102=CARTESIAN_POINT('Ctrl Pts',(-30.978041716002,6.46745316602708,-51.4855159642758));
#45103=CARTESIAN_POINT('Ctrl Pts',(-30.9811428160557,6.78945791405842,-52.5670112445759));
#45104=CARTESIAN_POINT('Ctrl Pts',(-30.9970510764194,6.96480480004668,-53.2670657700029));
#45105=CARTESIAN_POINT('Ctrl Pts',(-31.0064285723702,7.03170351427957,-53.5392492637444));
#45106=CARTESIAN_POINT('Ctrl Pts',(-31.0326877123139,7.15826974874841,-54.0831438919574));
#45107=CARTESIAN_POINT('Ctrl Pts',(-31.0979191767971,7.36020117964626,-55.0168985615787));
#45108=CARTESIAN_POINT('Ctrl Pts',(-31.2896973541456,7.70799341593398,-56.8222191651518));
#45109=CARTESIAN_POINT('Ctrl Pts',(-31.497485286898,7.96396009958822,-58.2388060297082));
#45110=CARTESIAN_POINT('Ctrl Pts',(-31.5887272365142,8.19120176241539,-59.1805492639164));
#45111=CARTESIAN_POINT('Ctrl Pts',(-31.5990764671936,8.2224649382114,-59.3108895456909));
#45112=CARTESIAN_POINT('Ctrl Pts',(-31.6197333534618,8.28260653878693,-59.5617233241845));
#45113=CARTESIAN_POINT('Ctrl Pts',(-31.6546315166755,8.38839280464436,-60.0031196869982));
#45114=CARTESIAN_POINT('Ctrl Pts',(-31.7201519725577,8.59874712174735,-60.8735024669699));
#45115=CARTESIAN_POINT('Ctrl Pts',(-31.7844306350037,8.84623710641239,-61.8476249668478));
#45116=CARTESIAN_POINT('Ctrl Pts',(-31.8381023844806,9.11392474038865,-62.7945648109811));
#45117=CARTESIAN_POINT('Ctrl Pts',(-31.86434745316,9.27444966434412,-63.3170202209645));
#45118=CARTESIAN_POINT('Ctrl Pts',(-31.88021843648,9.38649190763133,-63.660719691302));
#45119=CARTESIAN_POINT('Ctrl Pts',(-31.8903662560553,9.46259095181462,-63.8886476577213));
#45120=CARTESIAN_POINT('Ctrl Pts',(-31.8998665590296,9.54085525566165,-64.1146813512576));
#45121=CARTESIAN_POINT('Ctrl Pts',(-31.9076150710329,9.611406861697,-64.3108408424311));
#45122=CARTESIAN_POINT('Ctrl Pts',(-31.9118818780292,9.65233176333279,-64.4224604598438));
#45123=CARTESIAN_POINT('Ctrl Pts',(-31.9181213851423,9.7143368276467,-64.5894108045165));
#45124=CARTESIAN_POINT('Ctrl Pts',(-31.9229860229439,9.76731811762333,-64.7275449754731));
#45125=CARTESIAN_POINT('Ctrl Pts',(-31.9306003920534,9.85682715760974,-64.9547647015626));
#45126=CARTESIAN_POINT('Ctrl Pts',(-31.9375255667317,9.94891926487566,-65.1800840300211));
#45127=CARTESIAN_POINT('Ctrl Pts',(-31.9478464044456,10.1491387361118,-65.6392670359826));
#45128=CARTESIAN_POINT('Ctrl Pts',(-31.9578012633066,10.532255897598,-66.4475219583118));
#45129=CARTESIAN_POINT('Ctrl Pts',(-31.9541438804769,11.4152325015982,-68.1022353353483));
#45130=CARTESIAN_POINT('Ctrl Pts',(-31.9354552882024,12.2921436404521,-69.5953401290514));
#45131=CARTESIAN_POINT('Ctrl Pts',(-31.9359968812566,12.9175177203876,-70.7840181532909));
#45132=CARTESIAN_POINT('Ctrl Pts',(-31.9361668766121,13.0467763077856,-71.0294219679257));
#45133=CARTESIAN_POINT('Ctrl Pts',(-31.9363879221274,13.3118785132307,-71.5314973325199));
#45134=CARTESIAN_POINT('Ctrl Pts',(-31.9365470443432,13.6420033726205,-72.1546266983309));
#45135=CARTESIAN_POINT('Ctrl Pts',(-31.9365676954674,14.0409873041072,-72.9052454390513));
#45136=CARTESIAN_POINT('Ctrl Pts',(-31.9363854854439,14.8405233797907,-74.4058924595146));
#45137=CARTESIAN_POINT('Ctrl Pts',(-31.9359498821979,15.5105306107026,-75.6591137597579));
#45138=CARTESIAN_POINT('Ctrl Pts',(-31.9359321500433,16.4823855390668,-77.4868224586133));
#45139=CARTESIAN_POINT('Ctrl Pts',(-31.9359354932352,16.9181033333288,-78.3062452673089));
#45140=CARTESIAN_POINT('Ctrl Pts',(-31.9359354932352,17.3546249207183,-79.1272229694073));
#45141=CARTESIAN_POINT('Ctrl Pts',(-30.0675473741683,4.07402549386851,24.830628633993));
#45142=CARTESIAN_POINT('Ctrl Pts',(-30.0676366759476,4.07402543500512,24.7817491347503));
#45143=CARTESIAN_POINT('Ctrl Pts',(-30.067730334401,4.07402537490366,24.7328706888072));
#45144=CARTESIAN_POINT('Ctrl Pts',(-30.0688363277657,4.07402460311166,24.1822603333702));
#45145=CARTESIAN_POINT('Ctrl Pts',(-30.069681950142,4.07402006626856,23.1781204513434));
#45146=CARTESIAN_POINT('Ctrl Pts',(-30.0716489051951,4.07400793801025,21.1695184120988));
#45147=CARTESIAN_POINT('Ctrl Pts',(-30.0790094820679,4.07400246356816,19.6653665885618));
#45148=CARTESIAN_POINT('Ctrl Pts',(-30.0946304835923,4.0740102214446,18.4143194714129));
#45149=CARTESIAN_POINT('Ctrl Pts',(-30.1021211614365,4.07401293360225,17.9114920744124));
#45150=CARTESIAN_POINT('Ctrl Pts',(-30.1209291982291,4.07401803581239,16.9074937602044));
#45151=CARTESIAN_POINT('Ctrl Pts',(-30.1612714480777,4.074030090798,15.1536795468699));
#45152=CARTESIAN_POINT('Ctrl Pts',(-30.1996133066813,4.07405994681501,13.651966132142));
#45153=CARTESIAN_POINT('Ctrl Pts',(-30.2236762095638,4.07411155133605,12.3975373877242));
#45154=CARTESIAN_POINT('Ctrl Pts',(-30.2335165820057,4.07413652326603,11.8966014769226));
#45155=CARTESIAN_POINT('Ctrl Pts',(-30.2535882688967,4.07419984851666,10.8947841219751));
#45156=CARTESIAN_POINT('Ctrl Pts',(-30.2784183179358,4.07429593923365,9.64227346611599));
#45157=CARTESIAN_POINT('Ctrl Pts',(-30.3046226897621,4.0744145370772,8.13777604509942));
#45158=CARTESIAN_POINT('Ctrl Pts',(-30.3175799472559,4.07447773461984,7.13305118041901));
#45159=CARTESIAN_POINT('Ctrl Pts',(-30.3235995672069,4.07450799535757,6.50506041678156));
#45160=CARTESIAN_POINT('Ctrl Pts',(-30.3258729588873,4.07452529032412,6.25491067506208));
#45161=CARTESIAN_POINT('Ctrl Pts',(-30.3299307987399,4.07457685129505,5.75387614073744));
#45162=CARTESIAN_POINT('Ctrl Pts',(-30.3357596574654,4.07469880379446,4.87557589426331));
#45163=CARTESIAN_POINT('Ctrl Pts',(-30.3424189826996,4.07499137876109,3.11525589207107));
#45164=CARTESIAN_POINT('Ctrl Pts',(-30.3398667713788,4.07500554796219,1.60812326185725));
#45165=CARTESIAN_POINT('Ctrl Pts',(-30.3344478538389,4.07463707762726,0.548138186438529));
#45166=CARTESIAN_POINT('Ctrl Pts',(-30.3337393879005,4.07458997060624,0.421871593996724));
#45167=CARTESIAN_POINT('Ctrl Pts',(-30.332083641622,4.07447996188512,0.169564940125542));
#45168=CARTESIAN_POINT('Ctrl Pts',(-30.3285930551385,4.07425009251407,-0.271453082833765));
#45169=CARTESIAN_POINT('Ctrl Pts',(-30.3221036411615,4.0738244063566,-0.900113259040177));
#45170=CARTESIAN_POINT('Ctrl Pts',(-30.3125287108398,4.0732171318043,-1.65278904064886));
#45171=CARTESIAN_POINT('Ctrl Pts',(-30.2981953567222,4.07232465713225,-2.65468422165601));
#45172=CARTESIAN_POINT('Ctrl Pts',(-30.2788828023857,4.07118793598993,-3.90508783659838));
#45173=CARTESIAN_POINT('Ctrl Pts',(-30.2652180597821,4.07048380211638,-4.90578336174276));
#45174=CARTESIAN_POINT('Ctrl Pts',(-30.2582638943793,4.07019480836563,-5.5321987470797));
#45175=CARTESIAN_POINT('Ctrl Pts',(-30.2554674208861,4.07006342905616,-5.78335271280684));
#45176=CARTESIAN_POINT('Ctrl Pts',(-30.2498451412354,4.06974933691546,-6.28562567869495));
#45177=CARTESIAN_POINT('Ctrl Pts',(-30.2399996373138,4.0691059874119,-7.16506706819149));
#45178=CARTESIAN_POINT('Ctrl Pts',(-30.2263213749604,4.0681550594497,-8.42127536722444));
#45179=CARTESIAN_POINT('Ctrl Pts',(-30.2142344838837,4.06779375757901,-9.6746658182018));
#45180=CARTESIAN_POINT('Ctrl Pts',(-30.2071749736404,4.06818177662064,-10.5490624344194));
#45181=CARTESIAN_POINT('Ctrl Pts',(-30.2036219784775,4.0686333078625,-11.047660424527));
#45182=CARTESIAN_POINT('Ctrl Pts',(-30.2020193523223,4.06894315636935,-11.2965754227479));
#45183=CARTESIAN_POINT('Ctrl Pts',(-30.2008828480245,4.06921141590645,-11.4838718769006));
#45184=CARTESIAN_POINT('Ctrl Pts',(-30.2001418485536,4.06942052903896,-11.6092503899531));
#45185=CARTESIAN_POINT('Ctrl Pts',(-30.1987489579567,4.06994714066987,-11.8600866123641));
#45186=CARTESIAN_POINT('Ctrl Pts',(-30.1965370296849,4.07113030733344,-12.2984702198424));
#45187=CARTESIAN_POINT('Ctrl Pts',(-30.1929519161861,4.07435959782404,-13.1739479246322));
#45188=CARTESIAN_POINT('Ctrl Pts',(-30.1898527505392,4.08044633503893,-14.4229139491848));
#45189=CARTESIAN_POINT('Ctrl Pts',(-30.1886103060245,4.08523009014515,-15.5503981026885));
#45190=CARTESIAN_POINT('Ctrl Pts',(-30.1880553727537,4.08710042461392,-16.3056759814081));
#45191=CARTESIAN_POINT('Ctrl Pts',(-30.1877324707432,4.0879276757656,-16.8102984030727));
#45192=CARTESIAN_POINT('Ctrl Pts',(-30.1875161787576,4.08798924987499,-17.1902005082812));
#45193=CARTESIAN_POINT('Ctrl Pts',(-30.1873176376361,4.087649726645,-17.5068895628413));
#45194=CARTESIAN_POINT('Ctrl Pts',(-30.1872864991048,4.08753026540084,-17.6309577100965));
#45195=CARTESIAN_POINT('Ctrl Pts',(-30.1873954803442,4.08732989101367,-17.8801050928944));
#45196=CARTESIAN_POINT('Ctrl Pts',(-30.1877395017226,4.08717171477966,-18.1292535832108));
#45197=CARTESIAN_POINT('Ctrl Pts',(-30.188272206513,4.08702454294921,-18.3788607310938));
#45198=CARTESIAN_POINT('Ctrl Pts',(-30.1886744597833,4.08692973609548,-18.5349573794094));
#45199=CARTESIAN_POINT('Ctrl Pts',(-30.1890320505783,4.08684843166254,-18.6599241566505));
#45200=CARTESIAN_POINT('Ctrl Pts',(-30.1893167576907,4.08678357731685,-18.7536843811132));
#45201=CARTESIAN_POINT('Ctrl Pts',(-30.1895665721995,4.08672547288396,-18.8318516893039));
#45202=CARTESIAN_POINT('Ctrl Pts',(-30.1897732558483,4.08667606963648,-18.8944041645065));
#45203=CARTESIAN_POINT('Ctrl Pts',(-30.1915663197643,4.08623841124574,-19.4262122114691));
#45204=CARTESIAN_POINT('Ctrl Pts',(-30.1961051285031,4.084756062735,-20.4465526066575));
#45205=CARTESIAN_POINT('Ctrl Pts',(-30.2000726864718,4.0767318936048,-21.9637745112584));
#45206=CARTESIAN_POINT('Ctrl Pts',(-30.1970612147022,4.06469762621023,-22.9826839794627));
#45207=CARTESIAN_POINT('Ctrl Pts',(-30.1922398076992,4.05430688545523,-23.6202436765408));
#45208=CARTESIAN_POINT('Ctrl Pts',(-30.1900841185594,4.04954170941843,-23.8762747110122));
#45209=CARTESIAN_POINT('Ctrl Pts',(-30.1849026782126,4.038054721385,-24.3851642562897));
#45210=CARTESIAN_POINT('Ctrl Pts',(-30.1737620723978,4.01359240397717,-25.2744023890998));
#45211=CARTESIAN_POINT('Ctrl Pts',(-30.153374942618,3.97123564483179,-26.5359941979714));
#45212=CARTESIAN_POINT('Ctrl Pts',(-30.125265030707,3.92399396408896,-28.0332589680397));
#45213=CARTESIAN_POINT('Ctrl Pts',(-30.1064831648513,3.90367821899851,-29.017034788648));
#45214=CARTESIAN_POINT('Ctrl Pts',(-30.0966406455218,3.89767197354323,-29.5657610185313));
#45215=CARTESIAN_POINT('Ctrl Pts',(-30.0944609291319,3.89633147642119,-29.6910552886119));
#45216=CARTESIAN_POINT('Ctrl Pts',(-30.0900751736587,3.89382702416348,-29.9397090057612));
#45217=CARTESIAN_POINT('Ctrl Pts',(-30.0823646844887,3.88984108615631,-30.3757454776289));
#45218=CARTESIAN_POINT('Ctrl Pts',(-30.0667267592323,3.8836768128489,-31.2466347196678));
#45219=CARTESIAN_POINT('Ctrl Pts',(-30.0437366592632,3.88081109793407,-32.4893336913118));
#45220=CARTESIAN_POINT('Ctrl Pts',(-30.0195566094771,3.88798774614015,-33.7272588745916));
#45221=CARTESIAN_POINT('Ctrl Pts',(-29.99929937702,3.90098056847106,-34.713666847604));
#45222=CARTESIAN_POINT('Ctrl Pts',(-29.9889033231973,3.91007156124506,-35.205463866196));
#45223=CARTESIAN_POINT('Ctrl Pts',(-29.9809496953176,3.91795641437902,-35.5746304575847));
#45224=CARTESIAN_POINT('Ctrl Pts',(-29.9757247956522,3.92359657690754,-35.8222355664664));
#45225=CARTESIAN_POINT('Ctrl Pts',(-29.9655909133275,3.93621230622192,-36.3168732239133));
#45226=CARTESIAN_POINT('Ctrl Pts',(-29.9485042705045,3.96170418644016,-37.1822130401085));
#45227=CARTESIAN_POINT('Ctrl Pts',(-29.9148282975304,4.02477077950527,-38.9112115550624));
#45228=CARTESIAN_POINT('Ctrl Pts',(-29.8803151829792,4.09588590235412,-40.3991715419146));
#45229=CARTESIAN_POINT('Ctrl Pts',(-29.8409368948539,4.16016983935756,-41.645949356613));
#45230=CARTESIAN_POINT('Ctrl Pts',(-29.8287653164624,4.17737158193141,-42.0423769521704));
#45231=CARTESIAN_POINT('Ctrl Pts',(-29.812285671004,4.19545129807948,-42.550403082089));
#45232=CARTESIAN_POINT('Ctrl Pts',(-29.7954272548127,4.21204061790188,-43.0568282251492));
#45233=CARTESIAN_POINT('Ctrl Pts',(-29.7736265859651,4.23139475890916,-43.679106759112));
#45234=CARTESIAN_POINT('Ctrl Pts',(-29.7459868576208,4.25826632456728,-44.4114653271861));
#45235=CARTESIAN_POINT('Ctrl Pts',(-29.7216040642617,4.28808117317888,-45.0085382005776));
#45236=CARTESIAN_POINT('Ctrl Pts',(-29.7013125022927,4.31888083235695,-45.4784239432683));
#45237=CARTESIAN_POINT('Ctrl Pts',(-29.6856987012504,4.34606221934751,-45.8268876643508));
#45238=CARTESIAN_POINT('Ctrl Pts',(-29.6697101706248,4.37791652624086,-46.1714516272928));
#45239=CARTESIAN_POINT('Ctrl Pts',(-29.6479468882477,4.42737618133044,-46.6256554120005));
#45240=CARTESIAN_POINT('Ctrl Pts',(-29.6311296267172,4.4732106611538,-46.9605697088143));
#45241=CARTESIAN_POINT('Ctrl Pts',(-29.6140874606994,4.52607833559169,-47.2924570705504));
#45242=CARTESIAN_POINT('Ctrl Pts',(-29.601454255548,4.56334903637515,-47.5109312911585));
#45243=CARTESIAN_POINT('Ctrl Pts',(-29.5715572021337,4.64912737284354,-47.9589282930229));
#45244=CARTESIAN_POINT('Ctrl Pts',(-29.5095826736441,4.82546368650228,-48.7609818353961));
#45245=CARTESIAN_POINT('Ctrl Pts',(-29.4060280130564,5.14309673276399,-49.9598599459976));
#45246=CARTESIAN_POINT('Ctrl Pts',(-29.2939203496264,5.5865688094809,-51.4683674505085));
#45247=CARTESIAN_POINT('Ctrl Pts',(-29.2506392080023,5.89078625919428,-52.5164596458079));
#45248=CARTESIAN_POINT('Ctrl Pts',(-29.2424084661624,6.07296061824513,-53.1860502356983));
#45249=CARTESIAN_POINT('Ctrl Pts',(-29.2423888404739,6.14330686674367,-53.4427131291745));
#45250=CARTESIAN_POINT('Ctrl Pts',(-29.2484601891129,6.28494795741891,-53.9603595226558));
#45251=CARTESIAN_POINT('Ctrl Pts',(-29.2762156007057,6.53032030038241,-54.8545936563589));
#45252=CARTESIAN_POINT('Ctrl Pts',(-29.386306161652,7.01946605134849,-56.6135247633875));
#45253=CARTESIAN_POINT('Ctrl Pts',(-29.5327218189415,7.43982329257562,-58.0587381433518));
#45254=CARTESIAN_POINT('Ctrl Pts',(-29.6071951435415,7.75666376505009,-59.0529229961379));
#45255=CARTESIAN_POINT('Ctrl Pts',(-29.6158112741558,7.79760401764963,-59.1815399771206));
#45256=CARTESIAN_POINT('Ctrl Pts',(-29.6340659881628,7.87795458167348,-59.433655151946));
#45257=CARTESIAN_POINT('Ctrl Pts',(-29.6674699345856,8.01899017550212,-59.8754139377655));
#45258=CARTESIAN_POINT('Ctrl Pts',(-29.7397624843917,8.30013581198258,-60.7500981697734));
#45259=CARTESIAN_POINT('Ctrl Pts',(-29.8288267579884,8.62401116474369,-61.7328369750638));
#45260=CARTESIAN_POINT('Ctrl Pts',(-29.9122990683941,8.9582165401791,-62.6941998000547));
#45261=CARTESIAN_POINT('Ctrl Pts',(-29.9548376484439,9.15202992907867,-63.2266334707154));
#45262=CARTESIAN_POINT('Ctrl Pts',(-29.9804497778331,9.28441793274911,-63.5777856666572));
#45263=CARTESIAN_POINT('Ctrl Pts',(-29.9967341462232,9.37358979794334,-63.8108739102784));
#45264=CARTESIAN_POINT('Ctrl Pts',(-30.0117427869623,9.46418362784269,-64.0423652390109));
#45265=CARTESIAN_POINT('Ctrl Pts',(-30.0236146379465,9.54486559698578,-64.2435224642254));
#45266=CARTESIAN_POINT('Ctrl Pts',(-30.0300177327675,9.5913903607628,-64.3580586040495));
#45267=CARTESIAN_POINT('Ctrl Pts',(-30.0392317902084,9.6616067090032,-64.5294440809629));
#45268=CARTESIAN_POINT('Ctrl Pts',(-30.0460738261263,9.72103464484501,-64.6713910113177));
#45269=CARTESIAN_POINT('Ctrl Pts',(-30.056193231707,9.82070532959067,-64.9051026213648));
#45270=CARTESIAN_POINT('Ctrl Pts',(-30.0654035719528,9.92328050974094,-65.1394534429073));
#45271=CARTESIAN_POINT('Ctrl Pts',(-30.0792738868105,10.1403139254679,-65.6129717102997));
#45272=CARTESIAN_POINT('Ctrl Pts',(-30.0930380186134,10.5441203219372,-66.4419902424388));
#45273=CARTESIAN_POINT('Ctrl Pts',(-30.0897570522684,11.4372879264921,-68.1188888326908));
#45274=CARTESIAN_POINT('Ctrl Pts',(-30.0662549327026,12.2908443686912,-69.6081388008406));
#45275=CARTESIAN_POINT('Ctrl Pts',(-30.0677206779153,12.9093005226094,-70.781419220543));
#45276=CARTESIAN_POINT('Ctrl Pts',(-30.0680132094674,13.0394825228367,-71.0281447542001));
#45277=CARTESIAN_POINT('Ctrl Pts',(-30.068443337793,13.3048534320091,-71.5300820404047));
#45278=CARTESIAN_POINT('Ctrl Pts',(-30.0687264348823,13.6356514928772,-72.1540785489046));
#45279=CARTESIAN_POINT('Ctrl Pts',(-30.0687559042375,14.0348079013757,-72.9049827833199));
#45280=CARTESIAN_POINT('Ctrl Pts',(-30.0683798170397,14.8343904396941,-74.4062939876644));
#45281=CARTESIAN_POINT('Ctrl Pts',(-30.0675396968737,15.503662396096,-75.6594521589913));
#45282=CARTESIAN_POINT('Ctrl Pts',(-30.0675325757361,16.475143996278,-77.4865030812836));
#45283=CARTESIAN_POINT('Ctrl Pts',(-30.0675297169312,16.9110122292074,-78.3062315870108));
#45284=CARTESIAN_POINT('Ctrl Pts',(-30.0675297169313,17.3475338165968,-79.1272092891091));
#45285=CARTESIAN_POINT('Ctrl Pts',(-28.5063700143004,4.0751307694223,24.8306290855513));
#45286=CARTESIAN_POINT('Ctrl Pts',(-28.5064550410518,4.0751305156724,24.7817495992412));
#45287=CARTESIAN_POINT('Ctrl Pts',(-28.5065442166203,4.07513025010105,24.7328711645537));
#45288=CARTESIAN_POINT('Ctrl Pts',(-28.5075972303578,4.07512709922709,24.1822610181398));
#45289=CARTESIAN_POINT('Ctrl Pts',(-28.5084048846699,4.07512163837621,23.1781227303733));
#45290=CARTESIAN_POINT('Ctrl Pts',(-28.5102858747354,4.0751071477093,21.1695205266819));
#45291=CARTESIAN_POINT('Ctrl Pts',(-28.5172933353407,4.0750862730656,19.6653675836014));
#45292=CARTESIAN_POINT('Ctrl Pts',(-28.5321520913383,4.07505702437731,18.4143191318779));
#45293=CARTESIAN_POINT('Ctrl Pts',(-28.5392785618885,4.07504184758454,17.9114918157889));
#45294=CARTESIAN_POINT('Ctrl Pts',(-28.5571741550791,4.07500190159066,16.9074943019247));
#45295=CARTESIAN_POINT('Ctrl Pts',(-28.5955586169002,4.07491678343083,15.1536833936334));
#45296=CARTESIAN_POINT('Ctrl Pts',(-28.6320203529255,4.07485449752761,13.6519735110304));
#45297=CARTESIAN_POINT('Ctrl Pts',(-28.6548705454507,4.07484721171388,12.3975437498382));
#45298=CARTESIAN_POINT('Ctrl Pts',(-28.6642113546693,4.07484787230247,11.896607515957));
#45299=CARTESIAN_POINT('Ctrl Pts',(-28.6832524227466,4.07486075549552,10.8947894472725));
#45300=CARTESIAN_POINT('Ctrl Pts',(-28.706789245084,4.07489478299759,9.64227929161552));
#45301=CARTESIAN_POINT('Ctrl Pts',(-28.7316119959556,4.07494686114839,8.13778312608962));
#45302=CARTESIAN_POINT('Ctrl Pts',(-28.7438779121553,4.07497928221181,7.13306000887749));
#45303=CARTESIAN_POINT('Ctrl Pts',(-28.7495750949822,4.07499518723171,6.5050732982054));
#45304=CARTESIAN_POINT('Ctrl Pts',(-28.7517254796684,4.07501222499112,6.25499083013756));
#45305=CARTESIAN_POINT('Ctrl Pts',(-28.7555591252596,4.07508135353952,5.75402907367263));
#45306=CARTESIAN_POINT('Ctrl Pts',(-28.7610532102808,4.07527284770306,4.8758210208063));
#45307=CARTESIAN_POINT('Ctrl Pts',(-28.7672864360839,4.07577030561028,3.11544649156435));
#45308=CARTESIAN_POINT('Ctrl Pts',(-28.7648084158001,4.0758076728453,1.60790548044939));
#45309=CARTESIAN_POINT('Ctrl Pts',(-28.759685738567,4.07510385438478,0.547427834192141));
#45310=CARTESIAN_POINT('Ctrl Pts',(-28.7590167480848,4.07501238119254,0.421072873216588));
#45311=CARTESIAN_POINT('Ctrl Pts',(-28.7574541748833,4.07480022248746,0.168617210843751));
#45312=CARTESIAN_POINT('Ctrl Pts',(-28.7541625555416,4.0743573888518,-0.27264522366889));
#45313=CARTESIAN_POINT('Ctrl Pts',(-28.7480452405828,4.0735475875382,-0.901576117862987));
#45314=CARTESIAN_POINT('Ctrl Pts',(-28.7390252374076,4.07238446689408,-1.65445988487398));
#45315=CARTESIAN_POINT('Ctrl Pts',(-28.7255170393529,4.07069572979033,-2.65646957341181));
#45316=CARTESIAN_POINT('Ctrl Pts',(-28.7073114843065,4.0685533590852,-3.90670358762708));
#45317=CARTESIAN_POINT('Ctrl Pts',(-28.6943975210421,4.06728409919296,-4.90692352017473));
#45318=CARTESIAN_POINT('Ctrl Pts',(-28.6878098793571,4.06678114894455,-5.5329357353639));
#45319=CARTESIAN_POINT('Ctrl Pts',(-28.6851829138752,4.06657269379081,-5.7840063726452));
#45320=CARTESIAN_POINT('Ctrl Pts',(-28.6799716070688,4.06614085446737,-6.28609299293432));
#45321=CARTESIAN_POINT('Ctrl Pts',(-28.6709850712771,4.06537575387857,-7.16528470639284));
#45322=CARTESIAN_POINT('Ctrl Pts',(-28.6586549502862,4.06443450811702,-8.42127718018226));
#45323=CARTESIAN_POINT('Ctrl Pts',(-28.6473426314964,4.06416607144442,-9.6746534608699));
#45324=CARTESIAN_POINT('Ctrl Pts',(-28.6401376477395,4.06457818071917,-10.5491379927501));
#45325=CARTESIAN_POINT('Ctrl Pts',(-28.6362491756948,4.06502038333421,-11.0478169769201));
#45326=CARTESIAN_POINT('Ctrl Pts',(-28.6343852406347,4.06531621003876,-11.2967818689912));
#45327=CARTESIAN_POINT('Ctrl Pts',(-28.6330134062058,4.06556938824069,-11.4841215256739));
#45328=CARTESIAN_POINT('Ctrl Pts',(-28.6320889975595,4.06576455600266,-11.6095836028888));
#45329=CARTESIAN_POINT('Ctrl Pts',(-28.6302349510895,4.06625052056912,-11.860540528078));
#45330=CARTESIAN_POINT('Ctrl Pts',(-28.626986601601,4.06733209686087,-12.2991155322276));
#45331=CARTESIAN_POINT('Ctrl Pts',(-28.620553195512,4.0702680235487,-13.1748182689849));
#45332=CARTESIAN_POINT('Ctrl Pts',(-28.6120116468468,4.07581010149929,-14.4236955364312));
#45333=CARTESIAN_POINT('Ctrl Pts',(-28.6062014687261,4.08032597813081,-15.5505911344308));
#45334=CARTESIAN_POINT('Ctrl Pts',(-28.6035717107567,4.08226334584899,-16.3052735984145));
#45335=CARTESIAN_POINT('Ctrl Pts',(-28.6021821982076,4.08321002851602,-16.809445977369));
#45336=CARTESIAN_POINT('Ctrl Pts',(-28.6015792694236,4.08346631588465,-17.1889521925233));
#45337=CARTESIAN_POINT('Ctrl Pts',(-28.6013643203449,4.08335371643104,-17.5052794437319));
#45338=CARTESIAN_POINT('Ctrl Pts',(-28.6012901999452,4.08333057890033,-17.6291360036696));
#45339=CARTESIAN_POINT('Ctrl Pts',(-28.601189881543,4.08335630502948,-17.8779284626584));
#45340=CARTESIAN_POINT('Ctrl Pts',(-28.6011630597932,4.08347247635335,-18.1267423503286));
#45341=CARTESIAN_POINT('Ctrl Pts',(-28.6012200531399,4.08363962845014,-18.3760617391668));
#45342=CARTESIAN_POINT('Ctrl Pts',(-28.6012912010045,4.08375797076782,-18.5319920711977));
#45343=CARTESIAN_POINT('Ctrl Pts',(-28.601370882673,4.08385588435406,-18.6568361478655));
#45344=CARTESIAN_POINT('Ctrl Pts',(-28.6014420633411,4.08392986485814,-18.7505088520711));
#45345=CARTESIAN_POINT('Ctrl Pts',(-28.6015110779462,4.08399098076577,-18.8286071854719));
#45346=CARTESIAN_POINT('Ctrl Pts',(-28.6015723337452,4.08403888408376,-18.8911068965197));
#45347=CARTESIAN_POINT('Ctrl Pts',(-28.6021268874594,4.08443912596546,-19.4224795120135));
#45348=CARTESIAN_POINT('Ctrl Pts',(-28.6042230114293,4.08496632011906,-20.4423636620365));
#45349=CARTESIAN_POINT('Ctrl Pts',(-28.6114274699414,4.07995838922308,-21.9601597456664));
#45350=CARTESIAN_POINT('Ctrl Pts',(-28.619503512616,4.06945508613115,-22.9801762124166));
#45351=CARTESIAN_POINT('Ctrl Pts',(-28.6257698020092,4.05959453037469,-23.6185528436904));
#45352=CARTESIAN_POINT('Ctrl Pts',(-28.6285572713742,4.05511040085929,-23.8738673293465));
#45353=CARTESIAN_POINT('Ctrl Pts',(-28.6351809674563,4.04428158215644,-24.3821280903121));
#45354=CARTESIAN_POINT('Ctrl Pts',(-28.6491269721366,4.02108099402648,-25.2704435909963));
#45355=CARTESIAN_POINT('Ctrl Pts',(-28.6732965824566,3.97993891514751,-26.5323065338286));
#45356=CARTESIAN_POINT('Ctrl Pts',(-28.7018521611686,3.93045200794019,-28.032558331282));
#45357=CARTESIAN_POINT('Ctrl Pts',(-28.7155747876185,3.90598509535247,-29.0207512993479));
#45358=CARTESIAN_POINT('Ctrl Pts',(-28.7204154682032,3.89695414396225,-29.5726464466516));
#45359=CARTESIAN_POINT('Ctrl Pts',(-28.7214583076406,3.89493494175957,-29.6979807591885));
#45360=CARTESIAN_POINT('Ctrl Pts',(-28.7234270387298,3.89104592353962,-29.9471303392517));
#45361=CARTESIAN_POINT('Ctrl Pts',(-28.7265480220933,3.88457570068822,-30.3839372380476));
#45362=CARTESIAN_POINT('Ctrl Pts',(-28.7315487045443,3.87312760492994,-31.2568834820553));
#45363=CARTESIAN_POINT('Ctrl Pts',(-28.7351751217934,3.86160851200574,-32.5034492176154));
#45364=CARTESIAN_POINT('Ctrl Pts',(-28.7343820386309,3.85810067807707,-33.7465790637076));
#45365=CARTESIAN_POINT('Ctrl Pts',(-28.7312693881602,3.86096952008346,-34.7378806771447));
#45366=CARTESIAN_POINT('Ctrl Pts',(-28.7288549713757,3.86444576642746,-35.232363519754));
#45367=CARTESIAN_POINT('Ctrl Pts',(-28.7267473971563,3.86787391775565,-35.6036315420276));
#45368=CARTESIAN_POINT('Ctrl Pts',(-28.7253477432298,3.87043906327854,-35.8524203389833));
#45369=CARTESIAN_POINT('Ctrl Pts',(-28.7225122816699,3.87659960051719,-36.349454367607));
#45370=CARTESIAN_POINT('Ctrl Pts',(-28.7171595060761,3.88996398124818,-37.2187366227478));
#45371=CARTESIAN_POINT('Ctrl Pts',(-28.7029719475229,3.92628709148851,-38.9548294958871));
#45372=CARTESIAN_POINT('Ctrl Pts',(-28.6779204357281,3.97080216786415,-40.4478543681075));
#45373=CARTESIAN_POINT('Ctrl Pts',(-28.6423881509124,4.01235594105461,-41.6981476026289));
#45374=CARTESIAN_POINT('Ctrl Pts',(-28.6315352422751,4.02217894774256,-42.0944833673719));
#45375=CARTESIAN_POINT('Ctrl Pts',(-28.6162226999484,4.03096771433208,-42.6034857846265));
#45376=CARTESIAN_POINT('Ctrl Pts',(-28.6002399953221,4.03821538774407,-43.1110327947022));
#45377=CARTESIAN_POINT('Ctrl Pts',(-28.5787798709528,4.04592744712491,-43.7353041116043));
#45378=CARTESIAN_POINT('Ctrl Pts',(-28.5499946061509,4.05846176348219,-44.4707212417988));
#45379=CARTESIAN_POINT('Ctrl Pts',(-28.5229565217032,4.07575591946211,-45.0708121467108));
#45380=CARTESIAN_POINT('Ctrl Pts',(-28.499168294948,4.09601759532599,-45.5431560064207));
#45381=CARTESIAN_POINT('Ctrl Pts',(-28.4802145464749,4.11495795764875,-45.8935119207955));
#45382=CARTESIAN_POINT('Ctrl Pts',(-28.460093112664,4.13816692206255,-46.2399527998875));
#45383=CARTESIAN_POINT('Ctrl Pts',(-28.4316329521809,4.17547161434323,-46.6966010435509));
#45384=CARTESIAN_POINT('Ctrl Pts',(-28.4084746211153,4.21132347192227,-47.0332160567307));
#45385=CARTESIAN_POINT('Ctrl Pts',(-28.3839470210442,4.25348435717159,-47.3668895389636));
#45386=CARTESIAN_POINT('Ctrl Pts',(-28.3656221545791,4.28446593068285,-47.5965828274277));
#45387=CARTESIAN_POINT('Ctrl Pts',(-28.3233891553743,4.35294575955154,-48.0565547357988));
#45388=CARTESIAN_POINT('Ctrl Pts',(-28.2373456970307,4.49024962874069,-48.8723990065144));
#45389=CARTESIAN_POINT('Ctrl Pts',(-28.0963832536994,4.72878871184675,-50.0638539523906));
#45390=CARTESIAN_POINT('Ctrl Pts',(-27.945559766733,5.06821689546968,-51.5342689199645));
#45391=CARTESIAN_POINT('Ctrl Pts',(-27.8839986235443,5.32293710473205,-52.5363887393521));
#45392=CARTESIAN_POINT('Ctrl Pts',(-27.8657892882708,5.48881051509036,-53.1689845861308));
#45393=CARTESIAN_POINT('Ctrl Pts',(-27.8608639796447,5.55444069071902,-53.414115153262));
#45394=CARTESIAN_POINT('Ctrl Pts',(-27.8561704081986,5.69137441975848,-53.9096594814404));
#45395=CARTESIAN_POINT('Ctrl Pts',(-27.8618563300706,5.94089897593999,-54.7725158528541));
#45396=CARTESIAN_POINT('Ctrl Pts',(-27.9177646884999,6.47867009676407,-56.49260068047));
#45397=CARTESIAN_POINT('Ctrl Pts',(-28.0108984258091,6.98600845197756,-57.9460750333808));
#45398=CARTESIAN_POINT('Ctrl Pts',(-28.0643986211443,7.3589749222962,-58.9632438768764));
#45399=CARTESIAN_POINT('Ctrl Pts',(-28.0710994995596,7.40486849700483,-59.087683827155));
#45400=CARTESIAN_POINT('Ctrl Pts',(-28.0855759991836,7.49712864453928,-59.3358262755601));
#45401=CARTESIAN_POINT('Ctrl Pts',(-28.113424438541,7.66043095015801,-59.7697091382071));
#45402=CARTESIAN_POINT('Ctrl Pts',(-28.1777711656,7.99344520754302,-60.6345834620239));
#45403=CARTESIAN_POINT('Ctrl Pts',(-28.263998444937,8.38646109980859,-61.6159036784955));
#45404=CARTESIAN_POINT('Ctrl Pts',(-28.3476765614693,8.78976844974455,-62.5875275250034));
#45405=CARTESIAN_POINT('Ctrl Pts',(-28.3908407896533,9.02066613610083,-63.1297655617631));
#45406=CARTESIAN_POINT('Ctrl Pts',(-28.4168182778754,9.17636660806815,-63.4891354787894));
#45407=CARTESIAN_POINT('Ctrl Pts',(-28.4333132625767,9.28066163268648,-63.7281312770182));
#45408=CARTESIAN_POINT('Ctrl Pts',(-28.4484611031149,9.38568378540385,-63.9661714729316));
#45409=CARTESIAN_POINT('Ctrl Pts',(-28.460340289617,9.47827546540508,-64.1735973287607));
#45410=CARTESIAN_POINT('Ctrl Pts',(-28.4667085162954,9.53138580096016,-64.2918666428035));
#45411=CARTESIAN_POINT('Ctrl Pts',(-28.4758274218159,9.61125209852722,-64.4689996591551));
#45412=CARTESIAN_POINT('Ctrl Pts',(-28.4824955134669,9.67823324425495,-64.6160482596983));
#45413=CARTESIAN_POINT('Ctrl Pts',(-28.4921574987008,9.78965958501148,-64.8585661182835));
#45414=CARTESIAN_POINT('Ctrl Pts',(-28.5009939422513,9.90260723979942,-65.1003323094549));
#45415=CARTESIAN_POINT('Ctrl Pts',(-28.5144236103671,10.1370570244854,-65.5875989379661));
#45416=CARTESIAN_POINT('Ctrl Pts',(-28.5280998476002,10.5618541082785,-66.4359100148839));
#45417=CARTESIAN_POINT('Ctrl Pts',(-28.5261452105889,11.4659601810288,-68.1353068432759));
#45418=CARTESIAN_POINT('Ctrl Pts',(-28.5042603208831,12.2971910227302,-69.6204181568186));
#45419=CARTESIAN_POINT('Ctrl Pts',(-28.5059868748442,12.9092160196114,-70.7787578014154));
#45420=CARTESIAN_POINT('Ctrl Pts',(-28.5063176518591,13.0403881297786,-71.026833006938));
#45421=CARTESIAN_POINT('Ctrl Pts',(-28.506810343618,13.3061510584708,-71.5287248539541));
#45422=CARTESIAN_POINT('Ctrl Pts',(-28.5071342080593,13.6377122596,-72.1536545062716));
#45423=CARTESIAN_POINT('Ctrl Pts',(-28.5071681221449,14.0370893088904,-72.9049205376012));
#45424=CARTESIAN_POINT('Ctrl Pts',(-28.5067378086829,14.8367082476652,-74.4069878530215));
#45425=CARTESIAN_POINT('Ctrl Pts',(-28.505786105334,15.5050694448925,-75.6599826656687));
#45426=CARTESIAN_POINT('Ctrl Pts',(-28.5057865286928,16.4760794038801,-77.486169472289));
#45427=CARTESIAN_POINT('Ctrl Pts',(-28.5057850703907,16.9121202092292,-78.306234167581));
#45428=CARTESIAN_POINT('Ctrl Pts',(-28.5057850703907,17.3486417966187,-79.1272118696792));
#45429=CARTESIAN_POINT('Ctrl Pts',(-27.2546101003228,4.0774086805339,24.8306314676615));
#45430=CARTESIAN_POINT('Ctrl Pts',(-27.2546915815672,4.07740844455158,24.781752056975));
#45431=CARTESIAN_POINT('Ctrl Pts',(-27.2547770374123,4.07740819882894,24.7328736991936));
#45432=CARTESIAN_POINT('Ctrl Pts',(-27.2557861793606,4.07740522247428,24.1822644399479));
#45433=CARTESIAN_POINT('Ctrl Pts',(-27.256561323909,4.07740099708737,23.17812767054));
#45434=CARTESIAN_POINT('Ctrl Pts',(-27.2583664216711,4.07739113571785,21.1695268379285));
#45435=CARTESIAN_POINT('Ctrl Pts',(-27.2650824454299,4.07737074475774,19.665373131343));
#45436=CARTESIAN_POINT('Ctrl Pts',(-27.2793176058701,4.07733690464952,18.4143239105435));
#45437=CARTESIAN_POINT('Ctrl Pts',(-27.2861452978621,4.07732008576429,17.911500928659));
#45438=CARTESIAN_POINT('Ctrl Pts',(-27.3032914192145,4.07727658330968,16.9075066894004));
#45439=CARTESIAN_POINT('Ctrl Pts',(-27.3400678380425,4.07718367084803,15.1536967473203));
#45440=CARTESIAN_POINT('Ctrl Pts',(-27.3749973994861,4.07710478697132,13.6519734005915));
#45441=CARTESIAN_POINT('Ctrl Pts',(-27.3968760234158,4.07707457179911,12.3975242999686));
#45442=CARTESIAN_POINT('Ctrl Pts',(-27.4058182811068,4.07706441082617,11.8965802318231));
#45443=CARTESIAN_POINT('Ctrl Pts',(-27.424042248115,4.07705098316843,10.894750841519));
#45444=CARTESIAN_POINT('Ctrl Pts',(-27.446564569103,4.07704337196664,9.64223235776427));
#45445=CARTESIAN_POINT('Ctrl Pts',(-27.470310851357,4.07704633646212,8.1377372100784));
#45446=CARTESIAN_POINT('Ctrl Pts',(-27.4820456322472,4.07704917215681,7.13302130766815));
#45447=CARTESIAN_POINT('Ctrl Pts',(-27.4874955577965,4.07705183733921,6.50504059377069));
#45448=CARTESIAN_POINT('Ctrl Pts',(-27.4895482840546,4.07706236045641,6.25493841669784));
#45449=CARTESIAN_POINT('Ctrl Pts',(-27.4931929702868,4.07711424196008,5.75395658505462));
#45450=CARTESIAN_POINT('Ctrl Pts',(-27.4983826152909,4.07726499461672,4.87572219825504));
#45451=CARTESIAN_POINT('Ctrl Pts',(-27.504164316388,4.0776733222571,3.11536628642292));
#45452=CARTESIAN_POINT('Ctrl Pts',(-27.5017982447368,4.07767661882587,1.6079464273222));
#45453=CARTESIAN_POINT('Ctrl Pts',(-27.4971755625774,4.07706353984626,0.547608728350889));
#45454=CARTESIAN_POINT('Ctrl Pts',(-27.4965710434973,4.07698495250432,0.421276638990806));
#45455=CARTESIAN_POINT('Ctrl Pts',(-27.4951593133511,4.07680194783564,0.168859992086856));
#45456=CARTESIAN_POINT('Ctrl Pts',(-27.4921842812917,4.07642036620931,-0.27233989131527));
#45457=CARTESIAN_POINT('Ctrl Pts',(-27.4866554523826,4.0757177072624,-0.901204689572938));
#45458=CARTESIAN_POINT('Ctrl Pts',(-27.4784840998671,4.07471961851841,-1.65404408891485));
#45459=CARTESIAN_POINT('Ctrl Pts',(-27.4662302513185,4.07326488974287,-2.65603895285884));
#45460=CARTESIAN_POINT('Ctrl Pts',(-27.4496442700658,4.0714363481666,-3.90633192945388));
#45461=CARTESIAN_POINT('Ctrl Pts',(-27.4377683739882,4.07035056189753,-4.90666001983112));
#45462=CARTESIAN_POINT('Ctrl Pts',(-27.4316383677891,4.06993201648509,-5.53275069722329));
#45463=CARTESIAN_POINT('Ctrl Pts',(-27.4291952297676,4.06976708145305,-5.78370899132702));
#45464=CARTESIAN_POINT('Ctrl Pts',(-27.4243521139342,4.06944661825676,-6.28569409154177));
#45465=CARTESIAN_POINT('Ctrl Pts',(-27.4160008254043,4.06892327742794,-7.16475965770132));
#45466=CARTESIAN_POINT('Ctrl Pts',(-27.4044868074976,4.06835875013137,-8.42087325927019));
#45467=CARTESIAN_POINT('Ctrl Pts',(-27.3936832198069,4.06824645545923,-9.67472110418459));
#45468=CARTESIAN_POINT('Ctrl Pts',(-27.3865749697245,4.06851597506718,-10.5497357044532));
#45469=CARTESIAN_POINT('Ctrl Pts',(-27.3826548941153,4.06878389138936,-11.0487735960245));
#45470=CARTESIAN_POINT('Ctrl Pts',(-27.3807442126837,4.06895811317885,-11.2979355567401));
#45471=CARTESIAN_POINT('Ctrl Pts',(-27.3793244097686,4.06910569315751,-11.4854355948755));
#45472=CARTESIAN_POINT('Ctrl Pts',(-27.3783585030531,4.06921942120932,-11.6111678989742));
#45473=CARTESIAN_POINT('Ctrl Pts',(-27.3763872065056,4.06950129246306,-11.8625350299554));
#45474=CARTESIAN_POINT('Ctrl Pts',(-27.3728503594407,4.07012625568385,-12.3017858467383));
#45475=CARTESIAN_POINT('Ctrl Pts',(-27.3655598205339,4.07181273452347,-13.1784443345948));
#45476=CARTESIAN_POINT('Ctrl Pts',(-27.3552722600769,4.07499453777574,-14.427651994048));
#45477=CARTESIAN_POINT('Ctrl Pts',(-27.3479622490176,4.07760858671024,-15.5535739483884));
#45478=CARTESIAN_POINT('Ctrl Pts',(-27.3446497885251,4.07876798806127,-16.307088587635));
#45479=CARTESIAN_POINT('Ctrl Pts',(-27.342907585337,4.07935477734326,-16.8103475162039));
#45480=CARTESIAN_POINT('Ctrl Pts',(-27.3421791743516,4.07954249347778,-17.1890064902595));
#45481=CARTESIAN_POINT('Ctrl Pts',(-27.3419588704251,4.07952326588427,-17.5045746536951));
#45482=CARTESIAN_POINT('Ctrl Pts',(-27.3418752611563,4.07953007569022,-17.6287095806376));
#45483=CARTESIAN_POINT('Ctrl Pts',(-27.3417287621694,4.07959279821592,-17.8776598485618));
#45484=CARTESIAN_POINT('Ctrl Pts',(-27.3416217867385,4.07971620085526,-18.1266789982541));
#45485=CARTESIAN_POINT('Ctrl Pts',(-27.3415769078325,4.0798783484122,-18.3760568720131));
#45486=CARTESIAN_POINT('Ctrl Pts',(-27.3415780390966,4.07999031882576,-18.5320055063777));
#45487=CARTESIAN_POINT('Ctrl Pts',(-27.3415994740873,4.08008358626996,-18.6568386635698));
#45488=CARTESIAN_POINT('Ctrl Pts',(-27.3416262524713,4.08015453248145,-18.7504946446562));
#45489=CARTESIAN_POINT('Ctrl Pts',(-27.3416579949172,4.08021387882802,-18.8285700716364));
#45490=CARTESIAN_POINT('Ctrl Pts',(-27.3416894772009,4.0802611446212,-18.8910467255343));
#45491=CARTESIAN_POINT('Ctrl Pts',(-27.341991802707,4.08066067875279,-19.4221941757928));
#45492=CARTESIAN_POINT('Ctrl Pts',(-27.3436410578754,4.08129684321048,-20.440725937771));
#45493=CARTESIAN_POINT('Ctrl Pts',(-27.351961923784,4.07891025829886,-21.953997325392));
#45494=CARTESIAN_POINT('Ctrl Pts',(-27.3630621133216,4.07297610046509,-22.9693110673969));
#45495=CARTESIAN_POINT('Ctrl Pts',(-27.3722796464463,4.06725958282786,-23.6042261310723));
#45496=CARTESIAN_POINT('Ctrl Pts',(-27.3763643044384,4.0646734681043,-23.8569164199335));
#45497=CARTESIAN_POINT('Ctrl Pts',(-27.3860541716508,4.05838892454659,-24.3613801869045));
#45498=CARTESIAN_POINT('Ctrl Pts',(-27.4064446332014,4.04484082022933,-25.2443384429749));
#45499=CARTESIAN_POINT('Ctrl Pts',(-27.4420556226772,4.02029323011283,-26.5035495796231));
#45500=CARTESIAN_POINT('Ctrl Pts',(-27.4848968440096,3.98986151530367,-28.0078199110668));
#45501=CARTESIAN_POINT('Ctrl Pts',(-27.5067731539225,3.97402841603677,-29.0035660851326));
#45502=CARTESIAN_POINT('Ctrl Pts',(-27.5154451374984,3.96791231174987,-29.560992238552));
#45503=CARTESIAN_POINT('Ctrl Pts',(-27.5173370691358,3.96655872264482,-29.6863747424985));
#45504=CARTESIAN_POINT('Ctrl Pts',(-27.5209678542977,3.9639284711308,-29.9363122547117));
#45505=CARTESIAN_POINT('Ctrl Pts',(-27.5269263449902,3.95950868834027,-30.3742227049902));
#45506=CARTESIAN_POINT('Ctrl Pts',(-27.5373167256218,3.95148861588675,-31.2498686218677));
#45507=CARTESIAN_POINT('Ctrl Pts',(-27.5480809685386,3.94270291613348,-32.5008060849347));
#45508=CARTESIAN_POINT('Ctrl Pts',(-27.5541815642533,3.93838291801496,-33.7492714989798));
#45509=CARTESIAN_POINT('Ctrl Pts',(-27.556738020654,3.93812425981094,-34.7453564932264));
#45510=CARTESIAN_POINT('Ctrl Pts',(-27.5573055494602,3.9391294137175,-35.2424175058302));
#45511=CARTESIAN_POINT('Ctrl Pts',(-27.557494604669,3.94034033135259,-35.6156931631465));
#45512=CARTESIAN_POINT('Ctrl Pts',(-27.5576458724682,3.94128873126373,-35.8658549594538));
#45513=CARTESIAN_POINT('Ctrl Pts',(-27.5579450503163,3.94371014608695,-36.3654927635573));
#45514=CARTESIAN_POINT('Ctrl Pts',(-27.5582209322075,3.94934036350232,-37.2390728137141));
#45515=CARTESIAN_POINT('Ctrl Pts',(-27.5556802719258,3.96573535501417,-38.9826258473562));
#45516=CARTESIAN_POINT('Ctrl Pts',(-27.5413304064018,3.98804089509753,-40.4803287991562));
#45517=CARTESIAN_POINT('Ctrl Pts',(-27.5148059809254,4.01012355087822,-41.7335732325126));
#45518=CARTESIAN_POINT('Ctrl Pts',(-27.506614799977,4.01382313814948,-42.1294899173214));
#45519=CARTESIAN_POINT('Ctrl Pts',(-27.4948038728113,4.01475197238754,-42.6392652194878));
#45520=CARTESIAN_POINT('Ctrl Pts',(-27.4823100500975,4.01410807310616,-43.1478052204435));
#45521=CARTESIAN_POINT('Ctrl Pts',(-27.4652056523953,4.01188834921534,-43.7741459445469));
#45522=CARTESIAN_POINT('Ctrl Pts',(-27.4416686637682,4.01205030286353,-44.5131850793774));
#45523=CARTESIAN_POINT('Ctrl Pts',(-27.4190118436299,4.01846618553771,-45.1172726644237));
#45524=CARTESIAN_POINT('Ctrl Pts',(-27.3987206949338,4.02951859982369,-45.5932733110073));
#45525=CARTESIAN_POINT('Ctrl Pts',(-27.3823587370145,4.04130353601179,-45.946621494624));
#45526=CARTESIAN_POINT('Ctrl Pts',(-27.3647800503514,4.05707927954136,-46.2962615516113));
#45527=CARTESIAN_POINT('Ctrl Pts',(-27.3396207882002,4.08405630656236,-46.757424891615));
#45528=CARTESIAN_POINT('Ctrl Pts',(-27.3187605625721,4.11169988508255,-47.0976336407574));
#45529=CARTESIAN_POINT('Ctrl Pts',(-27.2963805619571,4.14521705812,-47.4351463426626));
#45530=CARTESIAN_POINT('Ctrl Pts',(-27.2797829769067,4.17028343828459,-47.6747586518392));
#45531=CARTESIAN_POINT('Ctrl Pts',(-27.2414790687407,4.22420761329892,-48.1470192771235));
#45532=CARTESIAN_POINT('Ctrl Pts',(-27.1631572478958,4.33065416927353,-48.978912160315));
#45533=CARTESIAN_POINT('Ctrl Pts',(-27.0323943570625,4.51336562870429,-50.1699149604666));
#45534=CARTESIAN_POINT('Ctrl Pts',(-26.8879168085563,4.78197800293409,-51.6087945648171));
#45535=CARTESIAN_POINT('Ctrl Pts',(-26.8258901135032,4.99983547607388,-52.5715476767348));
#45536=CARTESIAN_POINT('Ctrl Pts',(-26.8050492994794,5.1504403653152,-53.1743205901841));
#45537=CARTESIAN_POINT('Ctrl Pts',(-26.7981595044316,5.21154340576477,-53.4118332759869));
#45538=CARTESIAN_POINT('Ctrl Pts',(-26.788298589805,5.34149963276008,-53.8916837498143));
#45539=CARTESIAN_POINT('Ctrl Pts',(-26.7811782829475,5.58568815680499,-54.7327463636641));
#45540=CARTESIAN_POINT('Ctrl Pts',(-26.8002012452745,6.13595090561274,-56.4249561946581));
#45541=CARTESIAN_POINT('Ctrl Pts',(-26.852938438552,6.68507130930734,-57.8797527558067));
#45542=CARTESIAN_POINT('Ctrl Pts',(-26.8887442028565,7.08853302756357,-58.906082215184));
#45543=CARTESIAN_POINT('Ctrl Pts',(-26.8936556302131,7.13656932665945,-59.0270937517182));
#45544=CARTESIAN_POINT('Ctrl Pts',(-26.9043644557737,7.23481899580833,-59.2714068910028));
#45545=CARTESIAN_POINT('Ctrl Pts',(-26.9257340549756,7.40989753960044,-59.698336006939));
#45546=CARTESIAN_POINT('Ctrl Pts',(-26.977105952746,7.77323377402914,-60.5544351623106));
#45547=CARTESIAN_POINT('Ctrl Pts',(-27.0487369914947,8.21176114729655,-61.5339877132366));
#45548=CARTESIAN_POINT('Ctrl Pts',(-27.1191502767737,8.66420917288523,-62.5122919003745));
#45549=CARTESIAN_POINT('Ctrl Pts',(-27.1556698679012,8.92247578068374,-63.0612434193802));
#45550=CARTESIAN_POINT('Ctrl Pts',(-27.1776461428923,9.09566073391902,-63.4263573086767));
#45551=CARTESIAN_POINT('Ctrl Pts',(-27.1915965005875,9.21136121266743,-63.6695170955314));
#45552=CARTESIAN_POINT('Ctrl Pts',(-27.2043815764802,9.32733994357597,-63.9122250866032));
#45553=CARTESIAN_POINT('Ctrl Pts',(-27.2143717790303,9.42901319226746,-64.1241851694408));
#45554=CARTESIAN_POINT('Ctrl Pts',(-27.2197112470884,9.48715099835241,-64.2451752724045));
#45555=CARTESIAN_POINT('Ctrl Pts',(-27.227338582932,9.57438723927106,-64.4265181282341));
#45556=CARTESIAN_POINT('Ctrl Pts',(-27.2328678760352,9.64713745024055,-64.5773521359468));
#45557=CARTESIAN_POINT('Ctrl Pts',(-27.2407911835927,9.76750941850949,-64.8264712414182));
#45558=CARTESIAN_POINT('Ctrl Pts',(-27.2480703587409,9.88789116991536,-65.0729942285441));
#45559=CARTESIAN_POINT('Ctrl Pts',(-27.2592171476814,10.13507491431,-65.5696917896668));
#45560=CARTESIAN_POINT('Ctrl Pts',(-27.2707948775918,10.5751087883559,-66.4312179139581));
#45561=CARTESIAN_POINT('Ctrl Pts',(-27.2700304119169,11.4873858665043,-68.1468579632658));
#45562=CARTESIAN_POINT('Ctrl Pts',(-27.2525109126437,12.3030078621601,-69.6289538873663));
#45563=CARTESIAN_POINT('Ctrl Pts',(-27.2541201495845,12.9106217789162,-70.7767840803218));
#45564=CARTESIAN_POINT('Ctrl Pts',(-27.2544305738434,13.0425342299894,-71.0258395726878));
#45565=CARTESIAN_POINT('Ctrl Pts',(-27.2548923449946,13.3086323235748,-71.5277397348066));
#45566=CARTESIAN_POINT('Ctrl Pts',(-27.2551935210388,13.6407795601621,-72.1533706167213));
#45567=CARTESIAN_POINT('Ctrl Pts',(-27.2552241432152,14.0403353165931,-72.9049310243895));
#45568=CARTESIAN_POINT('Ctrl Pts',(-27.2548176665827,14.839974311778,-74.4075839612337));
#45569=CARTESIAN_POINT('Ctrl Pts',(-27.2539131733232,15.5075997838829,-75.6604288636657));
#45570=CARTESIAN_POINT('Ctrl Pts',(-27.2539071141013,16.4782256544517,-77.4859121791665));
#45571=CARTESIAN_POINT('Ctrl Pts',(-27.2539024723065,16.9143985081388,-78.3062348671697));
#45572=CARTESIAN_POINT('Ctrl Pts',(-27.2539024723065,17.3509200955282,-79.1272125692679));
#45573=CARTESIAN_POINT('Ctrl Pts',(-26.0013011106398,4.07985819352921,24.8306343146944));
#45574=CARTESIAN_POINT('Ctrl Pts',(-26.0013789529674,4.07985804951133,24.7817549932913));
#45575=CARTESIAN_POINT('Ctrl Pts',(-26.0014605947771,4.07985789809793,24.7328767261139));
#45576=CARTESIAN_POINT('Ctrl Pts',(-26.0024245885624,4.07985612747913,24.1822685228224));
#45577=CARTESIAN_POINT('Ctrl Pts',(-26.0031642737342,4.07985491125827,23.1781333336685));
#45578=CARTESIAN_POINT('Ctrl Pts',(-26.0048881842587,4.07985181195996,21.1695342768379));
#45579=CARTESIAN_POINT('Ctrl Pts',(-26.0113025736306,4.07984033585152,19.6653805292443));
#45580=CARTESIAN_POINT('Ctrl Pts',(-26.0249020614195,4.07981521286216,18.4143310323347));
#45581=CARTESIAN_POINT('Ctrl Pts',(-26.0314251371612,4.07980293276608,17.9115134907684));
#45582=CARTESIAN_POINT('Ctrl Pts',(-26.0478061265009,4.07977192289328,16.9075232341124));
#45583=CARTESIAN_POINT('Ctrl Pts',(-26.082942053095,4.07970491200509,15.153713540109));
#45584=CARTESIAN_POINT('Ctrl Pts',(-26.1163096414983,4.07964468448795,13.6519733108666));
#45585=CARTESIAN_POINT('Ctrl Pts',(-26.1372103910028,4.07960974585599,12.3975008589439));
#45586=CARTESIAN_POINT('Ctrl Pts',(-26.1457529910553,4.07959572525298,11.8965472956601));
#45587=CARTESIAN_POINT('Ctrl Pts',(-26.1631632522454,4.07956765728665,10.8947040346659));
#45588=CARTESIAN_POINT('Ctrl Pts',(-26.1846759019604,4.0795364209103,9.64217637151487));
#45589=CARTESIAN_POINT('Ctrl Pts',(-26.2073607059512,4.07950398038011,8.13768241570142));
#45590=CARTESIAN_POINT('Ctrl Pts',(-26.2185663909266,4.07949098160033,7.13297738461757));
#45591=CARTESIAN_POINT('Ctrl Pts',(-26.2237726343733,4.07948462062371,6.50500244631245));
#45592=CARTESIAN_POINT('Ctrl Pts',(-26.225727981951,4.07948619840636,6.25483282875101));
#45593=CARTESIAN_POINT('Ctrl Pts',(-26.2291798508411,4.07950316165294,5.7537796075322));
#45594=CARTESIAN_POINT('Ctrl Pts',(-26.2340434904564,4.07956239453138,4.87545560005647));
#45595=CARTESIAN_POINT('Ctrl Pts',(-26.2393234114807,4.0797290922924,3.11516020236738));
#45596=CARTESIAN_POINT('Ctrl Pts',(-26.237030454936,4.07974833926762,1.60817566708211));
#45597=CARTESIAN_POINT('Ctrl Pts',(-26.2330023014032,4.07948610402459,0.548332138737982));
#45598=CARTESIAN_POINT('Ctrl Pts',(-26.2324770878948,4.07945134405716,0.422083829682385));
#45599=CARTESIAN_POINT('Ctrl Pts',(-26.2312481821157,4.07937089598177,0.169809390305926));
#45600=CARTESIAN_POINT('Ctrl Pts',(-26.2286559185981,4.07920222706464,-0.27115977582926));
#45601=CARTESIAN_POINT('Ctrl Pts',(-26.2238184296938,4.07889540886044,-0.899774172662865));
#45602=CARTESIAN_POINT('Ctrl Pts',(-26.2166636663486,4.07844774619556,-1.65243157223408));
#45603=CARTESIAN_POINT('Ctrl Pts',(-26.2058812029711,4.07780173875976,-2.65434197500388));
#45604=CARTESIAN_POINT('Ctrl Pts',(-26.1912186942687,4.07697792765496,-3.90481027092992));
#45605=CARTESIAN_POINT('Ctrl Pts',(-26.1805376495462,4.0765172745372,-4.90557994986776));
#45606=CARTESIAN_POINT('Ctrl Pts',(-26.1749400951133,4.07635014998955,-5.53202086932197));
#45607=CARTESIAN_POINT('Ctrl Pts',(-26.1727011491545,4.07628811967238,-5.78288697526722));
#45608=CARTESIAN_POINT('Ctrl Pts',(-26.1682289140555,4.07618740313827,-6.28485799474117));
#45609=CARTESIAN_POINT('Ctrl Pts',(-26.1604325178287,4.07606775162831,-7.16391906466739));
#45610=CARTESIAN_POINT('Ctrl Pts',(-26.1494816680626,4.07603758491267,-8.42033007674828));
#45611=CARTESIAN_POINT('Ctrl Pts',(-26.1390583937814,4.07613309366833,-9.67479848719443));
#45612=CARTESIAN_POINT('Ctrl Pts',(-26.1321868318539,4.07623167871274,-10.5504384656346));
#45613=CARTESIAN_POINT('Ctrl Pts',(-26.1284001112086,4.07629308869807,-11.0498864309384));
#45614=CARTESIAN_POINT('Ctrl Pts',(-26.1265564850085,4.07632463227181,-11.2992701474647));
#45615=CARTESIAN_POINT('Ctrl Pts',(-26.1251882913001,4.07634839740299,-11.4869495146409));
#45616=CARTESIAN_POINT('Ctrl Pts',(-26.1242555799087,4.07636641590398,-11.6129935292225));
#45617=CARTESIAN_POINT('Ctrl Pts',(-26.1223445077193,4.07640971360248,-11.8648337223802));
#45618=CARTESIAN_POINT('Ctrl Pts',(-26.1188970858275,4.07650331865429,-12.3048696473225));
#45619=CARTESIAN_POINT('Ctrl Pts',(-26.1117260730017,4.07674902706291,-13.1826603926455));
#45620=CARTESIAN_POINT('Ctrl Pts',(-26.101497548318,4.07719956532485,-14.4323339566743));
#45621=CARTESIAN_POINT('Ctrl Pts',(-26.094209581299,4.07757043836075,-15.5572475817683));
#45622=CARTESIAN_POINT('Ctrl Pts',(-26.0909394569588,4.07774555434298,-16.3095070995799));
#45623=CARTESIAN_POINT('Ctrl Pts',(-26.0892367197142,4.077839471914,-16.8117785888063));
#45624=CARTESIAN_POINT('Ctrl Pts',(-26.0885535312242,4.07788117066302,-17.1895156247893));
#45625=CARTESIAN_POINT('Ctrl Pts',(-26.0883821177462,4.07789384316656,-17.5042618733334));
#45626=CARTESIAN_POINT('Ctrl Pts',(-26.0883230229287,4.07790111607961,-17.628808694147));
#45627=CARTESIAN_POINT('Ctrl Pts',(-26.0882450051653,4.07792362052946,-17.8780681622715));
#45628=CARTESIAN_POINT('Ctrl Pts',(-26.0882341952123,4.07795736618271,-18.1274489041177));
#45629=CARTESIAN_POINT('Ctrl Pts',(-26.088304936263,4.0779971328375,-18.3769928741742));
#45630=CARTESIAN_POINT('Ctrl Pts',(-26.0883860806377,4.07802434284426,-18.5330186180899));
#45631=CARTESIAN_POINT('Ctrl Pts',(-26.0884749174287,4.07804674968717,-18.6578788062151));
#45632=CARTESIAN_POINT('Ctrl Pts',(-26.0885539625203,4.07806388881347,-18.7515431416536));
#45633=CARTESIAN_POINT('Ctrl Pts',(-26.0886305534487,4.07807837511368,-18.8296132271757));
#45634=CARTESIAN_POINT('Ctrl Pts',(-26.0886984753022,4.07808994493893,-18.8920790549508));
#45635=CARTESIAN_POINT('Ctrl Pts',(-26.0893139685706,4.07818866471405,-19.4230945168937));
#45636=CARTESIAN_POINT('Ctrl Pts',(-26.0917330611588,4.07841063103444,-20.4400949792451));
#45637=CARTESIAN_POINT('Ctrl Pts',(-26.1006601571851,4.07826175095829,-21.9476412695908));
#45638=CARTESIAN_POINT('Ctrl Pts',(-26.1114730684071,4.07759859850918,-22.9568095349218));
#45639=CARTESIAN_POINT('Ctrl Pts',(-26.1200732731373,4.07685326303561,-23.5871603310035));
#45640=CARTESIAN_POINT('Ctrl Pts',(-26.1238447233394,4.07651791001592,-23.8368150555011));
#45641=CARTESIAN_POINT('Ctrl Pts',(-26.1326887293755,4.07567329563507,-24.336735111528));
#45642=CARTESIAN_POINT('Ctrl Pts',(-26.1510952602828,4.07375702558255,-25.2132310967213));
#45643=CARTESIAN_POINT('Ctrl Pts',(-26.1830001890633,4.06986262685334,-26.468802499517));
#45644=CARTESIAN_POINT('Ctrl Pts',(-26.2215211544865,4.06399270040154,-27.9769098624109));
#45645=CARTESIAN_POINT('Ctrl Pts',(-26.2418385192627,4.06041574406107,-28.9807911429983));
#45646=CARTESIAN_POINT('Ctrl Pts',(-26.2502429726783,4.05888649081813,-29.5442314297393));
#45647=CARTESIAN_POINT('Ctrl Pts',(-26.2520732505535,4.05855306998243,-29.6696430577692));
#45648=CARTESIAN_POINT('Ctrl Pts',(-26.2555970918632,4.05789153584461,-29.9203997673132));
#45649=CARTESIAN_POINT('Ctrl Pts',(-26.261410577545,4.05676154246959,-30.3594301535443));
#45650=CARTESIAN_POINT('Ctrl Pts',(-26.2717052240543,4.05461490675908,-31.2378241849018));
#45651=CARTESIAN_POINT('Ctrl Pts',(-26.2830148460803,4.05196591433397,-32.4931655030781));
#45652=CARTESIAN_POINT('Ctrl Pts',(-26.2909663449978,4.0501119239892,-33.7469906547072));
#45653=CARTESIAN_POINT('Ctrl Pts',(-26.2960159444366,4.04922281675521,-34.7478634587198));
#45654=CARTESIAN_POINT('Ctrl Pts',(-26.2982099355632,4.04899711046201,-35.2475023730581));
#45655=CARTESIAN_POINT('Ctrl Pts',(-26.2997826761264,4.0489154594892,-35.6227846526373));
#45656=CARTESIAN_POINT('Ctrl Pts',(-26.3009025087611,4.04886072072356,-35.8743950226809));
#45657=CARTESIAN_POINT('Ctrl Pts',(-26.3033140765469,4.0487766255127,-36.3767187361697));
#45658=CARTESIAN_POINT('Ctrl Pts',(-26.3077126946144,4.048701942534,-37.2547021301723));
#45659=CARTESIAN_POINT('Ctrl Pts',(-26.3151948391617,4.04931673891994,-39.0056140064209));
#45660=CARTESIAN_POINT('Ctrl Pts',(-26.3121081978818,4.05196032314691,-40.507437776701));
#45661=CARTESIAN_POINT('Ctrl Pts',(-26.2962978934717,4.05673709347293,-41.7629658680623));
#45662=CARTESIAN_POINT('Ctrl Pts',(-26.2912875139118,4.05507580219809,-42.1583486673137));
#45663=CARTESIAN_POINT('Ctrl Pts',(-26.283791863667,4.0491342464197,-42.6687098541352));
#45664=CARTESIAN_POINT('Ctrl Pts',(-26.2756834339648,4.04155010070283,-43.1780724170856));
#45665=CARTESIAN_POINT('Ctrl Pts',(-26.2642595673674,4.03052052051979,-43.8062806290324));
#45666=CARTESIAN_POINT('Ctrl Pts',(-26.2480330835504,4.0194952467161,-44.5487497045344));
#45667=CARTESIAN_POINT('Ctrl Pts',(-26.2320172183841,4.0158442331942,-45.1567415924084));
#45668=CARTESIAN_POINT('Ctrl Pts',(-26.2174638323169,4.01834227502156,-45.6363901948794));
#45669=CARTESIAN_POINT('Ctrl Pts',(-26.2056203435843,4.02341069113659,-45.9927657037704));
#45670=CARTESIAN_POINT('Ctrl Pts',(-26.1927889704637,4.03215314673909,-46.3456933378785));
#45671=CARTESIAN_POINT('Ctrl Pts',(-26.1742863860446,4.04932860164585,-46.8115670714307));
#45672=CARTESIAN_POINT('Ctrl Pts',(-26.1587617170671,4.06906009399286,-47.1556407818341));
#45673=CARTESIAN_POINT('Ctrl Pts',(-26.1419956568944,4.09431737965409,-47.4973171236936));
#45674=CARTESIAN_POINT('Ctrl Pts',(-26.1296745959103,4.11338925269087,-47.7457981442306));
#45675=CARTESIAN_POINT('Ctrl Pts',(-26.1013205493372,4.15316604518592,-48.2295842951589));
#45676=CARTESIAN_POINT('Ctrl Pts',(-26.043416140312,4.23037271286573,-49.0771569518487));
#45677=CARTESIAN_POINT('Ctrl Pts',(-25.9455247181537,4.36377552848887,-50.2707023199233));
#45678=CARTESIAN_POINT('Ctrl Pts',(-25.8328678181711,4.574975096906,-51.6834281820652));
#45679=CARTESIAN_POINT('Ctrl Pts',(-25.7807568251049,4.76266701885439,-52.6109487298273));
#45680=CARTESIAN_POINT('Ctrl Pts',(-25.761061240267,4.89944564339107,-53.1875046786558));
#45681=CARTESIAN_POINT('Ctrl Pts',(-25.7537316641207,4.95647452053676,-53.4190926834034));
#45682=CARTESIAN_POINT('Ctrl Pts',(-25.7413216255973,5.07937523522014,-53.8860406962918));
#45683=CARTESIAN_POINT('Ctrl Pts',(-25.7251768408865,5.31590876729731,-54.7092722248442));
#45684=CARTESIAN_POINT('Ctrl Pts',(-25.7125117551334,5.86695869123698,-56.377799583334));
#45685=CARTESIAN_POINT('Ctrl Pts',(-25.7272665769259,6.4412901900278,-57.8308948707272));
#45686=CARTESIAN_POINT('Ctrl Pts',(-25.7450834120612,6.86571500273623,-58.861081018843));
#45687=CARTESIAN_POINT('Ctrl Pts',(-25.7479653604283,6.91488381928122,-58.9789732806086));
#45688=CARTESIAN_POINT('Ctrl Pts',(-25.7543567837446,7.0169659084858,-59.2195463362856));
#45689=CARTESIAN_POINT('Ctrl Pts',(-25.7678613171999,7.20000915828807,-59.6399468852958));
#45690=CARTESIAN_POINT('Ctrl Pts',(-25.8021625084514,7.58581364664845,-60.4878171982801));
#45691=CARTESIAN_POINT('Ctrl Pts',(-25.8524352509597,8.0611970776665,-61.4656187046925));
#45692=CARTESIAN_POINT('Ctrl Pts',(-25.90252465855,8.55513729052697,-62.4492671574831));
#45693=CARTESIAN_POINT('Ctrl Pts',(-25.928651178022,8.83691687892463,-63.0037282242701));
#45694=CARTESIAN_POINT('Ctrl Pts',(-25.944371873633,9.02523196372997,-63.373608830517));
#45695=CARTESIAN_POINT('Ctrl Pts',(-25.9543434819169,9.15082245505529,-63.6202400576412));
#45696=CARTESIAN_POINT('Ctrl Pts',(-25.9634734726841,9.27634197235377,-63.8668663154678));
#45697=CARTESIAN_POINT('Ctrl Pts',(-25.9705707619772,9.38593094629149,-64.0826638689853));
#45698=CARTESIAN_POINT('Ctrl Pts',(-25.9743509373666,9.44845327423451,-64.205966795196));
#45699=CARTESIAN_POINT('Ctrl Pts',(-25.9797346364237,9.54211734605829,-64.3908984026352));
#45700=CARTESIAN_POINT('Ctrl Pts',(-25.9836044565101,9.61990677396525,-64.5449847761923));
#45701=CARTESIAN_POINT('Ctrl Pts',(-25.9890686033632,9.74807232430769,-64.7998073145916));
#45702=CARTESIAN_POINT('Ctrl Pts',(-25.9941273732596,9.8747278984663,-65.0500852591708));
#45703=CARTESIAN_POINT('Ctrl Pts',(-26.0019533277936,10.1327864314665,-65.5545426485505));
#45704=CARTESIAN_POINT('Ctrl Pts',(-26.0103402635887,10.5858336795818,-66.4269375967908));
#45705=CARTESIAN_POINT('Ctrl Pts',(-26.0107942689654,11.5053252365357,-68.1563355054035));
#45706=CARTESIAN_POINT('Ctrl Pts',(-25.999427322288,12.3081687393399,-69.635923753248));
#45707=CARTESIAN_POINT('Ctrl Pts',(-26.0007804305651,12.9122366459945,-70.7750284298339));
#45708=CARTESIAN_POINT('Ctrl Pts',(-26.0010398240432,13.0447978230638,-71.0249228148133));
#45709=CARTESIAN_POINT('Ctrl Pts',(-26.0014260269405,13.3112219759726,-71.5268614383352));
#45710=CARTESIAN_POINT('Ctrl Pts',(-26.0016831772529,13.6439024713188,-72.1531133439487));
#45711=CARTESIAN_POINT('Ctrl Pts',(-26.0017116603525,14.0436285487339,-72.904950139645));
#45712=CARTESIAN_POINT('Ctrl Pts',(-26.001378475861,14.8432872869915,-74.4081331829722));
#45713=CARTESIAN_POINT('Ctrl Pts',(-26.0006442548659,15.5102605444829,-75.6608410472288));
#45714=CARTESIAN_POINT('Ctrl Pts',(-26.0006503198601,16.4805469958596,-77.4856768722736));
#45715=CARTESIAN_POINT('Ctrl Pts',(-26.0006527044304,16.9168473443495,-78.3062345927038));
#45716=CARTESIAN_POINT('Ctrl Pts',(-26.0006527044303,17.353368931739,-79.1272122948021));
#45717=CARTESIAN_POINT('Ctrl Pts',(-24.4328318080232,4.08203882016111,24.8306371264184));
#45718=CARTESIAN_POINT('Ctrl Pts',(-24.4329049339045,4.0820388383689,24.7817578938191));
#45719=CARTESIAN_POINT('Ctrl Pts',(-24.4329816263336,4.08203885856826,24.7328797194657));
#45720=CARTESIAN_POINT('Ctrl Pts',(-24.4338873085871,4.08203904250686,24.1822724775926));
#45721=CARTESIAN_POINT('Ctrl Pts',(-24.4345815096013,4.08204034390179,23.1781378187383));
#45722=CARTESIAN_POINT('Ctrl Pts',(-24.4361966771044,4.08204501789817,21.1695406054735));
#45723=CARTESIAN_POINT('Ctrl Pts',(-24.4422245118959,4.08204573173726,19.6653857265717));
#45724=CARTESIAN_POINT('Ctrl Pts',(-24.4550083596785,4.08204123836197,18.4143357624134));
#45725=CARTESIAN_POINT('Ctrl Pts',(-24.461139366778,4.08203963145082,17.9115238657484));
#45726=CARTESIAN_POINT('Ctrl Pts',(-24.4765351484309,4.08203632002672,16.9075371526626));
#45727=CARTESIAN_POINT('Ctrl Pts',(-24.5095575369227,4.08202883184548,15.1537261634006));
#45728=CARTESIAN_POINT('Ctrl Pts',(-24.5409310461033,4.08201346651148,13.6519635833544));
#45729=CARTESIAN_POINT('Ctrl Pts',(-24.5605971654187,4.08199050068771,12.3974651968261));
#45730=CARTESIAN_POINT('Ctrl Pts',(-24.5686366192223,4.08197955945333,11.8965012353701));
#45731=CARTESIAN_POINT('Ctrl Pts',(-24.5850253084715,4.08195250599241,10.8946432184679));
#45732=CARTESIAN_POINT('Ctrl Pts',(-24.6052886162435,4.08191075176859,9.64210302146757));
#45733=CARTESIAN_POINT('Ctrl Pts',(-24.6266610628654,4.08186049614118,8.13760746381553));
#45734=CARTESIAN_POINT('Ctrl Pts',(-24.6372300407483,4.08183116969183,7.13291059862724));
#45735=CARTESIAN_POINT('Ctrl Pts',(-24.6421399318701,4.08181766181541,6.50493464946377));
#45736=CARTESIAN_POINT('Ctrl Pts',(-24.6439794711074,4.08180069432847,6.25456031789306));
#45737=CARTESIAN_POINT('Ctrl Pts',(-24.6472120730065,4.08172914744407,5.7532871677214));
#45738=CARTESIAN_POINT('Ctrl Pts',(-24.6517372559496,4.08152611618778,4.87468424116016));
#45739=CARTESIAN_POINT('Ctrl Pts',(-24.6565509082759,4.08100382920229,3.11456026023057));
#45740=CARTESIAN_POINT('Ctrl Pts',(-24.6544724421558,4.08096941635004,1.60884222114878));
#45741=CARTESIAN_POINT('Ctrl Pts',(-24.6510280232343,4.08176327560631,0.550492677300362));
#45742=CARTESIAN_POINT('Ctrl Pts',(-24.6505764402692,4.0818674887422,0.424505967923186));
#45743=CARTESIAN_POINT('Ctrl Pts',(-24.6495208106213,4.08210721288495,0.172673872967497));
#45744=CARTESIAN_POINT('Ctrl Pts',(-24.6472916185596,4.08260571194979,-0.267573473778777));
#45745=CARTESIAN_POINT('Ctrl Pts',(-24.6431379587548,4.08350722699859,-0.89539679214541));
#45746=CARTESIAN_POINT('Ctrl Pts',(-24.6369546732155,4.08481003070192,-1.64746533107212));
#45747=CARTESIAN_POINT('Ctrl Pts',(-24.6276191157051,4.08669315246911,-2.6490839377641));
#45748=CARTESIAN_POINT('Ctrl Pts',(-24.6147929138544,4.08909943830927,-3.90010599264371));
#45749=CARTESIAN_POINT('Ctrl Pts',(-24.6052760567306,4.09052613332115,-4.90226333565535));
#45750=CARTESIAN_POINT('Ctrl Pts',(-24.6001745652444,4.0911094069591,-5.52984284895121));
#45751=CARTESIAN_POINT('Ctrl Pts',(-24.5981139992996,4.09133854899239,-5.78075163694452));
#45752=CARTESIAN_POINT('Ctrl Pts',(-24.5939307763709,4.09176691364529,-6.28304411230748));
#45753=CARTESIAN_POINT('Ctrl Pts',(-24.5864961556743,4.0924340328852,-7.16255514817445));
#45754=CARTESIAN_POINT('Ctrl Pts',(-24.5758102198082,4.09311888145363,-8.41971103227847));
#45755=CARTESIAN_POINT('Ctrl Pts',(-24.5657198327711,4.09336487731083,-9.67493210132952));
#45756=CARTESIAN_POINT('Ctrl Pts',(-24.5593270395084,4.09326574663779,-10.5511417958087));
#45757=CARTESIAN_POINT('Ctrl Pts',(-24.5559184005747,4.09312458412497,-11.0509217702293));
#45758=CARTESIAN_POINT('Ctrl Pts',(-24.5543044100236,4.09302472042004,-11.3004728765148));
#45759=CARTESIAN_POINT('Ctrl Pts',(-24.5531258794835,4.09293825499699,-11.4882861671064));
#45760=CARTESIAN_POINT('Ctrl Pts',(-24.5523292371509,4.09286885279553,-11.6146582364255));
#45761=CARTESIAN_POINT('Ctrl Pts',(-24.5507230495914,4.09268856485644,-11.8669790977079));
#45762=CARTESIAN_POINT('Ctrl Pts',(-24.5478895447913,4.0922717256907,-12.3078288871903));
#45763=CARTESIAN_POINT('Ctrl Pts',(-24.5422194094636,4.09109236813779,-13.1868118100637));
#45764=CARTESIAN_POINT('Ctrl Pts',(-24.5345995785184,4.08879228071369,-14.4370658744763));
#45765=CARTESIAN_POINT('Ctrl Pts',(-24.5295037913775,4.08683613387482,-15.5611030676991));
#45766=CARTESIAN_POINT('Ctrl Pts',(-24.5273395914017,4.08593960406076,-16.3122009915398));
#45767=CARTESIAN_POINT('Ctrl Pts',(-24.5262586921781,4.08547557780888,-16.81354768392));
#45768=CARTESIAN_POINT('Ctrl Pts',(-24.5258891314335,4.08529768429567,-17.1904158183016));
#45769=CARTESIAN_POINT('Ctrl Pts',(-24.525871558669,4.08527938997473,-17.5043838498736));
#45770=CARTESIAN_POINT('Ctrl Pts',(-24.5258950789288,4.08526014193185,-17.6294009867654));
#45771=CARTESIAN_POINT('Ctrl Pts',(-24.5260591397072,4.08517981266925,-17.8790538820908));
#45772=CARTESIAN_POINT('Ctrl Pts',(-24.5263888608286,4.08504415175307,-18.1288802872769));
#45773=CARTESIAN_POINT('Ctrl Pts',(-24.5268735697162,4.08487513717692,-18.3786568942798));
#45774=CARTESIAN_POINT('Ctrl Pts',(-24.5272366949415,4.08475852743056,-18.5347981650712));
#45775=CARTESIAN_POINT('Ctrl Pts',(-24.5275622637412,4.08466156176116,-18.6597126134333));
#45776=CARTESIAN_POINT('Ctrl Pts',(-24.5278232220106,4.08458737978976,-18.7534044844896));
#45777=CARTESIAN_POINT('Ctrl Pts',(-24.5280542699026,4.08452484047191,-18.8314840644228));
#45778=CARTESIAN_POINT('Ctrl Pts',(-24.528247206293,4.08447476208227,-18.8939501719104));
#45779=CARTESIAN_POINT('Ctrl Pts',(-24.5299314546868,4.084049330607,-19.42492452698));
#45780=CARTESIAN_POINT('Ctrl Pts',(-24.5344449948442,4.08321387971141,-20.440489043094));
#45781=CARTESIAN_POINT('Ctrl Pts',(-24.543292732778,4.08453791394782,-21.9420823662568));
#45782=CARTESIAN_POINT('Ctrl Pts',(-24.5492197690682,4.0886038396778,-22.9447655341206));
#45783=CARTESIAN_POINT('Ctrl Pts',(-24.5526086662065,4.09268061333238,-23.5702445968926));
#45784=CARTESIAN_POINT('Ctrl Pts',(-24.5540154132293,4.09451599983593,-23.8169099228532));
#45785=CARTESIAN_POINT('Ctrl Pts',(-24.5570285573681,4.09898656854328,-24.3122487178896));
#45786=CARTESIAN_POINT('Ctrl Pts',(-24.56276692588,4.1086444896345,-25.1821960973038));
#45787=CARTESIAN_POINT('Ctrl Pts',(-24.5717213878898,4.1260537718618,-26.4337457009266));
#45788=CARTESIAN_POINT('Ctrl Pts',(-24.5823806002763,4.14782107631549,-27.9449849114494));
#45789=CARTESIAN_POINT('Ctrl Pts',(-24.5882113254279,4.15925502228168,-28.9563911373271));
#45790=CARTESIAN_POINT('Ctrl Pts',(-24.5909041335844,4.16385336794095,-29.5254986098915));
#45791=CARTESIAN_POINT('Ctrl Pts',(-24.5914883029049,4.16486110508338,-29.6508494551747));
#45792=CARTESIAN_POINT('Ctrl Pts',(-24.5925818190287,4.16684169819357,-29.9022586813579));
#45793=CARTESIAN_POINT('Ctrl Pts',(-24.5943078067308,4.17019215812943,-30.3421240539426));
#45794=CARTESIAN_POINT('Ctrl Pts',(-24.5971328074952,4.17640539766817,-31.222757091628));
#45795=CARTESIAN_POINT('Ctrl Pts',(-24.5999405591706,4.18360004719004,-32.4819446905374));
#45796=CARTESIAN_POINT('Ctrl Pts',(-24.6026962750198,4.18782846510269,-33.7408644899318));
#45797=CARTESIAN_POINT('Ctrl Pts',(-24.6058556550442,4.18902405819699,-34.7465161247673));
#45798=CARTESIAN_POINT('Ctrl Pts',(-24.6078798771038,4.18880809483548,-35.2487775798259));
#45799=CARTESIAN_POINT('Ctrl Pts',(-24.6096428164083,4.18831568843446,-35.6261321945983));
#45800=CARTESIAN_POINT('Ctrl Pts',(-24.6109922385861,4.18783075681031,-35.8793571817228));
#45801=CARTESIAN_POINT('Ctrl Pts',(-24.6142480612817,4.18627899067943,-36.3845573802002));
#45802=CARTESIAN_POINT('Ctrl Pts',(-24.6211264422861,4.18222070996565,-37.2671076307625));
#45803=CARTESIAN_POINT('Ctrl Pts',(-24.6373570395079,4.16961321135485,-39.0249602698805));
#45804=CARTESIAN_POINT('Ctrl Pts',(-24.6481151660576,4.15524941752727,-40.529029949255));
#45805=CARTESIAN_POINT('Ctrl Pts',(-24.6468650886017,4.14524912570874,-41.7847319913609));
#45806=CARTESIAN_POINT('Ctrl Pts',(-24.6461897055816,4.13911340038055,-42.1793898963392));
#45807=CARTESIAN_POINT('Ctrl Pts',(-24.644668791987,4.12738681795716,-42.6898623098505));
#45808=CARTESIAN_POINT('Ctrl Pts',(-24.6427330915817,4.11399518827006,-43.1996065381906));
#45809=CARTESIAN_POINT('Ctrl Pts',(-24.6395043903164,4.09555658875821,-43.8290856052551));
#45810=CARTESIAN_POINT('Ctrl Pts',(-24.6342765471189,4.0749930739795,-44.5742566312117));
#45811=CARTESIAN_POINT('Ctrl Pts',(-24.628737628711,4.062590230283,-45.1855434242497));
#45812=CARTESIAN_POINT('Ctrl Pts',(-24.6235099419859,4.0573912958463,-45.668414193604));
#45813=CARTESIAN_POINT('Ctrl Pts',(-24.6192060886881,4.05635426243155,-46.0275212789887));
#45814=CARTESIAN_POINT('Ctrl Pts',(-24.6145069503963,4.05863219077922,-46.383481956892));
#45815=CARTESIAN_POINT('Ctrl Pts',(-24.6076814086831,4.06666093590869,-46.8537993280201));
#45816=CARTESIAN_POINT('Ctrl Pts',(-24.6019872099252,4.07901552762075,-47.2016372979207));
#45817=CARTESIAN_POINT('Ctrl Pts',(-24.5958055099508,4.09641618661044,-47.5474421678294));
#45818=CARTESIAN_POINT('Ctrl Pts',(-24.5913712683569,4.10934105902638,-47.8029417046537));
#45819=CARTESIAN_POINT('Ctrl Pts',(-24.5814056235319,4.13531445476801,-48.2963911892102));
#45820=CARTESIAN_POINT('Ctrl Pts',(-24.56146850896,4.18490193876664,-49.1575863425959));
#45821=CARTESIAN_POINT('Ctrl Pts',(-24.5279458200227,4.27556608531903,-50.3562070638942));
#45822=CARTESIAN_POINT('Ctrl Pts',(-24.4858938315039,4.4428837539764,-51.7517739671845));
#45823=CARTESIAN_POINT('Ctrl Pts',(-24.461390157077,4.60900827143757,-52.6525716423806));
#45824=CARTESIAN_POINT('Ctrl Pts',(-24.4484905108795,4.73487136224401,-53.209174977372));
#45825=CARTESIAN_POINT('Ctrl Pts',(-24.4430521465422,4.7887282884734,-53.4373806697681));
#45826=CARTESIAN_POINT('Ctrl Pts',(-24.4317192066847,4.90549509712483,-53.8956606386991));
#45827=CARTESIAN_POINT('Ctrl Pts',(-24.4109944470492,5.13372131329,-54.7067363051391));
#45828=CARTESIAN_POINT('Ctrl Pts',(-24.3692471227293,5.6763881660845,-56.3563509132911));
#45829=CARTESIAN_POINT('Ctrl Pts',(-24.3437675480632,6.25879991271785,-57.8032062975063));
#45830=CARTESIAN_POINT('Ctrl Pts',(-24.341029342272,6.69397786084169,-58.8307086524388));
#45831=CARTESIAN_POINT('Ctrl Pts',(-24.3411208671879,6.74332718681714,-58.9458372518527));
#45832=CARTESIAN_POINT('Ctrl Pts',(-24.3417062019115,6.84711130653536,-59.1827509561341));
#45833=CARTESIAN_POINT('Ctrl Pts',(-24.3441622193476,7.03433766881384,-59.597104178985));
#45834=CARTESIAN_POINT('Ctrl Pts',(-24.3536724791938,7.43467527392181,-60.4373789937337));
#45835=CARTESIAN_POINT('Ctrl Pts',(-24.3717943585678,7.93771663556469,-61.4133876658175));
#45836=CARTESIAN_POINT('Ctrl Pts',(-24.3912062535787,8.46470278441751,-62.4007111868074));
#45837=CARTESIAN_POINT('Ctrl Pts',(-24.4015908839533,8.76565248391554,-62.9592074918713));
#45838=CARTESIAN_POINT('Ctrl Pts',(-24.4078408521788,8.96641401262123,-63.3326671659236));
#45839=CARTESIAN_POINT('Ctrl Pts',(-24.4118013418662,9.10017247081078,-63.5819311992385));
#45840=CARTESIAN_POINT('Ctrl Pts',(-24.4153964693371,9.23358342739155,-63.8315662393309));
#45841=CARTESIAN_POINT('Ctrl Pts',(-24.4181517556313,9.34974746755446,-64.0503614778889));
#45842=CARTESIAN_POINT('Ctrl Pts',(-24.4196013510527,9.41591411187275,-64.1754862316753));
#45843=CARTESIAN_POINT('Ctrl Pts',(-24.4216454967201,9.5149237269704,-64.363260414974));
#45844=CARTESIAN_POINT('Ctrl Pts',(-24.4230600410192,9.59689381836826,-64.5199556443652));
#45845=CARTESIAN_POINT('Ctrl Pts',(-24.4249609908961,9.73152040519062,-64.7794075712368));
#45846=CARTESIAN_POINT('Ctrl Pts',(-24.4267618223247,9.86311129565224,-65.0323219641432));
#45847=CARTESIAN_POINT('Ctrl Pts',(-24.4296434015535,10.1299209242335,-65.5426374353664));
#45848=CARTESIAN_POINT('Ctrl Pts',(-24.4330147835845,10.5934173267333,-66.4232263642777));
#45849=CARTESIAN_POINT('Ctrl Pts',(-24.4345492745441,11.5191264205175,-68.1634877083546));
#45850=CARTESIAN_POINT('Ctrl Pts',(-24.4318062287518,12.3123138158534,-69.6410995187623));
#45851=CARTESIAN_POINT('Ctrl Pts',(-24.432600721665,12.9138097618783,-70.7735299662248));
#45852=CARTESIAN_POINT('Ctrl Pts',(-24.4327582500792,13.0469292258093,-71.0241120680269));
#45853=CARTESIAN_POINT('Ctrl Pts',(-24.4329908948791,13.3136862027866,-71.5261396769025));
#45854=CARTESIAN_POINT('Ctrl Pts',(-24.4331415881787,13.6468365578975,-72.1529333484963));
#45855=CARTESIAN_POINT('Ctrl Pts',(-24.4331565772736,14.0467232319219,-72.9050401218054));
#45856=CARTESIAN_POINT('Ctrl Pts',(-24.4329502855999,14.8463826590023,-74.4087072420885));
#45857=CARTESIAN_POINT('Ctrl Pts',(-24.4324854674872,15.5126901449289,-75.661261113541));
#45858=CARTESIAN_POINT('Ctrl Pts',(-24.4324768503252,16.4826221707385,-77.4854635085514));
#45859=CARTESIAN_POINT('Ctrl Pts',(-24.4324724381068,16.9190261641936,-78.3062332170589));
#45860=CARTESIAN_POINT('Ctrl Pts',(-24.4324724381067,17.3555477515831,-79.1272109191574));
#45861=CARTESIAN_POINT('Ctrl Pts',(-21.9235774316919,4.08176546808655,24.8306369193277));
#45862=CARTESIAN_POINT('Ctrl Pts',(-21.9236428686436,4.08176559550084,24.7817576776117));
#45863=CARTESIAN_POINT('Ctrl Pts',(-21.9237115034019,4.08176572794409,24.7328794977117));
#45864=CARTESIAN_POINT('Ctrl Pts',(-21.9245217528927,4.08176734214813,24.1822720255645));
#45865=CARTESIAN_POINT('Ctrl Pts',(-21.9251390018536,4.08177000133521,23.1781358417132));
#45866=CARTESIAN_POINT('Ctrl Pts',(-21.9265775308832,4.08177621167794,21.1695385153907));
#45867=CARTESIAN_POINT('Ctrl Pts',(-21.931967300021,4.08178749152863,19.6653818684061));
#45868=CARTESIAN_POINT('Ctrl Pts',(-21.9434164377662,4.08180437977525,18.4143314897164));
#45869=CARTESIAN_POINT('Ctrl Pts',(-21.9489070469889,4.08181284441495,17.9115194314412));
#45870=CARTESIAN_POINT('Ctrl Pts',(-21.962692535589,4.08183510532099,16.9075317986474));
#45871=CARTESIAN_POINT('Ctrl Pts',(-21.9922632008758,4.08188221339639,15.1537188588092));
#45872=CARTESIAN_POINT('Ctrl Pts',(-22.0203613754922,4.08192202667274,13.6519498725972));
#45873=CARTESIAN_POINT('Ctrl Pts',(-22.0380013105594,4.08193332806647,12.3974494658034));
#45874=CARTESIAN_POINT('Ctrl Pts',(-22.0452156220464,4.08193637672117,11.8964850375535));
#45875=CARTESIAN_POINT('Ctrl Pts',(-22.0599343937993,4.08193706348693,10.8946266597817));
#45876=CARTESIAN_POINT('Ctrl Pts',(-22.0781357558683,4.08193323531193,9.64208318336994));
#45877=CARTESIAN_POINT('Ctrl Pts',(-22.0973540656548,4.08192056571144,8.13758194942714));
#45878=CARTESIAN_POINT('Ctrl Pts',(-22.1068473001385,4.08191491682695,7.13288362235554));
#45879=CARTESIAN_POINT('Ctrl Pts',(-22.1112625152373,4.08191090019794,6.50489136045323));
#45880=CARTESIAN_POINT('Ctrl Pts',(-22.1129339805934,4.08187071317327,6.2541756805871));
#45881=CARTESIAN_POINT('Ctrl Pts',(-22.1159302305084,4.08166530353184,5.75253329691742));
#45882=CARTESIAN_POINT('Ctrl Pts',(-22.1202552130462,4.08105636817354,4.87346500119448));
#45883=CARTESIAN_POINT('Ctrl Pts',(-22.1252904987501,4.07943127155768,3.11362229719922));
#45884=CARTESIAN_POINT('Ctrl Pts',(-22.1233486580589,4.07943847898292,1.61002085166886));
#45885=CARTESIAN_POINT('Ctrl Pts',(-22.1191273452128,4.08201502643112,0.554171951867155));
#45886=CARTESIAN_POINT('Ctrl Pts',(-22.1185809770122,4.08234757373234,0.428627811525919));
#45887=CARTESIAN_POINT('Ctrl Pts',(-22.1173048402443,4.08311757684658,0.17754258976633));
#45888=CARTESIAN_POINT('Ctrl Pts',(-22.1146233333163,4.08471885183798,-0.261483756755618));
#45889=CARTESIAN_POINT('Ctrl Pts',(-22.1096271138227,4.08763792655448,-0.887964206484821));
#45890=CARTESIAN_POINT('Ctrl Pts',(-22.1023004342366,4.09180755483889,-1.63901543576647));
#45891=CARTESIAN_POINT('Ctrl Pts',(-22.0912885877694,4.09784759942708,-2.6400937353228));
#45892=CARTESIAN_POINT('Ctrl Pts',(-22.0764800317693,4.10546290482369,-3.89197073679173));
#45893=CARTESIAN_POINT('Ctrl Pts',(-22.0658875624004,4.10997294524229,-4.89651629795362));
#45894=CARTESIAN_POINT('Ctrl Pts',(-22.0604649547566,4.11175755709603,-5.52609779188864));
#45895=CARTESIAN_POINT('Ctrl Pts',(-22.0582785674025,4.11241613965768,-5.77736459149553));
#45896=CARTESIAN_POINT('Ctrl Pts',(-22.0538560973387,4.11355327378553,-6.28052764005114));
#45897=CARTESIAN_POINT('Ctrl Pts',(-22.0460405611013,4.11509599517109,-7.16122110620086));
#45898=CARTESIAN_POINT('Ctrl Pts',(-22.035023317356,4.11621653725926,-8.41952646924223));
#45899=CARTESIAN_POINT('Ctrl Pts',(-22.0252072449018,4.11638702652465,-9.67504511381552));
#45900=CARTESIAN_POINT('Ctrl Pts',(-22.0195001493991,4.11626305230175,-10.551046327456));
#45901=CARTESIAN_POINT('Ctrl Pts',(-22.0166399907367,4.11616099750827,-11.0505806179339));
#45902=CARTESIAN_POINT('Ctrl Pts',(-22.0153552585612,4.11610556640313,-11.2999664615218));
#45903=CARTESIAN_POINT('Ctrl Pts',(-22.0144478134254,4.11606442341051,-11.4876435024608));
#45904=CARTESIAN_POINT('Ctrl Pts',(-22.0138540387184,4.11602448348753,-11.6140705917933));
#45905=CARTESIAN_POINT('Ctrl Pts',(-22.0127286463286,4.1158983005132,-11.8664185595357));
#45906=CARTESIAN_POINT('Ctrl Pts',(-22.0109169925421,4.11556438990738,-12.3073563182658));
#45907=CARTESIAN_POINT('Ctrl Pts',(-22.0078885129695,4.11451108817903,-13.1864755014533));
#45908=CARTESIAN_POINT('Ctrl Pts',(-22.0051097943091,4.11227698280468,-14.4369204185599));
#45909=CARTESIAN_POINT('Ctrl Pts',(-22.0040372306832,4.11030463130404,-15.5610660660364));
#45910=CARTESIAN_POINT('Ctrl Pts',(-22.0037316517172,4.10937886081918,-16.3122209837995));
#45911=CARTESIAN_POINT('Ctrl Pts',(-22.0036266412943,4.1088893913568,-16.8136025089925));
#45912=CARTESIAN_POINT('Ctrl Pts',(-22.0036438981547,4.10870264560642,-17.1904843263817));
#45913=CARTESIAN_POINT('Ctrl Pts',(-22.0036951917498,4.10867018543604,-17.504465564421));
#45914=CARTESIAN_POINT('Ctrl Pts',(-22.0037659889596,4.10864491725128,-17.6294775934659));
#45915=CARTESIAN_POINT('Ctrl Pts',(-22.0040932027344,4.10855121224841,-17.8791295662324));
#45916=CARTESIAN_POINT('Ctrl Pts',(-22.0046769151716,4.10840623448712,-18.128953820262));
#45917=CARTESIAN_POINT('Ctrl Pts',(-22.0054653914267,4.10822204803957,-18.3787349404948));
#45918=CARTESIAN_POINT('Ctrl Pts',(-22.0060346622479,4.10809664613784,-18.5348796170474));
#45919=CARTESIAN_POINT('Ctrl Pts',(-22.0065291810761,4.10799121967166,-18.6597981955137));
#45920=CARTESIAN_POINT('Ctrl Pts',(-22.0069183975559,4.10791064669469,-18.7534935134071));
#45921=CARTESIAN_POINT('Ctrl Pts',(-22.0072567799537,4.10784275398157,-18.8315762882781));
#45922=CARTESIAN_POINT('Ctrl Pts',(-22.0075349816406,4.10778802035585,-18.894045286408));
#45923=CARTESIAN_POINT('Ctrl Pts',(-22.0099407089767,4.10732251351153,-19.4250452507967));
#45924=CARTESIAN_POINT('Ctrl Pts',(-22.0158676273032,4.10658108446762,-20.4406319853658));
#45925=CARTESIAN_POINT('Ctrl Pts',(-22.0218521912948,4.1077345212265,-21.9424997642546));
#45926=CARTESIAN_POINT('Ctrl Pts',(-22.0200896140808,4.11183365881191,-22.9454014931823));
#45927=CARTESIAN_POINT('Ctrl Pts',(-22.0158233431142,4.11578937010123,-23.5710372694473));
#45928=CARTESIAN_POINT('Ctrl Pts',(-22.0137758059422,4.11755454093115,-23.8178873383974));
#45929=CARTESIAN_POINT('Ctrl Pts',(-22.0084421212236,4.12185513611334,-24.313458612243));
#45930=CARTESIAN_POINT('Ctrl Pts',(-21.996249555066,4.13108818609894,-25.183677492712));
#45931=CARTESIAN_POINT('Ctrl Pts',(-21.9731850864931,4.14778597539684,-26.435164267108));
#45932=CARTESIAN_POINT('Ctrl Pts',(-21.9439116701733,4.16816279907211,-27.9458140794481));
#45933=CARTESIAN_POINT('Ctrl Pts',(-21.9287075806292,4.17906693665825,-28.9567014536259));
#45934=CARTESIAN_POINT('Ctrl Pts',(-21.9227518086004,4.18345337480103,-29.5254560071513));
#45935=CARTESIAN_POINT('Ctrl Pts',(-21.9214223740837,4.18441027764442,-29.6505983758409));
#45936=CARTESIAN_POINT('Ctrl Pts',(-21.9187727102683,4.1863190461755,-29.9016929409507));
#45937=CARTESIAN_POINT('Ctrl Pts',(-21.9141834554257,4.1896264486792,-30.3410451571695));
#45938=CARTESIAN_POINT('Ctrl Pts',(-21.9053248870368,4.19600438719776,-31.2209681407571));
#45939=CARTESIAN_POINT('Ctrl Pts',(-21.8944820204112,4.20391937808385,-32.4800239120499));
#45940=CARTESIAN_POINT('Ctrl Pts',(-21.8883548098301,4.20881889042443,-33.7400425912776));
#45941=CARTESIAN_POINT('Ctrl Pts',(-21.887617639785,4.2100143207476,-34.7472698398653));
#45942=CARTESIAN_POINT('Ctrl Pts',(-21.8889042016303,4.20958736160925,-35.2505797237338));
#45943=CARTESIAN_POINT('Ctrl Pts',(-21.8905619685024,4.20881940597667,-35.6288061396665));
#45944=CARTESIAN_POINT('Ctrl Pts',(-21.8920068332931,4.20808942994181,-35.8828728206073));
#45945=CARTESIAN_POINT('Ctrl Pts',(-21.8961129240444,4.20589306531138,-36.3893572918887));
#45946=CARTESIAN_POINT('Ctrl Pts',(-21.9061707588451,4.20023175270841,-37.2737103685978));
#45947=CARTESIAN_POINT('Ctrl Pts',(-21.9349294377932,4.18375091830845,-39.0326417841188));
#45948=CARTESIAN_POINT('Ctrl Pts',(-21.9646241043132,4.16583014116949,-40.5339723279037));
#45949=CARTESIAN_POINT('Ctrl Pts',(-21.9813682042444,4.15557559944031,-41.7856626536357));
#45950=CARTESIAN_POINT('Ctrl Pts',(-21.9860152656383,4.1495633104421,-42.1793854201093));
#45951=CARTESIAN_POINT('Ctrl Pts',(-21.9917218274079,4.1383477020153,-42.6888104928429));
#45952=CARTESIAN_POINT('Ctrl Pts',(-21.9971702168111,4.12558636061383,-43.1977055694632));
#45953=CARTESIAN_POINT('Ctrl Pts',(-22.0036410011809,4.10815216686057,-43.8264437346378));
#45954=CARTESIAN_POINT('Ctrl Pts',(-22.0112963508797,4.08889718092569,-44.5712397154641));
#45955=CARTESIAN_POINT('Ctrl Pts',(-22.0179509165056,4.07749348765273,-45.1826267742738));
#45956=CARTESIAN_POINT('Ctrl Pts',(-22.0237023803601,4.07311486143883,-45.6657982945412));
#45957=CARTESIAN_POINT('Ctrl Pts',(-22.0282650992984,4.07260145483311,-46.0252489840544));
#45958=CARTESIAN_POINT('Ctrl Pts',(-22.0331340331778,4.07530161386567,-46.3816695806118));
#45959=CARTESIAN_POINT('Ctrl Pts',(-22.0401242868195,4.0837933675503,-46.8527419744537));
#45960=CARTESIAN_POINT('Ctrl Pts',(-22.0459496522703,4.09616001883859,-47.2013306630543));
#45961=CARTESIAN_POINT('Ctrl Pts',(-22.0523457940746,4.11353119813929,-47.5479470185623));
#45962=CARTESIAN_POINT('Ctrl Pts',(-22.0571608519188,4.12645431671799,-47.8028791297642));
#45963=CARTESIAN_POINT('Ctrl Pts',(-22.0685778662445,4.15244870291563,-48.296016830207));
#45964=CARTESIAN_POINT('Ctrl Pts',(-22.0923296902346,4.20194781231465,-49.1568596486614));
#45965=CARTESIAN_POINT('Ctrl Pts',(-22.1317430375304,4.29109922835001,-50.3567511143593));
#45966=CARTESIAN_POINT('Ctrl Pts',(-22.1713398710979,4.4542309928279,-51.7572733996303));
#45967=CARTESIAN_POINT('Ctrl Pts',(-22.181252446771,4.61655584852366,-52.6633750773003));
#45968=CARTESIAN_POINT('Ctrl Pts',(-22.1790138673735,4.7402119578729,-53.2236003657393));
#45969=CARTESIAN_POINT('Ctrl Pts',(-22.1773613312003,4.79340059150215,-53.4548939485341));
#45970=CARTESIAN_POINT('Ctrl Pts',(-22.1710616093439,4.90792124447746,-53.9173152546218));
#45971=CARTESIAN_POINT('Ctrl Pts',(-22.1532457320423,5.1306025270621,-54.7336427674677));
#45972=CARTESIAN_POINT('Ctrl Pts',(-22.097832810942,5.65648884714921,-56.3839152515343));
#45973=CARTESIAN_POINT('Ctrl Pts',(-22.0412804464425,6.22052514945947,-57.8189670582374));
#45974=CARTESIAN_POINT('Ctrl Pts',(-22.0189286249449,6.64905674783341,-58.8339790672758));
#45975=CARTESIAN_POINT('Ctrl Pts',(-22.0160598135343,6.6977875963569,-58.9478428819848));
#45976=CARTESIAN_POINT('Ctrl Pts',(-22.0104898930308,6.80055946754283,-59.1823098250968));
#45977=CARTESIAN_POINT('Ctrl Pts',(-22.0009046471323,6.98681000058887,-59.5929273377654));
#45978=CARTESIAN_POINT('Ctrl Pts',(-21.982673689945,7.38793968462431,-60.4275067502826));
#45979=CARTESIAN_POINT('Ctrl Pts',(-21.9642676050404,7.89731311453462,-61.4005064487699));
#45980=CARTESIAN_POINT('Ctrl Pts',(-21.9486371893967,8.4331972379869,-62.3874427884229));
#45981=CARTESIAN_POINT('Ctrl Pts',(-21.9409298355057,8.73956202027487,-62.9466873437175));
#45982=CARTESIAN_POINT('Ctrl Pts',(-21.9362778305471,8.94388529536134,-63.3210484177726));
#45983=CARTESIAN_POINT('Ctrl Pts',(-21.9333047699389,9.07997994977837,-63.5710250472529));
#45984=CARTESIAN_POINT('Ctrl Pts',(-21.9305422257701,9.21568664341698,-63.8215442929583));
#45985=CARTESIAN_POINT('Ctrl Pts',(-21.9283022575873,9.33374338713387,-64.0412705670625));
#45986=CARTESIAN_POINT('Ctrl Pts',(-21.9270760103423,9.40095793915379,-64.1669746443105));
#45987=CARTESIAN_POINT('Ctrl Pts',(-21.9252902074149,9.50149970378208,-64.355664476691));
#45988=CARTESIAN_POINT('Ctrl Pts',(-21.9239217402965,9.5846818151938,-64.5132321112613));
#45989=CARTESIAN_POINT('Ctrl Pts',(-21.9218097860302,9.72113866943812,-64.7742454997469));
#45990=CARTESIAN_POINT('Ctrl Pts',(-21.9199176222883,9.85377102502329,-65.0273934732946));
#45991=CARTESIAN_POINT('Ctrl Pts',(-21.9171231090912,10.122766700094,-65.5388654369393));
#45992=CARTESIAN_POINT('Ctrl Pts',(-21.914604314553,10.5891346610821,-66.4208834436944));
#45993=CARTESIAN_POINT('Ctrl Pts',(-21.9167516425982,11.518063809149,-68.1633649555777));
#45994=CARTESIAN_POINT('Ctrl Pts',(-21.9235258434315,12.3111662021817,-69.6409891056379));
#45995=CARTESIAN_POINT('Ctrl Pts',(-21.923595127208,12.9129986925668,-70.7726319617749));
#45996=CARTESIAN_POINT('Ctrl Pts',(-21.9236052602591,13.0463776976675,-71.0234454630726));
#45997=CARTESIAN_POINT('Ctrl Pts',(-21.9236212938625,13.3134462292093,-71.5256714763303));
#45998=CARTESIAN_POINT('Ctrl Pts',(-21.9236369455585,13.6469034947314,-72.1527626977125));
#45999=CARTESIAN_POINT('Ctrl Pts',(-21.9236407216763,14.0469291203077,-72.9050903947083));
#46000=CARTESIAN_POINT('Ctrl Pts',(-21.9236332599525,14.8465939166301,-74.4090732064259));
#46001=CARTESIAN_POINT('Ctrl Pts',(-21.9236258769294,15.5125217173332,-75.6615475097951));
#46002=CARTESIAN_POINT('Ctrl Pts',(-21.9236382256523,16.4822523474001,-77.4853125317373));
#46003=CARTESIAN_POINT('Ctrl Pts',(-21.9236445933878,16.9187529102801,-78.3062336744952));
#46004=CARTESIAN_POINT('Ctrl Pts',(-21.9236445933879,17.3552744976696,-79.1272113765938));
#46005=CARTESIAN_POINT('Ctrl Pts',(-19.4188565084394,4.07909071047731,24.8306335196013));
#46006=CARTESIAN_POINT('Ctrl Pts',(-19.4189144201637,4.07909071025974,24.7817541701314));
#46007=CARTESIAN_POINT('Ctrl Pts',(-19.4189751571496,4.0790907049392,24.7328758768994));
#46008=CARTESIAN_POINT('Ctrl Pts',(-19.4196923876615,4.07909087600898,24.1822672626248));
#46009=CARTESIAN_POINT('Ctrl Pts',(-19.4202407064515,4.07909166990852,23.1781304961313));
#46010=CARTESIAN_POINT('Ctrl Pts',(-19.4215160787714,4.07908986719448,21.1695310296501));
#46011=CARTESIAN_POINT('Ctrl Pts',(-19.426289339984,4.07909351817457,19.6653765872538));
#46012=CARTESIAN_POINT('Ctrl Pts',(-19.4364196794994,4.07909840105154,18.4143272842976));
#46013=CARTESIAN_POINT('Ctrl Pts',(-19.4412776063029,4.07910001848308,17.9115087189125));
#46014=CARTESIAN_POINT('Ctrl Pts',(-19.4534754210926,4.07910422482297,16.9075170749824));
#46015=CARTESIAN_POINT('Ctrl Pts',(-19.4796391806934,4.0791122270718,15.1537053608657));
#46016=CARTESIAN_POINT('Ctrl Pts',(-19.5045032710635,4.07913096690056,13.6519635683124));
#46017=CARTESIAN_POINT('Ctrl Pts',(-19.5201045959927,4.07914726620125,12.3974942144212));
#46018=CARTESIAN_POINT('Ctrl Pts',(-19.5264842586753,4.07915434258511,11.896542204204));
#46019=CARTESIAN_POINT('Ctrl Pts',(-19.5394958902427,4.07916874348645,10.8947012600692));
#46020=CARTESIAN_POINT('Ctrl Pts',(-19.5555899316981,4.07919772714864,9.64217422998216));
#46021=CARTESIAN_POINT('Ctrl Pts',(-19.5725737761371,4.07922586275185,8.13767545606689));
#46022=CARTESIAN_POINT('Ctrl Pts',(-19.5809711503705,4.07925222390256,7.13297024095191));
#46023=CARTESIAN_POINT('Ctrl Pts',(-19.5848728343503,4.07926169557044,6.50497879949647));
#46024=CARTESIAN_POINT('Ctrl Pts',(-19.5864491654674,4.0792439713941,6.25448301513597));
#46025=CARTESIAN_POINT('Ctrl Pts',(-19.5896190891136,4.07913977975641,5.75307864744289));
#46026=CARTESIAN_POINT('Ctrl Pts',(-19.5950152883982,4.07882488805074,4.8743156679763));
#46027=CARTESIAN_POINT('Ctrl Pts',(-19.6036496630048,4.07796294666085,3.11429706875541));
#46028=CARTESIAN_POINT('Ctrl Pts',(-19.6019882907535,4.07803371099858,1.6093259597056));
#46029=CARTESIAN_POINT('Ctrl Pts',(-19.5914809645,4.07953662306137,0.55191876525641));
#46030=CARTESIAN_POINT('Ctrl Pts',(-19.5901156534471,4.07973084939819,0.426115855158161));
#46031=CARTESIAN_POINT('Ctrl Pts',(-19.5869560461142,4.08018266915907,0.174592789548162));
#46032=CARTESIAN_POINT('Ctrl Pts',(-19.5803692316278,4.08112680912326,-0.2651329658887));
#46033=CARTESIAN_POINT('Ctrl Pts',(-19.5683254774567,4.08287488315803,-0.892339759225695));
#46034=CARTESIAN_POINT('Ctrl Pts',(-19.5508973207309,4.08537642564393,-1.64387354498816));
#46035=CARTESIAN_POINT('Ctrl Pts',(-19.5253228951273,4.08905894197638,-2.64510896972974));
#46036=CARTESIAN_POINT('Ctrl Pts',(-19.4920303955031,4.09375623345862,-3.89635263559461));
#46037=CARTESIAN_POINT('Ctrl Pts',(-19.4705336110349,4.09651502910892,-4.89961645688803));
#46038=CARTESIAN_POINT('Ctrl Pts',(-19.4608138031559,4.09751505218955,-5.52819109994924));
#46039=CARTESIAN_POINT('Ctrl Pts',(-19.4570673380576,4.09787183139317,-5.77948023960965));
#46040=CARTESIAN_POINT('Ctrl Pts',(-19.4500850879881,4.09840732325652,-6.2824257765495));
#46041=CARTESIAN_POINT('Ctrl Pts',(-19.4391418185303,4.09894170854077,-7.16281346606619));
#46042=CARTESIAN_POINT('Ctrl Pts',(-19.4266986568119,4.09882741407656,-8.42044957381485));
#46043=CARTESIAN_POINT('Ctrl Pts',(-19.4173000333354,4.09830972651637,-9.6751036262812));
#46044=CARTESIAN_POINT('Ctrl Pts',(-19.411683681216,4.09813931643307,-10.550346813374));
#46045=CARTESIAN_POINT('Ctrl Pts',(-19.4086593216313,4.09815973988217,-11.049410070983));
#46046=CARTESIAN_POINT('Ctrl Pts',(-19.4071935988682,4.09821928491534,-11.2985484047833));
#46047=CARTESIAN_POINT('Ctrl Pts',(-19.4061016703888,4.09828621552437,-11.4860268244713));
#46048=CARTESIAN_POINT('Ctrl Pts',(-19.4053889610689,4.09833451669103,-11.6120758387663));
#46049=CARTESIAN_POINT('Ctrl Pts',(-19.4040478993421,4.09844474528975,-11.8638542487384));
#46050=CARTESIAN_POINT('Ctrl Pts',(-19.4019142713054,4.09867082756035,-12.3038372498591));
#46051=CARTESIAN_POINT('Ctrl Pts',(-19.3984419752592,4.09923523312725,-13.1815572929444));
#46052=CARTESIAN_POINT('Ctrl Pts',(-19.3954236776363,4.10022022112895,-14.4313183962024));
#46053=CARTESIAN_POINT('Ctrl Pts',(-19.3942430125099,4.10101548245803,-15.5564931439516));
#46054=CARTESIAN_POINT('Ctrl Pts',(-19.3937611428457,4.10138097884389,-16.3090052985942));
#46055=CARTESIAN_POINT('Ctrl Pts',(-19.3934990598768,4.10157134265437,-16.8114637197718));
#46056=CARTESIAN_POINT('Ctrl Pts',(-19.3933453844142,4.10164968431484,-17.1893673535936));
#46057=CARTESIAN_POINT('Ctrl Pts',(-19.3932120541238,4.10166468090102,-17.5042559018109));
#46058=CARTESIAN_POINT('Ctrl Pts',(-19.3931882586075,4.10167787745367,-17.6286958130394));
#46059=CARTESIAN_POINT('Ctrl Pts',(-19.3932482448541,4.10172972165035,-17.8778588266014));
#46060=CARTESIAN_POINT('Ctrl Pts',(-19.393458056388,4.10181608223137,-18.1271358502433));
#46061=CARTESIAN_POINT('Ctrl Pts',(-19.3937911139831,4.10192414140768,-18.3766235315614));
#46062=CARTESIAN_POINT('Ctrl Pts',(-19.3940459177017,4.10199930922547,-18.532621742218));
#46063=CARTESIAN_POINT('Ctrl Pts',(-19.3942743151561,4.10206229662538,-18.6574686311859));
#46064=CARTESIAN_POINT('Ctrl Pts',(-19.3944572207307,4.10211079231994,-18.7511261562));
#46065=CARTESIAN_POINT('Ctrl Pts',(-19.3946186656907,4.10215198667377,-18.8291937325066));
#46066=CARTESIAN_POINT('Ctrl Pts',(-19.3947527847797,4.10218516304723,-18.8916592729327));
#46067=CARTESIAN_POINT('Ctrl Pts',(-19.3959200298335,4.10246849959459,-19.422682847279));
#46068=CARTESIAN_POINT('Ctrl Pts',(-19.3990121909925,4.10306965440659,-20.4400186150423));
#46069=CARTESIAN_POINT('Ctrl Pts',(-19.4026974986641,4.10265013343473,-21.9490122710558));
#46070=CARTESIAN_POINT('Ctrl Pts',(-19.4025081334354,4.1006829999806,-22.959760455145));
#46071=CARTESIAN_POINT('Ctrl Pts',(-19.4008678069037,4.09862369634203,-23.5912798455614));
#46072=CARTESIAN_POINT('Ctrl Pts',(-19.4000563059062,4.09769125775524,-23.8416787264623));
#46073=CARTESIAN_POINT('Ctrl Pts',(-19.3978729269907,4.09541369523697,-24.3427273431573));
#46074=CARTESIAN_POINT('Ctrl Pts',(-19.3927666416296,4.09048021303807,-25.2208302452691));
#46075=CARTESIAN_POINT('Ctrl Pts',(-19.382960522823,4.08155628938632,-26.4773520158594));
#46076=CARTESIAN_POINT('Ctrl Pts',(-19.3706483773465,4.0703783508801,-27.9846482869812));
#46077=CARTESIAN_POINT('Ctrl Pts',(-19.3645265659457,4.06445530686772,-28.9867106559561));
#46078=CARTESIAN_POINT('Ctrl Pts',(-19.3623143059621,4.06204892202967,-29.5487718058104));
#46079=CARTESIAN_POINT('Ctrl Pts',(-19.3617887426652,4.06152821541918,-29.6739785277925));
#46080=CARTESIAN_POINT('Ctrl Pts',(-19.3606271661027,4.06052591044494,-29.924295428993));
#46081=CARTESIAN_POINT('Ctrl Pts',(-19.3583456092779,4.05887871158711,-30.3626493341679));
#46082=CARTESIAN_POINT('Ctrl Pts',(-19.3531065570849,4.05597509268942,-31.2399346833751));
#46083=CARTESIAN_POINT('Ctrl Pts',(-19.3455509589286,4.05277684067842,-32.4945228341436));
#46084=CARTESIAN_POINT('Ctrl Pts',(-19.342886321836,4.05050865357068,-33.7487538153502));
#46085=CARTESIAN_POINT('Ctrl Pts',(-19.3466959544024,4.04908784624401,-34.7506312934264));
#46086=CARTESIAN_POINT('Ctrl Pts',(-19.3510933821798,4.04847947531361,-35.2509902487381));
#46087=CARTESIAN_POINT('Ctrl Pts',(-19.3555228250233,4.04805620740768,-35.6268907199721));
#46088=CARTESIAN_POINT('Ctrl Pts',(-19.3590680438941,4.04775668024797,-35.8791435250017));
#46089=CARTESIAN_POINT('Ctrl Pts',(-19.36816067504,4.04710559137667,-36.382362044537));
#46090=CARTESIAN_POINT('Ctrl Pts',(-19.3886133016165,4.04585131481258,-37.2613946857405));
#46091=CARTESIAN_POINT('Ctrl Pts',(-19.4419700485823,4.04379142196048,-39.0119443279322));
#46092=CARTESIAN_POINT('Ctrl Pts',(-19.4897443702684,4.04450815238889,-40.5099559810813));
#46093=CARTESIAN_POINT('Ctrl Pts',(-19.5092037083466,4.04898130135962,-41.7616588739113));
#46094=CARTESIAN_POINT('Ctrl Pts',(-19.5141254539957,4.04751785876212,-42.1556346767663));
#46095=CARTESIAN_POINT('Ctrl Pts',(-19.519258397388,4.04216514831402,-42.6647192527348));
#46096=CARTESIAN_POINT('Ctrl Pts',(-19.5235371682125,4.03534398895192,-43.173000899783));
#46097=CARTESIAN_POINT('Ctrl Pts',(-19.5274942672393,4.0254984979779,-43.8003461392944));
#46098=CARTESIAN_POINT('Ctrl Pts',(-19.5306677744146,4.01601169365967,-44.5425023123782));
#46099=CARTESIAN_POINT('Ctrl Pts',(-19.5325488160087,4.01356414554306,-45.1508563034701));
#46100=CARTESIAN_POINT('Ctrl Pts',(-19.5339462963064,4.01691209593236,-45.6311767756409));
#46101=CARTESIAN_POINT('Ctrl Pts',(-19.5350135354646,4.0225413178937,-45.988244691636));
#46102=CARTESIAN_POINT('Ctrl Pts',(-19.5361832905115,4.03175746973702,-46.3420566735754));
#46103=CARTESIAN_POINT('Ctrl Pts',(-19.537995792819,4.04944337200258,-46.8093552824749));
#46104=CARTESIAN_POINT('Ctrl Pts',(-19.5397356363166,4.06940154039066,-47.1547886134318));
#46105=CARTESIAN_POINT('Ctrl Pts',(-19.5419182619491,4.09479685435151,-47.4979406828226));
#46106=CARTESIAN_POINT('Ctrl Pts',(-19.5435334867921,4.1138493185823,-47.7456057168678));
#46107=CARTESIAN_POINT('Ctrl Pts',(-19.5472777159859,4.15410363555502,-48.2292431210855));
#46108=CARTESIAN_POINT('Ctrl Pts',(-19.5548283176533,4.23316883664525,-49.0770214660487));
#46109=CARTESIAN_POINT('Ctrl Pts',(-19.5665014862628,4.37257037850929,-50.273815532423));
#46110=CARTESIAN_POINT('Ctrl Pts',(-19.5759347453678,4.59321970380592,-51.6928488604303));
#46111=CARTESIAN_POINT('Ctrl Pts',(-19.5753145264093,4.78270750833221,-52.6256970027234));
#46112=CARTESIAN_POINT('Ctrl Pts',(-19.5717048935925,4.91701513352802,-53.2063435376452));
#46113=CARTESIAN_POINT('Ctrl Pts',(-19.5698774486865,4.97335057603374,-53.4432071091416));
#46114=CARTESIAN_POINT('Ctrl Pts',(-19.564839020945,5.09200111043759,-53.9168187775379));
#46115=CARTESIAN_POINT('Ctrl Pts',(-19.5528544887985,5.315862262297,-54.7488188928104));
#46116=CARTESIAN_POINT('Ctrl Pts',(-19.519714948239,5.82468467822303,-56.4189019825902));
#46117=CARTESIAN_POINT('Ctrl Pts',(-19.4875512323991,6.35507020672527,-57.8515777580455));
#46118=CARTESIAN_POINT('Ctrl Pts',(-19.4739216276912,6.76494875051892,-58.8574606822304));
#46119=CARTESIAN_POINT('Ctrl Pts',(-19.4722267612937,6.81250672350762,-58.9726691727967));
#46120=CARTESIAN_POINT('Ctrl Pts',(-19.4689282701839,6.91201454254276,-59.2082470192108));
#46121=CARTESIAN_POINT('Ctrl Pts',(-19.4633090465908,7.09221172375984,-59.6210873424176));
#46122=CARTESIAN_POINT('Ctrl Pts',(-19.4527741824522,7.47861963072649,-60.4579968506153));
#46123=CARTESIAN_POINT('Ctrl Pts',(-19.4424270794853,7.96727305279303,-61.4310058399773));
#46124=CARTESIAN_POINT('Ctrl Pts',(-19.4337880037515,8.4815689226549,-62.415404281155));
#46125=CARTESIAN_POINT('Ctrl Pts',(-19.42955639736,8.77612817315247,-62.9723177505061));
#46126=CARTESIAN_POINT('Ctrl Pts',(-19.4269982550432,8.97296445687754,-63.3446966839675));
#46127=CARTESIAN_POINT('Ctrl Pts',(-19.4253615222896,9.10419333608518,-63.5932357054671));
#46128=CARTESIAN_POINT('Ctrl Pts',(-19.423833517323,9.2352300133487,-63.8421327758543));
#46129=CARTESIAN_POINT('Ctrl Pts',(-19.422586985817,9.34943527202489,-64.0602672270396));
#46130=CARTESIAN_POINT('Ctrl Pts',(-19.421901420598,9.41452027800235,-64.18500938873));
#46131=CARTESIAN_POINT('Ctrl Pts',(-19.4208996084222,9.51194377766199,-64.3722033831314));
#46132=CARTESIAN_POINT('Ctrl Pts',(-19.420122800325,9.59268180683019,-64.5284065828826));
#46133=CARTESIAN_POINT('Ctrl Pts',(-19.4189102932834,9.72535993830748,-64.7870027589046));
#46134=CARTESIAN_POINT('Ctrl Pts',(-19.417812089868,9.85477348590642,-65.0381168227013));
#46135=CARTESIAN_POINT('Ctrl Pts',(-19.4161674651852,10.1184235473867,-65.5456921147163));
#46136=CARTESIAN_POINT('Ctrl Pts',(-19.4145954672988,10.5786112295253,-66.4220152425714));
#46137=CARTESIAN_POINT('Ctrl Pts',(-19.4154119518332,11.5053109976952,-68.1572980681037));
#46138=CARTESIAN_POINT('Ctrl Pts',(-19.4188586142071,12.3063044713339,-69.6365282019122));
#46139=CARTESIAN_POINT('Ctrl Pts',(-19.4187886877509,12.9106168296157,-70.7731110993884));
#46140=CARTESIAN_POINT('Ctrl Pts',(-19.4187743904881,13.0437826002373,-71.0235704261403));
#46141=CARTESIAN_POINT('Ctrl Pts',(-19.4187532716427,13.3108824368978,-71.5259270802934));
#46142=CARTESIAN_POINT('Ctrl Pts',(-19.4187412531874,13.6442196591592,-72.1528487987563));
#46143=CARTESIAN_POINT('Ctrl Pts',(-19.4187406843765,14.0442371429415,-72.9051710091742));
#46144=CARTESIAN_POINT('Ctrl Pts',(-19.4187613474451,14.8438780416534,-74.4090580694602));
#46145=CARTESIAN_POINT('Ctrl Pts',(-19.4188107046995,15.5098573501397,-75.6615328720702));
#46146=CARTESIAN_POINT('Ctrl Pts',(-19.4188153389072,16.4796045062356,-77.4853508948796));
#46147=CARTESIAN_POINT('Ctrl Pts',(-19.4188177230362,16.9160785638965,-78.3062334798541));
#46148=CARTESIAN_POINT('Ctrl Pts',(-19.4188177230362,17.3526001512859,-79.1272111819523));
#46149=CARTESIAN_POINT('Ctrl Pts',(-16.9146734095705,4.07920360686077,24.830633653217));
#46150=CARTESIAN_POINT('Ctrl Pts',(-16.9147239272192,4.07920356885915,24.78175430811));
#46151=CARTESIAN_POINT('Ctrl Pts',(-16.9147769162984,4.0792035341183,24.7328759880602));
#46152=CARTESIAN_POINT('Ctrl Pts',(-16.9154023366309,4.07920289336669,24.1822684761053));
#46153=CARTESIAN_POINT('Ctrl Pts',(-16.9158796858389,4.07920058846839,23.1781406679383));
#46154=CARTESIAN_POINT('Ctrl Pts',(-16.9169949468356,4.07919802534268,21.1695421788302));
#46155=CARTESIAN_POINT('Ctrl Pts',(-16.9211539003465,4.07919142487426,19.6654092661205));
#46156=CARTESIAN_POINT('Ctrl Pts',(-16.9299836755634,4.07918594088012,18.4143692135952));
#46157=CARTESIAN_POINT('Ctrl Pts',(-16.9342190088254,4.07918359559448,17.911552167174));
#46158=CARTESIAN_POINT('Ctrl Pts',(-16.944853731395,4.0791769820853,16.9075667994273));
#46159=CARTESIAN_POINT('Ctrl Pts',(-16.9676658429407,4.07916395102957,15.1537619834732));
#46160=CARTESIAN_POINT('Ctrl Pts',(-16.9893295738655,4.07914805388708,13.6520698339233));
#46161=CARTESIAN_POINT('Ctrl Pts',(-17.0029134267273,4.07914506892092,12.3976233718372));
#46162=CARTESIAN_POINT('Ctrl Pts',(-17.0084672384419,4.07914475479534,11.8966774963043));
#46163=CARTESIAN_POINT('Ctrl Pts',(-17.0197930215528,4.07914818539066,10.8948438791706));
#46164=CARTESIAN_POINT('Ctrl Pts',(-17.0337871110875,4.07914865402405,9.64235194184012));
#46165=CARTESIAN_POINT('Ctrl Pts',(-17.0485553653208,4.07915702810575,8.13790849406833));
#46166=CARTESIAN_POINT('Ctrl Pts',(-17.0558421657869,4.07915203742613,7.13321404971454));
#46167=CARTESIAN_POINT('Ctrl Pts',(-17.0592306979639,4.07915243507481,6.50537190516661));
#46168=CARTESIAN_POINT('Ctrl Pts',(-17.0608323426246,4.07937877383712,6.2580752164868));
#46169=CARTESIAN_POINT('Ctrl Pts',(-17.0648048542448,4.08056269253945,5.76013765874217));
#46170=CARTESIAN_POINT('Ctrl Pts',(-17.073138987226,4.08411724516116,4.88575206743614));
#46171=CARTESIAN_POINT('Ctrl Pts',(-17.0903689206984,4.09355139007925,3.12310947319482));
#46172=CARTESIAN_POINT('Ctrl Pts',(-17.0888209075592,4.09356162540644,1.59817064052181));
#46173=CARTESIAN_POINT('Ctrl Pts',(-17.0638392445282,4.07800224041429,0.517411790217176));
#46174=CARTESIAN_POINT('Ctrl Pts',(-17.0605983359294,4.07597591758405,0.387514432140873));
#46175=CARTESIAN_POINT('Ctrl Pts',(-17.0531021045699,4.07129525632049,0.129079376660313));
#46176=CARTESIAN_POINT('Ctrl Pts',(-17.0374966370187,4.0615425736139,-0.321907681662813));
#46177=CARTESIAN_POINT('Ctrl Pts',(-17.0090210424416,4.04369114790545,-0.961387761059511));
#46178=CARTESIAN_POINT('Ctrl Pts',(-16.9681086459772,4.01780806705043,-1.72194422763307));
#46179=CARTESIAN_POINT('Ctrl Pts',(-16.908583693265,3.97976448878331,-2.72744523146189));
#46180=CARTESIAN_POINT('Ctrl Pts',(-16.8327228434125,3.93040577419916,-3.96971456218046));
#46181=CARTESIAN_POINT('Ctrl Pts',(-16.7866766418018,3.90033598244312,-4.95111724077728));
#46182=CARTESIAN_POINT('Ctrl Pts',(-16.7675066186055,3.88833732536696,-5.56177000535768));
#46183=CARTESIAN_POINT('Ctrl Pts',(-16.7603205981865,3.88388173809189,-5.80991553107169));
#46184=CARTESIAN_POINT('Ctrl Pts',(-16.7477446490098,3.87636163463991,-6.3051397414101));
#46185=CARTESIAN_POINT('Ctrl Pts',(-16.7300208455842,3.86649997340302,-7.17503824389738));
#46186=CARTESIAN_POINT('Ctrl Pts',(-16.7146210384598,3.86009960228098,-8.42235446624796));
#46187=CARTESIAN_POINT('Ctrl Pts',(-16.7063299309972,3.85895696124205,-9.67406515743436));
#46188=CARTESIAN_POINT('Ctrl Pts',(-16.7010623786273,3.85823357875107,-10.5508147844575));
#46189=CARTESIAN_POINT('Ctrl Pts',(-16.6977378741451,3.85745234181625,-11.0518219182477));
#46190=CARTESIAN_POINT('Ctrl Pts',(-16.6958938377715,3.85687410082937,-11.3022954189243));
#46191=CARTESIAN_POINT('Ctrl Pts',(-16.6944082136604,3.85634386019955,-11.4908747518974));
#46192=CARTESIAN_POINT('Ctrl Pts',(-16.6934391066798,3.85601265813483,-11.6162364634123));
#46193=CARTESIAN_POINT('Ctrl Pts',(-16.6916127399259,3.85544149913119,-11.867480742801));
#46194=CARTESIAN_POINT('Ctrl Pts',(-16.6887003015182,3.85467069657949,-12.3062120146968));
#46195=CARTESIAN_POINT('Ctrl Pts',(-16.6839294279526,3.85394295505111,-13.1820737698753));
#46196=CARTESIAN_POINT('Ctrl Pts',(-16.6797255183182,3.8546942229523,-14.4300495819467));
#46197=CARTESIAN_POINT('Ctrl Pts',(-16.6780423749029,3.85617929848326,-15.5549559973584));
#46198=CARTESIAN_POINT('Ctrl Pts',(-16.6773678851618,3.8569475200662,-16.3077964022937));
#46199=CARTESIAN_POINT('Ctrl Pts',(-16.6770114378945,3.85736444136179,-16.8106178945354));
#46200=CARTESIAN_POINT('Ctrl Pts',(-16.6768069891574,3.8575226412861,-17.1889465823843));
#46201=CARTESIAN_POINT('Ctrl Pts',(-16.6766437114414,3.85752565497502,-17.5042654103635));
#46202=CARTESIAN_POINT('Ctrl Pts',(-16.6765941790477,3.85753490940607,-17.6286496634979));
#46203=CARTESIAN_POINT('Ctrl Pts',(-16.676553307684,3.85758249987073,-17.8778326479976));
#46204=CARTESIAN_POINT('Ctrl Pts',(-16.6765944303759,3.85766789456493,-18.1270789699173));
#46205=CARTESIAN_POINT('Ctrl Pts',(-16.6767149275073,3.85778279386269,-18.3765614210905));
#46206=CARTESIAN_POINT('Ctrl Pts',(-16.6768209495527,3.85786444593357,-18.5325500358368));
#46207=CARTESIAN_POINT('Ctrl Pts',(-16.6769240126647,3.85793466997555,-18.6573913142302));
#46208=CARTESIAN_POINT('Ctrl Pts',(-16.6770100315899,3.85798940704359,-18.7510439476394));
#46209=CARTESIAN_POINT('Ctrl Pts',(-16.6770888212736,3.85803649701773,-18.8291075849918));
#46210=CARTESIAN_POINT('Ctrl Pts',(-16.6771561255174,3.85807492954543,-18.8915698592054));
#46211=CARTESIAN_POINT('Ctrl Pts',(-16.6777514591514,3.85840532900616,-19.4225653497714));
#46212=CARTESIAN_POINT('Ctrl Pts',(-16.6795788425869,3.85912931741145,-20.4398404028269));
#46213=CARTESIAN_POINT('Ctrl Pts',(-16.6836451022944,3.8592636505166,-21.9487053700047));
#46214=CARTESIAN_POINT('Ctrl Pts',(-16.686670540002,3.85786544788114,-22.9593455552285));
#46215=CARTESIAN_POINT('Ctrl Pts',(-16.6885257593456,3.85628204344558,-23.5907847375866));
#46216=CARTESIAN_POINT('Ctrl Pts',(-16.6893050970785,3.85555855841181,-23.8410988560408));
#46217=CARTESIAN_POINT('Ctrl Pts',(-16.6910099656135,3.85377419173882,-24.3420261589137));
#46218=CARTESIAN_POINT('Ctrl Pts',(-16.6943343835605,3.84988498908126,-25.2199567032052));
#46219=CARTESIAN_POINT('Ctrl Pts',(-16.6997260151302,3.84281878110687,-26.4763414811346));
#46220=CARTESIAN_POINT('Ctrl Pts',(-16.7063745797174,3.83412124678864,-27.9837612304857));
#46221=CARTESIAN_POINT('Ctrl Pts',(-16.7102487178192,3.82957501937168,-28.9859581556077));
#46222=CARTESIAN_POINT('Ctrl Pts',(-16.7121190144433,3.82776231710041,-29.5483117409518));
#46223=CARTESIAN_POINT('Ctrl Pts',(-16.7124390843753,3.8272861697604,-29.6752367072504));
#46224=CARTESIAN_POINT('Ctrl Pts',(-16.7127211941321,3.82611062581586,-29.9277638206352));
#46225=CARTESIAN_POINT('Ctrl Pts',(-16.712372166923,3.82351988117654,-30.3697764617688));
#46226=CARTESIAN_POINT('Ctrl Pts',(-16.7090563975436,3.81676731864626,-31.2512803990046));
#46227=CARTESIAN_POINT('Ctrl Pts',(-16.7011820320115,3.80576715739035,-32.504239566492));
#46228=CARTESIAN_POINT('Ctrl Pts',(-16.7005638350862,3.80132834083306,-33.7463250851312));
#46229=CARTESIAN_POINT('Ctrl Pts',(-16.7112561468823,3.80667288732683,-34.7322118103997));
#46230=CARTESIAN_POINT('Ctrl Pts',(-16.7214848608452,3.81311635167405,-35.2223970544754));
#46231=CARTESIAN_POINT('Ctrl Pts',(-16.731439234743,3.8196556960259,-35.5897483194025));
#46232=CARTESIAN_POINT('Ctrl Pts',(-16.7392623374465,3.82483202377554,-35.8335364392361));
#46233=CARTESIAN_POINT('Ctrl Pts',(-16.7589744320517,3.83802309018381,-36.3235593738663));
#46234=CARTESIAN_POINT('Ctrl Pts',(-16.8026965129352,3.86750392921385,-37.1835674124926));
#46235=CARTESIAN_POINT('Ctrl Pts',(-16.9147604342526,3.94311926201518,-38.9174593726877));
#46236=CARTESIAN_POINT('Ctrl Pts',(-17.0108408419884,4.00831363951242,-40.4386822878126));
#46237=CARTESIAN_POINT('Ctrl Pts',(-17.0428387141216,4.03597245536776,-41.7311804966786));
#46238=CARTESIAN_POINT('Ctrl Pts',(-17.0502703194235,4.0401683438514,-42.1300884229979));
#46239=CARTESIAN_POINT('Ctrl Pts',(-17.0566388284558,4.03976300543393,-42.6475183153195));
#46240=CARTESIAN_POINT('Ctrl Pts',(-17.0608900330414,4.03653857718181,-43.1624867273373));
#46241=CARTESIAN_POINT('Ctrl Pts',(-17.0626425437171,4.02893033341949,-43.7968719369589));
#46242=CARTESIAN_POINT('Ctrl Pts',(-17.0604043454077,4.01967372408898,-44.5446528351534));
#46243=CARTESIAN_POINT('Ctrl Pts',(-17.0560465675541,4.01620165395783,-45.1555878484918));
#46244=CARTESIAN_POINT('Ctrl Pts',(-17.0516948081744,4.0183894712776,-45.6366450360375));
#46245=CARTESIAN_POINT('Ctrl Pts',(-17.0481868260204,4.02311208554269,-45.9936189369653));
#46246=CARTESIAN_POINT('Ctrl Pts',(-17.0446004597252,4.03148077372419,-46.3466764435411));
#46247=CARTESIAN_POINT('Ctrl Pts',(-17.0399245092123,4.04822086533075,-46.8121131557728));
#46248=CARTESIAN_POINT('Ctrl Pts',(-17.0368366978271,4.06787393045612,-47.1551568300095));
#46249=CARTESIAN_POINT('Ctrl Pts',(-17.0343068286104,4.09333570883227,-47.4953825531079));
#46250=CARTESIAN_POINT('Ctrl Pts',(-17.0323684226327,4.11260883491083,-47.7444525481771));
#46251=CARTESIAN_POINT('Ctrl Pts',(-17.027621205699,4.15295468238058,-48.2288090773729));
#46252=CARTESIAN_POINT('Ctrl Pts',(-17.017323823215,4.23179762527297,-49.0783707505405));
#46253=CARTESIAN_POINT('Ctrl Pts',(-16.9986226932743,4.37015641608352,-50.2759118463673));
#46254=CARTESIAN_POINT('Ctrl Pts',(-16.974839604241,4.58949006108651,-51.6943299428451));
#46255=CARTESIAN_POINT('Ctrl Pts',(-16.9615417398334,4.77851385430702,-52.6257397035579));
#46256=CARTESIAN_POINT('Ctrl Pts',(-16.954964164518,4.91266531028849,-53.2053103446949));
#46257=CARTESIAN_POINT('Ctrl Pts',(-16.9523001823878,4.96899968854369,-53.4420760996642));
#46258=CARTESIAN_POINT('Ctrl Pts',(-16.9470116768378,5.08761857516938,-53.9153594023399));
#46259=CARTESIAN_POINT('Ctrl Pts',(-16.9379222492454,5.31147588450487,-54.7470295920851));
#46260=CARTESIAN_POINT('Ctrl Pts',(-16.920927864664,5.82039604793575,-56.4168686594285));
#46261=CARTESIAN_POINT('Ctrl Pts',(-16.9102911907989,6.35114099148479,-57.8500060872888));
#46262=CARTESIAN_POINT('Ctrl Pts',(-16.9065358465525,6.76139515416387,-58.8561565137549));
#46263=CARTESIAN_POINT('Ctrl Pts',(-16.9061445217287,6.80895991225671,-58.9713364239509));
#46264=CARTESIAN_POINT('Ctrl Pts',(-16.90550255376,6.90851827002603,-59.2069006559096));
#46265=CARTESIAN_POINT('Ctrl Pts',(-16.9047646267965,7.08881899845472,-59.6197202484487));
#46266=CARTESIAN_POINT('Ctrl Pts',(-16.9046305846275,7.47557253268014,-60.4566671436843));
#46267=CARTESIAN_POINT('Ctrl Pts',(-16.9067386267066,7.96483632081048,-61.4297876094401));
#46268=CARTESIAN_POINT('Ctrl Pts',(-16.9096057624689,8.47990584339476,-62.4143366719387));
#46269=CARTESIAN_POINT('Ctrl Pts',(-16.911225990679,8.77492881447765,-62.9713548920425));
#46270=CARTESIAN_POINT('Ctrl Pts',(-16.9121898023996,8.97207021405464,-63.3438190469933));
#46271=CARTESIAN_POINT('Ctrl Pts',(-16.912794811064,9.1035031542903,-63.5924195313673));
#46272=CARTESIAN_POINT('Ctrl Pts',(-16.9133261407537,9.23473080571758,-63.8413848735041));
#46273=CARTESIAN_POINT('Ctrl Pts',(-16.9137109132029,9.34910125829025,-64.0595880294941));
#46274=CARTESIAN_POINT('Ctrl Pts',(-16.9139041360755,9.41427802137335,-64.1843721158538));
#46275=CARTESIAN_POINT('Ctrl Pts',(-16.9141661003506,9.5118369834402,-64.3716318601805));
#46276=CARTESIAN_POINT('Ctrl Pts',(-16.9143206201335,9.59267662726585,-64.5278947897286));
#46277=CARTESIAN_POINT('Ctrl Pts',(-16.9144796684479,9.72551688476094,-64.786600053596));
#46278=CARTESIAN_POINT('Ctrl Pts',(-16.9146214511875,9.85505637385379,-65.0377894321718));
#46279=CARTESIAN_POINT('Ctrl Pts',(-16.914834479387,10.1189220825822,-65.545521407322));
#46280=CARTESIAN_POINT('Ctrl Pts',(-16.9150312999542,10.5793317586482,-66.4220661365077));
#46281=CARTESIAN_POINT('Ctrl Pts',(-16.914926439779,11.5060543253365,-68.1576437448239));
#46282=CARTESIAN_POINT('Ctrl Pts',(-16.9144808086033,12.3066091050813,-69.6367687451921));
#46283=CARTESIAN_POINT('Ctrl Pts',(-16.914488061616,12.9107783194121,-70.7731245831863));
#46284=CARTESIAN_POINT('Ctrl Pts',(-16.9144905361333,13.0439496335314,-71.0235966846109));
#46285=CARTESIAN_POINT('Ctrl Pts',(-16.9144939206435,13.3110413128027,-71.5259434402883));
#46286=CARTESIAN_POINT('Ctrl Pts',(-16.9144943255004,13.6443733781517,-72.1528660310182));
#46287=CARTESIAN_POINT('Ctrl Pts',(-16.9144936325431,14.0443864387566,-72.9051840662007));
#46288=CARTESIAN_POINT('Ctrl Pts',(-16.9144883889213,14.8440237580498,-74.4090689669014));
#46289=CARTESIAN_POINT('Ctrl Pts',(-16.9144733780915,15.5099868122522,-75.661536888092));
#46290=CARTESIAN_POINT('Ctrl Pts',(-16.9144688934797,16.4797239446511,-77.485353891126));
#46291=CARTESIAN_POINT('Ctrl Pts',(-16.9144665841287,16.9161914735935,-78.3062333820799));
#46292=CARTESIAN_POINT('Ctrl Pts',(-16.9144665841287,17.3527130609829,-79.1272110841781));
#46293=CARTESIAN_POINT('Ctrl Pts',(-15.0355537871551,4.07980364542041,24.8306344346923));
#46294=CARTESIAN_POINT('Ctrl Pts',(-15.0355987159917,4.0798036226416,24.7817551132038));
#46295=CARTESIAN_POINT('Ctrl Pts',(-15.0356458337054,4.07980358298019,24.732876760882));
#46296=CARTESIAN_POINT('Ctrl Pts',(-15.0362023699372,4.07980383215307,24.1822714211911));
#46297=CARTESIAN_POINT('Ctrl Pts',(-15.0366296099556,4.07980792182674,23.1781597882922));
#46298=CARTESIAN_POINT('Ctrl Pts',(-15.0376222054118,4.07980751034299,21.1695635006398));
#46299=CARTESIAN_POINT('Ctrl Pts',(-15.0413273538726,4.07981667851586,19.6654699357026));
#46300=CARTESIAN_POINT('Ctrl Pts',(-15.0491822708977,4.07981816742211,18.4144469747709));
#46301=CARTESIAN_POINT('Ctrl Pts',(-15.0529491711425,4.07981724239166,17.9116339513916));
#46302=CARTESIAN_POINT('Ctrl Pts',(-15.0624084365526,4.0798161087169,16.907660694229));
#46303=CARTESIAN_POINT('Ctrl Pts',(-15.0826972523316,4.07981019820557,15.1538675175825));
#46304=CARTESIAN_POINT('Ctrl Pts',(-15.1019756384676,4.07982792821452,13.6522604636661));
#46305=CARTESIAN_POINT('Ctrl Pts',(-15.1140599265239,4.07983658797161,12.3978501330781));
#46306=CARTESIAN_POINT('Ctrl Pts',(-15.118999927868,4.07983948633581,11.8969137604361));
#46307=CARTESIAN_POINT('Ctrl Pts',(-15.1290699569862,4.07983945762267,10.8950887987764));
#46308=CARTESIAN_POINT('Ctrl Pts',(-15.1415231892606,4.07986321498447,9.64266293595803));
#46309=CARTESIAN_POINT('Ctrl Pts',(-15.1546563515223,4.0798728821423,8.13830711977429));
#46310=CARTESIAN_POINT('Ctrl Pts',(-15.1611533789286,4.07991162203139,7.13365716272063));
#46311=CARTESIAN_POINT('Ctrl Pts',(-15.1641703541679,4.07992053271181,6.50603943843838));
#46312=CARTESIAN_POINT('Ctrl Pts',(-15.1658166076348,4.08049707291913,6.26337464950295));
#46313=CARTESIAN_POINT('Ctrl Pts',(-15.1705110079943,4.0835139590614,5.77045446573432));
#46314=CARTESIAN_POINT('Ctrl Pts',(-15.1814161643698,4.09267154088208,4.90241598307794));
#46315=CARTESIAN_POINT('Ctrl Pts',(-15.2060220994827,4.11704547635916,3.13599603857746));
#46316=CARTESIAN_POINT('Ctrl Pts',(-15.2047643807156,4.11788885254558,1.58241888815762));
#46317=CARTESIAN_POINT('Ctrl Pts',(-15.1675668382405,4.0764560708923,0.467940949357721));
#46318=CARTESIAN_POINT('Ctrl Pts',(-15.1627329495942,4.07095125001953,0.332095056170709));
#46319=CARTESIAN_POINT('Ctrl Pts',(-15.1515618273976,4.05832775712855,0.0636346843564117));
#46320=CARTESIAN_POINT('Ctrl Pts',(-15.1283184960179,4.03207150092787,-0.403681010059032));
#46321=CARTESIAN_POINT('Ctrl Pts',(-15.0860236033019,3.9844390875535,-1.06091900375415));
#46322=CARTESIAN_POINT('Ctrl Pts',(-15.0253548820853,3.91589806628914,-1.83452126081223));
#46323=CARTESIAN_POINT('Ctrl Pts',(-14.9374539251796,3.81626383930631,-2.84620724666584));
#46324=CARTESIAN_POINT('Ctrl Pts',(-14.8260214252139,3.68880024344429,-4.07548581332824));
#46325=CARTESIAN_POINT('Ctrl Pts',(-14.7594363908475,3.61301318315625,-5.02518833160673));
#46326=CARTESIAN_POINT('Ctrl Pts',(-14.732296786269,3.58308427120848,-5.60980532717593));
#46327=CARTESIAN_POINT('Ctrl Pts',(-14.7222950121233,3.57175513847179,-5.85331734149995));
#46328=CARTESIAN_POINT('Ctrl Pts',(-14.7051522824233,3.55288734903858,-6.3372651837452));
#46329=CARTESIAN_POINT('Ctrl Pts',(-14.6820755031784,3.52849851665087,-7.19188587500867));
#46330=CARTESIAN_POINT('Ctrl Pts',(-14.6648046124832,3.51403102114489,-8.42435063298136));
#46331=CARTESIAN_POINT('Ctrl Pts',(-14.6581099236016,3.51313576173022,-9.67204027371791));
#46332=CARTESIAN_POINT('Ctrl Pts',(-14.6536278741172,3.51217596509686,-10.5512063673995));
#46333=CARTESIAN_POINT('Ctrl Pts',(-14.6503694622625,3.51044997141002,-11.0551883304677));
#46334=CARTESIAN_POINT('Ctrl Pts',(-14.6483819555578,3.50901243037069,-11.3076840335205));
#46335=CARTESIAN_POINT('Ctrl Pts',(-14.6467027667886,3.50764329676335,-11.4979269040331));
#46336=CARTESIAN_POINT('Ctrl Pts',(-14.6456093912494,3.50678869858926,-11.6223550640012));
#46337=CARTESIAN_POINT('Ctrl Pts',(-14.6435757682735,3.50526761061104,-11.8729327016961));
#46338=CARTESIAN_POINT('Ctrl Pts',(-14.6403980129151,3.50310280032409,-12.3100266747562));
#46339=CARTESIAN_POINT('Ctrl Pts',(-14.6354559223704,3.50055398087762,-13.1834847279314));
#46340=CARTESIAN_POINT('Ctrl Pts',(-14.6317533744831,3.50086511785969,-14.4290661100897));
#46341=CARTESIAN_POINT('Ctrl Pts',(-14.6308576624301,3.50318988050142,-15.5534808436544));
#46342=CARTESIAN_POINT('Ctrl Pts',(-14.6306099354699,3.50445651101314,-16.3066179862937));
#46343=CARTESIAN_POINT('Ctrl Pts',(-14.6304928384944,3.50514632219001,-16.8098153537103));
#46344=CARTESIAN_POINT('Ctrl Pts',(-14.6304146638658,3.50541618468216,-17.1886154981013));
#46345=CARTESIAN_POINT('Ctrl Pts',(-14.6302952156756,3.50539935393863,-17.5044281144483));
#46346=CARTESIAN_POINT('Ctrl Pts',(-14.6302612721091,3.50539702227164,-17.6288670554403));
#46347=CARTESIAN_POINT('Ctrl Pts',(-14.6302453022539,3.50540897852697,-17.8782159379193));
#46348=CARTESIAN_POINT('Ctrl Pts',(-14.6303068483174,3.50544687608919,-18.127563739392));
#46349=CARTESIAN_POINT('Ctrl Pts',(-14.6304382209476,3.50550318977588,-18.377130410457));
#46350=CARTESIAN_POINT('Ctrl Pts',(-14.6305494440017,3.50554667481252,-18.5331538178356));
#46351=CARTESIAN_POINT('Ctrl Pts',(-14.6306547530545,3.50558531974963,-18.6580160550547));
#46352=CARTESIAN_POINT('Ctrl Pts',(-14.6307419615824,3.50561638167107,-18.7516798291178));
#46353=CARTESIAN_POINT('Ctrl Pts',(-14.6308213744854,3.50564391289322,-18.8297493429282));
#46354=CARTESIAN_POINT('Ctrl Pts',(-14.6308887686871,3.50566675064361,-18.8922142432608));
#46355=CARTESIAN_POINT('Ctrl Pts',(-14.6314838374563,3.50586612291774,-19.423219916044));
#46356=CARTESIAN_POINT('Ctrl Pts',(-14.6333692311182,3.50645317370486,-20.4401021876619));
#46357=CARTESIAN_POINT('Ctrl Pts',(-14.637476383763,3.50727050936296,-21.9473554866998));
#46358=CARTESIAN_POINT('Ctrl Pts',(-14.640808196621,3.50759270313843,-22.9561906327422));
#46359=CARTESIAN_POINT('Ctrl Pts',(-14.6428984515547,3.50759068760652,-23.5862944233562));
#46360=CARTESIAN_POINT('Ctrl Pts',(-14.643776352525,3.5075725191586,-23.8358209976824));
#46361=CARTESIAN_POINT('Ctrl Pts',(-14.6457331369259,3.50748751849172,-24.3355293750873));
#46362=CARTESIAN_POINT('Ctrl Pts',(-14.6496020318851,3.50721605211125,-25.2117220717688));
#46363=CARTESIAN_POINT('Ctrl Pts',(-14.656062504619,3.50660548397868,-26.4670089019858));
#46364=CARTESIAN_POINT('Ctrl Pts',(-14.6638903330453,3.50569606625201,-27.9752590018877));
#46365=CARTESIAN_POINT('Ctrl Pts',(-14.6683851504733,3.50527204895064,-28.9793144013429));
#46366=CARTESIAN_POINT('Ctrl Pts',(-14.6704277006154,3.50512795918196,-29.5433007449167));
#46367=CARTESIAN_POINT('Ctrl Pts',(-14.6707365850827,3.50490718889653,-29.6726937137558));
#46368=CARTESIAN_POINT('Ctrl Pts',(-14.6708316651918,3.50381704401876,-29.9285479609433));
#46369=CARTESIAN_POINT('Ctrl Pts',(-14.669766140098,3.50037881001467,-30.3760195620317));
#46370=CARTESIAN_POINT('Ctrl Pts',(-14.6637912291401,3.48885467862556,-31.2640688745989));
#46371=CARTESIAN_POINT('Ctrl Pts',(-14.6505638037055,3.46726542975816,-32.5155080392028));
#46372=CARTESIAN_POINT('Ctrl Pts',(-14.6478928861451,3.46031026411328,-33.7412400276083));
#46373=CARTESIAN_POINT('Ctrl Pts',(-14.6622999885151,3.47585215242021,-34.7050909198485));
#46374=CARTESIAN_POINT('Ctrl Pts',(-14.6767699741126,3.4925415200364,-35.1811795603407));
#46375=CARTESIAN_POINT('Ctrl Pts',(-14.6910527445473,3.5091074255739,-35.5366216765077));
#46376=CARTESIAN_POINT('Ctrl Pts',(-14.7023761429481,3.5219724789133,-35.7685022859579));
#46377=CARTESIAN_POINT('Ctrl Pts',(-14.730937498059,3.55480412742927,-36.2400471584948));
#46378=CARTESIAN_POINT('Ctrl Pts',(-14.7942510401053,3.62778769933195,-37.0735872305291));
#46379=CARTESIAN_POINT('Ctrl Pts',(-14.9567147007777,3.81530290395057,-38.7854056166029));
#46380=CARTESIAN_POINT('Ctrl Pts',(-15.0959365109023,3.97608959573285,-40.3405038655363));
#46381=CARTESIAN_POINT('Ctrl Pts',(-15.143164900117,4.03760057498106,-41.6917264284665));
#46382=CARTESIAN_POINT('Ctrl Pts',(-15.1542138680894,4.04952544452372,-42.0977073649019));
#46383=CARTESIAN_POINT('Ctrl Pts',(-15.1638448099992,4.05573631238654,-42.6272440819555));
#46384=CARTESIAN_POINT('Ctrl Pts',(-15.1704002909234,4.05695035430358,-43.1519747485755));
#46385=CARTESIAN_POINT('Ctrl Pts',(-15.1734737725596,4.05143422664606,-43.7967650097556));
#46386=CARTESIAN_POINT('Ctrl Pts',(-15.170994477228,4.04083420994993,-44.553127516674));
#46387=CARTESIAN_POINT('Ctrl Pts',(-15.1654680262509,4.03426710769119,-45.1683279110718));
#46388=CARTESIAN_POINT('Ctrl Pts',(-15.1600154170591,4.03353776034087,-45.6509597754355));
#46389=CARTESIAN_POINT('Ctrl Pts',(-15.1556442267631,4.03595897748892,-46.0082226248127));
#46390=CARTESIAN_POINT('Ctrl Pts',(-15.1512467507119,4.04205999799744,-46.3606502180971));
#46391=CARTESIAN_POINT('Ctrl Pts',(-15.1457005016869,4.05602078723531,-46.8240512717451));
#46392=CARTESIAN_POINT('Ctrl Pts',(-15.1422353107102,4.07396288140231,-47.1641699149808));
#46393=CARTESIAN_POINT('Ctrl Pts',(-15.139783459693,4.09827668768204,-47.5007304572948));
#46394=CARTESIAN_POINT('Ctrl Pts',(-15.1378420733016,4.11697806106922,-47.7531191415305));
#46395=CARTESIAN_POINT('Ctrl Pts',(-15.1328692251381,4.15525952282944,-48.2402312180556));
#46396=CARTESIAN_POINT('Ctrl Pts',(-15.1216753544551,4.22898695996459,-49.0948921174904));
#46397=CARTESIAN_POINT('Ctrl Pts',(-15.100570697442,4.35657973853331,-50.2945599673458));
#46398=CARTESIAN_POINT('Ctrl Pts',(-15.0740064986484,4.56209516926598,-51.7096344631151));
#46399=CARTESIAN_POINT('Ctrl Pts',(-15.0599764883946,4.74406573161041,-52.6344612450797));
#46400=CARTESIAN_POINT('Ctrl Pts',(-15.0537823319715,4.87549664531731,-53.208858641316));
#46401=CARTESIAN_POINT('Ctrl Pts',(-15.0513274604829,4.93110049792611,-53.444560390365));
#46402=CARTESIAN_POINT('Ctrl Pts',(-15.0466664614285,5.04865651751058,-53.9154426794593));
#46403=CARTESIAN_POINT('Ctrl Pts',(-15.0391166960127,5.2719822782236,-54.7438660195013));
#46404=CARTESIAN_POINT('Ctrl Pts',(-15.0265276021994,5.78405374259164,-56.409570029445));
#46405=CARTESIAN_POINT('Ctrl Pts',(-15.0201709336733,6.32184752352393,-57.8432803524839));
#46406=CARTESIAN_POINT('Ctrl Pts',(-15.0182848745529,6.73606148976995,-58.8513097528353));
#46407=CARTESIAN_POINT('Ctrl Pts',(-15.0181457177407,6.78388562980237,-58.9661899051116));
#46408=CARTESIAN_POINT('Ctrl Pts',(-15.0179891980911,6.88415653941591,-59.2014913298822));
#46409=CARTESIAN_POINT('Ctrl Pts',(-15.0181027948521,7.06579558906368,-59.6137866798083));
#46410=CARTESIAN_POINT('Ctrl Pts',(-15.0196034230197,7.45580435909341,-60.4501270204543));
#46411=CARTESIAN_POINT('Ctrl Pts',(-15.0234366830025,7.94966348909133,-61.4231487032632));
#46412=CARTESIAN_POINT('Ctrl Pts',(-15.0277521223662,8.46944302555454,-62.4082043767788));
#46413=CARTESIAN_POINT('Ctrl Pts',(-15.0300772962333,8.76701551587498,-62.9657228405259));
#46414=CARTESIAN_POINT('Ctrl Pts',(-15.0314650428341,8.96576570835786,-63.3386197971633));
#46415=CARTESIAN_POINT('Ctrl Pts',(-15.0323370111439,9.09823921246122,-63.5875349222999));
#46416=CARTESIAN_POINT('Ctrl Pts',(-15.0331248233671,9.2304705284566,-63.8368589352409));
#46417=CARTESIAN_POINT('Ctrl Pts',(-15.0337110597418,9.34566130836768,-64.0554130119618));
#46418=CARTESIAN_POINT('Ctrl Pts',(-15.0340144772916,9.41129110852897,-64.1804091802084));
#46419=CARTESIAN_POINT('Ctrl Pts',(-15.0344360007435,9.50951220481309,-64.3679984751364));
#46420=CARTESIAN_POINT('Ctrl Pts',(-15.0347177360903,9.59087461061657,-64.5245636207363));
#46421=CARTESIAN_POINT('Ctrl Pts',(-15.035067183854,9.72451684020435,-64.7838009731992));
#46422=CARTESIAN_POINT('Ctrl Pts',(-15.0353848133514,9.85473546692574,-65.0354253794396));
#46423=CARTESIAN_POINT('Ctrl Pts',(-15.0358612467763,10.1197277183049,-65.5439941961108));
#46424=CARTESIAN_POINT('Ctrl Pts',(-15.036335484482,10.5814515751937,-66.4217577653916));
#46425=CARTESIAN_POINT('Ctrl Pts',(-15.0361595669505,11.5086582574723,-68.1588609058033));
#46426=CARTESIAN_POINT('Ctrl Pts',(-15.0352657890704,12.3076050285516,-69.6376806593423));
#46427=CARTESIAN_POINT('Ctrl Pts',(-15.0353109350272,12.9112669501562,-70.7730023962225));
#46428=CARTESIAN_POINT('Ctrl Pts',(-15.035317222821,13.0444823135873,-71.0235484969299));
#46429=CARTESIAN_POINT('Ctrl Pts',(-15.0353274433012,13.3115672104804,-71.5258671392746));
#46430=CARTESIAN_POINT('Ctrl Pts',(-15.035336734874,13.6449287129749,-72.1528267593996));
#46431=CARTESIAN_POINT('Ctrl Pts',(-15.0353388634009,14.0449452184326,-72.9051457867444));
#46432=CARTESIAN_POINT('Ctrl Pts',(-15.0353334562094,14.8445920828781,-74.409051124372));
#46433=CARTESIAN_POINT('Ctrl Pts',(-15.0353264001462,15.5105658529013,-75.6615289922393));
#46434=CARTESIAN_POINT('Ctrl Pts',(-15.0353329405934,16.480312824235,-77.4853437224222));
#46435=CARTESIAN_POINT('Ctrl Pts',(-15.0353363076073,16.9167915016479,-78.3062334786655));
#46436=CARTESIAN_POINT('Ctrl Pts',(-15.0353363076072,17.3533130890374,-79.1272111807638));
#46437=CARTESIAN_POINT('Ctrl Pts',(-13.1557741379781,4.0803530524235,24.8306351545581));
#46438=CARTESIAN_POINT('Ctrl Pts',(-13.155813449685,4.08035305770157,24.7817558560973));
#46439=CARTESIAN_POINT('Ctrl Pts',(-13.1558546955356,4.08035307132234,24.7328774658928));
#46440=CARTESIAN_POINT('Ctrl Pts',(-13.1563410160438,4.08035286385746,24.1822744603286));
#46441=CARTESIAN_POINT('Ctrl Pts',(-13.1567093000387,4.0803508857895,23.1781803757718));
#46442=CARTESIAN_POINT('Ctrl Pts',(-13.1575765152318,4.08035147881019,21.1695864438393));
#46443=CARTESIAN_POINT('Ctrl Pts',(-13.1608052881424,4.08034627445879,19.6655358129393));
#46444=CARTESIAN_POINT('Ctrl Pts',(-13.1676736389584,4.08034350989803,18.414531537443));
#46445=CARTESIAN_POINT('Ctrl Pts',(-13.1709691910712,4.08034306295088,17.9117228044668));
#46446=CARTESIAN_POINT('Ctrl Pts',(-13.1792431927653,4.08034143992823,16.9077626620281));
#46447=CARTESIAN_POINT('Ctrl Pts',(-13.1969938389414,4.08033960128086,15.1539821060121));
#46448=CARTESIAN_POINT('Ctrl Pts',(-13.2138360265775,4.08032543633712,13.6524680930802));
#46449=CARTESIAN_POINT('Ctrl Pts',(-13.2244006454422,4.0803162635778,12.3980978193184));
#46450=CARTESIAN_POINT('Ctrl Pts',(-13.2287206857489,4.08031267404826,11.8971713269556));
#46451=CARTESIAN_POINT('Ctrl Pts',(-13.2375352633826,4.08030766451321,10.8953582505344));
#46452=CARTESIAN_POINT('Ctrl Pts',(-13.248411252422,4.08028902017245,9.64299864571605));
#46453=CARTESIAN_POINT('Ctrl Pts',(-13.2599009573185,4.08027574336008,8.13875529480386));
#46454=CARTESIAN_POINT('Ctrl Pts',(-13.2655477218758,4.0802526817982,7.13412346351715));
#46455=CARTESIAN_POINT('Ctrl Pts',(-13.2681799922693,4.0802448409878,6.50681185355107));
#46456=CARTESIAN_POINT('Ctrl Pts',(-13.2698019650851,4.08129294003242,6.27069253695577));
#46457=CARTESIAN_POINT('Ctrl Pts',(-13.274869162831,4.08682299769191,5.78485948929902));
#46458=CARTESIAN_POINT('Ctrl Pts',(-13.2872608605326,4.10369449867301,4.9257321017469));
#46459=CARTESIAN_POINT('Ctrl Pts',(-13.3164404286073,4.14919628450794,3.15395855145886));
#46460=CARTESIAN_POINT('Ctrl Pts',(-13.315061179104,4.15106871629214,1.55950246456322));
#46461=CARTESIAN_POINT('Ctrl Pts',(-13.270022580591,4.07031984608163,0.397516099160289));
#46462=CARTESIAN_POINT('Ctrl Pts',(-13.2641837990596,4.05942680369637,0.253300780986643));
#46463=CARTESIAN_POINT('Ctrl Pts',(-13.2506873468413,4.0346271829898,-0.0292291062131075));
#46464=CARTESIAN_POINT('Ctrl Pts',(-13.2226347076824,3.98323177920193,-0.519379279762533));
#46465=CARTESIAN_POINT('Ctrl Pts',(-13.1716378979934,3.8908084463512,-1.20123437706951));
#46466=CARTESIAN_POINT('Ctrl Pts',(-13.0989093337486,3.76003838001366,-1.99266219901469));
#46467=CARTESIAN_POINT('Ctrl Pts',(-12.9938191153109,3.57258968988866,-3.0124316173263));
#46468=CARTESIAN_POINT('Ctrl Pts',(-12.8614488653646,3.33863883231242,-4.22335814509426));
#46469=CARTESIAN_POINT('Ctrl Pts',(-12.7828099642305,3.20391268284202,-5.12908160087711));
#46470=CARTESIAN_POINT('Ctrl Pts',(-12.7511993924182,3.15155164599807,-5.67737368538212));
#46471=CARTESIAN_POINT('Ctrl Pts',(-12.7397758415395,3.13119206439564,-5.91439685386655));
#46472=CARTESIAN_POINT('Ctrl Pts',(-12.7203920322258,3.09763464973176,-6.38256542323508));
#46473=CARTESIAN_POINT('Ctrl Pts',(-12.695007138571,3.05430418906382,-7.2157590598277));
#46474=CARTESIAN_POINT('Ctrl Pts',(-12.6776718135492,3.02944506063389,-8.42731350929475));
#46475=CARTESIAN_POINT('Ctrl Pts',(-12.6727238131215,3.02933833013982,-9.66922524532342));
#46476=CARTESIAN_POINT('Ctrl Pts',(-12.6693075261318,3.02850998640237,-10.5517126348689));
#46477=CARTESIAN_POINT('Ctrl Pts',(-12.6664440131268,3.0257287217791,-11.059826352415));
#46478=CARTESIAN_POINT('Ctrl Pts',(-12.6645572626772,3.02322189370004,-11.3151362286705));
#46479=CARTESIAN_POINT('Ctrl Pts',(-12.6629101700705,3.02078100540286,-11.5076955248054));
#46480=CARTESIAN_POINT('Ctrl Pts',(-12.6618363318287,3.01928578080132,-11.6307891682924));
#46481=CARTESIAN_POINT('Ctrl Pts',(-12.6598686173034,3.01660753345846,-11.8803936099287));
#46482=CARTESIAN_POINT('Ctrl Pts',(-12.6568544052628,3.01279400055832,-12.3151264615418));
#46483=CARTESIAN_POINT('Ctrl Pts',(-12.6524002126988,3.00824205225206,-13.1851012690669));
#46484=CARTESIAN_POINT('Ctrl Pts',(-12.6497510856662,3.00868004220166,-14.4272726811341));
#46485=CARTESIAN_POINT('Ctrl Pts',(-12.6498267002527,3.01268518483088,-15.5510916707221));
#46486=CARTESIAN_POINT('Ctrl Pts',(-12.6500765443154,3.01488093698965,-16.3047646394304));
#46487=CARTESIAN_POINT('Ctrl Pts',(-12.6502466351578,3.01608794512074,-16.8085885957819));
#46488=CARTESIAN_POINT('Ctrl Pts',(-12.6502978693836,3.01654274968049,-17.1881348839868));
#46489=CARTESIAN_POINT('Ctrl Pts',(-12.650242819155,3.01651275050804,-17.5047195654652));
#46490=CARTESIAN_POINT('Ctrl Pts',(-12.6502371990516,3.01650268132953,-17.6291867393314));
#46491=CARTESIAN_POINT('Ctrl Pts',(-12.6502869006965,3.01648961217202,-17.878728330494));
#46492=CARTESIAN_POINT('Ctrl Pts',(-12.6504204710308,3.01648624162333,-18.1281731377591));
#46493=CARTESIAN_POINT('Ctrl Pts',(-12.6506330434434,3.01649653244229,-18.3778357309691));
#46494=CARTESIAN_POINT('Ctrl Pts',(-12.6507955528867,3.01650821404336,-18.5338973524979));
#46495=CARTESIAN_POINT('Ctrl Pts',(-12.6509428358872,3.01652123263419,-18.6587846325459));
#46496=CARTESIAN_POINT('Ctrl Pts',(-12.6510614160913,3.01653275679845,-18.7524622004311));
#46497=CARTESIAN_POINT('Ctrl Pts',(-12.6511667650687,3.01654387489522,-18.8305399070751));
#46498=CARTESIAN_POINT('Ctrl Pts',(-12.6512549082132,3.01655373743753,-18.893009216131));
#46499=CARTESIAN_POINT('Ctrl Pts',(-12.6520247925854,3.01664273458606,-19.4240399806288));
#46500=CARTESIAN_POINT('Ctrl Pts',(-12.6541237713984,3.01697758963585,-20.4405711730087));
#46501=CARTESIAN_POINT('Ctrl Pts',(-12.6579294211245,3.01815475287891,-21.9462443601063));
#46502=CARTESIAN_POINT('Ctrl Pts',(-12.6601102583778,3.01950882106249,-22.9533052565657));
#46503=CARTESIAN_POINT('Ctrl Pts',(-12.6611267318529,3.0205721594055,-23.5820735238017));
#46504=CARTESIAN_POINT('Ctrl Pts',(-12.6615286489473,3.021036564125,-23.8308286121961));
#46505=CARTESIAN_POINT('Ctrl Pts',(-12.6623261605263,3.02212153715255,-24.3293299145022));
#46506=CARTESIAN_POINT('Ctrl Pts',(-12.6637013086328,3.0243729156782,-25.2038048961164));
#46507=CARTESIAN_POINT('Ctrl Pts',(-12.6656051280685,3.0282974288727,-26.4579245903748));
#46508=CARTESIAN_POINT('Ctrl Pts',(-12.6677582628302,3.03312831756597,-27.966944419098));
#46509=CARTESIAN_POINT('Ctrl Pts',(-12.6691030075266,3.03577301881281,-28.9727051263296));
#46510=CARTESIAN_POINT('Ctrl Pts',(-12.6698168999596,3.03689787633675,-29.538357854649));
#46511=CARTESIAN_POINT('Ctrl Pts',(-12.6698132891089,3.03681104734995,-29.6711654578784));
#46512=CARTESIAN_POINT('Ctrl Pts',(-12.6692264069125,3.0353901770263,-29.9315464351366));
#46513=CARTESIAN_POINT('Ctrl Pts',(-12.6668345501107,3.03000301729997,-30.3864535953205));
#46514=CARTESIAN_POINT('Ctrl Pts',(-12.6578010215643,3.01039128155299,-31.2832523688234));
#46515=CARTESIAN_POINT('Ctrl Pts',(-12.6400066653409,2.97271146032919,-32.5320185755455));
#46516=CARTESIAN_POINT('Ctrl Pts',(-12.634845042572,2.96155909789071,-33.7345365602532));
#46517=CARTESIAN_POINT('Ctrl Pts',(-12.6501589419524,2.99012090783457,-34.6675071863071));
#46518=CARTESIAN_POINT('Ctrl Pts',(-12.6664685503625,3.02013697144729,-35.1238909076441));
#46519=CARTESIAN_POINT('Ctrl Pts',(-12.6827882943889,3.049667945086,-35.4627784713065));
#46520=CARTESIAN_POINT('Ctrl Pts',(-12.6958962012237,3.07215903548757,-35.6781859331147));
#46521=CARTESIAN_POINT('Ctrl Pts',(-12.7289805976222,3.13026629146692,-36.1242333697363));
#46522=CARTESIAN_POINT('Ctrl Pts',(-12.8028819866128,3.26100972646761,-36.9212545038253));
#46523=CARTESIAN_POINT('Ctrl Pts',(-12.9933548010237,3.60308348033867,-38.6016123397764));
#46524=CARTESIAN_POINT('Ctrl Pts',(-13.1613535575174,3.91182696291085,-40.201227918605));
#46525=CARTESIAN_POINT('Ctrl Pts',(-13.2211242393456,4.0282859866978,-41.6340139791982));
#46526=CARTESIAN_POINT('Ctrl Pts',(-13.2353144482749,4.05210923693267,-42.049869291881));
#46527=CARTESIAN_POINT('Ctrl Pts',(-13.2481818620755,4.06877955506982,-42.5962981492808));
#46528=CARTESIAN_POINT('Ctrl Pts',(-13.2574554867026,4.07711819302276,-43.1346449505987));
#46529=CARTESIAN_POINT('Ctrl Pts',(-13.2630683506023,4.0753602797487,-43.7938911993317));
#46530=CARTESIAN_POINT('Ctrl Pts',(-13.2627669354662,4.06365334098689,-44.5620551546818));
#46531=CARTESIAN_POINT('Ctrl Pts',(-13.2587465444613,4.05346862938487,-45.182994918791));
#46532=CARTESIAN_POINT('Ctrl Pts',(-13.2544578172475,4.04912257365654,-45.6676124144258));
#46533=CARTESIAN_POINT('Ctrl Pts',(-13.2510435147074,4.0487418057528,-46.0251003309895));
#46534=CARTESIAN_POINT('Ctrl Pts',(-13.2477397541082,4.05214987408337,-46.3764502468696));
#46535=CARTESIAN_POINT('Ctrl Pts',(-13.2438843323439,4.06288446089586,-46.8367149905799));
#46536=CARTESIAN_POINT('Ctrl Pts',(-13.2421308030081,4.07915836117823,-47.1724957266347));
#46537=CARTESIAN_POINT('Ctrl Pts',(-13.2417038676613,4.10249590966452,-47.5036559955688));
#46538=CARTESIAN_POINT('Ctrl Pts',(-13.2412069334258,4.12079522222734,-47.7601351750562));
#46539=CARTESIAN_POINT('Ctrl Pts',(-13.2394376932609,4.15718998577154,-48.2503877348323));
#46540=CARTESIAN_POINT('Ctrl Pts',(-13.2345417506537,4.22597034088981,-49.1111956569178));
#46541=CARTESIAN_POINT('Ctrl Pts',(-13.2236926141566,4.34316506975111,-50.3137302436462));
#46542=CARTESIAN_POINT('Ctrl Pts',(-13.2084156954445,4.53571596044538,-51.7255112759695));
#46543=CARTESIAN_POINT('Ctrl Pts',(-13.1995064977252,4.71143017567789,-52.6432201079995));
#46544=CARTESIAN_POINT('Ctrl Pts',(-13.1950938359785,4.84036713241892,-53.2119901498542));
#46545=CARTESIAN_POINT('Ctrl Pts',(-13.1932531878942,4.89533619012327,-53.446669547819));
#46546=CARTESIAN_POINT('Ctrl Pts',(-13.1894471040342,5.01193375313325,-53.9151122049486));
#46547=CARTESIAN_POINT('Ctrl Pts',(-13.18252847065,5.2347879202242,-54.7403346482864));
#46548=CARTESIAN_POINT('Ctrl Pts',(-13.1683828939882,5.74963013160343,-56.4019610873787));
#46549=CARTESIAN_POINT('Ctrl Pts',(-13.1582582282907,6.29384249941408,-57.8364241727682));
#46550=CARTESIAN_POINT('Ctrl Pts',(-13.154613161905,6.71177253080708,-58.8463268050262));
#46551=CARTESIAN_POINT('Ctrl Pts',(-13.1542220352886,6.75981670567772,-58.9609073836496));
#46552=CARTESIAN_POINT('Ctrl Pts',(-13.1535344633131,6.86072859200631,-59.1959507798566));
#46553=CARTESIAN_POINT('Ctrl Pts',(-13.1526023913756,7.04356752142575,-59.6077438258746));
#46554=CARTESIAN_POINT('Ctrl Pts',(-13.1516823831064,7.43658361850669,-60.4435582936179));
#46555=CARTESIAN_POINT('Ctrl Pts',(-13.1522569428826,7.93476027138594,-61.4165822262003));
#46556=CARTESIAN_POINT('Ctrl Pts',(-13.1534691360712,8.45913900066764,-62.402197109673));
#46557=CARTESIAN_POINT('Ctrl Pts',(-13.1542076397542,8.75925507630414,-62.9602249755118));
#46558=CARTESIAN_POINT('Ctrl Pts',(-13.15464405715,8.95962476308872,-63.3335566079143));
#46559=CARTESIAN_POINT('Ctrl Pts',(-13.1549160091587,9.09315589969736,-63.5827869386175));
#46560=CARTESIAN_POINT('Ctrl Pts',(-13.1551470658275,9.22639420779388,-63.8324666552708));
#46561=CARTESIAN_POINT('Ctrl Pts',(-13.1553038367501,9.34242301433713,-64.0513705625043));
#46562=CARTESIAN_POINT('Ctrl Pts',(-13.1553778405755,9.40851629243358,-64.1765783028481));
#46563=CARTESIAN_POINT('Ctrl Pts',(-13.1554724963636,9.50741702443271,-64.3644968293088));
#46564=CARTESIAN_POINT('Ctrl Pts',(-13.1555131491166,9.58930603781651,-64.5213614335515));
#46565=CARTESIAN_POINT('Ctrl Pts',(-13.155522246675,9.72376824731968,-64.7811308655079));
#46566=CARTESIAN_POINT('Ctrl Pts',(-13.1555299564657,9.85467392491661,-65.0331856010803));
#46567=CARTESIAN_POINT('Ctrl Pts',(-13.1555456366966,10.1208173755968,-65.5425902208122));
#46568=CARTESIAN_POINT('Ctrl Pts',(-13.1555658222632,10.5838519520742,-66.4215649205693));
#46569=CARTESIAN_POINT('Ctrl Pts',(-13.1556095707056,11.5115232537443,-68.1602044429875));
#46570=CARTESIAN_POINT('Ctrl Pts',(-13.155630456193,12.3087055590539,-69.6386566768396));
#46571=CARTESIAN_POINT('Ctrl Pts',(-13.1556403819816,12.9118168263674,-70.7729135669995));
#46572=CARTESIAN_POINT('Ctrl Pts',(-13.1556432693842,13.045079585473,-71.02353707039));
#46573=CARTESIAN_POINT('Ctrl Pts',(-13.1556472608338,13.3121586661121,-71.5258293803497));
#46574=CARTESIAN_POINT('Ctrl Pts',(-13.1556485304927,13.6455411657879,-72.1528256372706));
#46575=CARTESIAN_POINT('Ctrl Pts',(-13.1556480993221,14.0455574812149,-72.9051471364947));
#46576=CARTESIAN_POINT('Ctrl Pts',(-13.1556428636615,14.8452036750472,-74.4090743177834));
#46577=CARTESIAN_POINT('Ctrl Pts',(-13.1556286022721,15.5111376687713,-75.6615429776088));
#46578=CARTESIAN_POINT('Ctrl Pts',(-13.1556251422331,16.4808633570863,-77.4853364516287));
#46579=CARTESIAN_POINT('Ctrl Pts',(-13.1556233624458,16.917340718603,-78.306233401254));
#46580=CARTESIAN_POINT('Ctrl Pts',(-13.1556233624458,17.3538623059925,-79.1272111033524));
#46581=CARTESIAN_POINT('Ctrl Pts',(-10.6492819238592,4.08038167169719,24.8306351998132));
#46582=CARTESIAN_POINT('Ctrl Pts',(-10.6493137195392,4.08038168982262,24.7817559021637));
#46583=CARTESIAN_POINT('Ctrl Pts',(-10.6493470556338,4.08038166878299,24.7328773938009));
#46584=CARTESIAN_POINT('Ctrl Pts',(-10.6497412032544,4.08038324018666,24.1822784019949));
#46585=CARTESIAN_POINT('Ctrl Pts',(-10.6500453740232,4.0803948996082,23.1782177160824));
#46586=CARTESIAN_POINT('Ctrl Pts',(-10.6507462455772,4.08039723979176,21.1696274351929));
#46587=CARTESIAN_POINT('Ctrl Pts',(-10.6533744236306,4.08042667579571,19.6656599209132));
#46588=CARTESIAN_POINT('Ctrl Pts',(-10.6589390571556,4.0804407818347,18.4146918653329));
#46589=CARTESIAN_POINT('Ctrl Pts',(-10.6616065234231,4.08044366935237,17.9118887952537));
#46590=CARTESIAN_POINT('Ctrl Pts',(-10.6683052245384,4.08045433741086,16.9079522161296));
#46591=CARTESIAN_POINT('Ctrl Pts',(-10.6826712896214,4.08046841990858,15.1541963112138));
#46592=CARTESIAN_POINT('Ctrl Pts',(-10.6963377737673,4.08053651180721,13.6528713310165));
#46593=CARTESIAN_POINT('Ctrl Pts',(-10.7049088628403,4.08056603843003,12.3985897102618));
#46594=CARTESIAN_POINT('Ctrl Pts',(-10.7084129630787,4.08057570316825,11.8976881183865));
#46595=CARTESIAN_POINT('Ctrl Pts',(-10.7155548414695,4.08057795085157,10.8959012527467));
#46596=CARTESIAN_POINT('Ctrl Pts',(-10.7244027862711,4.08063665394617,9.64368478691638));
#46597=CARTESIAN_POINT('Ctrl Pts',(-10.7337288856492,4.08065595706751,8.13963068459924));
#46598=CARTESIAN_POINT('Ctrl Pts',(-10.7383620587042,4.08074986366022,7.13507936017797));
#46599=CARTESIAN_POINT('Ctrl Pts',(-10.7405096838567,4.08076913956257,6.50825519786931));
#46600=CARTESIAN_POINT('Ctrl Pts',(-10.741909153158,4.08252227758183,6.28231854453814));
#46601=CARTESIAN_POINT('Ctrl Pts',(-10.746456212477,4.09181511766032,5.80751570745706));
#46602=CARTESIAN_POINT('Ctrl Pts',(-10.7578124704736,4.12054662565677,4.96219824056498));
#46603=CARTESIAN_POINT('Ctrl Pts',(-10.784998696866,4.19944237288572,3.18240041367406));
#46604=CARTESIAN_POINT('Ctrl Pts',(-10.7841087575516,4.20563462630991,1.52424222051406));
#46605=CARTESIAN_POINT('Ctrl Pts',(-10.7423817296544,4.05827404435424,0.290146045282327));
#46606=CARTESIAN_POINT('Ctrl Pts',(-10.7369639268377,4.03787106784976,0.13323147767058));
#46607=CARTESIAN_POINT('Ctrl Pts',(-10.7245029251417,3.99201318730094,-0.170415006145854));
#46608=CARTESIAN_POINT('Ctrl Pts',(-10.6987448320663,3.89762597078122,-0.694336325539465));
#46609=CARTESIAN_POINT('Ctrl Pts',(-10.6526167146807,3.73129383433858,-1.4112761495687));
#46610=CARTESIAN_POINT('Ctrl Pts',(-10.5873503968315,3.50241778183169,-2.2275339890855));
#46611=CARTESIAN_POINT('Ctrl Pts',(-10.4931468457969,3.18400912617635,-3.25905161930202));
#46612=CARTESIAN_POINT('Ctrl Pts',(-10.3710530115233,2.80490032403984,-4.44792213541537));
#46613=CARTESIAN_POINT('Ctrl Pts',(-10.291981634001,2.60132190971847,-5.29067996192501));
#46614=CARTESIAN_POINT('Ctrl Pts',(-10.259322478708,2.52389752423809,-5.78301376090809));
#46615=CARTESIAN_POINT('Ctrl Pts',(-10.2482225058791,2.49208086099759,-6.01004845414477));
#46616=CARTESIAN_POINT('Ctrl Pts',(-10.2292708277151,2.44043284506256,-6.45365676938782));
#46617=CARTESIAN_POINT('Ctrl Pts',(-10.205360681967,2.37340808795552,-7.2531223258534));
#46618=CARTESIAN_POINT('Ctrl Pts',(-10.1910379110981,2.3361078750475,-8.43147609383172));
#46619=CARTESIAN_POINT('Ctrl Pts',(-10.1890967787696,2.33838464644536,-9.66414306851534));
#46620=CARTESIAN_POINT('Ctrl Pts',(-10.1873900792642,2.33855686624078,-10.551771751452));
#46621=CARTESIAN_POINT('Ctrl Pts',(-10.1854661676253,2.33473549177642,-11.066367517675));
#46622=CARTESIAN_POINT('Ctrl Pts',(-10.184042692168,2.33093798611811,-11.3261071331523));
#46623=CARTESIAN_POINT('Ctrl Pts',(-10.1827439703201,2.32713737341463,-11.5223106200541));
#46624=CARTESIAN_POINT('Ctrl Pts',(-10.1818623385683,2.32489346802413,-11.6431857937223));
#46625=CARTESIAN_POINT('Ctrl Pts',(-10.1802954994666,2.32086307815761,-11.8911005848554));
#46626=CARTESIAN_POINT('Ctrl Pts',(-10.1779607276946,2.31523914030324,-12.3218418170449));
#46627=CARTESIAN_POINT('Ctrl Pts',(-10.1748417521086,2.30894474871518,-13.1859670501784));
#46628=CARTESIAN_POINT('Ctrl Pts',(-10.1738155008547,2.31102400307239,-14.4226015029144));
#46629=CARTESIAN_POINT('Ctrl Pts',(-10.1749096307113,2.31844253624813,-15.5457906685208));
#46630=CARTESIAN_POINT('Ctrl Pts',(-10.1756110161507,2.32242724348455,-16.3007012118884));
#46631=CARTESIAN_POINT('Ctrl Pts',(-10.1760099430421,2.32459889120294,-16.8058145157111));
#46632=CARTESIAN_POINT('Ctrl Pts',(-10.1761869447333,2.32545056715243,-17.1868384155883));
#46633=CARTESIAN_POINT('Ctrl Pts',(-10.1761822187404,2.32543659934831,-17.5048968202555));
#46634=CARTESIAN_POINT('Ctrl Pts',(-10.1761964886654,2.32543216834755,-17.6291972230455));
#46635=CARTESIAN_POINT('Ctrl Pts',(-10.1762858482566,2.32542812266568,-17.8788418177221));
#46636=CARTESIAN_POINT('Ctrl Pts',(-10.1764633139881,2.32543489780847,-18.1282238990403));
#46637=CARTESIAN_POINT('Ctrl Pts',(-10.176709640203,2.32544837257372,-18.3779084247801));
#46638=CARTESIAN_POINT('Ctrl Pts',(-10.1768912054176,2.32546123226444,-18.5339633782873));
#46639=CARTESIAN_POINT('Ctrl Pts',(-10.1770504328865,2.32547350977745,-18.6588523774397));
#46640=CARTESIAN_POINT('Ctrl Pts',(-10.1771767398731,2.32548401121934,-18.7525291247011));
#46641=CARTESIAN_POINT('Ctrl Pts',(-10.1772873744373,2.32549385467383,-18.8306067078381));
#46642=CARTESIAN_POINT('Ctrl Pts',(-10.1773787570869,2.3255022748062,-18.893075633532));
#46643=CARTESIAN_POINT('Ctrl Pts',(-10.1781722001408,2.32557784693258,-19.4241027318974));
#46644=CARTESIAN_POINT('Ctrl Pts',(-10.1802391085788,2.32588556059833,-20.4405830164739));
#46645=CARTESIAN_POINT('Ctrl Pts',(-10.1829097809687,2.32671242001792,-21.9461597427201));
#46646=CARTESIAN_POINT('Ctrl Pts',(-10.1833711322145,2.32765213655555,-22.9531075140253));
#46647=CARTESIAN_POINT('Ctrl Pts',(-10.1828438775792,2.32834169386881,-23.5818011088191));
#46648=CARTESIAN_POINT('Ctrl Pts',(-10.182556795248,2.32863831763781,-23.8305131431512));
#46649=CARTESIAN_POINT('Ctrl Pts',(-10.1817206536772,2.32932917945615,-24.3289448593721));
#46650=CARTESIAN_POINT('Ctrl Pts',(-10.1796488766789,2.33075497774474,-25.2033338196031));
#46651=CARTESIAN_POINT('Ctrl Pts',(-10.1754960322699,2.33324047082322,-26.4573585609411));
#46652=CARTESIAN_POINT('Ctrl Pts',(-10.1701133843866,2.33624987105413,-27.9665370845329));
#46653=CARTESIAN_POINT('Ctrl Pts',(-10.167392028961,2.33789044740065,-28.9722307369851));
#46654=CARTESIAN_POINT('Ctrl Pts',(-10.1663804217523,2.33858566329863,-29.538352557414));
#46655=CARTESIAN_POINT('Ctrl Pts',(-10.1660110912668,2.33819003936893,-29.6765341761858));
#46656=CARTESIAN_POINT('Ctrl Pts',(-10.164777103551,2.33532769799564,-29.9437575708518));
#46657=CARTESIAN_POINT('Ctrl Pts',(-10.1614248907804,2.32554339954716,-30.4100054116301));
#46658=CARTESIAN_POINT('Ctrl Pts',(-10.1509829711924,2.29164239193802,-31.3196602435576));
#46659=CARTESIAN_POINT('Ctrl Pts',(-10.1314429635782,2.22865322636961,-32.5630530289834));
#46660=CARTESIAN_POINT('Ctrl Pts',(-10.1239578463117,2.20990497774048,-33.7276319436604));
#46661=CARTESIAN_POINT('Ctrl Pts',(-10.1382272091451,2.25365471385146,-34.6108266770133));
#46662=CARTESIAN_POINT('Ctrl Pts',(-10.1545213545452,2.2995154614481,-35.0359677653007));
#46663=CARTESIAN_POINT('Ctrl Pts',(-10.1711414781042,2.34440310676093,-35.3489526983482));
#46664=CARTESIAN_POINT('Ctrl Pts',(-10.1851098617071,2.37744042159386,-35.5389379447642));
#46665=CARTESIAN_POINT('Ctrl Pts',(-10.219077321318,2.46500957214916,-35.9465551226477));
#46666=CARTESIAN_POINT('Ctrl Pts',(-10.2925513678124,2.66590288201721,-36.6907927120213));
#46667=CARTESIAN_POINT('Ctrl Pts',(-10.4672915221739,3.21377553661836,-38.3318422142825));
#46668=CARTESIAN_POINT('Ctrl Pts',(-10.6127099001957,3.76161631783265,-39.985236248682));
#46669=CARTESIAN_POINT('Ctrl Pts',(-10.669499445744,3.97735825964587,-41.5392455494394));
#46670=CARTESIAN_POINT('Ctrl Pts',(-10.6834790497686,4.02170688238063,-41.9700526817855));
#46671=CARTESIAN_POINT('Ctrl Pts',(-10.6968123531277,4.05775966332809,-42.5420665740536));
#46672=CARTESIAN_POINT('Ctrl Pts',(-10.7069670754181,4.07969938553161,-43.1010554995864));
#46673=CARTESIAN_POINT('Ctrl Pts',(-10.7143533231186,4.08658995129601,-43.7820402933545));
#46674=CARTESIAN_POINT('Ctrl Pts',(-10.7170251331761,4.07621708661553,-44.5674691109912));
#46675=CARTESIAN_POINT('Ctrl Pts',(-10.7160390580498,4.06305808236085,-45.1962275583449));
#46676=CARTESIAN_POINT('Ctrl Pts',(-10.7145238579317,4.05561185326259,-45.6829976418167));
#46677=CARTESIAN_POINT('Ctrl Pts',(-10.7133007288124,4.05286283457337,-46.040081421822));
#46678=CARTESIAN_POINT('Ctrl Pts',(-10.7122864672143,4.05418486041162,-46.3889558225569));
#46679=CARTESIAN_POINT('Ctrl Pts',(-10.7116148380017,4.06290648666823,-46.8432204483996));
#46680=CARTESIAN_POINT('Ctrl Pts',(-10.7122825915524,4.07881746233585,-47.1713383938465));
#46681=CARTESIAN_POINT('Ctrl Pts',(-10.7143508228806,4.10302756806235,-47.4931458846201));
#46682=CARTESIAN_POINT('Ctrl Pts',(-10.715686897772,4.12265857937166,-47.753639792098));
#46683=CARTESIAN_POINT('Ctrl Pts',(-10.718164607178,4.16057100812037,-48.2457370669567));
#46684=CARTESIAN_POINT('Ctrl Pts',(-10.7219473309798,4.23079720928861,-49.1118649713687));
#46685=CARTESIAN_POINT('Ctrl Pts',(-10.7255526649831,4.34667077707044,-50.3176218146149));
#46686=CARTESIAN_POINT('Ctrl Pts',(-10.7265601494607,4.53579485376256,-51.7301734409053));
#46687=CARTESIAN_POINT('Ctrl Pts',(-10.7245563309438,4.70950264467719,-52.6453714483989));
#46688=CARTESIAN_POINT('Ctrl Pts',(-10.7223848813205,4.83783044140274,-53.2119653734534));
#46689=CARTESIAN_POINT('Ctrl Pts',(-10.7213419894687,4.89280876274709,-53.4468056233345));
#46690=CARTESIAN_POINT('Ctrl Pts',(-10.7185909308167,5.00933732238949,-53.9149973687165));
#46691=CARTESIAN_POINT('Ctrl Pts',(-10.7122736331623,5.23224005705955,-54.7401180405057));
#46692=CARTESIAN_POINT('Ctrl Pts',(-10.6953636514727,5.74746593397295,-56.4013982419585));
#46693=CARTESIAN_POINT('Ctrl Pts',(-10.6795026822741,6.29233680493474,-57.8359715964635));
#46694=CARTESIAN_POINT('Ctrl Pts',(-10.6729996788152,6.71055227811244,-58.8460496147919));
#46695=CARTESIAN_POINT('Ctrl Pts',(-10.6721930196659,6.75861817572571,-58.9606199063025));
#46696=CARTESIAN_POINT('Ctrl Pts',(-10.6706386559564,6.85958025905996,-59.1956605069516));
#46697=CARTESIAN_POINT('Ctrl Pts',(-10.6680297375051,7.04250853252697,-59.6074430378433));
#46698=CARTESIAN_POINT('Ctrl Pts',(-10.6632723032891,7.43570291173815,-60.4432491785754));
#46699=CARTESIAN_POINT('Ctrl Pts',(-10.6588558170839,7.93410394761738,-61.4162871376521));
#46700=CARTESIAN_POINT('Ctrl Pts',(-10.6552771893509,8.45866189811967,-62.4019273521771));
#46701=CARTESIAN_POINT('Ctrl Pts',(-10.6535421547273,8.75885908803885,-62.9599707044205));
#46702=CARTESIAN_POINT('Ctrl Pts',(-10.6524909466147,8.9592766719587,-63.3333135438091));
#46703=CARTESIAN_POINT('Ctrl Pts',(-10.6518156015038,9.09283556102529,-63.5825506072565));
#46704=CARTESIAN_POINT('Ctrl Pts',(-10.651184724697,9.22610620049791,-63.8322398641344));
#46705=CARTESIAN_POINT('Ctrl Pts',(-10.6506626166579,9.34215666827589,-64.0511504440258));
#46706=CARTESIAN_POINT('Ctrl Pts',(-10.6503735525664,9.40826187449771,-64.1763620347625));
#46707=CARTESIAN_POINT('Ctrl Pts',(-10.6499487261179,9.50717944570217,-64.364286131224));
#46708=CARTESIAN_POINT('Ctrl Pts',(-10.649616156931,9.5890857669874,-64.5211573177303));
#46709=CARTESIAN_POINT('Ctrl Pts',(-10.6490865991625,9.72357093821706,-64.7809357767682));
#46710=CARTESIAN_POINT('Ctrl Pts',(-10.6486084730312,9.85450403883141,-65.0330096286938));
#46711=CARTESIAN_POINT('Ctrl Pts',(-10.6478935030841,10.1206875040802,-65.5424428653429));
#46712=CARTESIAN_POINT('Ctrl Pts',(-10.6472235238906,10.5837849990798,-66.4214697243471));
#46713=CARTESIAN_POINT('Ctrl Pts',(-10.6476327795485,11.5114983625212,-68.1601729075373));
#46714=CARTESIAN_POINT('Ctrl Pts',(-10.6492165339314,12.3086856507892,-69.6386485829911));
#46715=CARTESIAN_POINT('Ctrl Pts',(-10.6492051597913,12.911799051916,-70.7728833401244));
#46716=CARTESIAN_POINT('Ctrl Pts',(-10.6492012024291,13.04506371583,-71.0235095231732));
#46717=CARTESIAN_POINT('Ctrl Pts',(-10.6491958831625,13.3121443479147,-71.5258020179872));
#46718=CARTESIAN_POINT('Ctrl Pts',(-10.6491947187677,13.6455327598224,-72.1528025111679));
#46719=CARTESIAN_POINT('Ctrl Pts',(-10.6491955778798,14.0455513877889,-72.9051254391018));
#46720=CARTESIAN_POINT('Ctrl Pts',(-10.6492032628139,14.8452014831371,-74.4090555915023));
#46721=CARTESIAN_POINT('Ctrl Pts',(-10.649224822732,15.5111509976849,-75.6615339080009));
#46722=CARTESIAN_POINT('Ctrl Pts',(-10.6492307550641,16.4808865796188,-77.4853330368044));
#46723=CARTESIAN_POINT('Ctrl Pts',(-10.6492338083976,16.91736931297,-78.3062334180857));
#46724=CARTESIAN_POINT('Ctrl Pts',(-10.6492338083975,17.3538909003594,-79.1272111201841));
#46725=CARTESIAN_POINT('Ctrl Pts',(-8.14359067365561,4.07985970540613,24.8306345375628));
#46726=CARTESIAN_POINT('Ctrl Pts',(-8.14361498400114,4.07985970354231,24.7817552188885));
#46727=CARTESIAN_POINT('Ctrl Pts',(-8.14364047300421,4.07985966976465,24.7328766250053));
#46728=CARTESIAN_POINT('Ctrl Pts',(-8.14394180053891,4.07986071796207,24.1822795439549));
#46729=CARTESIAN_POINT('Ctrl Pts',(-8.14417414872545,4.0798695436064,23.1782365679108));
#46730=CARTESIAN_POINT('Ctrl Pts',(-8.14471009420409,4.07987017975739,21.1696477877977));
#46731=CARTESIAN_POINT('Ctrl Pts',(-8.14671893325979,4.07989225735344,19.6657249052665));
#46732=CARTESIAN_POINT('Ctrl Pts',(-8.15097310704072,4.07990210697193,18.4147762947717));
#46733=CARTESIAN_POINT('Ctrl Pts',(-8.15301249508394,4.07990363804429,17.9119749489971));
#46734=CARTESIAN_POINT('Ctrl Pts',(-8.15813390489173,4.07991001310458,16.9080501386704));
#46735=CARTESIAN_POINT('Ctrl Pts',(-8.16911747042228,4.07991677228478,15.1543077434332));
#46736=CARTESIAN_POINT('Ctrl Pts',(-8.17956482346294,4.07996837376312,13.653088880244));
#46737=CARTESIAN_POINT('Ctrl Pts',(-8.18611672759872,4.07999333067391,12.3988607914225));
#46738=CARTESIAN_POINT('Ctrl Pts',(-8.18879534967467,4.08000198216328,11.897974147008));
#46739=CARTESIAN_POINT('Ctrl Pts',(-8.1942549631774,4.08000682487738,10.896207146212));
#46740=CARTESIAN_POINT('Ctrl Pts',(-8.20101754403269,4.08005903324089,9.64406333425493));
#46741=CARTESIAN_POINT('Ctrl Pts',(-8.20814595172556,4.08008149013275,8.14012995143153));
#46742=CARTESIAN_POINT('Ctrl Pts',(-8.21168550255051,4.08016083230667,7.13558566831604));
#46743=CARTESIAN_POINT('Ctrl Pts',(-8.21332645458666,4.08017726326418,6.50909204522029));
#46744=CARTESIAN_POINT('Ctrl Pts',(-8.21413897927589,4.08237190936357,6.29028482577281));
#46745=CARTESIAN_POINT('Ctrl Pts',(-8.21626693784459,4.09412056112342,5.82321881151269));
#46746=CARTESIAN_POINT('Ctrl Pts',(-8.22090193607751,4.13075485442928,4.98737536189332));
#46747=CARTESIAN_POINT('Ctrl Pts',(-8.23093289196322,4.2335233754299,3.20246421710022));
#46748=CARTESIAN_POINT('Ctrl Pts',(-8.23022472659282,4.24340874447766,1.49794937469472));
#46749=CARTESIAN_POINT('Ctrl Pts',(-8.21578280303809,4.04343673099212,0.216408376068755));
#46750=CARTESIAN_POINT('Ctrl Pts',(-8.2139091204433,4.01529420171371,0.0512402447371398));
#46751=CARTESIAN_POINT('Ctrl Pts',(-8.20962119499329,3.95270323742799,-0.265737629226556));
#46752=CARTESIAN_POINT('Ctrl Pts',(-8.20081942730489,3.82480741036837,-0.810098156167453));
#46753=CARTESIAN_POINT('Ctrl Pts',(-8.18531801461245,3.60340048820505,-1.54625681655442));
#46754=CARTESIAN_POINT('Ctrl Pts',(-8.16359583366465,3.30577257714691,-2.37574729524026));
#46755=CARTESIAN_POINT('Ctrl Pts',(-8.13205640026516,2.90059244028148,-3.41528007458188));
#46756=CARTESIAN_POINT('Ctrl Pts',(-8.08937811281637,2.4355293602073,-4.60151152308765));
#46757=CARTESIAN_POINT('Ctrl Pts',(-8.05746883191124,2.20819553877365,-5.41164033896553));
#46758=CARTESIAN_POINT('Ctrl Pts',(-8.04345040864611,2.1263656741961,-5.86462386581994));
#46759=CARTESIAN_POINT('Ctrl Pts',(-8.03895818083086,2.08989753972466,-6.08463724447221));
#46760=CARTESIAN_POINT('Ctrl Pts',(-8.03108232980876,2.03198126703692,-6.51016269028769));
#46761=CARTESIAN_POINT('Ctrl Pts',(-8.02117765134921,1.95592016996364,-7.28340190344963));
#46762=CARTESIAN_POINT('Ctrl Pts',(-8.01522206297929,1.91357126242899,-8.43458939573691));
#46763=CARTESIAN_POINT('Ctrl Pts',(-8.01425114707161,1.91732011821017,-9.65957978464447));
#46764=CARTESIAN_POINT('Ctrl Pts',(-8.01335348109672,1.91845193485591,-10.5513493386686));
#46765=CARTESIAN_POINT('Ctrl Pts',(-8.01248383477213,1.9142489375257,-11.0712064747836));
#46766=CARTESIAN_POINT('Ctrl Pts',(-8.0118763575149,1.90981310339595,-11.33455059115));
#46767=CARTESIAN_POINT('Ctrl Pts',(-8.01133566115346,1.90530015540803,-11.5337232509074));
#46768=CARTESIAN_POINT('Ctrl Pts',(-8.01094689215894,1.90277321047312,-11.6527536236799));
#46769=CARTESIAN_POINT('Ctrl Pts',(-8.01025266008061,1.89818676723235,-11.8992409803262));
#46770=CARTESIAN_POINT('Ctrl Pts',(-8.00918009773255,1.89189696236533,-12.3266360319494));
#46771=CARTESIAN_POINT('Ctrl Pts',(-8.00761285103791,1.88516044318482,-13.1858364518625));
#46772=CARTESIAN_POINT('Ctrl Pts',(-8.00664309424968,1.88871336098231,-14.4179058392809));
#46773=CARTESIAN_POINT('Ctrl Pts',(-8.00659588312024,1.89837865245115,-15.5407647870117));
#46774=CARTESIAN_POINT('Ctrl Pts',(-8.00662679781179,1.90352367064465,-16.2968921892087));
#46775=CARTESIAN_POINT('Ctrl Pts',(-8.00664346099735,1.90632656545951,-16.8032216726378));
#46776=CARTESIAN_POINT('Ctrl Pts',(-8.00664413152868,1.90742099344714,-17.1855914707571));
#46777=CARTESIAN_POINT('Ctrl Pts',(-8.00660749593276,1.90742145720269,-17.5049782515705));
#46778=CARTESIAN_POINT('Ctrl Pts',(-8.00660252735443,1.90742315116677,-17.6290173248691));
#46779=CARTESIAN_POINT('Ctrl Pts',(-8.0066285599827,1.90743215431583,-17.8786228825783));
#46780=CARTESIAN_POINT('Ctrl Pts',(-8.00670679073166,1.90744943452059,-18.1278229010574));
#46781=CARTESIAN_POINT('Ctrl Pts',(-8.00682588342566,1.90747185469976,-18.3774486894127));
#46782=CARTESIAN_POINT('Ctrl Pts',(-8.00691672070047,1.90748801250143,-18.533459000571));
#46783=CARTESIAN_POINT('Ctrl Pts',(-8.00699772411189,1.90750178011767,-18.6583280627768));
#46784=CARTESIAN_POINT('Ctrl Pts',(-8.00706258068671,1.90751254413139,-18.7519917259217));
#46785=CARTESIAN_POINT('Ctrl Pts',(-8.00711983429507,1.90752183146061,-18.8300624342547));
#46786=CARTESIAN_POINT('Ctrl Pts',(-8.00716736235425,1.90752938420153,-18.8925276007566));
#46787=CARTESIAN_POINT('Ctrl Pts',(-8.00758134301623,1.90759445283299,-19.4235338608292));
#46788=CARTESIAN_POINT('Ctrl Pts',(-8.0086962754387,1.90775669668981,-20.4403124276682));
#46789=CARTESIAN_POINT('Ctrl Pts',(-8.01014433860419,1.90779978173849,-21.9473206928697));
#46790=CARTESIAN_POINT('Ctrl Pts',(-8.01034363847009,1.90756341118158,-22.9558654320696));
#46791=CARTESIAN_POINT('Ctrl Pts',(-8.00999713654423,1.90727111718054,-23.5857649516545));
#46792=CARTESIAN_POINT('Ctrl Pts',(-8.00981335169339,1.90713624766546,-23.8351803292311));
#46793=CARTESIAN_POINT('Ctrl Pts',(-8.00928852377032,1.90680231431617,-24.3347012742357));
#46794=CARTESIAN_POINT('Ctrl Pts',(-8.00800826908139,1.90607221168703,-25.2106658285509));
#46795=CARTESIAN_POINT('Ctrl Pts',(-8.0054751748871,1.90473976488522,-26.4656402154394));
#46796=CARTESIAN_POINT('Ctrl Pts',(-8.00226388458962,1.90307892723492,-27.9742477266283));
#46797=CARTESIAN_POINT('Ctrl Pts',(-8.00069638142823,1.90219781638892,-28.9780396393795));
#46798=CARTESIAN_POINT('Ctrl Pts',(-8.00015292486548,1.90184633791688,-29.5431662744624));
#46799=CARTESIAN_POINT('Ctrl Pts',(-7.99998955053817,1.90105102284858,-29.6857229368641));
#46800=CARTESIAN_POINT('Ctrl Pts',(-7.99949651434298,1.89694107561718,-29.9583428203848));
#46801=CARTESIAN_POINT('Ctrl Pts',(-7.99822851669594,1.8839487287467,-30.4336135537794));
#46802=CARTESIAN_POINT('Ctrl Pts',(-7.99437868132817,1.84095506174159,-31.3532492515463));
#46803=CARTESIAN_POINT('Ctrl Pts',(-7.98693475241986,1.76463960510802,-32.5918758214193));
#46804=CARTESIAN_POINT('Ctrl Pts',(-7.98386044087593,1.74322772090953,-33.7234925777175));
#46805=CARTESIAN_POINT('Ctrl Pts',(-7.99005560425241,1.7911516553672,-34.5645435207993));
#46806=CARTESIAN_POINT('Ctrl Pts',(-7.99711971545115,1.84073247083906,-34.9647455338871));
#46807=CARTESIAN_POINT('Ctrl Pts',(-8.00427652327302,1.88895588939534,-35.2583124376742));
#46808=CARTESIAN_POINT('Ctrl Pts',(-8.01052992775479,1.92243043124532,-35.4299041084946));
#46809=CARTESIAN_POINT('Ctrl Pts',(-8.02486144232338,2.01643622035667,-35.8128967008395));
#46810=CARTESIAN_POINT('Ctrl Pts',(-8.05402181482127,2.24231511479637,-36.5298589220037));
#46811=CARTESIAN_POINT('Ctrl Pts',(-8.11431219801583,2.90130270715427,-38.1671665136789));
#46812=CARTESIAN_POINT('Ctrl Pts',(-8.15836776367972,3.61801973043291,-39.8396120423116));
#46813=CARTESIAN_POINT('Ctrl Pts',(-8.17719495330526,3.91520482254767,-41.4700177478095));
#46814=CARTESIAN_POINT('Ctrl Pts',(-8.18205149246931,3.97542999084137,-41.910711262013));
#46815=CARTESIAN_POINT('Ctrl Pts',(-8.1868566749838,4.02740123566261,-42.499800897281));
#46816=CARTESIAN_POINT('Ctrl Pts',(-8.19066643647986,4.06077088406066,-43.0727636686921));
#46817=CARTESIAN_POINT('Ctrl Pts',(-8.19371029383873,4.07580536115162,-43.7684561040316));
#46818=CARTESIAN_POINT('Ctrl Pts',(-8.19530062342225,4.06862371922948,-44.5653141924112));
#46819=CARTESIAN_POINT('Ctrl Pts',(-8.19551033397204,4.05540999605244,-45.1988643282004));
#46820=CARTESIAN_POINT('Ctrl Pts',(-8.19539543435627,4.04743325365432,-45.6865563975787));
#46821=CARTESIAN_POINT('Ctrl Pts',(-8.1952518247706,4.0443339961423,-46.042885636124));
#46822=CARTESIAN_POINT('Ctrl Pts',(-8.19514514727457,4.04556228771761,-46.3895285851106));
#46823=CARTESIAN_POINT('Ctrl Pts',(-8.19518123664623,4.05472027090549,-46.8388990362217));
#46824=CARTESIAN_POINT('Ctrl Pts',(-8.19553163699906,4.07185001917136,-47.1611021829135));
#46825=CARTESIAN_POINT('Ctrl Pts',(-8.19629659062148,4.09802470116959,-47.4758325557082));
#46826=CARTESIAN_POINT('Ctrl Pts',(-8.19679452923414,4.11986249700318,-47.7376494555348));
#46827=CARTESIAN_POINT('Ctrl Pts',(-8.19773917498253,4.16167351614696,-48.2291392276498));
#46828=CARTESIAN_POINT('Ctrl Pts',(-8.19920722922556,4.23888748557492,-49.0963063923987));
#46829=CARTESIAN_POINT('Ctrl Pts',(-8.20054154878142,4.36400652509188,-50.3035936590456));
#46830=CARTESIAN_POINT('Ctrl Pts',(-8.20025279113926,4.56221439394529,-51.720273945602));
#46831=CARTESIAN_POINT('Ctrl Pts',(-8.19827155368996,4.74008618271685,-52.6391087835333));
#46832=CARTESIAN_POINT('Ctrl Pts',(-8.19633734306815,4.87024377764062,-53.2082681627338));
#46833=CARTESIAN_POINT('Ctrl Pts',(-8.1954469406703,4.92590316907518,-53.4443026616136));
#46834=CARTESIAN_POINT('Ctrl Pts',(-8.19322130190796,5.04332674104089,-53.9145154326853));
#46835=CARTESIAN_POINT('Ctrl Pts',(-8.1883333481497,5.26676583637175,-54.7426361152984));
#46836=CARTESIAN_POINT('Ctrl Pts',(-8.1757679372123,5.77947514538758,-56.407552918538));
#46837=CARTESIAN_POINT('Ctrl Pts',(-8.16434196831385,6.31847818783456,-57.8418435904684));
#46838=CARTESIAN_POINT('Ctrl Pts',(-8.15963822163446,6.73329256363275,-58.8503748905591));
#46839=CARTESIAN_POINT('Ctrl Pts',(-8.15905775023175,6.78114781912818,-58.9652211373289));
#46840=CARTESIAN_POINT('Ctrl Pts',(-8.1579455881897,6.88150913430379,-59.2005123816663));
#46841=CARTESIAN_POINT('Ctrl Pts',(-8.15609615307335,7.06330301541337,-59.6127829607361));
#46842=CARTESIAN_POINT('Ctrl Pts',(-8.15278801562376,7.45367427950311,-60.4491444615007));
#46843=CARTESIAN_POINT('Ctrl Pts',(-8.14983256375181,7.94800603254326,-61.4222671566292));
#46844=CARTESIAN_POINT('Ctrl Pts',(-8.14750217146235,8.4682998967399,-62.4074483788712));
#46845=CARTESIAN_POINT('Ctrl Pts',(-8.14638568785422,8.76616086589802,-62.9650380015432));
#46846=CARTESIAN_POINT('Ctrl Pts',(-8.14570869227385,8.96509688931052,-63.337988342902));
#46847=CARTESIAN_POINT('Ctrl Pts',(-8.14527332588339,9.09769332760823,-63.5869388592505));
#46848=CARTESIAN_POINT('Ctrl Pts',(-8.14486437782742,9.2300394234522,-63.8363037865726));
#46849=CARTESIAN_POINT('Ctrl Pts',(-8.14452353060581,9.34532853518197,-64.0548942082687));
#46850=CARTESIAN_POINT('Ctrl Pts',(-8.14433379730441,9.41101293112661,-64.1799120519233));
#46851=CARTESIAN_POINT('Ctrl Pts',(-8.14405386623975,9.50931459878488,-64.3675345624609));
#46852=CARTESIAN_POINT('Ctrl Pts',(-8.14383173923921,9.59073785194436,-64.5241303521888));
#46853=CARTESIAN_POINT('Ctrl Pts',(-8.14347388326224,9.72447785071259,-64.7834206217065));
#46854=CARTESIAN_POINT('Ctrl Pts',(-8.14315059498215,9.85478583013289,-65.0351043708353));
#46855=CARTESIAN_POINT('Ctrl Pts',(-8.1426673769054,10.1199249327764,-65.5437777065966));
#46856=CARTESIAN_POINT('Ctrl Pts',(-8.14221292863375,10.5818120711918,-66.421701667515));
#46857=CARTESIAN_POINT('Ctrl Pts',(-8.14248547303518,11.5090685253749,-68.159007849325));
#46858=CARTESIAN_POINT('Ctrl Pts',(-8.14354628768597,12.307761001971,-69.6377922875381));
#46859=CARTESIAN_POINT('Ctrl Pts',(-8.14353620190536,12.911344014831,-70.772980942748));
#46860=CARTESIAN_POINT('Ctrl Pts',(-8.14353341552564,13.0445655981629,-71.0235373309712));
#46861=CARTESIAN_POINT('Ctrl Pts',(-8.14352953341891,13.3116493812976,-71.5258532489965));
#46862=CARTESIAN_POINT('Ctrl Pts',(-8.14352815373002,13.6450115100796,-72.1528189545927));
#46863=CARTESIAN_POINT('Ctrl Pts',(-8.14352849833392,14.0450270936495,-72.9051390601201));
#46864=CARTESIAN_POINT('Ctrl Pts',(-8.14353340536773,14.844672016046,-74.4090483631363));
#46865=CARTESIAN_POINT('Ctrl Pts',(-8.14354658110851,15.510632305582,-75.6615281122465));
#46866=CARTESIAN_POINT('Ctrl Pts',(-8.14354957689417,16.4803713305245,-77.4853414851555));
#46867=CARTESIAN_POINT('Ctrl Pts',(-8.1435511206182,16.9168474424909,-78.3062334150556));
#46868=CARTESIAN_POINT('Ctrl Pts',(-8.14355112061824,17.3533690298803,-79.1272111171539));
#46869=CARTESIAN_POINT('Ctrl Pts',(-5.63811983077158,4.0798110453911,24.8306344764173));
#46870=CARTESIAN_POINT('Ctrl Pts',(-5.63813667009515,4.07981103868737,24.7817551557504));
#46871=CARTESIAN_POINT('Ctrl Pts',(-5.63815433701764,4.07981101700637,24.7328765654611));
#46872=CARTESIAN_POINT('Ctrl Pts',(-5.63836268468167,4.07981142746535,24.1822792717705));
#46873=CARTESIAN_POINT('Ctrl Pts',(-5.63852065580303,4.07981535515741,23.1782346942006));
#46874=CARTESIAN_POINT('Ctrl Pts',(-5.63889205174658,4.07981527489587,21.1696456974601));
#46875=CARTESIAN_POINT('Ctrl Pts',(-5.64027572822364,4.07982496773713,19.6657188641483));
#46876=CARTESIAN_POINT('Ctrl Pts',(-5.64321826748117,4.07982890067983,18.4147685276945));
#46877=CARTESIAN_POINT('Ctrl Pts',(-5.64463005020993,4.07982928332439,17.9119667849834));
#46878=CARTESIAN_POINT('Ctrl Pts',(-5.6481745914777,4.07983135640826,16.9080407682842));
#46879=CARTESIAN_POINT('Ctrl Pts',(-5.65577873214206,4.07983263368459,15.154297247445));
#46880=CARTESIAN_POINT('Ctrl Pts',(-5.66299499426907,4.07985516961286,13.653069830235));
#46881=CARTESIAN_POINT('Ctrl Pts',(-5.66752169513739,4.07986678165392,12.3988381804721));
#46882=CARTESIAN_POINT('Ctrl Pts',(-5.66937274434828,4.07987093327248,11.89795019356));
#46883=CARTESIAN_POINT('Ctrl Pts',(-5.67314947714156,4.07987374563993,10.8961834958768));
#46884=CARTESIAN_POINT('Ctrl Pts',(-5.6778107271837,4.07989921039916,9.64402970194642));
#46885=CARTESIAN_POINT('Ctrl Pts',(-5.68273433584236,4.07991095381561,8.14009705099834));
#46886=CARTESIAN_POINT('Ctrl Pts',(-5.68515560070412,4.07994929304356,7.13553148672606));
#46887=CARTESIAN_POINT('Ctrl Pts',(-5.68628369286022,4.0799558810801,6.50905008299334));
#46888=CARTESIAN_POINT('Ctrl Pts',(-5.68661227828105,4.0821707734076,6.29061534047278));
#46889=CARTESIAN_POINT('Ctrl Pts',(-5.68685741652079,4.09404275133035,5.82395335480346));
#46890=CARTESIAN_POINT('Ctrl Pts',(-5.68640262743183,4.131057365138,4.98858149230052));
#46891=CARTESIAN_POINT('Ctrl Pts',(-5.68350530942708,4.23503160832966,3.2034216507204));
#46892=CARTESIAN_POINT('Ctrl Pts',(-5.68296470658803,4.24486610544271,1.49622009174376));
#46893=CARTESIAN_POINT('Ctrl Pts',(-5.68852203732585,4.04203039227358,0.212287520177693));
#46894=CARTESIAN_POINT('Ctrl Pts',(-5.68924321529777,4.01347849406751,0.046709235164253));
#46895=CARTESIAN_POINT('Ctrl Pts',(-5.69088416757088,3.9499993638592,-0.270911948875149));
#46896=CARTESIAN_POINT('Ctrl Pts',(-5.69423798732707,3.82032929950973,-0.816214955379421));
#46897=CARTESIAN_POINT('Ctrl Pts',(-5.70010751539234,3.59593446010334,-1.5531574030428));
#46898=CARTESIAN_POINT('Ctrl Pts',(-5.70831033464785,3.29442582652292,-2.38303934284124));
#46899=CARTESIAN_POINT('Ctrl Pts',(-5.72007629462961,2.8838231834602,-3.42257142321862));
#46900=CARTESIAN_POINT('Ctrl Pts',(-5.73560085827451,2.41218424234636,-4.60822872165754));
#46901=CARTESIAN_POINT('Ctrl Pts',(-5.74639098412996,2.18193168509263,-5.41705257416455));
#46902=CARTESIAN_POINT('Ctrl Pts',(-5.75084932986925,2.09939451036815,-5.86836611662692));
#46903=CARTESIAN_POINT('Ctrl Pts',(-5.75224887165708,2.06251312929618,-6.08806225844426));
#46904=CARTESIAN_POINT('Ctrl Pts',(-5.75455662346494,2.00400564527647,-6.51278227068597));
#46905=CARTESIAN_POINT('Ctrl Pts',(-5.75704323174046,1.92716346979754,-7.28481605243417));
#46906=CARTESIAN_POINT('Ctrl Pts',(-5.75728937144342,1.88443606838965,-8.43471994322465));
#46907=CARTESIAN_POINT('Ctrl Pts',(-5.75559647584818,1.88839172766654,-9.65933007796948));
#46908=CARTESIAN_POINT('Ctrl Pts',(-5.75460419604941,1.88968255320358,-10.551294966269));
#46909=CARTESIAN_POINT('Ctrl Pts',(-5.75422580639182,1.88549557238442,-11.0713987092988));
#46910=CARTESIAN_POINT('Ctrl Pts',(-5.75412343706888,1.88103143023836,-11.3349108742082));
#46911=CARTESIAN_POINT('Ctrl Pts',(-5.75408795885295,1.87647917972426,-11.5342224131919));
#46912=CARTESIAN_POINT('Ctrl Pts',(-5.75406875447422,1.87393821481755,-11.6531700417011));
#46913=CARTESIAN_POINT('Ctrl Pts',(-5.75399196516393,1.86932816043943,-11.8995959559439));
#46914=CARTESIAN_POINT('Ctrl Pts',(-5.7537833470847,1.86302260711046,-12.3268436624762));
#46915=CARTESIAN_POINT('Ctrl Pts',(-5.75309093117271,1.85632747869761,-13.1858188002743));
#46916=CARTESIAN_POINT('Ctrl Pts',(-5.75161172540509,1.86012550832003,-14.4176857778353));
#46917=CARTESIAN_POINT('Ctrl Pts',(-5.7502891758143,1.87006941090163,-15.5405400231519));
#46918=CARTESIAN_POINT('Ctrl Pts',(-5.74965739204831,1.87535308030911,-16.2967352293748));
#46919=CARTESIAN_POINT('Ctrl Pts',(-5.74932122610216,1.87823317940958,-16.8031330828915));
#46920=CARTESIAN_POINT('Ctrl Pts',(-5.74917455039559,1.879353507465,-17.185567783641));
#46921=CARTESIAN_POINT('Ctrl Pts',(-5.74913660367459,1.87935773662425,-17.5050226590233));
#46922=CARTESIAN_POINT('Ctrl Pts',(-5.74912715497621,1.87936050099831,-17.6290501583932));
#46923=CARTESIAN_POINT('Ctrl Pts',(-5.74912915980342,1.87936960977166,-17.8786570132928));
#46924=CARTESIAN_POINT('Ctrl Pts',(-5.74915993777671,1.87938259823583,-18.1278504175768));
#46925=CARTESIAN_POINT('Ctrl Pts',(-5.74921789244708,1.87939863353372,-18.3774774876771));
#46926=CARTESIAN_POINT('Ctrl Pts',(-5.74926434468946,1.87940930689548,-18.5334881547362));
#46927=CARTESIAN_POINT('Ctrl Pts',(-5.74930744438421,1.87941812042794,-18.6583586298963));
#46928=CARTESIAN_POINT('Ctrl Pts',(-5.74934257466472,1.87942477883083,-18.7520234824479));
#46929=CARTESIAN_POINT('Ctrl Pts',(-5.74937411282463,1.87943032838155,-18.8300954190059));
#46930=CARTESIAN_POINT('Ctrl Pts',(-5.74940066971533,1.87943474528755,-18.8925617257007));
#46931=CARTESIAN_POINT('Ctrl Pts',(-5.74963349497633,1.87947194613293,-19.4235781652291));
#46932=CARTESIAN_POINT('Ctrl Pts',(-5.75030680770628,1.87953828501115,-20.4403864579149));
#46933=CARTESIAN_POINT('Ctrl Pts',(-5.75154253932412,1.87937850948638,-21.9475145185662));
#46934=CARTESIAN_POINT('Ctrl Pts',(-5.75227231363554,1.8789637696449,-22.9561714893139));
#46935=CARTESIAN_POINT('Ctrl Pts',(-5.75260896559746,1.87855701901834,-23.5861600617612));
#46936=CARTESIAN_POINT('Ctrl Pts',(-5.75274090704472,1.8783738852912,-23.8356407747635));
#46937=CARTESIAN_POINT('Ctrl Pts',(-5.7530035915229,1.87793175921572,-24.3352573609035));
#46938=CARTESIAN_POINT('Ctrl Pts',(-5.75345623247728,1.87698444246526,-25.2113610809742));
#46939=CARTESIAN_POINT('Ctrl Pts',(-5.75410335253425,1.87529370544626,-26.466402231886));
#46940=CARTESIAN_POINT('Ctrl Pts',(-5.75485157533096,1.87319974044047,-27.9749319318986));
#46941=CARTESIAN_POINT('Ctrl Pts',(-5.75536475828074,1.8720902164559,-28.978520248079));
#46942=CARTESIAN_POINT('Ctrl Pts',(-5.75564477714037,1.87163363136333,-29.5435243172313));
#46943=CARTESIAN_POINT('Ctrl Pts',(-5.75572710239254,1.87079791844986,-29.6862583907702));
#46944=CARTESIAN_POINT('Ctrl Pts',(-5.7559732761709,1.86657647359971,-29.9590863694963));
#46945=CARTESIAN_POINT('Ctrl Pts',(-5.75660291355869,1.85331399580364,-30.4347040823306));
#46946=CARTESIAN_POINT('Ctrl Pts',(-5.75849635156875,1.80957603802193,-31.354691687085));
#46947=CARTESIAN_POINT('Ctrl Pts',(-5.76213394704484,1.73216882177498,-32.593021500266));
#46948=CARTESIAN_POINT('Ctrl Pts',(-5.76395912661161,1.71051409224138,-33.7231624390665));
#46949=CARTESIAN_POINT('Ctrl Pts',(-5.76191446825069,1.75882557122053,-34.5624086421025));
#46950=CARTESIAN_POINT('Ctrl Pts',(-5.75931374360727,1.80882201987154,-34.9615780699163));
#46951=CARTESIAN_POINT('Ctrl Pts',(-5.75661140344506,1.85745189559095,-35.2543857289109));
#46952=CARTESIAN_POINT('Ctrl Pts',(-5.75427502016558,1.89113913253961,-35.4252911706769));
#46953=CARTESIAN_POINT('Ctrl Pts',(-5.74877203670678,1.98604763646328,-35.8074191182881));
#46954=CARTESIAN_POINT('Ctrl Pts',(-5.73730659438168,2.21474178036547,-36.5234184675721));
#46955=CARTESIAN_POINT('Ctrl Pts',(-5.7120749720574,2.88286698981103,-38.1598829728828));
#46956=CARTESIAN_POINT('Ctrl Pts',(-5.69254673513104,3.60881415531633,-39.8324051191482));
#46957=CARTESIAN_POINT('Ctrl Pts',(-5.68452159299678,3.91054498186973,-41.4662679038483));
#46958=CARTESIAN_POINT('Ctrl Pts',(-5.68254013735191,3.97166842840602,-41.9074238116326));
#46959=CARTESIAN_POINT('Ctrl Pts',(-5.68068243579163,4.02453622596769,-42.4973296815815));
#46960=CARTESIAN_POINT('Ctrl Pts',(-5.67928607379443,4.0585773765675,-43.0709771707241));
#46961=CARTESIAN_POINT('Ctrl Pts',(-5.67830151490437,4.07413410278548,-43.7673981168678));
#46962=CARTESIAN_POINT('Ctrl Pts',(-5.6779462875509,4.06725357191368,-44.5648212529693));
#46963=CARTESIAN_POINT('Ctrl Pts',(-5.6780039507709,4.0541686872801,-45.1986001289027));
#46964=CARTESIAN_POINT('Ctrl Pts',(-5.67805168872495,4.04624934430059,-45.6863132704687));
#46965=CARTESIAN_POINT('Ctrl Pts',(-5.67804111261185,4.04319948342737,-46.0425841801101));
#46966=CARTESIAN_POINT('Ctrl Pts',(-5.6779325512445,4.04449142376855,-46.3890923889201));
#46967=CARTESIAN_POINT('Ctrl Pts',(-5.67758811612929,4.0537583517493,-46.8381819987723));
#46968=CARTESIAN_POINT('Ctrl Pts',(-5.67703248391526,4.07102816651889,-47.1600641227476));
#46969=CARTESIAN_POINT('Ctrl Pts',(-5.67617262740912,4.09736871655714,-47.4744092201946));
#46970=CARTESIAN_POINT('Ctrl Pts',(-5.67557902458743,4.11938395574063,-47.7362172898861));
#46971=CARTESIAN_POINT('Ctrl Pts',(-5.67432229286351,4.1615378138823,-48.2275780346156));
#46972=CARTESIAN_POINT('Ctrl Pts',(-5.67196155999899,4.2394187879887,-49.0946582274887));
#46973=CARTESIAN_POINT('Ctrl Pts',(-5.66822236433425,4.36555257025762,-50.3019818330166));
#46974=CARTESIAN_POINT('Ctrl Pts',(-5.66346122247667,4.56483521974948,-51.7190419955286));
#46975=CARTESIAN_POINT('Ctrl Pts',(-5.66031908717494,4.7432141219391,-52.6383322139147));
#46976=CARTESIAN_POINT('Ctrl Pts',(-5.65842641225892,4.87357529674077,-53.2078297316513));
#46977=CARTESIAN_POINT('Ctrl Pts',(-5.65763279334113,4.92930042573472,-53.443979103778));
#46978=CARTESIAN_POINT('Ctrl Pts',(-5.65595953066154,5.04680714972081,-53.9144063560435));
#46979=CARTESIAN_POINT('Ctrl Pts',(-5.65284695680694,5.27027637536506,-54.7428396598825));
#46980=CARTESIAN_POINT('Ctrl Pts',(-5.64627494076859,5.78265301008943,-56.4081584805099));
#46981=CARTESIAN_POINT('Ctrl Pts',(-5.64135921227858,6.32101790767107,-57.8424309602114));
#46982=CARTESIAN_POINT('Ctrl Pts',(-5.63949652665682,6.73547863584439,-58.8507904213972));
#46983=CARTESIAN_POINT('Ctrl Pts',(-5.63928653869847,6.78331076444176,-58.9656636362908));
#46984=CARTESIAN_POINT('Ctrl Pts',(-5.63890771027011,6.88360892110182,-59.2009780371113));
#46985=CARTESIAN_POINT('Ctrl Pts',(-5.63835540921954,7.0652864652122,-59.6132948878965));
#46986=CARTESIAN_POINT('Ctrl Pts',(-5.63764220325501,7.45537724520633,-60.4497076603056));
#46987=CARTESIAN_POINT('Ctrl Pts',(-5.63752431161293,7.94931941092904,-61.4228364605725));
#46988=CARTESIAN_POINT('Ctrl Pts',(-5.63770957434784,8.46920822877576,-62.407972028973));
#46989=CARTESIAN_POINT('Ctrl Pts',(-5.63785544356127,8.76684757852313,-62.9655179354984));
#46990=CARTESIAN_POINT('Ctrl Pts',(-5.63793954007321,8.96564323452173,-63.3384309712243));
#46991=CARTESIAN_POINT('Ctrl Pts',(-5.63799004492039,9.0981483133153,-63.587354346538));
#46992=CARTESIAN_POINT('Ctrl Pts',(-5.6380293700383,9.23040715162897,-63.8366888380974));
#46993=CARTESIAN_POINT('Ctrl Pts',(-5.63804839120191,9.34562407058914,-64.0552493238614));
#46994=CARTESIAN_POINT('Ctrl Pts',(-5.63805412223214,9.41126855868899,-64.1802491025035));
#46995=CARTESIAN_POINT('Ctrl Pts',(-5.63805717980536,9.50951176212536,-64.367843532021));
#46996=CARTESIAN_POINT('Ctrl Pts',(-5.6380475231002,9.59088940584664,-64.5244138604548));
#46997=CARTESIAN_POINT('Ctrl Pts',(-5.63801079305937,9.72455865382169,-64.7836590069625));
#46998=CARTESIAN_POINT('Ctrl Pts',(-5.63797762980282,9.85480612401591,-65.0353043348998));
#46999=CARTESIAN_POINT('Ctrl Pts',(-5.63792896814358,10.1198445789927,-65.5439043825807));
#47000=CARTESIAN_POINT('Ctrl Pts',(-5.63788600675246,10.5816154268398,-66.4217215340489));
#47001=CARTESIAN_POINT('Ctrl Pts',(-5.63793010151783,11.5088280393636,-68.1588933370336));
#47002=CARTESIAN_POINT('Ctrl Pts',(-5.63805867663479,12.3076693165761,-69.6377086440991));
#47003=CARTESIAN_POINT('Ctrl Pts',(-5.63806207846908,12.9112986908887,-70.7729897237731));
#47004=CARTESIAN_POINT('Ctrl Pts',(-5.63806259215821,13.0445160360343,-71.0235393008888));
#47005=CARTESIAN_POINT('Ctrl Pts',(-5.63806340997343,13.3116000922036,-71.5258574053085));
#47006=CARTESIAN_POINT('Ctrl Pts',(-5.63806407959717,13.6449599288231,-72.1528197375819));
#47007=CARTESIAN_POINT('Ctrl Pts',(-5.63806420954367,14.0449753198509,-72.9051395116483));
#47008=CARTESIAN_POINT('Ctrl Pts',(-5.63806367905351,14.8446200315156,-74.4090467420857));
#47009=CARTESIAN_POINT('Ctrl Pts',(-5.63806272604161,15.5105827584323,-75.6615270456325));
#47010=CARTESIAN_POINT('Ctrl Pts',(-5.63806304115205,16.480322977286,-77.4853422474358));
#47011=CARTESIAN_POINT('Ctrl Pts',(-5.63806320330682,16.9167987952306,-78.3062334097084));
#47012=CARTESIAN_POINT('Ctrl Pts',(-5.6380632033068,17.3533203826201,-79.1272111118068));
#47013=CARTESIAN_POINT('Ctrl Pts',(-3.13246153243128,4.07997651007201,24.8306346929376));
#47014=CARTESIAN_POINT('Ctrl Pts',(-3.13247089418538,4.07997650841963,24.7817553791099));
#47015=CARTESIAN_POINT('Ctrl Pts',(-3.13248073019575,4.0799764999824,24.7328768125166));
#47016=CARTESIAN_POINT('Ctrl Pts',(-3.13259608346308,4.07997670521336,24.182279036014));
#47017=CARTESIAN_POINT('Ctrl Pts',(-3.13268004192053,4.07997855846402,23.1782298566771));
#47018=CARTESIAN_POINT('Ctrl Pts',(-3.13288642205627,4.07997867910101,21.1696404964704));
#47019=CARTESIAN_POINT('Ctrl Pts',(-3.13364578221095,4.0799832324987,19.6657020199627));
#47020=CARTESIAN_POINT('Ctrl Pts',(-3.13527679700413,4.07998506525854,18.4147466082921));
#47021=CARTESIAN_POINT('Ctrl Pts',(-3.13606077657042,4.07998526998077,17.9119444889898));
#47022=CARTESIAN_POINT('Ctrl Pts',(-3.13802802788143,4.079986323548,16.9080154538795));
#47023=CARTESIAN_POINT('Ctrl Pts',(-3.14225142760585,4.07998710858101,15.1542683993348));
#47024=CARTESIAN_POINT('Ctrl Pts',(-3.14623899167219,4.07999743609788,13.6530130576789));
#47025=CARTESIAN_POINT('Ctrl Pts',(-3.14874291676554,4.08000231729095,12.3987670988987));
#47026=CARTESIAN_POINT('Ctrl Pts',(-3.14976743684663,4.08000400625095,11.8978751789854));
#47027=CARTESIAN_POINT('Ctrl Pts',(-3.15186309537897,4.08000461207694,10.8961027948064));
#47028=CARTESIAN_POINT('Ctrl Pts',(-3.15442891598582,4.08001544469706,9.64393077047484));
#47029=CARTESIAN_POINT('Ctrl Pts',(-3.15715276547804,4.08001919774166,8.13996416710522));
#47030=CARTESIAN_POINT('Ctrl Pts',(-3.15846279414889,4.08003674923533,7.13540126819946));
#47031=CARTESIAN_POINT('Ctrl Pts',(-3.15908062329773,4.08003816023285,6.50882474162827));
#47032=CARTESIAN_POINT('Ctrl Pts',(-3.15911526939308,4.08212367410461,6.28831552518569));
#47033=CARTESIAN_POINT('Ctrl Pts',(-3.15848048672026,4.09328390772445,5.81940001756711));
#47034=CARTESIAN_POINT('Ctrl Pts',(-3.15591326515943,4.12798838607392,4.98127924385807));
#47035=CARTESIAN_POINT('Ctrl Pts',(-3.14813166420412,4.22506805010056,3.1975816317331));
#47036=CARTESIAN_POINT('Ctrl Pts',(-3.14767244725756,4.23363944617766,1.50398696059777));
#47037=CARTESIAN_POINT('Ctrl Pts',(-3.16052292115839,4.04611907631244,0.233676737286712));
#47038=CARTESIAN_POINT('Ctrl Pts',(-3.16219766233936,4.01982942180956,0.0704551119528957));
#47039=CARTESIAN_POINT('Ctrl Pts',(-3.16602623261079,3.96123348196748,-0.243381219684303));
#47040=CARTESIAN_POINT('Ctrl Pts',(-3.17389848003272,3.84135099620151,-0.782942923159161));
#47041=CARTESIAN_POINT('Ctrl Pts',(-3.18779167569196,3.63307987540551,-1.51464036672391));
#47042=CARTESIAN_POINT('Ctrl Pts',(-3.20735638942522,3.35219275299679,-2.34117066500064));
#47043=CARTESIAN_POINT('Ctrl Pts',(-3.235439752456,2.96839254434012,-3.37911107320271));
#47044=CARTESIAN_POINT('Ctrl Pts',(-3.27229518195219,2.52562813688982,-4.56654235231478));
#47045=CARTESIAN_POINT('Ctrl Pts',(-3.29720237517238,2.30579650243325,-5.38435096611615));
#47046=CARTESIAN_POINT('Ctrl Pts',(-3.30756077574448,2.22596212631942,-5.84630274445772));
#47047=CARTESIAN_POINT('Ctrl Pts',(-3.31093007785766,2.19093741307251,-6.06793896740053));
#47048=CARTESIAN_POINT('Ctrl Pts',(-3.31658942747022,2.1351222476834,-6.49759373842264));
#47049=CARTESIAN_POINT('Ctrl Pts',(-3.32319163754923,2.06203087472526,-7.27678156850551));
#47050=CARTESIAN_POINT('Ctrl Pts',(-3.32558236466508,2.02145012095799,-8.43403990693677));
#47051=CARTESIAN_POINT('Ctrl Pts',(-3.32378280330904,2.02503484919292,-9.66070491288416));
#47052=CARTESIAN_POINT('Ctrl Pts',(-3.32287201840796,2.02613264416804,-10.5515289245055));
#47053=CARTESIAN_POINT('Ctrl Pts',(-3.3227346144408,2.02215742955986,-11.0701974470837));
#47054=CARTESIAN_POINT('Ctrl Pts',(-3.32284448389422,2.01795424274816,-11.332729479163));
#47055=CARTESIAN_POINT('Ctrl Pts',(-3.32301404466847,2.01367939488763,-11.53123457802));
#47056=CARTESIAN_POINT('Ctrl Pts',(-3.32313722498826,2.0112677782415,-11.6506787843114));
#47057=CARTESIAN_POINT('Ctrl Pts',(-3.32331103943599,2.00690467237838,-11.89748565759));
#47058=CARTESIAN_POINT('Ctrl Pts',(-3.32347258593085,2.00092018770441,-12.3256288866842));
#47059=CARTESIAN_POINT('Ctrl Pts',(-3.32325066510606,1.99451852403883,-13.1859183629539));
#47060=CARTESIAN_POINT('Ctrl Pts',(-3.32188896287377,1.99795361317701,-14.4189916107135));
#47061=CARTESIAN_POINT('Ctrl Pts',(-3.32036839223327,2.00719741951532,-15.5419137868954));
#47062=CARTESIAN_POINT('Ctrl Pts',(-3.31962915770245,2.0121124570523,-16.2977655403261));
#47063=CARTESIAN_POINT('Ctrl Pts',(-3.31924152176754,2.01479460229474,-16.8038237906487));
#47064=CARTESIAN_POINT('Ctrl Pts',(-3.31907592200134,2.0158314682654,-17.1858894679804));
#47065=CARTESIAN_POINT('Ctrl Pts',(-3.31905512549647,2.01583203163852,-17.5049792714126));
#47066=CARTESIAN_POINT('Ctrl Pts',(-3.31905012686686,2.01583245129892,-17.6290757830511));
#47067=CARTESIAN_POINT('Ctrl Pts',(-3.31905184801735,2.01583331426224,-17.8786891251921));
#47068=CARTESIAN_POINT('Ctrl Pts',(-3.31906757056976,2.0158323002434,-18.1279282353765));
#47069=CARTESIAN_POINT('Ctrl Pts',(-3.3191013384169,2.01583191589402,-18.3775666952059));
#47070=CARTESIAN_POINT('Ctrl Pts',(-3.31912836294918,2.0158310957928,-18.5335866639419));
#47071=CARTESIAN_POINT('Ctrl Pts',(-3.31915410127115,2.01583041472837,-18.6584601282889));
#47072=CARTESIAN_POINT('Ctrl Pts',(-3.31917520496812,2.01582976162608,-18.7521266979761));
#47073=CARTESIAN_POINT('Ctrl Pts',(-3.31919428468052,2.01582910533478,-18.8301989563573));
#47074=CARTESIAN_POINT('Ctrl Pts',(-3.31921051348002,2.01582854200645,-18.8926650096216));
#47075=CARTESIAN_POINT('Ctrl Pts',(-3.31935299454499,2.0158230802846,-19.4236763218564));
#47076=CARTESIAN_POINT('Ctrl Pts',(-3.31977038350789,2.01580030672302,-20.4403885523284));
#47077=CARTESIAN_POINT('Ctrl Pts',(-3.32075106855808,2.01570023176383,-21.9470893374715));
#47078=CARTESIAN_POINT('Ctrl Pts',(-3.32157181599372,2.01557941182674,-22.95528802852));
#47079=CARTESIAN_POINT('Ctrl Pts',(-3.32211753059002,2.01547700548503,-23.5849287034935));
#47080=CARTESIAN_POINT('Ctrl Pts',(-3.32234988652394,2.01543157385401,-23.8341936474416));
#47081=CARTESIAN_POINT('Ctrl Pts',(-3.32287360422468,2.0153254693473,-24.3334809007202));
#47082=CARTESIAN_POINT('Ctrl Pts',(-3.32391775778534,2.015101851755,-25.2091088476071));
#47083=CARTESIAN_POINT('Ctrl Pts',(-3.32568020140797,2.01471957590141,-26.4638705192032));
#47084=CARTESIAN_POINT('Ctrl Pts',(-3.32780197716411,2.01423265478938,-27.972595312808));
#47085=CARTESIAN_POINT('Ctrl Pts',(-3.32900799672057,2.01398247390041,-28.9767733412754));
#47086=CARTESIAN_POINT('Ctrl Pts',(-3.32953413642664,2.01387212968397,-29.5421018627301));
#47087=CARTESIAN_POINT('Ctrl Pts',(-3.3296939340843,2.01317464310576,-29.6836563222014));
#47088=CARTESIAN_POINT('Ctrl Pts',(-3.33017578351236,2.00938412158686,-29.9550375559271));
#47089=CARTESIAN_POINT('Ctrl Pts',(-3.3314167404306,1.99724251365359,-30.4282373494448));
#47090=CARTESIAN_POINT('Ctrl Pts',(-3.335147244172,1.95671829490059,-31.3455852780583));
#47091=CARTESIAN_POINT('Ctrl Pts',(-3.34221805110568,1.88426174339899,-32.5852768887308));
#47092=CARTESIAN_POINT('Ctrl Pts',(-3.34538128669468,1.86377396555026,-33.7243082369932));
#47093=CARTESIAN_POINT('Ctrl Pts',(-3.34072556069709,1.9101320036685,-34.5749221415604));
#47094=CARTESIAN_POINT('Ctrl Pts',(-3.33517800218729,1.95825190715931,-34.980815480244));
#47095=CARTESIAN_POINT('Ctrl Pts',(-3.32946088735476,2.00508871093003,-35.2788486519617));
#47096=CARTESIAN_POINT('Ctrl Pts',(-3.32456081222768,2.0379715366224,-35.4546634245683));
#47097=CARTESIAN_POINT('Ctrl Pts',(-3.31293460674144,2.12929789170878,-35.8433961205832));
#47098=CARTESIAN_POINT('Ctrl Pts',(-3.28853996207654,2.34714506486481,-36.5669426610266));
#47099=CARTESIAN_POINT('Ctrl Pts',(-3.23364031644196,2.97565071964737,-38.2060920481217));
#47100=CARTESIAN_POINT('Ctrl Pts',(-3.19027619222017,3.65154768324503,-39.8744107469863));
#47101=CARTESIAN_POINT('Ctrl Pts',(-3.17249759774021,3.92919268912927,-41.4864989281616));
#47102=CARTESIAN_POINT('Ctrl Pts',(-3.16803503881843,3.98560986978033,-41.924808302215));
#47103=CARTESIAN_POINT('Ctrl Pts',(-3.16371082319947,4.03374733958927,-42.50977881643));
#47104=CARTESIAN_POINT('Ctrl Pts',(-3.16036569044979,4.06439536447749,-43.0793682933223));
#47105=CARTESIAN_POINT('Ctrl Pts',(-3.15781356584725,4.0775254173288,-43.7715087583553));
#47106=CARTESIAN_POINT('Ctrl Pts',(-3.15660863415327,4.06967246134424,-44.565604580691));
#47107=CARTESIAN_POINT('Ctrl Pts',(-3.15650839641553,4.05658252237076,-45.1979952075419));
#47108=CARTESIAN_POINT('Ctrl Pts',(-3.1565435502555,4.04877553148677,-45.6854537913944));
#47109=CARTESIAN_POINT('Ctrl Pts',(-3.15654584245324,4.04580005442802,-46.041956843755));
#47110=CARTESIAN_POINT('Ctrl Pts',(-3.15642264233075,4.04709350286183,-46.3891292965313));
#47111=CARTESIAN_POINT('Ctrl Pts',(-3.15595207495515,4.05619279220323,-46.8396663700083));
#47112=CARTESIAN_POINT('Ctrl Pts',(-3.15513097215849,4.07310082458682,-47.1632866091112));
#47113=CARTESIAN_POINT('Ctrl Pts',(-3.15377542439868,4.09884678590371,-47.479707997432));
#47114=CARTESIAN_POINT('Ctrl Pts',(-3.15285511663029,4.12018476751298,-47.7411685674074));
#47115=CARTESIAN_POINT('Ctrl Pts',(-3.15096410426876,4.16112998813786,-48.2327556738879));
#47116=CARTESIAN_POINT('Ctrl Pts',(-3.14756930875271,4.23681882402646,-49.0995994041402));
#47117=CARTESIAN_POINT('Ctrl Pts',(-3.14267760636433,4.36001820587265,-50.306498772196));
#47118=CARTESIAN_POINT('Ctrl Pts',(-3.13732213977395,4.55632511369512,-51.7222573422902));
#47119=CARTESIAN_POINT('Ctrl Pts',(-3.13455778158426,4.73336117998014,-52.6403571490209));
#47120=CARTESIAN_POINT('Ctrl Pts',(-3.13319134074485,4.86313021560044,-53.2089975544419));
#47121=CARTESIAN_POINT('Ctrl Pts',(-3.13265006762838,4.9186361337781,-53.4447701301428));
#47122=CARTESIAN_POINT('Ctrl Pts',(-3.13165517397761,5.0358537111696,-53.9145483609616));
#47123=CARTESIAN_POINT('Ctrl Pts',(-3.13012078195967,5.25915546982874,-54.7420249668827));
#47124=CARTESIAN_POINT('Ctrl Pts',(-3.12782238958505,5.77235304821454,-56.4061734854649));
#47125=CARTESIAN_POINT('Ctrl Pts',(-3.12698248255127,6.31259359307923,-57.8405523875656));
#47126=CARTESIAN_POINT('Ctrl Pts',(-3.12685681546202,6.72814653701198,-58.849405680646));
#47127=CARTESIAN_POINT('Ctrl Pts',(-3.12686554296575,6.77604672446337,-58.9641874740558));
#47128=CARTESIAN_POINT('Ctrl Pts',(-3.12691057834388,6.87653925030669,-59.1994174594256));
#47129=CARTESIAN_POINT('Ctrl Pts',(-3.12707983102319,7.05858307805198,-59.6115712603959));
#47130=CARTESIAN_POINT('Ctrl Pts',(-3.12771527570457,7.44958961654466,-60.4477976005926));
#47131=CARTESIAN_POINT('Ctrl Pts',(-3.12891079783518,7.94484369168065,-61.4208959414217));
#47132=CARTESIAN_POINT('Ctrl Pts',(-3.13018924482141,8.46611794513808,-62.4061818623611));
#47133=CARTESIAN_POINT('Ctrl Pts',(-3.13087047740976,8.76452013934969,-62.9638769612226));
#47134=CARTESIAN_POINT('Ctrl Pts',(-3.13127832354795,8.96380018570062,-63.3369195977));
#47135=CARTESIAN_POINT('Ctrl Pts',(-3.13153624858351,9.09662106248193,-63.5859376992535));
#47136=CARTESIAN_POINT('Ctrl Pts',(-3.13176873496221,9.2291808216599,-63.83537918543));
#47137=CARTESIAN_POINT('Ctrl Pts',(-3.13194584755131,9.34464736072837,-64.0540456196372));
#47138=CARTESIAN_POINT('Ctrl Pts',(-3.13203856099171,9.41042981104675,-64.1791095351821));
#47139=CARTESIAN_POINT('Ctrl Pts',(-3.13216881558075,9.50887516367422,-64.366803852895));
#47140=CARTESIAN_POINT('Ctrl Pts',(-3.13225753513511,9.59040972990737,-64.5234650042444));
#47141=CARTESIAN_POINT('Ctrl Pts',(-3.13237482956374,9.72432258242432,-64.7828716127369));
#47142=CARTESIAN_POINT('Ctrl Pts',(-3.13248085500744,9.85477252074289,-65.034643864059));
#47143=CARTESIAN_POINT('Ctrl Pts',(-3.13264062512874,10.1201508479262,-65.5434924893009));
#47144=CARTESIAN_POINT('Ctrl Pts',(-3.1327947935228,10.5823097329533,-66.4216676465916));
#47145=CARTESIAN_POINT('Ctrl Pts',(-3.13272766180581,11.5096631589717,-68.1592918173623));
#47146=CARTESIAN_POINT('Ctrl Pts',(-3.13240624429524,12.3079906420031,-69.6379977184845));
#47147=CARTESIAN_POINT('Ctrl Pts',(-3.13241552222347,12.9114595629432,-70.7729642751072));
#47148=CARTESIAN_POINT('Ctrl Pts',(-3.13241753864319,13.0446909444888,-71.0235366909736));
#47149=CARTESIAN_POINT('Ctrl Pts',(-3.13242047804576,13.3117734755119,-71.5258470058919));
#47150=CARTESIAN_POINT('Ctrl Pts',(-3.13242201833982,13.6451400591592,-72.1528200751521));
#47151=CARTESIAN_POINT('Ctrl Pts',(-3.13242202368236,14.0451556384799,-72.9051405493436));
#47152=CARTESIAN_POINT('Ctrl Pts',(-3.13241896755619,14.8448005576505,-74.4090541744763));
#47153=CARTESIAN_POINT('Ctrl Pts',(-3.13241140148778,15.5107532458981,-75.6615314781162));
#47154=CARTESIAN_POINT('Ctrl Pts',(-3.13241038779428,16.4804882519172,-77.4853402167882));
#47155=CARTESIAN_POINT('Ctrl Pts',(-3.13240986624166,16.9169642383694,-78.3062334166578));
#47156=CARTESIAN_POINT('Ctrl Pts',(-3.13240986624168,17.3534858257588,-79.1272111187562));
#47157=CARTESIAN_POINT('Ctrl Pts',(-0.626489942748934,4.0801671767227,24.8306349417617));
#47158=CARTESIAN_POINT('Ctrl Pts',(-0.626491814773436,4.08016718222176,
24.7817556358665));
#47159=CARTESIAN_POINT('Ctrl Pts',(-0.626493779413045,4.08016720727904,
24.7328771092215));
#47160=CARTESIAN_POINT('Ctrl Pts',(-0.626516920716058,4.08016662587312,
24.182278353298));
#47161=CARTESIAN_POINT('Ctrl Pts',(-0.626534327747216,4.08016137226147,
23.1782203340369));
#47162=CARTESIAN_POINT('Ctrl Pts',(-0.626575654255332,4.08016124138042,
21.1696301744221));
#47163=CARTESIAN_POINT('Ctrl Pts',(-0.626729038647951,4.08014822905217,
19.6656695004389));
#47164=CARTESIAN_POINT('Ctrl Pts',(-0.627055871811892,4.08014275662489,
18.4147044193244));
#47165=CARTESIAN_POINT('Ctrl Pts',(-0.62721275050798,4.08014208569092,17.9119012894618));
#47166=CARTESIAN_POINT('Ctrl Pts',(-0.62760657371311,4.08013891698227,16.9079662909586));
#47167=CARTESIAN_POINT('Ctrl Pts',(-0.628451593361296,4.08013626969629,
15.1542125529137));
#47168=CARTESIAN_POINT('Ctrl Pts',(-0.62925243724752,4.08010618381641,13.6529049111324));
#47169=CARTESIAN_POINT('Ctrl Pts',(-0.629754803362929,4.08009117188779,
12.3986331440833));
#47170=CARTESIAN_POINT('Ctrl Pts',(-0.629960240843974,4.08008594873699,
11.897733474683));
#47171=CARTESIAN_POINT('Ctrl Pts',(-0.630379618087822,4.08008258640544,
10.8959534737225));
#47172=CARTESIAN_POINT('Ctrl Pts',(-0.630896102434399,4.08005075094835,
9.64374037929921));
#47173=CARTESIAN_POINT('Ctrl Pts',(-0.631442292110968,4.08003511285241,
8.13972854909915));
#47174=CARTESIAN_POINT('Ctrl Pts',(-0.631709402747086,4.0799883832829,7.13513557854196));
#47175=CARTESIAN_POINT('Ctrl Pts',(-0.631834242062847,4.07997432028845,
6.50844855969211));
#47176=CARTESIAN_POINT('Ctrl Pts',(-0.631844614514806,4.08191249849963,
6.28569231433929));
#47177=CARTESIAN_POINT('Ctrl Pts',(-0.631735142604194,4.09228480802917,
5.81433836489286));
#47178=CARTESIAN_POINT('Ctrl Pts',(-0.631274195858156,4.12442247278467,
4.97319700222089));
#47179=CARTESIAN_POINT('Ctrl Pts',(-0.629860619545034,4.21411506066098,
3.19112813899561));
#47180=CARTESIAN_POINT('Ctrl Pts',(-0.629791657573271,4.22109561476111,
1.51180927237363));
#47181=CARTESIAN_POINT('Ctrl Pts',(-0.632171170914168,4.04961537706138,
0.256602357936203));
#47182=CARTESIAN_POINT('Ctrl Pts',(-0.632480675376951,4.02569735160545,
0.0960267302433405));
#47183=CARTESIAN_POINT('Ctrl Pts',(-0.633192562617259,3.97225933444396,
-0.213513276617349));
#47184=CARTESIAN_POINT('Ctrl Pts',(-0.634665809148591,3.86280982150925,
-0.746439893912946));
#47185=CARTESIAN_POINT('Ctrl Pts',(-0.637309271984396,3.67201501892076,
-1.47185578101335));
#47186=CARTESIAN_POINT('Ctrl Pts',(-0.641060370430275,3.41398006846141,
-2.29439316562927));
#47187=CARTESIAN_POINT('Ctrl Pts',(-0.646459524138124,3.0603623086103,-3.33078441011147));
#47188=CARTESIAN_POINT('Ctrl Pts',(-0.653388431714947,2.65109651410505,
-4.52187255833751));
#47189=CARTESIAN_POINT('Ctrl Pts',(-0.657692228357949,2.44619870872637,
-5.35101148090401));
#47190=CARTESIAN_POINT('Ctrl Pts',(-0.659392538492093,2.37141568249575,
-5.82433526064073));
#47191=CARTESIAN_POINT('Ctrl Pts',(-0.659974674390838,2.33899498785793,
-6.04804706925782));
#47192=CARTESIAN_POINT('Ctrl Pts',(-0.660931900586046,2.28720350004628,
-6.4828345029374));
#47193=CARTESIAN_POINT('Ctrl Pts',(-0.662055433531732,2.21949663209103,
-7.26920638472244));
#47194=CARTESIAN_POINT('Ctrl Pts',(-0.662459190736586,2.18173152333761,
-8.43357231943025));
#47195=CARTESIAN_POINT('Ctrl Pts',(-0.662129105637019,2.18458676173904,
-9.66218372788113));
#47196=CARTESIAN_POINT('Ctrl Pts',(-0.661950743587544,2.18532888680784,
-10.5518893013257));
#47197=CARTESIAN_POINT('Ctrl Pts',(-0.661920949871916,2.18155228774363,
-11.0691565471711));
#47198=CARTESIAN_POINT('Ctrl Pts',(-0.661939777952425,2.1776415075515,-11.3307324556826));
#47199=CARTESIAN_POINT('Ctrl Pts',(-0.661970318081918,2.17368544069136,
-11.528452907198));
#47200=CARTESIAN_POINT('Ctrl Pts',(-0.661990145017018,2.17143769689881,
-11.6483872617774));
#47201=CARTESIAN_POINT('Ctrl Pts',(-0.662018178672468,2.16737085478223,
-11.8955738266779));
#47202=CARTESIAN_POINT('Ctrl Pts',(-0.662041705006974,2.16176155662304,
-12.3246017479885));
#47203=CARTESIAN_POINT('Ctrl Pts',(-0.661995639177148,2.15563339321882,
-13.186166875794));
#47204=CARTESIAN_POINT('Ctrl Pts',(-0.661743624243537,2.15842740530346,
-14.4204024640238));
#47205=CARTESIAN_POINT('Ctrl Pts',(-0.661466000143103,2.16664586238682,
-15.5433657694493));
#47206=CARTESIAN_POINT('Ctrl Pts',(-0.661331657161525,2.17103469169633,
-16.2988620090364));
#47207=CARTESIAN_POINT('Ctrl Pts',(-0.661260755828687,2.17343601808264,
-16.8045796697433));
#47208=CARTESIAN_POINT('Ctrl Pts',(-0.661232601289069,2.17435470474185,
-17.1862644825228));
#47209=CARTESIAN_POINT('Ctrl Pts',(-0.661229808429,2.17434774916163,-17.504987389934));
#47210=CARTESIAN_POINT('Ctrl Pts',(-0.661229375315021,2.17434446174097,
-17.6291628974737));
#47211=CARTESIAN_POINT('Ctrl Pts',(-0.661231038625573,2.17433502257422,
-17.8787952656615));
#47212=CARTESIAN_POINT('Ctrl Pts',(-0.661236308189677,2.17431832730332,
-18.1280903669047));
#47213=CARTESIAN_POINT('Ctrl Pts',(-0.661245023730644,2.17430181783555,
-18.3777490651285));
#47214=CARTESIAN_POINT('Ctrl Pts',(-0.661251840931363,2.17429020416771,
-18.5337827354254));
#47215=CARTESIAN_POINT('Ctrl Pts',(-0.66125807792693,2.17428113906084,-18.6586623836088));
#47216=CARTESIAN_POINT('Ctrl Pts',(-0.661263144357075,2.17427422324021,
-18.7523327597983));
#47217=CARTESIAN_POINT('Ctrl Pts',(-0.661267684128452,2.17426842469942,
-18.8304068037653));
#47218=CARTESIAN_POINT('Ctrl Pts',(-0.661271499064604,2.17426388385676,
-18.8928736980894));
#47219=CARTESIAN_POINT('Ctrl Pts',(-0.661304869403966,2.17422491496471,
-19.4238879371911));
#47220=CARTESIAN_POINT('Ctrl Pts',(-0.661408696326335,2.1741421121425,-20.4404752420419));
#47221=CARTESIAN_POINT('Ctrl Pts',(-0.661612851666169,2.17427137833039,
-21.9466489991897));
#47222=CARTESIAN_POINT('Ctrl Pts',(-0.661780504171708,2.17465166882404,
-22.9542604711863));
#47223=CARTESIAN_POINT('Ctrl Pts',(-0.661879102679922,2.17503052377509,
-23.5834625714101));
#47224=CARTESIAN_POINT('Ctrl Pts',(-0.661919681293023,2.17520111792069,
-23.8324682152386));
#47225=CARTESIAN_POINT('Ctrl Pts',(-0.662010577041759,2.17561554973492,
-24.3313537864961));
#47226=CARTESIAN_POINT('Ctrl Pts',(-0.662187905112522,2.17650319209165,
-25.2064036746852));
#47227=CARTESIAN_POINT('Ctrl Pts',(-0.662493004231223,2.17811119590231,
-26.4607956985645));
#47228=CARTESIAN_POINT('Ctrl Pts',(-0.662845425188931,2.1800960472974,-27.969739115956));
#47229=CARTESIAN_POINT('Ctrl Pts',(-0.663056991857019,2.18117899739333,
-28.9745709795876));
#47230=CARTESIAN_POINT('Ctrl Pts',(-0.663146177495585,2.18161630695882,
-29.5402963951528));
#47231=CARTESIAN_POINT('Ctrl Pts',(-0.663174331064102,2.18110727130679,
-29.6807158367692));
#47232=CARTESIAN_POINT('Ctrl Pts',(-0.663261355597737,2.17788395250686,
-29.9507176610373));
#47233=CARTESIAN_POINT('Ctrl Pts',(-0.663488486205343,2.16718741222019,
-30.4216090598993));
#47234=CARTESIAN_POINT('Ctrl Pts',(-0.664171713171707,2.13081229108742,
-31.3364747557897));
#47235=CARTESIAN_POINT('Ctrl Pts',(-0.665424904517377,2.06516675737071,
-32.5775794288945));
#47236=CARTESIAN_POINT('Ctrl Pts',(-0.665939168101847,2.04682008967083,
-33.724921159572));
#47237=CARTESIAN_POINT('Ctrl Pts',(-0.665151885456072,2.08990577602317,
-34.5863090658768));
#47238=CARTESIAN_POINT('Ctrl Pts',(-0.664231052307106,2.13458516649471,
-34.9988077951298));
#47239=CARTESIAN_POINT('Ctrl Pts',(-0.663286717012051,2.17810461561118,
-35.3021916075847));
#47240=CARTESIAN_POINT('Ctrl Pts',(-0.662504202219517,2.20886847117035,
-35.4831201754591));
#47241=CARTESIAN_POINT('Ctrl Pts',(-0.660573758768274,2.29385816431863,
-35.879283915027));
#47242=CARTESIAN_POINT('Ctrl Pts',(-0.656358451963326,2.49604065491868,
-36.6124714084662));
#47243=CARTESIAN_POINT('Ctrl Pts',(-0.646125278213893,3.07686033436265,
-38.2580869723516));
#47244=CARTESIAN_POINT('Ctrl Pts',(-0.637514600615515,3.69735238323864,
-39.9207196729455));
#47245=CARTESIAN_POINT('Ctrl Pts',(-0.634131214466014,3.94947125472227,
-41.5084348507479));
#47246=CARTESIAN_POINT('Ctrl Pts',(-0.633299524802236,4.00082265203612,
-41.9436263914889));
#47247=CARTESIAN_POINT('Ctrl Pts',(-0.632497763223773,4.04390306304625,
-42.5232040466185));
#47248=CARTESIAN_POINT('Ctrl Pts',(-0.631877942908767,4.07091687109544,
-43.0884028834181));
#47249=CARTESIAN_POINT('Ctrl Pts',(-0.631403866133522,4.08143863771991,
-43.7759368949309));
#47250=CARTESIAN_POINT('Ctrl Pts',(-0.631173823256158,4.07251593555644,
-44.5664798657698));
#47251=CARTESIAN_POINT('Ctrl Pts',(-0.631144921188736,4.05940256355705,
-45.1974103929395));
#47252=CARTESIAN_POINT('Ctrl Pts',(-0.631151658052729,4.0516753068334,-45.6846131613201));
#47253=CARTESIAN_POINT('Ctrl Pts',(-0.631151885609456,4.04874981742623,
-46.0413830804863));
#47254=CARTESIAN_POINT('Ctrl Pts',(-0.63112949477881,4.05001188630386,-46.3892896948824));
#47255=CARTESIAN_POINT('Ctrl Pts',(-0.631047652199094,4.05887470331206,
-46.8414111240637));
#47256=CARTESIAN_POINT('Ctrl Pts',(-0.630894301455481,4.0753520081225,-47.1669327535106));
#47257=CARTESIAN_POINT('Ctrl Pts',(-0.630651332879306,4.10039201692055,
-47.4856239270558));
#47258=CARTESIAN_POINT('Ctrl Pts',(-0.630487551701003,4.12096948175222,
-47.7467517270561));
#47259=CARTESIAN_POINT('Ctrl Pts',(-0.630154495654072,4.16053412003427,
-48.2386420047998));
#47260=CARTESIAN_POINT('Ctrl Pts',(-0.62956310707126,4.23372113623803,-49.1053130915966));
#47261=CARTESIAN_POINT('Ctrl Pts',(-0.628705658823615,4.35357045286472,
-50.3117921743022));
#47262=CARTESIAN_POINT('Ctrl Pts',(-0.627777228097765,4.54650043282676,
-51.7260360891742));
#47263=CARTESIAN_POINT('Ctrl Pts',(-0.627265563061771,4.72202453586099,
-52.6426923320876));
#47264=CARTESIAN_POINT('Ctrl Pts',(-0.627007232715583,4.85111897731866,
-53.21028566008));
#47265=CARTESIAN_POINT('Ctrl Pts',(-0.626905395879994,4.90637750017685,
-53.4456175769788));
#47266=CARTESIAN_POINT('Ctrl Pts',(-0.626712820260931,5.02326501300372,
-53.9146294532301));
#47267=CARTESIAN_POINT('Ctrl Pts',(-0.626400013410281,5.2463741033518,-54.740988576581));
#47268=CARTESIAN_POINT('Ctrl Pts',(-0.625884681626927,5.76048931055464,
-56.4037876031312));
#47269=CARTESIAN_POINT('Ctrl Pts',(-0.625628602711532,6.30290639745082,
-57.8383262442653));
#47270=CARTESIAN_POINT('Ctrl Pts',(-0.62556760393444,6.71972642508893,-58.8477735636256));
#47271=CARTESIAN_POINT('Ctrl Pts',(-0.625565074343473,6.76770295818769,
-58.9624515883609));
#47272=CARTESIAN_POINT('Ctrl Pts',(-0.625564963139768,6.86841667036773,
-59.1975883170748));
#47273=CARTESIAN_POINT('Ctrl Pts',(-0.625582440524659,7.05087714573764,
-59.6095610877));
#47274=CARTESIAN_POINT('Ctrl Pts',(-0.625673206560115,7.44292862931509,
-60.4455864505415));
#47275=CARTESIAN_POINT('Ctrl Pts',(-0.625872074682469,7.93968636878086,
-61.4186616931697));
#47276=CARTESIAN_POINT('Ctrl Pts',(-0.626087693556141,8.46255259730151,
-62.4041259227318));
#47277=CARTESIAN_POINT('Ctrl Pts',(-0.626202559137751,8.76183196942706,
-62.9619931718646));
#47278=CARTESIAN_POINT('Ctrl Pts',(-0.626271105041649,8.96166958627571,
-63.3351844249496));
#47279=CARTESIAN_POINT('Ctrl Pts',(-0.626314051407471,9.09485393613067,
-63.5843109543157));
#47280=CARTESIAN_POINT('Ctrl Pts',(-0.626353422975541,9.22776053699843,
-63.8338747428221));
#47281=CARTESIAN_POINT('Ctrl Pts',(-0.626382660366308,9.34351472712429,
-64.0526621517202));
#47282=CARTESIAN_POINT('Ctrl Pts',(-0.626397882303084,9.40945620428944,
-64.1777992852074));
#47283=CARTESIAN_POINT('Ctrl Pts',(-0.626419095447353,9.50813458955278,
-64.3656076235132));
#47284=CARTESIAN_POINT('Ctrl Pts',(-0.626433803134328,9.58985026494963,
-64.5223724391017));
#47285=CARTESIAN_POINT('Ctrl Pts',(-0.62645237198052,9.72404424936194,-64.781963414885));
#47286=CARTESIAN_POINT('Ctrl Pts',(-0.626469427968082,9.85472875964012,
-65.0338821160099));
#47287=CARTESIAN_POINT('Ctrl Pts',(-0.62649494875858,10.120500285871,-65.5430168405376));
#47288=CARTESIAN_POINT('Ctrl Pts',(-0.626521563386984,10.583108636538,-66.4216051356352));
#47289=CARTESIAN_POINT('Ctrl Pts',(-0.626514660886955,11.5106242457288,
-68.159752861177));
#47290=CARTESIAN_POINT('Ctrl Pts',(-0.626471931535449,12.3083591820501,
-69.6383321739738));
#47291=CARTESIAN_POINT('Ctrl Pts',(-0.626475713088361,12.9116431096455,
-70.772934983678));
#47292=CARTESIAN_POINT('Ctrl Pts',(-0.62647610542718,13.0448906637832,-71.0235337534905));
#47293=CARTESIAN_POINT('Ctrl Pts',(-0.626476804845756,13.3119713946603,
-71.5258349837059));
#47294=CARTESIAN_POINT('Ctrl Pts',(-0.626477660859164,13.6453459070808,
-72.1528203904278));
#47295=CARTESIAN_POINT('Ctrl Pts',(-0.626477922591584,14.0453617548795,
-72.9051416022612));
#47296=CARTESIAN_POINT('Ctrl Pts',(-0.626477840681796,14.8450070813496,
-74.4090625301667));
#47297=CARTESIAN_POINT('Ctrl Pts',(-0.626478397258742,15.5109489945228,
-75.6615364417598));
#47298=CARTESIAN_POINT('Ctrl Pts',(-0.626479385432316,16.4806784860373,
-77.4853378891171));
#47299=CARTESIAN_POINT('Ctrl Pts',(-0.626479894410933,16.9171548624124,
-78.306233408562));
#47300=CARTESIAN_POINT('Ctrl Pts',(-0.626479894410927,17.3536764498018,
-79.1272111106602));
#47301=CARTESIAN_POINT('Ctrl Pts',(1.87947659458304,4.08007594746654,24.8306348252651));
#47302=CARTESIAN_POINT('Ctrl Pts',(1.87948221099211,4.08007594968897,24.7817555155472));
#47303=CARTESIAN_POINT('Ctrl Pts',(1.87948805643874,4.08007595214576,24.7328769635291));
#47304=CARTESIAN_POINT('Ctrl Pts',(1.87955912761084,4.08007597527773,24.1822788856086));
#47305=CARTESIAN_POINT('Ctrl Pts',(1.87962507094508,4.08007601162104,23.1782268448629));
#47306=CARTESIAN_POINT('Ctrl Pts',(1.87975055067327,4.08007620678542,21.1696372570538));
#47307=CARTESIAN_POINT('Ctrl Pts',(1.88024483547882,4.08007630445103,19.6656915530713));
#47308=CARTESIAN_POINT('Ctrl Pts',(1.88124023009051,4.08007640018488,18.4147329928714));
#47309=CARTESIAN_POINT('Ctrl Pts',(1.88171316333228,4.08007647531142,17.9119306359609));
#47310=CARTESIAN_POINT('Ctrl Pts',(1.88290437608708,4.08007669263161,16.9079997217721));
#47311=CARTESIAN_POINT('Ctrl Pts',(1.88544967491957,4.08007715433846,15.1542504685811));
#47312=CARTESIAN_POINT('Ctrl Pts',(1.88793047536297,4.08007721488852,13.6529777849061));
#47313=CARTESIAN_POINT('Ctrl Pts',(1.88947377904792,4.08007674283328,12.3987229743159));
#47314=CARTESIAN_POINT('Ctrl Pts',(1.8901022907834,4.08007652487329,11.8978285550643));
#47315=CARTESIAN_POINT('Ctrl Pts',(1.89136530752485,4.08007577694653,10.8960528593377));
#47316=CARTESIAN_POINT('Ctrl Pts',(1.89299043191257,4.08007482542856,9.64386894862191));
#47317=CARTESIAN_POINT('Ctrl Pts',(1.89465944971945,4.08007271810909,8.13988290786252));
#47318=CARTESIAN_POINT('Ctrl Pts',(1.8955778547512,4.0800729105106,7.13531874534234));
#47319=CARTESIAN_POINT('Ctrl Pts',(1.89598038811047,4.08007012513435,6.50868913529077));
#47320=CARTESIAN_POINT('Ctrl Pts',(1.89601487495568,4.0820814863956,6.28703299979524));
#47321=CARTESIAN_POINT('Ctrl Pts',(1.89567557410536,4.09284104044257,5.81687291560801));
#47322=CARTESIAN_POINT('Ctrl Pts',(1.89432085510484,4.12624777332536,4.97722214089179));
#47323=CARTESIAN_POINT('Ctrl Pts',(1.88997973046473,4.21956716125387,3.19436157629692));
#47324=CARTESIAN_POINT('Ctrl Pts',(1.89051464550626,4.2274313393854,1.50818455468003));
#47325=CARTESIAN_POINT('Ctrl Pts',(1.89814047422308,4.04814526942004,0.24558502820507));
#47326=CARTESIAN_POINT('Ctrl Pts',(1.89909636332055,4.02306735979135,0.0837071483672661));
#47327=CARTESIAN_POINT('Ctrl Pts',(1.90131393495655,3.96710837696693,-0.227949918977011));
#47328=CARTESIAN_POINT('Ctrl Pts',(1.90587879504138,3.85255773904514,-0.764156068895517));
#47329=CARTESIAN_POINT('Ctrl Pts',(1.91420954102354,3.65323868491061,-1.49269331038278));
#47330=CARTESIAN_POINT('Ctrl Pts',(1.92566809001345,3.38408538280297,-2.31724895313642));
#47331=CARTESIAN_POINT('Ctrl Pts',(1.94250971673815,3.01590503454656,-3.35448813837129));
#47332=CARTESIAN_POINT('Ctrl Pts',(1.96404049201351,2.5907524101948,-4.543864836452));
#47333=CARTESIAN_POINT('Ctrl Pts',(1.97858408945532,2.37892223453074,-5.36738331377946));
#47334=CARTESIAN_POINT('Ctrl Pts',(1.98431559394949,2.301777985992,-5.83505938258291));
#47335=CARTESIAN_POINT('Ctrl Pts',(1.98619310963592,2.26812487877299,-6.05774566153013));
#47336=CARTESIAN_POINT('Ctrl Pts',(1.98933774331585,2.21443117732476,-6.48999499635696));
#47337=CARTESIAN_POINT('Ctrl Pts',(1.99312146425114,2.14417478968173,-7.27282828987392));
#47338=CARTESIAN_POINT('Ctrl Pts',(1.99484765517173,2.10508432184969,-8.43371821930893));
#47339=CARTESIAN_POINT('Ctrl Pts',(1.99424722760277,2.10829809461501,-9.6613988767828));
#47340=CARTESIAN_POINT('Ctrl Pts',(1.99381843790417,2.10921397899,-10.5516621456655));
#47341=CARTESIAN_POINT('Ctrl Pts',(1.99377849010985,2.10534531638977,-11.0696232807361));
#47342=CARTESIAN_POINT('Ctrl Pts',(1.99385757119846,2.10129650540405,-11.3316723035792));
#47343=CARTESIAN_POINT('Ctrl Pts',(1.99396021712955,2.09718960351093,-11.5297803969733));
#47344=CARTESIAN_POINT('Ctrl Pts',(1.99402955970695,2.09486460711147,-11.6494722329179));
#47345=CARTESIAN_POINT('Ctrl Pts',(1.99412849328614,2.09065807860872,-11.8964705807442));
#47346=CARTESIAN_POINT('Ctrl Pts',(1.99422975986236,2.08487238506963,-12.3250611021437));
#47347=CARTESIAN_POINT('Ctrl Pts',(1.99420175990704,2.07861770114086,-13.1860047724658));
#47348=CARTESIAN_POINT('Ctrl Pts',(1.99355029263019,2.08171997518577,-14.4196756638712));
#47349=CARTESIAN_POINT('Ctrl Pts',(1.99277695148483,2.09042777614687,-15.5426265039093));
#47350=CARTESIAN_POINT('Ctrl Pts',(1.99239862064165,2.09506734930592,-16.2983011418255));
#47351=CARTESIAN_POINT('Ctrl Pts',(1.99218242082944,2.09760234861235,-16.8041858254556));
#47352=CARTESIAN_POINT('Ctrl Pts',(1.99212726152234,2.09857751742776,-17.1860629660676));
#47353=CARTESIAN_POINT('Ctrl Pts',(1.99212324243369,2.09857411333236,-17.5049672230762));
#47354=CARTESIAN_POINT('Ctrl Pts',(1.99212260694304,2.09857258119165,-17.629102871608));
#47355=CARTESIAN_POINT('Ctrl Pts',(1.99212711575014,2.09856799767051,-17.8787244471707));
#47356=CARTESIAN_POINT('Ctrl Pts',(1.99214707955899,2.09855884278737,-18.1279914322703));
#47357=CARTESIAN_POINT('Ctrl Pts',(1.99217121064863,2.09854993548065,-18.3776388365096));
#47358=CARTESIAN_POINT('Ctrl Pts',(1.99219109351607,2.09854343429611,-18.5336651340886));
#47359=CARTESIAN_POINT('Ctrl Pts',(1.99220833699324,2.09853830249942,-18.6585410991645));
#47360=CARTESIAN_POINT('Ctrl Pts',(1.99222244021897,2.09853432338726,-18.7522091484825));
#47361=CARTESIAN_POINT('Ctrl Pts',(1.99223512176153,2.09853093513328,-18.8302819559127));
#47362=CARTESIAN_POINT('Ctrl Pts',(1.9922456377348,2.09852824720193,-18.8927481245961));
#47363=CARTESIAN_POINT('Ctrl Pts',(1.99233906194416,2.09850488269869,-19.423758499618));
#47364=CARTESIAN_POINT('Ctrl Pts',(1.99263748504989,2.09845420519683,-20.4404115015207));
#47365=CARTESIAN_POINT('Ctrl Pts',(1.99324071658104,2.0984714180227,-21.9468464155744));
#47366=CARTESIAN_POINT('Ctrl Pts',(1.99372053067635,2.09861418681217,-22.9547557228035));
#47367=CARTESIAN_POINT('Ctrl Pts',(1.99402170436847,2.0987614672874,-23.5841774312742));
#47368=CARTESIAN_POINT('Ctrl Pts',(1.99414888338287,2.09882784153572,-23.8333094826695));
#47369=CARTESIAN_POINT('Ctrl Pts',(1.99442808139027,2.09899124156944,-24.3323927034768));
#47370=CARTESIAN_POINT('Ctrl Pts',(1.9949894335052,2.09934240565073,-25.207726496462));
#47371=CARTESIAN_POINT('Ctrl Pts',(1.99586532682244,2.09998984977607,-26.4623110682351));
#47372=CARTESIAN_POINT('Ctrl Pts',(1.99696734244082,2.10077165076235,-27.9711556415455));
#47373=CARTESIAN_POINT('Ctrl Pts',(1.99748202186661,2.10120441087972,-28.9756868843356));
#47374=CARTESIAN_POINT('Ctrl Pts',(1.99773809301026,2.10137348076256,-29.5412243672071));
#47375=CARTESIAN_POINT('Ctrl Pts',(1.99782461908708,2.10077377950784,-29.6822068893583));
#47376=CARTESIAN_POINT('Ctrl Pts',(1.99809062042496,2.09727817819766,-29.9528940217472));
#47377=CARTESIAN_POINT('Ctrl Pts',(1.99876117898229,2.08588995074677,-30.424934709598));
#47378=CARTESIAN_POINT('Ctrl Pts',(2.00080463385646,2.04753260577408,-31.341042499164));
#47379=CARTESIAN_POINT('Ctrl Pts',(2.00443833713365,1.97863167455129,-32.5814847638249));
#47380=CARTESIAN_POINT('Ctrl Pts',(2.00575704994606,1.95924823295857,-33.7247553979965));
#47381=CARTESIAN_POINT('Ctrl Pts',(2.00310055141625,2.00388697303159,-34.5808237926425));
#47382=CARTESIAN_POINT('Ctrl Pts',(1.99994623957741,2.05019955009036,-34.9900584642322));
#47383=CARTESIAN_POINT('Ctrl Pts',(1.99683464745504,2.0952884493422,-35.2907818633749));
#47384=CARTESIAN_POINT('Ctrl Pts',(1.99420955065897,2.12704744684203,-35.4691589148058));
#47385=CARTESIAN_POINT('Ctrl Pts',(1.98793892913517,2.215006136549,-35.8616030816837));
#47386=CARTESIAN_POINT('Ctrl Pts',(1.9741086581221,2.42449271247474,-36.5899729258883));
#47387=CARTESIAN_POINT('Ctrl Pts',(1.94235791924633,3.02780501619578,-38.2325436184006));
#47388=CARTESIAN_POINT('Ctrl Pts',(1.91493319356227,3.67522197999023,-39.8980747271658));
#47389=CARTESIAN_POINT('Ctrl Pts',(1.90390518409755,3.93974100445547,-41.4977896434242));
#47390=CARTESIAN_POINT('Ctrl Pts',(1.90123344083393,3.99355337234143,-41.9345096696509));
#47391=CARTESIAN_POINT('Ctrl Pts',(1.89871335543755,4.03909746335217,-42.5167344189122));
#47392=CARTESIAN_POINT('Ctrl Pts',(1.89673229126996,4.06787736429817,-43.0840821363168));
#47393=CARTESIAN_POINT('Ctrl Pts',(1.89519489619482,4.07966267988032,-43.7738675543103));
#47394=CARTESIAN_POINT('Ctrl Pts',(1.89438522140316,4.07124691226921,-44.5661414710187));
#47395=CARTESIAN_POINT('Ctrl Pts',(1.89418118018047,4.05812745696965,-45.1977774831885));
#47396=CARTESIAN_POINT('Ctrl Pts',(1.8941899847956,4.05035676149492,-45.6851056130695));
#47397=CARTESIAN_POINT('Ctrl Pts',(1.89417050151014,4.04740249946183,-46.0417443946409));
#47398=CARTESIAN_POINT('Ctrl Pts',(1.89407717984001,4.04867558437408,-46.3892911665539));
#47399=CARTESIAN_POINT('Ctrl Pts',(1.89380533637415,4.0576506306873,-46.8406378683643));
#47400=CARTESIAN_POINT('Ctrl Pts',(1.89326484112894,4.07433109677534,-47.16522580503));
#47401=CARTESIAN_POINT('Ctrl Pts',(1.89248217238794,4.0997139568233,-47.4828054835067));
#47402=CARTESIAN_POINT('Ctrl Pts',(1.89195427391836,4.12065987577668,-47.7440998580142));
#47403=CARTESIAN_POINT('Ctrl Pts',(1.8908787918323,4.16089174064189,-48.235845718434));
#47404=CARTESIAN_POINT('Ctrl Pts',(1.88894392970756,4.23527963439326,-49.1026062613519));
#47405=CARTESIAN_POINT('Ctrl Pts',(1.88608565034801,4.35671213750319,-50.3092845028095));
#47406=CARTESIAN_POINT('Ctrl Pts',(1.88303048014428,4.55121233841588,-51.7242608361643));
#47407=CARTESIAN_POINT('Ctrl Pts',(1.88135443518853,4.7274313373995,-52.6416057279167));
#47408=CARTESIAN_POINT('Ctrl Pts',(1.88053521133268,4.85684152954458,-53.2096995393921));
#47409=CARTESIAN_POINT('Ctrl Pts',(1.88021774466022,4.91221706540757,-53.4452444549671));
#47410=CARTESIAN_POINT('Ctrl Pts',(1.87962430010965,5.02926173532985,-53.9146251526131));
#47411=CARTESIAN_POINT('Ctrl Pts',(1.87867687116386,5.25246543255048,-54.7415196101994));
#47412=CARTESIAN_POINT('Ctrl Pts',(1.87717820026664,5.76616052127753,-56.4049580061723));
#47413=CARTESIAN_POINT('Ctrl Pts',(1.87653737221588,6.30754371972887,-57.839407555238));
#47414=CARTESIAN_POINT('Ctrl Pts',(1.87640334479534,6.72375863927511,-58.8485669790888));
#47415=CARTESIAN_POINT('Ctrl Pts',(1.87640011896581,6.77169968585435,-58.9632945249556));
#47416=CARTESIAN_POINT('Ctrl Pts',(1.87640981753854,6.87230907632589,-59.1984753526718));
#47417=CARTESIAN_POINT('Ctrl Pts',(1.87648229107633,7.05457266535652,-59.6105336799863));
#47418=CARTESIAN_POINT('Ctrl Pts',(1.87680035709759,7.44612737564027,-60.4466524112431));
#47419=CARTESIAN_POINT('Ctrl Pts',(1.87746091747657,7.94216601405338,-61.4197358246611));
#47420=CARTESIAN_POINT('Ctrl Pts',(1.87816443196974,8.46426789803593,-62.4051128652444));
#47421=CARTESIAN_POINT('Ctrl Pts',(1.87853578964412,8.76312548481773,-62.9628970204466));
#47422=CARTESIAN_POINT('Ctrl Pts',(1.87875745517044,8.96269469371772,-63.3360167182748));
#47423=CARTESIAN_POINT('Ctrl Pts',(1.87889594354275,9.09570400878161,-63.5850910655754));
#47424=CARTESIAN_POINT('Ctrl Pts',(1.87902391190774,9.22844354699239,-63.8345960668322));
#47425=CARTESIAN_POINT('Ctrl Pts',(1.87911865784649,9.34405909156172,-64.0533253020349));
#47426=CARTESIAN_POINT('Ctrl Pts',(1.87916810345619,9.40992390351972,-64.1784272248205));
#47427=CARTESIAN_POINT('Ctrl Pts',(1.87923707273549,9.50848992668408,-64.3661807228412));
#47428=CARTESIAN_POINT('Ctrl Pts',(1.87928562178054,9.59011831493283,-64.5228957103385));
#47429=CARTESIAN_POINT('Ctrl Pts',(1.87934726761746,9.72417672732782,-64.7823979902518));
#47430=CARTESIAN_POINT('Ctrl Pts',(1.87940408839605,9.85474818543953,-65.0342463738239));
#47431=CARTESIAN_POINT('Ctrl Pts',(1.87948883825274,10.1203301393946,-65.5432435490755));
#47432=CARTESIAN_POINT('Ctrl Pts',(1.87957813188275,10.5827220547072,-66.4216332770441));
#47433=CARTESIAN_POINT('Ctrl Pts',(1.87955592502107,11.5101601419476,-68.1595288613347));
#47434=CARTESIAN_POINT('Ctrl Pts',(1.87941633705314,12.308181502804,-69.638170043014));
#47435=CARTESIAN_POINT('Ctrl Pts',(1.87942945470135,12.9115548163983,-70.7729484576077));
#47436=CARTESIAN_POINT('Ctrl Pts',(1.87943072721303,13.0447945853888,-71.023534534485));
#47437=CARTESIAN_POINT('Ctrl Pts',(1.87943305073928,13.3118762099186,-71.5258401738176));
#47438=CARTESIAN_POINT('Ctrl Pts',(1.87943606223055,13.6452469615933,-72.1528197111203));
#47439=CARTESIAN_POINT('Ctrl Pts',(1.8794370299544,14.0452627075202,-72.9051406045083));
#47440=CARTESIAN_POINT('Ctrl Pts',(1.8794369920951,14.8449078780946,-74.4090580719077));
#47441=CARTESIAN_POINT('Ctrl Pts',(1.87943984359169,15.5108551515139,-75.6615338419008));
#47442=CARTESIAN_POINT('Ctrl Pts',(1.87944367170075,16.4805874064928,-77.4853389352122));
#47443=CARTESIAN_POINT('Ctrl Pts',(1.87944564302009,16.9170636542885,-78.3062334138863));
#47444=CARTESIAN_POINT('Ctrl Pts',(1.8794456430201,17.3535852416779,-79.1272111159846));
#47445=CARTESIAN_POINT('Ctrl Pts',(4.38536333748957,4.07987500441129,24.8306345674609));
#47446=CARTESIAN_POINT('Ctrl Pts',(4.38537644142124,4.07987499919676,24.7817552497562));
#47447=CARTESIAN_POINT('Ctrl Pts',(4.38539019131228,4.07987502084466,24.7328766839669));
#47448=CARTESIAN_POINT('Ctrl Pts',(4.38555225646271,4.07987404404021,24.1822787020537));
#47449=CARTESIAN_POINT('Ctrl Pts',(4.3856747483447,4.07986630447217,23.1782281351487));
#47450=CARTESIAN_POINT('Ctrl Pts',(4.38596401523434,4.07986513301286,21.1696385469548));
#47451=CARTESIAN_POINT('Ctrl Pts',(4.38703941713429,4.07984579442867,19.6656967303803));
#47452=CARTESIAN_POINT('Ctrl Pts',(4.3893281034198,4.07983704306533,18.4147398652079));
#47453=CARTESIAN_POINT('Ctrl Pts',(4.39042640426722,4.07983550220427,17.9119372926431));
#47454=CARTESIAN_POINT('Ctrl Pts',(4.39318382647735,4.07982939511974,16.9080071514512));
#47455=CARTESIAN_POINT('Ctrl Pts',(4.39909969012431,4.07982219497109,15.1542591595331));
#47456=CARTESIAN_POINT('Ctrl Pts',(4.40471075664177,4.07977796237531,13.6529969540059));
#47457=CARTESIAN_POINT('Ctrl Pts',(4.40822987883419,4.07975814035652,12.3987485900475));
#47458=CARTESIAN_POINT('Ctrl Pts',(4.40966888530907,4.07975160201974,11.8978553946956));
#47459=CARTESIAN_POINT('Ctrl Pts',(4.41260517655036,4.07974945549079,10.8960846994662));
#47460=CARTESIAN_POINT('Ctrl Pts',(4.41622620052564,4.07970917257484,9.64390133458129));
#47461=CARTESIAN_POINT('Ctrl Pts',(4.42005210494712,4.07969335842138,8.13994421962362));
#47462=CARTESIAN_POINT('Ctrl Pts',(4.42192997405278,4.07963098116463,7.13534735212569));
#47463=CARTESIAN_POINT('Ctrl Pts',(4.42280559066173,4.07961328863103,6.50881337281083));
#47464=CARTESIAN_POINT('Ctrl Pts',(4.42293307896198,4.08176225758811,6.28940021210922));
#47465=CARTESIAN_POINT('Ctrl Pts',(4.42244849043344,4.0932928132071,5.82167475603086));
#47466=CARTESIAN_POINT('Ctrl Pts',(4.4200863997875,4.12915550142465,4.9849811635924));
#47467=CARTESIAN_POINT('Ctrl Pts',(4.41241717172237,4.22980045467592,3.2004838586177));
#47468=CARTESIAN_POINT('Ctrl Pts',(4.41204017706113,4.23846381586494,1.49941031600799));
#47469=CARTESIAN_POINT('Ctrl Pts',(4.42494515964956,4.04271426178755,0.221825490814583));
#47470=CARTESIAN_POINT('Ctrl Pts',(4.42661641531885,4.0152420162272,0.0573597170611306));
#47471=CARTESIAN_POINT('Ctrl Pts',(4.4304302399912,3.9540711684284,-0.258476534902446));
#47472=CARTESIAN_POINT('Ctrl Pts',(4.43823658554011,3.82901928023654,-0.801066190085443));
#47473=CARTESIAN_POINT('Ctrl Pts',(4.45194015309164,3.61203368465594,-1.53552136893551));
#47474=CARTESIAN_POINT('Ctrl Pts',(4.47106293497066,3.3199525683178,-2.36372384087933));
#47475=CARTESIAN_POINT('Ctrl Pts',(4.49864317522206,2.92101932090935,-3.40223334408898));
#47476=CARTESIAN_POINT('Ctrl Pts',(4.53542070388085,2.46108360630587,-4.58820248705211));
#47477=CARTESIAN_POINT('Ctrl Pts',(4.56191929905351,2.23372943426866,-5.40116324087532));
#47478=CARTESIAN_POINT('Ctrl Pts',(4.57315509374485,2.15171291670083,-5.85772518827808));
#47479=CARTESIAN_POINT('Ctrl Pts',(4.57670152996441,2.11547655848202,-6.07836468920828));
#47480=CARTESIAN_POINT('Ctrl Pts',(4.582716130402,2.05783159343524,-6.50551317008511));
#47481=CARTESIAN_POINT('Ctrl Pts',(4.58968617993058,1.98221611247772,-7.28107077938575));
#47482=CARTESIAN_POINT('Ctrl Pts',(4.59211110960528,1.9400984689788,-8.43457496086372));
#47483=CARTESIAN_POINT('Ctrl Pts',(4.59006804493711,1.94376555103631,-9.66013921101102));
#47484=CARTESIAN_POINT('Ctrl Pts',(4.58898801115239,1.94494955250666,-10.5515189657516));
#47485=CARTESIAN_POINT('Ctrl Pts',(4.58876503502354,1.94083551824235,-11.0708986295732));
#47486=CARTESIAN_POINT('Ctrl Pts',(4.5888378182298,1.93647095036939,-11.3339173258097));
#47487=CARTESIAN_POINT('Ctrl Pts',(4.58898044581554,1.9320289308661,-11.5328241242325));
#47488=CARTESIAN_POINT('Ctrl Pts',(4.58909258905083,1.92953498247887,-11.6520206994036));
#47489=CARTESIAN_POINT('Ctrl Pts',(4.58923477242463,1.92501889552757,-11.8986379229506));
#47490=CARTESIAN_POINT('Ctrl Pts',(4.58933380737592,1.91883182976867,-12.3263335876568));
#47491=CARTESIAN_POINT('Ctrl Pts',(4.5889612591559,1.91221848125152,-13.1859475603198));
#47492=CARTESIAN_POINT('Ctrl Pts',(4.587318679081,1.9158525167072,-14.418398477512));
#47493=CARTESIAN_POINT('Ctrl Pts',(4.5855655965159,1.92551125242793,-15.5412749212642));
#47494=CARTESIAN_POINT('Ctrl Pts',(4.58471565917111,1.93064565913078,-16.2972959138459));
#47495=CARTESIAN_POINT('Ctrl Pts',(4.58426483520442,1.93345284275731,-16.8035285788579));
#47496=CARTESIAN_POINT('Ctrl Pts',(4.58407707180408,1.93452735537964,-17.1857733190268));
#47497=CARTESIAN_POINT('Ctrl Pts',(4.5840470977447,1.93452805010875,-17.5050472253787));
#47498=CARTESIAN_POINT('Ctrl Pts',(4.58403936442119,1.93452939854136,-17.629109521674));
#47499=CARTESIAN_POINT('Ctrl Pts',(4.58403953885549,1.93453465720278,-17.878721089651));
#47500=CARTESIAN_POINT('Ctrl Pts',(4.58406047028114,1.93453815462779,-18.1279372137167));
#47501=CARTESIAN_POINT('Ctrl Pts',(4.58410385317871,1.93454639285833,-18.3775718376653));
#47502=CARTESIAN_POINT('Ctrl Pts',(4.58413908782597,1.9345510030292,-18.5335880862641));
#47503=CARTESIAN_POINT('Ctrl Pts',(4.58417245068831,1.93455529671514,-18.6584611447923));
#47504=CARTESIAN_POINT('Ctrl Pts',(4.58419984423577,1.93455840446897,-18.7521276726347));
#47505=CARTESIAN_POINT('Ctrl Pts',(4.58422461966875,1.93456089354058,-18.8302004655324));
#47506=CARTESIAN_POINT('Ctrl Pts',(4.5842456542114,1.93456293899492,-18.8926672614959));
#47507=CARTESIAN_POINT('Ctrl Pts',(4.58443082577052,1.9345792498428,-19.423686178086));
#47508=CARTESIAN_POINT('Ctrl Pts',(4.58496027623401,1.93456884799325,-20.4404491402449));
#47509=CARTESIAN_POINT('Ctrl Pts',(4.58618165970048,1.9344005047072,-21.9473837554038));
#47510=CARTESIAN_POINT('Ctrl Pts',(4.58711829273437,1.93405548562601,-22.9558218416924));
#47511=CARTESIAN_POINT('Ctrl Pts',(4.58772761688267,1.9337519453812,-23.5856474626337));
#47512=CARTESIAN_POINT('Ctrl Pts',(4.58798722362885,1.93361765012697,-23.8350334454882));
#47513=CARTESIAN_POINT('Ctrl Pts',(4.58856197923874,1.93329611518799,-24.3345016458647));
#47514=CARTESIAN_POINT('Ctrl Pts',(4.5896991750285,1.93260966205005,-25.2103932074912));
#47515=CARTESIAN_POINT('Ctrl Pts',(4.591550770956,1.93139848748939,-26.465283098573));
#47516=CARTESIAN_POINT('Ctrl Pts',(4.59382185748777,1.92990784656879,-27.9738813170967));
#47517=CARTESIAN_POINT('Ctrl Pts',(4.59507579392218,1.92914138268994,-28.9776841894854));
#47518=CARTESIAN_POINT('Ctrl Pts',(4.59565480542664,1.92882029442061,-29.5428136074289));
#47519=CARTESIAN_POINT('Ctrl Pts',(4.59582783748557,1.92803885515975,-29.684947655115));
#47520=CARTESIAN_POINT('Ctrl Pts',(4.59634175778087,1.92398854183494,-29.9570348851275));
#47521=CARTESIAN_POINT('Ctrl Pts',(4.59764796517775,1.9111777944852,-30.4314080380904));
#47522=CARTESIAN_POINT('Ctrl Pts',(4.60157654881394,1.86871729029142,-31.3500132358661));
#47523=CARTESIAN_POINT('Ctrl Pts',(4.60911287557201,1.79325708873194,-32.5889100139117));
#47524=CARTESIAN_POINT('Ctrl Pts',(4.61261035047527,1.7720747183762,-33.7234649575452));
#47525=CARTESIAN_POINT('Ctrl Pts',(4.60753754323484,1.81984412989276,-34.5684483652512));
#47526=CARTESIAN_POINT('Ctrl Pts',(4.60140294800719,1.86939920594346,-34.9709802963835));
#47527=CARTESIAN_POINT('Ctrl Pts',(4.59511193844088,1.91758874644636,-35.2664108115237));
#47528=CARTESIAN_POINT('Ctrl Pts',(4.58963954516065,1.95124546012824,-35.439790623163));
#47529=CARTESIAN_POINT('Ctrl Pts',(4.57693004491039,2.04526178261014,-35.8251973478166));
#47530=CARTESIAN_POINT('Ctrl Pts',(4.55072141029509,2.270694842524,-36.5447481259702));
#47531=CARTESIAN_POINT('Ctrl Pts',(4.49479158256959,2.92339492318843,-38.1815208936028));
#47532=CARTESIAN_POINT('Ctrl Pts',(4.45249879856879,3.62724493168932,-39.8519362779289));
#47533=CARTESIAN_POINT('Ctrl Pts',(4.43466967627358,3.91809437366026,-41.4754857864873));
#47534=CARTESIAN_POINT('Ctrl Pts',(4.43017000357502,3.97709485988986,-41.9152990727862));
#47535=CARTESIAN_POINT('Ctrl Pts',(4.425827541932,4.02777358199978,-42.5028677550952));
#47536=CARTESIAN_POINT('Ctrl Pts',(4.42246125187646,4.06027634685567,-43.0746021926373));
#47537=CARTESIAN_POINT('Ctrl Pts',(4.41989661915659,4.07476176701532,-43.7690088010663));
#47538=CARTESIAN_POINT('Ctrl Pts',(4.41868148866089,4.06753369221726,-44.5648753139305));
#47539=CARTESIAN_POINT('Ctrl Pts',(4.41855604666776,4.05457249544316,-45.1980149881577));
#47540=CARTESIAN_POINT('Ctrl Pts',(4.41856191984839,4.04673730074029,-45.6856037469499));
#47541=CARTESIAN_POINT('Ctrl Pts',(4.4185280849828,4.0437552693733,-46.0419819892028));
#47542=CARTESIAN_POINT('Ctrl Pts',(4.41835264491565,4.04508359659981,-46.3888010287877));
#47543=CARTESIAN_POINT('Ctrl Pts',(4.41778696449461,4.05430232211172,-46.8385669942812));
#47544=CARTESIAN_POINT('Ctrl Pts',(4.41685949765896,4.07147622244023,-47.1612706663254));
#47545=CARTESIAN_POINT('Ctrl Pts',(4.41536946806902,4.09757043631557,-47.4765909598496));
#47546=CARTESIAN_POINT('Ctrl Pts',(4.41435203698925,4.11929124632499,-47.7382165277383));
#47547=CARTESIAN_POINT('Ctrl Pts',(4.4122399511489,4.16093071003005,-48.2296622826269));
#47548=CARTESIAN_POINT('Ctrl Pts',(4.40839107586531,4.23790657624569,-49.0965996831726));
#47549=CARTESIAN_POINT('Ctrl Pts',(4.40271949235705,4.36296011274574,-50.303743139869));
#47550=CARTESIAN_POINT('Ctrl Pts',(4.39630422969031,4.56115621044263,-51.7202397963496));
#47551=CARTESIAN_POINT('Ctrl Pts',(4.39285149901682,4.73911963744755,-52.6390688392893));
#47552=CARTESIAN_POINT('Ctrl Pts',(4.39107069326482,4.86926846690536,-53.208222653553));
#47553=CARTESIAN_POINT('Ctrl Pts',(4.39035315731622,4.92490591277966,-53.4442090160124));
#47554=CARTESIAN_POINT('Ctrl Pts',(4.38898384735229,5.0422973626307,-53.91436147999));
#47555=CARTESIAN_POINT('Ctrl Pts',(4.38674847868596,5.2657075848358,-54.7423984527176));
#47556=CARTESIAN_POINT('Ctrl Pts',(4.38294788630294,5.77841808917209,-56.4072487986332));
#47557=CARTESIAN_POINT('Ctrl Pts',(4.38096907610789,6.31757183978602,-57.8416242539194));
#47558=CARTESIAN_POINT('Ctrl Pts',(4.38039617593613,6.73249390457944,-58.8502076860662));
#47559=CARTESIAN_POINT('Ctrl Pts',(4.38035268196383,6.78035283114945,-58.9650419437206));
#47560=CARTESIAN_POINT('Ctrl Pts',(4.38030271467523,6.88073060928624,-59.2003213018297));
#47561=CARTESIAN_POINT('Ctrl Pts',(4.38032783148236,7.06255659537741,-59.6125709230305));
#47562=CARTESIAN_POINT('Ctrl Pts',(4.38075906502676,7.45302567903753,-60.4489111504564));
#47563=CARTESIAN_POINT('Ctrl Pts',(4.3818642947659,7.94750072908113,-61.42203394979));
#47564=CARTESIAN_POINT('Ctrl Pts',(4.38312813103595,8.46796870792654,-62.4072381816166));
#47565=CARTESIAN_POINT('Ctrl Pts',(4.38381483419207,8.76593203701963,-62.9648487067993));
#47566=CARTESIAN_POINT('Ctrl Pts',(4.38422545017223,8.96493468569735,-63.3378178866081));
#47567=CARTESIAN_POINT('Ctrl Pts',(4.38448507376358,9.09757619626695,-63.5867822852778));
#47568=CARTESIAN_POINT('Ctrl Pts',(4.38471622829962,9.22996208210611,-63.836162652083));
#47569=CARTESIAN_POINT('Ctrl Pts',(4.38489057482387,9.34528683550233,-64.0547689414924));
#47570=CARTESIAN_POINT('Ctrl Pts',(4.38498080317418,9.4109909530479,-64.179796468545));
#47571=CARTESIAN_POINT('Ctrl Pts',(4.38510646844273,9.50932185593333,-64.3674341859458));
#47572=CARTESIAN_POINT('Ctrl Pts',(4.38518833568825,9.59076550330329,-64.5240432970581));
#47573=CARTESIAN_POINT('Ctrl Pts',(4.38529138354864,9.72453937360013,-64.7833581652172));
#47574=CARTESIAN_POINT('Ctrl Pts',(4.38538407252477,9.85487227307931,-65.035057292464));
#47575=CARTESIAN_POINT('Ctrl Pts',(4.38552442823488,10.1200556226403,-65.5437636921788));
#47576=CARTESIAN_POINT('Ctrl Pts',(4.3856575075042,10.5819839959435,-66.4217312990546));
#47577=CARTESIAN_POINT('Ctrl Pts',(4.38559842036056,11.5092437243743,-68.1590931464431));
#47578=CARTESIAN_POINT('Ctrl Pts',(4.38530922003596,12.3078328578379,-69.6378481640055));
#47579=CARTESIAN_POINT('Ctrl Pts',(4.38531495596378,12.9113831497213,-70.7729887387607));
#47580=CARTESIAN_POINT('Ctrl Pts',(4.3853169169871,13.0446063543478,-71.023548114357));
#47581=CARTESIAN_POINT('Ctrl Pts',(4.38531956388404,13.3116888718657,-71.525862452528));
#47582=CARTESIAN_POINT('Ctrl Pts',(4.38532013350853,13.6450490574467,-72.1528282923326));
#47583=CARTESIAN_POINT('Ctrl Pts',(4.38531970441808,14.0450633921025,-72.9051478568788));
#47584=CARTESIAN_POINT('Ctrl Pts',(4.38531587669047,14.8447062959071,-74.4090569962067));
#47585=CARTESIAN_POINT('Ctrl Pts',(4.385305149308,15.5106566049086,-75.6615323927856));
#47586=CARTESIAN_POINT('Ctrl Pts',(4.38530219686728,16.4803894785991,-77.4853425381236));
#47587=CARTESIAN_POINT('Ctrl Pts',(4.38530067674068,16.9168627416068,-78.3062334060089));
#47588=CARTESIAN_POINT('Ctrl Pts',(4.3853006767407,17.3533843289963,-79.1272111081073));
#47589=CARTESIAN_POINT('Ctrl Pts',(7.51718551955428,4.07971249010422,24.8306343608847));
#47590=CARTESIAN_POINT('Ctrl Pts',(7.51720795965804,4.07971248230645,24.7817550363318));
#47591=CARTESIAN_POINT('Ctrl Pts',(7.51723151850014,4.07971246428584,24.7328764315142));
#47592=CARTESIAN_POINT('Ctrl Pts',(7.51750862931441,4.07971269960442,24.1822794479906));
#47593=CARTESIAN_POINT('Ctrl Pts',(7.51771450023927,4.07971520126788,23.178237778938));
#47594=CARTESIAN_POINT('Ctrl Pts',(7.51820836771084,4.07971475633899,21.1696490239213));
#47595=CARTESIAN_POINT('Ctrl Pts',(7.52004122986227,4.07972100155323,19.6657295586513));
#47596=CARTESIAN_POINT('Ctrl Pts',(7.52395863738461,4.07972361209946,18.4147824381763));
#47597=CARTESIAN_POINT('Ctrl Pts',(7.52583963789275,4.07972381789213,17.9119809679059));
#47598=CARTESIAN_POINT('Ctrl Pts',(7.53056086896264,4.07972501141388,16.9080568779214));
#47599=CARTESIAN_POINT('Ctrl Pts',(7.54069280565535,4.07972549092514,15.1543155686738));
#47600=CARTESIAN_POINT('Ctrl Pts',(7.55028728769419,4.07974077033179,13.6531056527217));
#47601=CARTESIAN_POINT('Ctrl Pts',(7.55631193962428,4.07974973893671,12.3988829128982));
#47602=CARTESIAN_POINT('Ctrl Pts',(7.55877660319472,4.07975313865664,11.8979973028344));
#47603=CARTESIAN_POINT('Ctrl Pts',(7.56381238794902,4.07975664999347,10.8962342796642));
#47604=CARTESIAN_POINT('Ctrl Pts',(7.57000663770048,4.07977634071094,9.64409150183717));
#47605=CARTESIAN_POINT('Ctrl Pts',(7.57656628504353,4.07978723733203,8.14018162411911));
#47606=CARTESIAN_POINT('Ctrl Pts',(7.57976001741483,4.07981510291455,7.13561214357882));
#47607=CARTESIAN_POINT('Ctrl Pts',(7.58125680054209,4.07981937530554,6.50919565034343));
#47608=CARTESIAN_POINT('Ctrl Pts',(7.58190445541536,4.08212174401879,6.29218907834675));
#47609=CARTESIAN_POINT('Ctrl Pts',(7.58334841215747,4.09448343752714,5.82707715320434));
#47610=CARTESIAN_POINT('Ctrl Pts',(7.58603525732085,4.13307212013271,4.99360215410308));
#47611=CARTESIAN_POINT('Ctrl Pts',(7.59114415438726,4.24184534711902,3.20739308478373));
#47612=CARTESIAN_POINT('Ctrl Pts',(7.59004899911565,4.25238286087194,1.49090484084568));
#47613=CARTESIAN_POINT('Ctrl Pts',(7.58318134817281,4.03889895130787,0.197408840081295));
#47614=CARTESIAN_POINT('Ctrl Pts',(7.58231136318647,4.0087808203859,0.0301756810361527));
#47615=CARTESIAN_POINT('Ctrl Pts',(7.58031603100438,3.94191656764389,-0.290127652373105));
#47616=CARTESIAN_POINT('Ctrl Pts',(7.57625546587106,3.80547464262213,-0.839555082672826));
#47617=CARTESIAN_POINT('Ctrl Pts',(7.56912588627309,3.56998135672488,-1.58040980943646));
#47618=CARTESIAN_POINT('Ctrl Pts',(7.55942200879824,3.25483991395464,-2.41305020166659));
#47619=CARTESIAN_POINT('Ctrl Pts',(7.54501194597211,2.82737969524278,-3.4543956916464));
#47620=CARTESIAN_POINT('Ctrl Pts',(7.52463208509811,2.33996709990814,-4.63990578299861));
#47621=CARTESIAN_POINT('Ctrl Pts',(7.50678308517936,2.10606535617851,-5.44201721582885));
#47622=CARTESIAN_POINT('Ctrl Pts',(7.49865343326163,2.02298974534607,-5.88524536138439));
#47623=CARTESIAN_POINT('Ctrl Pts',(7.4961743744293,1.98529253310316,-6.10350764048164));
#47624=CARTESIAN_POINT('Ctrl Pts',(7.49170906930816,1.92570574334559,-6.52452416988688));
#47625=CARTESIAN_POINT('Ctrl Pts',(7.48600371876777,1.84722654992848,-7.29119138736624));
#47626=CARTESIAN_POINT('Ctrl Pts',(7.48223921884591,1.80346041576881,-8.43552251871391));
#47627=CARTESIAN_POINT('Ctrl Pts',(7.48114785215769,1.80751161779657,-9.65853465431959));
#47628=CARTESIAN_POINT('Ctrl Pts',(7.48034069466382,1.8088735491368,-10.5513280174558));
#47629=CARTESIAN_POINT('Ctrl Pts',(7.47971069675407,1.80456152724868,-11.0724961195177));
#47630=CARTESIAN_POINT('Ctrl Pts',(7.47931248800309,1.79995476801641,-11.3367392235495));
#47631=CARTESIAN_POINT('Ctrl Pts',(7.47897576300961,1.79525363342574,-11.5366535550938));
#47632=CARTESIAN_POINT('Ctrl Pts',(7.47872605975369,1.79265101902759,-11.6552228910092));
#47633=CARTESIAN_POINT('Ctrl Pts',(7.47827238577484,1.78791663242365,-11.9013536899149));
#47634=CARTESIAN_POINT('Ctrl Pts',(7.47753715478061,1.78144720805231,-12.3279114350663));
#47635=CARTESIAN_POINT('Ctrl Pts',(7.47631034478809,1.77457410597943,-13.1858634282511));
#47636=CARTESIAN_POINT('Ctrl Pts',(7.47519368111145,1.77849238136237,-14.4167742231908));
#47637=CARTESIAN_POINT('Ctrl Pts',(7.47469258483126,1.78873356384644,-15.5395400353667));
#47638=CARTESIAN_POINT('Ctrl Pts',(7.47447448713808,1.79417730311737,-16.2959696860391));
#47639=CARTESIAN_POINT('Ctrl Pts',(7.47436135191072,1.7971460417357,-16.8026074185616));
#47640=CARTESIAN_POINT('Ctrl Pts',(7.47428469225115,1.79829761012166,-17.1853088109618));
#47641=CARTESIAN_POINT('Ctrl Pts',(7.47423445214067,1.79830077211436,-17.5050291743713));
#47642=CARTESIAN_POINT('Ctrl Pts',(7.47422280456671,1.798303905888,-17.6290014884559));
#47643=CARTESIAN_POINT('Ctrl Pts',(7.4742295721944,1.79831639151149,-17.8785965052693));
#47644=CARTESIAN_POINT('Ctrl Pts',(7.47427497297558,1.79833527958903,-18.1277486173107));
#47645=CARTESIAN_POINT('Ctrl Pts',(7.47435786033162,1.79836039462119,-18.3773597741528));
#47646=CARTESIAN_POINT('Ctrl Pts',(7.47442244316509,1.79837741451397,-18.5333588142296));
#47647=CARTESIAN_POINT('Ctrl Pts',(7.47448174564885,1.7983918361177,-18.6582232456114));
#47648=CARTESIAN_POINT('Ctrl Pts',(7.47452957608076,1.79840285346194,-18.7518839382005));
#47649=CARTESIAN_POINT('Ctrl Pts',(7.47457208182688,1.79841214200524,-18.8299532242847));
#47650=CARTESIAN_POINT('Ctrl Pts',(7.4746076747586,1.79841963674975,-18.8924177727002));
#47651=CARTESIAN_POINT('Ctrl Pts',(7.47491817122276,1.79848316570936,-19.4234214886521));
#47652=CARTESIAN_POINT('Ctrl Pts',(7.47573077242387,1.798595156224,-20.4402710521663));
#47653=CARTESIAN_POINT('Ctrl Pts',(7.4768952047759,1.79842921761441,-21.9476656360667));
#47654=CARTESIAN_POINT('Ctrl Pts',(7.47706144613008,1.79786860312304,-22.9566283715109));
#47655=CARTESIAN_POINT('Ctrl Pts',(7.47683450636963,1.79731318435664,-23.586850451328));
#47656=CARTESIAN_POINT('Ctrl Pts',(7.47671387984677,1.79706369455515,-23.8364592611807));
#47657=CARTESIAN_POINT('Ctrl Pts',(7.47635510879953,1.79645667756257,-24.3362770759908));
#47658=CARTESIAN_POINT('Ctrl Pts',(7.47545952068536,1.79514926597529,-25.2126720882539));
#47659=CARTESIAN_POINT('Ctrl Pts',(7.4736450424381,1.79278506910037,-26.4678871554683));
#47660=CARTESIAN_POINT('Ctrl Pts',(7.47138283293608,1.78984400962715,-27.9763225649068));
#47661=CARTESIAN_POINT('Ctrl Pts',(7.47032691179317,1.78826943081053,-28.9795605867428));
#47662=CARTESIAN_POINT('Ctrl Pts',(7.46999420387175,1.78762815323461,-29.5443956378212));
#47663=CARTESIAN_POINT('Ctrl Pts',(7.46990607068809,1.78672312463406,-29.6880393564753));
#47664=CARTESIAN_POINT('Ctrl Pts',(7.46965834635643,1.78227818555402,-29.9619945701119));
#47665=CARTESIAN_POINT('Ctrl Pts',(7.46905787927587,1.76843599696719,-30.439494351754));
#47666=CARTESIAN_POINT('Ctrl Pts',(7.46726279487216,1.72304890119731,-31.3615763778818));
#47667=CARTESIAN_POINT('Ctrl Pts',(7.46375939358869,1.64326849658029,-32.5989290413864));
#47668=CARTESIAN_POINT('Ctrl Pts',(7.46238748486115,1.62120267413446,-33.7222449914166));
#47669=CARTESIAN_POINT('Ctrl Pts',(7.46601907277839,1.67023374333108,-34.5527699895573));
#47670=CARTESIAN_POINT('Ctrl Pts',(7.47010888017429,1.72081975290891,-34.9467534976082));
#47671=CARTESIAN_POINT('Ctrl Pts',(7.47415782070678,1.76993633235586,-35.2355142231742));
#47672=CARTESIAN_POINT('Ctrl Pts',(7.4777999551406,1.80355688229369,-35.4025766836103));
#47673=CARTESIAN_POINT('Ctrl Pts',(7.48573753704329,1.89930931743001,-35.7795483373344));
#47674=CARTESIAN_POINT('Ctrl Pts',(7.50131995334051,2.13196249717656,-36.4898823831495));
#47675=CARTESIAN_POINT('Ctrl Pts',(7.52885994573029,2.81990008131359,-38.1261297125887));
#47676=CARTESIAN_POINT('Ctrl Pts',(7.54646135782687,3.57997481633,-39.8028011410274));
#47677=CARTESIAN_POINT('Ctrl Pts',(7.55506134819746,3.89828012158619,-41.4522755413143));
#47678=CARTESIAN_POINT('Ctrl Pts',(7.55738012845925,3.96260520846499,-41.8954550225072));
#47679=CARTESIAN_POINT('Ctrl Pts',(7.55974983873441,4.01868373996087,-42.4888348031539));
#47680=CARTESIAN_POINT('Ctrl Pts',(7.56174736166402,4.05502464972836,-43.0653222631363));
#47681=CARTESIAN_POINT('Ctrl Pts',(7.56352824653193,4.07221139566532,-43.7647290043707));
#47682=CARTESIAN_POINT('Ctrl Pts',(7.56478227701937,4.06595245960517,-44.5644779518473));
#47683=CARTESIAN_POINT('Ctrl Pts',(7.56533148651779,4.05283857703286,-45.1992427947033));
#47684=CARTESIAN_POINT('Ctrl Pts',(7.56553354918689,4.04478798258784,-45.6871550449717));
#47685=CARTESIAN_POINT('Ctrl Pts',(7.5656428385536,4.04165025393199,-46.043284316581));
#47686=CARTESIAN_POINT('Ctrl Pts',(7.56574019074214,4.04290621007078,-46.3893532108146));
#47687=CARTESIAN_POINT('Ctrl Pts',(7.56588033119948,4.05223544847548,-46.8374697517941));
#47688=CARTESIAN_POINT('Ctrl Pts',(7.56612231469326,4.06973784094667,-47.1581709597959));
#47689=CARTESIAN_POINT('Ctrl Pts',(7.56644470873198,4.09645379880801,-47.4711009352875));
#47690=CARTESIAN_POINT('Ctrl Pts',(7.56664923644244,4.11889435515154,-47.7332118947828));
#47691=CARTESIAN_POINT('Ctrl Pts',(7.56702704076722,4.16178288413229,-48.22449728));
#47692=CARTESIAN_POINT('Ctrl Pts',(7.56757644835753,4.24095012196946,-49.0918571760979));
#47693=CARTESIAN_POINT('Ctrl Pts',(7.56790794403495,4.36869434493729,-50.2995294266277));
#47694=CARTESIAN_POINT('Ctrl Pts',(7.56674498299714,4.56943457631291,-51.7173816663438));
#47695=CARTESIAN_POINT('Ctrl Pts',(7.56463708563956,4.74847674481168,-52.6373167573546));
#47696=CARTESIAN_POINT('Ctrl Pts',(7.56272848288763,4.87914678571234,-53.2072484319363));
#47697=CARTESIAN_POINT('Ctrl Pts',(7.56186059988464,4.93499175495422,-53.443617226946));
#47698=CARTESIAN_POINT('Ctrl Pts',(7.55976715503288,5.05266256760958,-53.9144056700956));
#47699=CARTESIAN_POINT('Ctrl Pts',(7.55531846507066,5.2762603192113,-54.7433752709434));
#47700=CARTESIAN_POINT('Ctrl Pts',(7.54421884355346,5.78831119318727,-56.4093170580287));
#47701=CARTESIAN_POINT('Ctrl Pts',(7.53434277323058,6.32574074251072,-57.8435279363008));
#47702=CARTESIAN_POINT('Ctrl Pts',(7.53028057508383,6.73962490994349,-58.8516240716937));
#47703=CARTESIAN_POINT('Ctrl Pts',(7.5297836098851,6.7874239169442,-58.9665470204583));
#47704=CARTESIAN_POINT('Ctrl Pts',(7.52883630432498,6.88762233423541,-59.2019071068476));
#47705=CARTESIAN_POINT('Ctrl Pts',(7.5272717350224,7.06910816068731,-59.6143115109346));
#47706=CARTESIAN_POINT('Ctrl Pts',(7.52452689433495,7.45870700081999,-60.4508213037396));
#47707=CARTESIAN_POINT('Ctrl Pts',(7.52214269466404,7.95191257071366,-61.4239593595716));
#47708=CARTESIAN_POINT('Ctrl Pts',(7.52032781922298,8.47101662510095,-62.4090068565059));
#47709=CARTESIAN_POINT('Ctrl Pts',(7.51947604021343,8.76822269947309,-62.9664674348229));
#47710=CARTESIAN_POINT('Ctrl Pts',(7.51895952889291,8.96674264835317,-63.339307001888));
#47711=CARTESIAN_POINT('Ctrl Pts',(7.51862913853834,9.09906857249673,-63.588176763506));
#47712=CARTESIAN_POINT('Ctrl Pts',(7.51831176641175,9.23115450301005,-63.837450489128));
#47713=CARTESIAN_POINT('Ctrl Pts',(7.51804847893112,9.34622920040807,-64.0559509774442));
#47714=CARTESIAN_POINT('Ctrl Pts',(7.51790092374494,9.41179504082436,-64.1809144183687));
#47715=CARTESIAN_POINT('Ctrl Pts',(7.51768262198302,9.50992314869041,-64.3684522626355));
#47716=CARTESIAN_POINT('Ctrl Pts',(7.51750366928883,9.59121012018809,-64.5249707181327));
#47717=CARTESIAN_POINT('Ctrl Pts',(7.51721456528255,9.72473987575942,-64.7841239316579));
#47718=CARTESIAN_POINT('Ctrl Pts',(7.51695154925424,9.85487124438173,-65.0356980537645));
#47719=CARTESIAN_POINT('Ctrl Pts',(7.51655986773369,10.1197152427305,-65.5441577753383));
#47720=CARTESIAN_POINT('Ctrl Pts',(7.51617932888529,10.5812597640262,-66.4217711154117));
#47721=CARTESIAN_POINT('Ctrl Pts',(7.51637926889889,11.5083859878242,-68.1586823730641));
#47722=CARTESIAN_POINT('Ctrl Pts',(7.51718838686394,12.3075015417636,-69.6375526163581));
#47723=CARTESIAN_POINT('Ctrl Pts',(7.51716645787803,12.9112162672006,-70.7730095811495));
#47724=CARTESIAN_POINT('Ctrl Pts',(7.51716390165521,13.0444256040857,-71.0235462226635));
#47725=CARTESIAN_POINT('Ctrl Pts',(7.51715952057163,13.3115101026409,-71.5258686016946));
#47726=CARTESIAN_POINT('Ctrl Pts',(7.51715469827561,13.6448646470806,-72.1528242965523));
#47727=CARTESIAN_POINT('Ctrl Pts',(7.5171533384676,14.0448792873963,-72.9051434628418));
#47728=CARTESIAN_POINT('Ctrl Pts',(7.51715455299824,14.8445227247772,-74.4090466856942));
#47729=CARTESIAN_POINT('Ctrl Pts',(7.51715350869284,15.5104861014003,-75.6615266096123));
#47730=CARTESIAN_POINT('Ctrl Pts',(7.51714857446979,16.4802261084657,-77.4853440369576));
#47731=CARTESIAN_POINT('Ctrl Pts',(7.51714603172462,16.9167002668011,-78.306233429594));
#47732=CARTESIAN_POINT('Ctrl Pts',(7.5171460317246,17.3532218541906,-79.1272111316924));
#47733=CARTESIAN_POINT('Ctrl Pts',(10.9624646798336,4.08045736333527,24.8306353233982));
#47734=CARTESIAN_POINT('Ctrl Pts',(10.9624974112732,4.08045738492077,24.7817560292463));
#47735=CARTESIAN_POINT('Ctrl Pts',(10.9625317350798,4.0804573829706,24.7328775366951));
#47736=CARTESIAN_POINT('Ctrl Pts',(10.9629372601565,4.08045847670549,24.1822781736734));
#47737=CARTESIAN_POINT('Ctrl Pts',(10.9632485186784,4.08046588120829,23.1782140967866));
#47738=CARTESIAN_POINT('Ctrl Pts',(10.9639697700664,4.08046799907804,21.1696235179717));
#47739=CARTESIAN_POINT('Ctrl Pts',(10.9666707335973,4.08048691112784,19.6656474654337));
#47740=CARTESIAN_POINT('Ctrl Pts',(10.9723972261602,4.0804966227945,18.4146756888765));
#47741=CARTESIAN_POINT('Ctrl Pts',(10.9751429165286,4.08049896285481,17.9118722585523));
#47742=CARTESIAN_POINT('Ctrl Pts',(10.9820375662411,4.08050702316906,16.9079334045807));
#47743=CARTESIAN_POINT('Ctrl Pts',(10.9968251949538,4.08051890113854,15.1541749240292));
#47744=CARTESIAN_POINT('Ctrl Pts',(11.0108841762241,4.08056270929919,13.6528297088379));
#47745=CARTESIAN_POINT('Ctrl Pts',(11.0197032179328,4.08058047523023,12.3985380152264));
#47746=CARTESIAN_POINT('Ctrl Pts',(11.0233090516766,4.0805860831325,11.8976334291727));
#47747=CARTESIAN_POINT('Ctrl Pts',(11.0306607980321,4.08058621139806,10.8958434397728));
#47748=CARTESIAN_POINT('Ctrl Pts',(11.0397602248644,4.08061971854824,9.64361147068879));
#47749=CARTESIAN_POINT('Ctrl Pts',(11.049357601229,4.08062788610815,8.13953906117807));
#47750=CARTESIAN_POINT('Ctrl Pts',(11.0541129858031,4.08068358210231,7.13497790928695));
#47751=CARTESIAN_POINT('Ctrl Pts',(11.0563205349784,4.08069356878045,6.50810793756284));
#47752=CARTESIAN_POINT('Ctrl Pts',(11.0578003392729,4.08238703533895,6.2812286397764));
#47753=CARTESIAN_POINT('Ctrl Pts',(11.0626898963694,4.09135641957855,5.80540232705015));
#47754=CARTESIAN_POINT('Ctrl Pts',(11.0749984328579,4.11902224542694,4.95882848560147));
#47755=CARTESIAN_POINT('Ctrl Pts',(11.1046504104053,4.19473247930313,3.17968685652564));
#47756=CARTESIAN_POINT('Ctrl Pts',(11.1036402821399,4.20015554547666,1.5276097462183));
#47757=CARTESIAN_POINT('Ctrl Pts',(11.0579407115821,4.05981651715574,0.299696259065808));
#47758=CARTESIAN_POINT('Ctrl Pts',(11.0520116181057,4.04046613063924,0.143859829319175));
#47759=CARTESIAN_POINT('Ctrl Pts',(11.0383688353589,3.99686870684385,-0.15805611788381));
#47760=CARTESIAN_POINT('Ctrl Pts',(11.0101613797018,3.90700136384924,-0.679347896305351));
#47761=CARTESIAN_POINT('Ctrl Pts',(10.9595892987304,3.74798647031421,-1.39388395716988));
#47762=CARTESIAN_POINT('Ctrl Pts',(10.8880526310442,3.52822646669199,-2.20853931547687));
#47763=CARTESIAN_POINT('Ctrl Pts',(10.7848130904019,3.22105878258507,-3.2390988854101));
#47764=CARTESIAN_POINT('Ctrl Pts',(10.6513887040697,2.85284672812267,-4.42823588303147));
#47765=CARTESIAN_POINT('Ctrl Pts',(10.5655199263466,2.65190863334669,-5.27510542835426));
#47766=CARTESIAN_POINT('Ctrl Pts',(10.5301425486311,2.57492197176225,-5.77252875520469));
#47767=CARTESIAN_POINT('Ctrl Pts',(10.5180961403591,2.54369111238152,-6.00047614868717));
#47768=CARTESIAN_POINT('Ctrl Pts',(10.4975524844,2.49281502581667,-6.44643200010511));
#47769=CARTESIAN_POINT('Ctrl Pts',(10.4716388096329,2.42689514909976,-7.24930178718183));
#47770=CARTESIAN_POINT('Ctrl Pts',(10.4561427601609,2.39011928274206,-8.4311631487814));
#47771=CARTESIAN_POINT('Ctrl Pts',(10.454094044526,2.39207050169796,-9.66480471721667));
#47772=CARTESIAN_POINT('Ctrl Pts',(10.4522985336733,2.39207600035412,-10.5518894638563));
#47773=CARTESIAN_POINT('Ctrl Pts',(10.4502394625745,2.38828612858452,-11.0657987432211));
#47774=CARTESIAN_POINT('Ctrl Pts',(10.4487075309053,2.38456441505993,-11.3250687490037));
#47775=CARTESIAN_POINT('Ctrl Pts',(10.4473070301966,2.38085337186641,-11.5208859320258));
#47776=CARTESIAN_POINT('Ctrl Pts',(10.4463583875329,2.37864387283397,-11.6420016120887));
#47777=CARTESIAN_POINT('Ctrl Pts',(10.4446744419706,2.37468153201103,-11.8901027852085));
#47778=CARTESIAN_POINT('Ctrl Pts',(10.4421721669975,2.36913398587217,-12.3212797555185));
#47779=CARTESIAN_POINT('Ctrl Pts',(10.4388561688442,2.36285626689449,-13.1860420530998));
#47780=CARTESIAN_POINT('Ctrl Pts',(10.4378552861942,2.36469137873023,-14.423262317235));
#47781=CARTESIAN_POINT('Ctrl Pts',(10.4391338276668,2.37177576636951,-15.5464880771636));
#47782=CARTESIAN_POINT('Ctrl Pts',(10.4399406768736,2.37559028962932,-16.3012341882906));
#47783=CARTESIAN_POINT('Ctrl Pts',(10.4403999741264,2.37767480820586,-16.8061852749493));
#47784=CARTESIAN_POINT('Ctrl Pts',(10.44060257823,2.37848080144773,-17.1870308097338));
#47785=CARTESIAN_POINT('Ctrl Pts',(10.440603319085,2.37846229885705,-17.5049134003353));
#47786=CARTESIAN_POINT('Ctrl Pts',(10.4406208058462,2.37845624979895,-17.6292519804825));
#47787=CARTESIAN_POINT('Ctrl Pts',(10.4407204731566,2.3784494134481,-17.8789060526275));
#47788=CARTESIAN_POINT('Ctrl Pts',(10.4409123918676,2.37845080985169,-18.1283166835446));
#47789=CARTESIAN_POINT('Ctrl Pts',(10.4411782512159,2.37846197013343,-18.3780117776051));
#47790=CARTESIAN_POINT('Ctrl Pts',(10.4413733035248,2.37847312744644,-18.5340741512269));
#47791=CARTESIAN_POINT('Ctrl Pts',(10.441544359038,2.37848476145854,-18.6589666563742));
#47792=CARTESIAN_POINT('Ctrl Pts',(10.4416798768071,2.37849485565446,-18.7526456803256));
#47793=CARTESIAN_POINT('Ctrl Pts',(10.4417984461137,2.3785044379206,-18.8307245329558));
#47794=CARTESIAN_POINT('Ctrl Pts',(10.4418963892107,2.37851283166161,-18.8931941630973));
#47795=CARTESIAN_POINT('Ctrl Pts',(10.4427467029551,2.37858826050148,-19.4242255273232));
#47796=CARTESIAN_POINT('Ctrl Pts',(10.4448940853641,2.37886351740411,-20.440668336297));
#47797=CARTESIAN_POINT('Ctrl Pts',(10.4477033212108,2.37979135147078,-21.9460157760457));
#47798=CARTESIAN_POINT('Ctrl Pts',(10.4480698678651,2.38084786701659,-22.9527105822916));
#47799=CARTESIAN_POINT('Ctrl Pts',(10.4474558488072,2.38167163198556,-23.5812081457634));
#47800=CARTESIAN_POINT('Ctrl Pts',(10.4471330270657,2.38203091629453,-23.8298055877299));
#47801=CARTESIAN_POINT('Ctrl Pts',(10.4461958941223,2.38286906347281,-24.3280584766635));
#47802=CARTESIAN_POINT('Ctrl Pts',(10.4438980219011,2.3846101529119,-25.2021910563275));
#47803=CARTESIAN_POINT('Ctrl Pts',(10.4392357405293,2.38763519968205,-26.4560467041742));
#47804=CARTESIAN_POINT('Ctrl Pts',(10.433280894909,2.39137954388358,-27.9653174676155));
#47805=CARTESIAN_POINT('Ctrl Pts',(10.4301731559634,2.39340640289701,-28.9712942079044));
#47806=CARTESIAN_POINT('Ctrl Pts',(10.4290290267676,2.39427462377435,-29.5375862367704));
#47807=CARTESIAN_POINT('Ctrl Pts',(10.4286212480674,2.3939419742561,-29.6752033047866));
#47808=CARTESIAN_POINT('Ctrl Pts',(10.4272628698591,2.39126233326746,-29.941736351058));
#47809=CARTESIAN_POINT('Ctrl Pts',(10.4235781498688,2.38193132510707,-30.4068259305923));
#47810=CARTESIAN_POINT('Ctrl Pts',(10.4121237168613,2.3492732871545,-31.3152106151894));
#47811=CARTESIAN_POINT('Ctrl Pts',(10.3907411254912,2.28811111526887,-32.559221395248));
#47812=CARTESIAN_POINT('Ctrl Pts',(10.3825197668055,2.26979831419424,-33.7280316465651));
#47813=CARTESIAN_POINT('Ctrl Pts',(10.39795839888,2.31307366271173,-34.6166593913203));
#47814=CARTESIAN_POINT('Ctrl Pts',(10.4156112942381,2.35851940812219,-35.0450053773708));
#47815=CARTESIAN_POINT('Ctrl Pts',(10.4336262420655,2.40301971240747,-35.3604888544365));
#47816=CARTESIAN_POINT('Ctrl Pts',(10.4487446471554,2.43604685187258,-35.5528315719723));
#47817=CARTESIAN_POINT('Ctrl Pts',(10.4855848805768,2.52287245628984,-35.9635953787419));
#47818=CARTESIAN_POINT('Ctrl Pts',(10.5654929538693,2.72085013989271,-36.7112829926298));
#47819=CARTESIAN_POINT('Ctrl Pts',(10.7565856506919,3.25488597070165,-38.3527194747804));
#47820=CARTESIAN_POINT('Ctrl Pts',(10.9170481196781,3.78092103798195,-40.0042489860928));
#47821=CARTESIAN_POINT('Ctrl Pts',(10.9795150310049,3.98577979631989,-41.5483666219995));
#47822=CARTESIAN_POINT('Ctrl Pts',(10.9948567121963,4.028017025414,-41.9778845998627));
#47823=CARTESIAN_POINT('Ctrl Pts',(11.0094600365173,4.06189769773347,-42.547662950352));
#47824=CARTESIAN_POINT('Ctrl Pts',(11.020579781767,4.08228371762755,-43.1048191371307));
#47825=CARTESIAN_POINT('Ctrl Pts',(11.0286564301021,4.08804953783849,-43.783876357993));
#47826=CARTESIAN_POINT('Ctrl Pts',(11.0315794804677,4.07721734166889,-44.5678175389575));
#47827=CARTESIAN_POINT('Ctrl Pts',(11.0305256425759,4.064054799379,-45.1959666455832));
#47828=CARTESIAN_POINT('Ctrl Pts',(11.0288587160196,4.05661717032617,-45.6826348738755));
#47829=CARTESIAN_POINT('Ctrl Pts',(11.0275262074785,4.05387433928492,-46.0398346180674));
#47830=CARTESIAN_POINT('Ctrl Pts',(11.0264331705636,4.0551708360785,-46.3890211810534));
#47831=CARTESIAN_POINT('Ctrl Pts',(11.0257195434411,4.06376907747683,-46.8439571389145));
#47832=CARTESIAN_POINT('Ctrl Pts',(11.0265249261146,4.07951702892443,-47.1728757993545));
#47833=CARTESIAN_POINT('Ctrl Pts',(11.0288417663362,4.10343060615818,-47.4956385365803));
#47834=CARTESIAN_POINT('Ctrl Pts',(11.0303413896298,4.12272689329889,-47.7560094569819));
#47835=CARTESIAN_POINT('Ctrl Pts',(11.033139264776,4.16003680841996,-48.248255683235));
#47836=CARTESIAN_POINT('Ctrl Pts',(11.0374645879716,4.22917939920677,-49.1143392464993));
#47837=CARTESIAN_POINT('Ctrl Pts',(11.04184899311,4.34372908818247,-50.3199340632308));
#47838=CARTESIAN_POINT('Ctrl Pts',(11.0435083236951,4.53158843368009,-51.7317826449608));
#47839=CARTESIAN_POINT('Ctrl Pts',(11.0417924431526,4.70482052662216,-52.646310903103));
#47840=CARTESIAN_POINT('Ctrl Pts',(11.039663329745,4.83290160929832,-53.2124171963205));
#47841=CARTESIAN_POINT('Ctrl Pts',(11.0386162679699,4.88778364060814,-53.4470591412272));
#47842=CARTESIAN_POINT('Ctrl Pts',(11.0358085502369,5.00418278352712,-53.9149045068776));
#47843=CARTESIAN_POINT('Ctrl Pts',(11.0292893597981,5.22701505697702,-54.7395333124799));
#47844=CARTESIAN_POINT('Ctrl Pts',(11.0116266608252,5.7426033353743,-56.400240346654));
#47845=CARTESIAN_POINT('Ctrl Pts',(10.9949335907642,6.28836758405837,-57.8349512527431));
#47846=CARTESIAN_POINT('Ctrl Pts',(10.988087935204,6.70711748343476,-58.8453134842339));
#47847=CARTESIAN_POINT('Ctrl Pts',(10.9872366677291,6.75521207647722,-58.959839211309));
#47848=CARTESIAN_POINT('Ctrl Pts',(10.9855946313238,6.85626298130136,-59.1948421885943));
#47849=CARTESIAN_POINT('Ctrl Pts',(10.9828275348998,7.03935578536294,-59.6065522268112));
#47850=CARTESIAN_POINT('Ctrl Pts',(10.9777571326992,7.43297483611379,-60.4422881173784));
#47851=CARTESIAN_POINT('Ctrl Pts',(10.9729723326619,7.93198121156931,-61.4153348277046));
#47852=CARTESIAN_POINT('Ctrl Pts',(10.9690819296197,8.45721017371796,-62.4010643447095));
#47853=CARTESIAN_POINT('Ctrl Pts',(10.96719703468,8.75778667494156,-62.9591856758838));
#47854=CARTESIAN_POINT('Ctrl Pts',(10.9660565033908,8.95844769089226,-63.332594904036));
#47855=CARTESIAN_POINT('Ctrl Pts',(10.9653263751097,9.09216753085925,-63.5818802113062));
#47856=CARTESIAN_POINT('Ctrl Pts',(10.9646401134821,9.22558789845036,-63.8316230488872));
#47857=CARTESIAN_POINT('Ctrl Pts',(10.9640769863299,9.34176608562326,-64.0505869757395));
#47858=CARTESIAN_POINT('Ctrl Pts',(10.9637656030705,9.40794198473294,-64.1758308493704));
#47859=CARTESIAN_POINT('Ctrl Pts',(10.9633088727675,9.50696363874219,-64.3638052868478));
#47860=CARTESIAN_POINT('Ctrl Pts',(10.9629492508971,9.58894814837339,-64.520721446415));
#47861=CARTESIAN_POINT('Ctrl Pts',(10.9623815065997,9.72355770937703,-64.7805808924906));
#47862=CARTESIAN_POINT('Ctrl Pts',(10.961867348382,9.85459317907115,-65.0327186415835));
#47863=CARTESIAN_POINT('Ctrl Pts',(10.961100025666,10.1209500852642,-65.5422775660664));
#47864=CARTESIAN_POINT('Ctrl Pts',(10.9603700836074,10.5842356687815,-66.4214830775254));
#47865=CARTESIAN_POINT('Ctrl Pts',(10.960791456899,11.5120040023041,-68.1604138179985));
#47866=CARTESIAN_POINT('Ctrl Pts',(10.962444386315,12.3088852940989,-69.63881635891));
#47867=CARTESIAN_POINT('Ctrl Pts',(10.9624193577822,12.9119028977147,-70.7728829833708));
#47868=CARTESIAN_POINT('Ctrl Pts',(10.9624149235793,13.0451745975293,-71.0235209119673));
#47869=CARTESIAN_POINT('Ctrl Pts',(10.9624081676807,13.3122533538826,-71.525808947084));
#47870=CARTESIAN_POINT('Ctrl Pts',(10.9624034364209,13.6456418223831,-72.1528135877663));
#47871=CARTESIAN_POINT('Ctrl Pts',(10.962402792736,14.0456590372664,-72.9051362844501));
#47872=CARTESIAN_POINT('Ctrl Pts',(10.9624082559957,14.8453066308756,-74.4090687157949));
#47873=CARTESIAN_POINT('Ctrl Pts',(10.9624198923528,15.5112398060805,-75.6615407410724));
#47874=CARTESIAN_POINT('Ctrl Pts',(10.9624192066963,16.4809656828406,-77.4853334277387));
#47875=CARTESIAN_POINT('Ctrl Pts',(10.962418854705,16.9174449520636,-78.306233377601));
#47876=CARTESIAN_POINT('Ctrl Pts',(10.9624188547049,17.3539665394531,-79.1272110796992));
#47877=CARTESIAN_POINT('Ctrl Pts',(14.0957722616046,4.08025224202491,24.8306350534813));
#47878=CARTESIAN_POINT('Ctrl Pts',(14.0958143929042,4.08025223777848,24.7817557508935));
#47879=CARTESIAN_POINT('Ctrl Pts',(14.0958586147606,4.08025224020083,24.7328773999137));
#47880=CARTESIAN_POINT('Ctrl Pts',(14.0963792203118,4.08025195558791,24.1822728844133));
#47881=CARTESIAN_POINT('Ctrl Pts',(14.0967691662794,4.08025016189665,23.1781665546079));
#47882=CARTESIAN_POINT('Ctrl Pts',(14.0976986663016,4.08025040075573,21.1695712092763));
#47883=CARTESIAN_POINT('Ctrl Pts',(14.1011467099489,4.08024523061615,19.6654902060134));
#47884=CARTESIAN_POINT('Ctrl Pts',(14.1085012613688,4.08024146562352,18.4144726949287));
#47885=CARTESIAN_POINT('Ctrl Pts',(14.112031928167,4.08024039800909,17.9116616565299));
#47886=CARTESIAN_POINT('Ctrl Pts',(14.1208949819925,4.08023722409591,16.9076927383382));
#47887=CARTESIAN_POINT('Ctrl Pts',(14.1399130451043,4.0802318870913,15.1539031954854));
#47888=CARTESIAN_POINT('Ctrl Pts',(14.1579323195343,4.08021608260615,13.6523208445742));
#47889=CARTESIAN_POINT('Ctrl Pts',(14.1692375188454,4.08020641551546,12.3979191365052));
#47890=CARTESIAN_POINT('Ctrl Pts',(14.1738610753222,4.08020264368447,11.8969840543586));
#47891=CARTESIAN_POINT('Ctrl Pts',(14.1833011346846,4.08019722714216,10.8951616868544));
#47892=CARTESIAN_POINT('Ctrl Pts',(14.1949232190994,4.08017961625232,9.64275109698061));
#47893=CARTESIAN_POINT('Ctrl Pts',(14.2072172257641,4.08016715485986,8.13843619450838));
#47894=CARTESIAN_POINT('Ctrl Pts',(14.2132228690599,4.08014617977765,7.13377888058149));
#47895=CARTESIAN_POINT('Ctrl Pts',(14.2160315118066,4.08013942757265,6.50628030649056));
#47896=CARTESIAN_POINT('Ctrl Pts',(14.2176986615796,4.08091122936134,6.26622708525673));
#47897=CARTESIAN_POINT('Ctrl Pts',(14.2227661810843,4.08496578782836,5.77613445723852));
#47898=CARTESIAN_POINT('Ctrl Pts',(14.234951250782,4.09724160665188,4.91165706708067));
#47899=CARTESIAN_POINT('Ctrl Pts',(14.2633316246722,4.1299454694222,3.14305425317667));
#47900=CARTESIAN_POINT('Ctrl Pts',(14.26163274653,4.13064083791219,1.57311169508529));
#47901=CARTESIAN_POINT('Ctrl Pts',(14.217808675051,4.07483069290229,0.4393870841717));
#47902=CARTESIAN_POINT('Ctrl Pts',(14.2121377388243,4.06744144356774,0.300155285117995));
#47903=CARTESIAN_POINT('Ctrl Pts',(14.1990028839386,4.05046808579315,0.0259639762829477));
#47904=CARTESIAN_POINT('Ctrl Pts',(14.1716535834632,4.01513330090296,-0.45073499273355));
#47905=CARTESIAN_POINT('Ctrl Pts',(14.1216470640614,3.95077230622961,-1.11832601035692));
#47906=CARTESIAN_POINT('Ctrl Pts',(14.0501571326149,3.85790200844971,-1.89955855307956));
#47907=CARTESIAN_POINT('Ctrl Pts',(13.9466278931188,3.72218464731662,-2.91468587912626));
#47908=CARTESIAN_POINT('Ctrl Pts',(13.8170860215073,3.54757776024588,-4.1356917687126));
#47909=CARTESIAN_POINT('Ctrl Pts',(13.7417991770219,3.44328100973835,-5.06703193017387));
#47910=CARTESIAN_POINT('Ctrl Pts',(13.711768974192,3.4023133314411,-5.63700537744905));
#47911=CARTESIAN_POINT('Ctrl Pts',(13.7006597439476,3.38683006257498,-5.87789745435641));
#47912=CARTESIAN_POINT('Ctrl Pts',(13.6818070884903,3.36109180040963,-6.35550542504808));
#47913=CARTESIAN_POINT('Ctrl Pts',(13.6566827315685,3.32792252231433,-7.20154490850171));
#47914=CARTESIAN_POINT('Ctrl Pts',(13.6385492426767,3.30849333959344,-8.4256484574165));
#47915=CARTESIAN_POINT('Ctrl Pts',(13.6323192556659,3.30761361742229,-9.67105362490119));
#47916=CARTESIAN_POINT('Ctrl Pts',(13.6281947514418,3.30648369164368,-10.5515920750503));
#47917=CARTESIAN_POINT('Ctrl Pts',(13.6249884359623,3.30417686766909,-11.0572537158354));
#47918=CARTESIAN_POINT('Ctrl Pts',(13.6229551503502,3.30221720858706,-11.3108889561999));
#47919=CARTESIAN_POINT('Ctrl Pts',(13.621209461118,3.30034221345478,-11.5020704562404));
#47920=CARTESIAN_POINT('Ctrl Pts',(13.62008300239,3.29917053339368,-11.6259943206145));
#47921=CARTESIAN_POINT('Ctrl Pts',(13.6179969710272,3.29707286346251,-11.8762260717926));
#47922=CARTESIAN_POINT('Ctrl Pts',(13.6147649750364,3.29405214925987,-12.3124479418529));
#47923=CARTESIAN_POINT('Ctrl Pts',(13.609813655358,3.29032832992611,-13.1846089255078));
#47924=CARTESIAN_POINT('Ctrl Pts',(13.6064272849751,3.29024237402413,-14.4288653820665));
#47925=CARTESIAN_POINT('Ctrl Pts',(13.6059488544036,3.29295603188387,-15.552953552654));
#47926=CARTESIAN_POINT('Ctrl Pts',(13.605935987415,3.29446857233125,-16.3061936218231));
#47927=CARTESIAN_POINT('Ctrl Pts',(13.6059686566929,3.29530204022143,-16.809555982347));
#47928=CARTESIAN_POINT('Ctrl Pts',(13.6059428832185,3.29561151559316,-17.1885703521757));
#47929=CARTESIAN_POINT('Ctrl Pts',(13.6058577881079,3.29557809642926,-17.5046193636793));
#47930=CARTESIAN_POINT('Ctrl Pts',(13.6058394331441,3.29556697172451,-17.6291257712303));
#47931=CARTESIAN_POINT('Ctrl Pts',(13.6058606477582,3.29555273863726,-17.8786039504253));
#47932=CARTESIAN_POINT('Ctrl Pts',(13.6059585834602,3.29554968779625,-18.1280470931691));
#47933=CARTESIAN_POINT('Ctrl Pts',(13.6061371979844,3.29556150239626,-18.3776851657281));
#47934=CARTESIAN_POINT('Ctrl Pts',(13.606277848496,3.29557461284349,-18.5337408186998));
#47935=CARTESIAN_POINT('Ctrl Pts',(13.6064085950517,3.29558906102363,-18.6586223633998));
#47936=CARTESIAN_POINT('Ctrl Pts',(13.6065149691708,3.2956017869801,-18.7522970792157));
#47937=CARTESIAN_POINT('Ctrl Pts',(13.6066103946943,3.29561400434787,-18.8303728404865));
#47938=CARTESIAN_POINT('Ctrl Pts',(13.6066909378835,3.29562481863403,-18.8928410419629));
#47939=CARTESIAN_POINT('Ctrl Pts',(13.6073975306193,3.29572224056636,-19.4238647637186));
#47940=CARTESIAN_POINT('Ctrl Pts',(13.6093482782903,3.29607453019957,-20.4404632592027));
#47941=CARTESIAN_POINT('Ctrl Pts',(13.613515444394,3.29730127902555,-21.9464317716729));
#47942=CARTESIAN_POINT('Ctrl Pts',(13.6164149373181,3.29868046736958,-22.9538279358975));
#47943=CARTESIAN_POINT('Ctrl Pts',(13.6181684020297,3.2997613576573,-23.5828481007943));
#47944=CARTESIAN_POINT('Ctrl Pts',(13.6189062948723,3.30023460562879,-23.8317453714256));
#47945=CARTESIAN_POINT('Ctrl Pts',(13.6205041705563,3.30133462782811,-24.3304715166219));
#47946=CARTESIAN_POINT('Ctrl Pts',(13.6235890300596,3.30361070112582,-25.2052634597723));
#47947=CARTESIAN_POINT('Ctrl Pts',(13.6284676637919,3.30752238854275,-26.4596112213963));
#47948=CARTESIAN_POINT('Ctrl Pts',(13.634391932039,3.31228885898376,-27.9684620455715));
#47949=CARTESIAN_POINT('Ctrl Pts',(13.6377145543258,3.31484211483178,-28.9739530226395));
#47950=CARTESIAN_POINT('Ctrl Pts',(13.6392827711463,3.31593712679648,-29.5391966731624));
#47951=CARTESIAN_POINT('Ctrl Pts',(13.6394729395101,3.31592737394666,-29.6699683072265));
#47952=CARTESIAN_POINT('Ctrl Pts',(13.6392609164336,3.31499860145106,-29.9277267142216));
#47953=CARTESIAN_POINT('Ctrl Pts',(13.6375060047046,3.31123579619119,-30.3782995864193));
#47954=CARTESIAN_POINT('Ctrl Pts',(13.6296869144124,3.29716631537485,-31.2701338041608));
#47955=CARTESIAN_POINT('Ctrl Pts',(13.6136132998802,3.26961315261814,-32.5208407448675));
#47956=CARTESIAN_POINT('Ctrl Pts',(13.6098028170218,3.26146264647698,-33.7375415486611));
#47957=CARTESIAN_POINT('Ctrl Pts',(13.6251691852064,3.28331170129501,-34.6892215501438));
#47958=CARTESIAN_POINT('Ctrl Pts',(13.6409911101313,3.3062856843424,-35.1574771360631));
#47959=CARTESIAN_POINT('Ctrl Pts',(13.6566505661323,3.32898166052496,-35.506308737971));
#47960=CARTESIAN_POINT('Ctrl Pts',(13.668999090906,3.34657459397007,-35.7315463147679));
#47961=CARTESIAN_POINT('Ctrl Pts',(13.7005318287958,3.39149074550588,-36.192735153184));
#47962=CARTESIAN_POINT('Ctrl Pts',(13.7716810680424,3.49154222603004,-37.0111939547442));
#47963=CARTESIAN_POINT('Ctrl Pts',(13.9588609326516,3.74776357601237,-38.7093739498868));
#47964=CARTESIAN_POINT('Ctrl Pts',(14.1256135782939,3.96387662432988,-40.2853147475507));
#47965=CARTESIAN_POINT('Ctrl Pts',(14.1827832858029,4.0436959918171,-41.6701713771011));
#47966=CARTESIAN_POINT('Ctrl Pts',(14.1961412729749,4.05981198579182,-42.080172583266));
#47967=CARTESIAN_POINT('Ctrl Pts',(14.2079179531119,4.06939224831422,-42.616605568901));
#47968=CARTESIAN_POINT('Ctrl Pts',(14.2161502176523,4.0727928413343,-43.1469071634193));
#47969=CARTESIAN_POINT('Ctrl Pts',(14.2205227502483,4.068049750572,-43.7976710866968));
#47970=CARTESIAN_POINT('Ctrl Pts',(14.2187737413236,4.05621093007814,-44.5590470961975));
#47971=CARTESIAN_POINT('Ctrl Pts',(14.2135158820145,4.0475021396245,-45.1768425637423));
#47972=CARTESIAN_POINT('Ctrl Pts',(14.2080910805333,4.04466830914136,-45.6605239026345));
#47973=CARTESIAN_POINT('Ctrl Pts',(14.2037801847839,4.04544563623318,-46.0180830518693));
#47974=CARTESIAN_POINT('Ctrl Pts',(14.1995182434366,4.04991129743658,-46.3702990795996));
#47975=CARTESIAN_POINT('Ctrl Pts',(14.1942624653917,4.06177576419791,-46.8327555084787));
#47976=CARTESIAN_POINT('Ctrl Pts',(14.1913862340194,4.07843457326759,-47.1713943500007));
#47977=CARTESIAN_POINT('Ctrl Pts',(14.1896746126773,4.10168956138419,-47.5060662243987));
#47978=CARTESIAN_POINT('Ctrl Pts',(14.1882421443729,4.11971388651359,-47.7607279322735));
#47979=CARTESIAN_POINT('Ctrl Pts',(14.1843422192657,4.15604054285058,-48.2499237009795));
#47980=CARTESIAN_POINT('Ctrl Pts',(14.1751633013163,4.22530318057308,-49.1081940334974));
#47981=CARTESIAN_POINT('Ctrl Pts',(14.1573527711649,4.34454619162834,-50.3093484640539));
#47982=CARTESIAN_POINT('Ctrl Pts',(14.1342139911527,4.53993015134586,-51.7215503416932));
#47983=CARTESIAN_POINT('Ctrl Pts',(14.1220648297914,4.71705492839944,-52.6412484343876));
#47984=CARTESIAN_POINT('Ctrl Pts',(14.1166308064331,4.84652873809678,-53.2116158079059));
#47985=CARTESIAN_POINT('Ctrl Pts',(14.1144335582758,4.90158703428815,-53.4464345864701));
#47986=CARTESIAN_POINT('Ctrl Pts',(14.1102019568884,5.01835112087333,-53.9153774892103));
#47987=CARTESIAN_POINT('Ctrl Pts',(14.1032136620098,5.24128557042568,-54.7411838437102));
#47988=CARTESIAN_POINT('Ctrl Pts',(14.0910217927261,5.75569340563091,-56.4035773722642));
#47989=CARTESIAN_POINT('Ctrl Pts',(14.0842516957791,6.29879311260299,-57.8378372308137));
#47990=CARTESIAN_POINT('Ctrl Pts',(14.0821871841893,6.71606534019326,-58.847357500806));
#47991=CARTESIAN_POINT('Ctrl Pts',(14.0820201446177,6.76407497581951,-58.9619890616024));
#47992=CARTESIAN_POINT('Ctrl Pts',(14.0817963392215,6.86488035175096,-59.1970713693669));
#47993=CARTESIAN_POINT('Ctrl Pts',(14.0817453597218,7.04752046534795,-59.6089408651268));
#47994=CARTESIAN_POINT('Ctrl Pts',(14.0828023551031,7.44003213478346,-60.4448202950792));
#47995=CARTESIAN_POINT('Ctrl Pts',(14.0858669857287,7.93746207099117,-61.4178104786779));
#47996=CARTESIAN_POINT('Ctrl Pts',(14.0894545601233,8.46103266591766,-62.4033076833214));
#47997=CARTESIAN_POINT('Ctrl Pts',(14.0914184630386,8.76069829853051,-62.9612408477037));
#47998=CARTESIAN_POINT('Ctrl Pts',(14.0925922460478,8.96077987034812,-63.3344945335607));
#47999=CARTESIAN_POINT('Ctrl Pts',(14.0933353002373,9.09412300562768,-63.5836692652343));
#48000=CARTESIAN_POINT('Ctrl Pts',(14.0939919971598,9.22718035069599,-63.8332859109708));
#48001=CARTESIAN_POINT('Ctrl Pts',(14.0944870410185,9.34305914081278,-64.0521290136193));
#48002=CARTESIAN_POINT('Ctrl Pts',(14.0947422228291,9.40906933161946,-64.1773000676098));
#48003=CARTESIAN_POINT('Ctrl Pts',(14.0950967381913,9.50784824011138,-64.3651616698595));
#48004=CARTESIAN_POINT('Ctrl Pts',(14.0953227844898,9.58964162844254,-64.5219739377058));
#48005=CARTESIAN_POINT('Ctrl Pts',(14.0956028563449,9.72395560691955,-64.7816511915711));
#48006=CARTESIAN_POINT('Ctrl Pts',(14.0958535991115,9.85473427639552,-65.0336275755987));
#48007=CARTESIAN_POINT('Ctrl Pts',(14.0962351499526,10.1206663563831,-65.5428821753181));
#48008=CARTESIAN_POINT('Ctrl Pts',(14.0965914144919,10.5834552915213,-66.421634553396));
#48009=CARTESIAN_POINT('Ctrl Pts',(14.0964307007463,11.5110342044253,-68.1599880905661));
#48010=CARTESIAN_POINT('Ctrl Pts',(14.0956266991408,12.3085214622441,-69.638494485163));
#48011=CARTESIAN_POINT('Ctrl Pts',(14.0956363216235,12.9117270788187,-70.7729400381487));
#48012=CARTESIAN_POINT('Ctrl Pts',(14.0956420689467,13.0449809453102,-71.0235492813001));
#48013=CARTESIAN_POINT('Ctrl Pts',(14.0956493556449,13.3120603585623,-71.5258457831659));
#48014=CARTESIAN_POINT('Ctrl Pts',(14.0956490445603,13.6454375622873,-72.1528340724319));
#48015=CARTESIAN_POINT('Ctrl Pts',(14.0956468516569,14.0454532421441,-72.9051544342605));
#48016=CARTESIAN_POINT('Ctrl Pts',(14.0956338135297,14.8450986579214,-74.4090765669485));
#48017=CARTESIAN_POINT('Ctrl Pts',(14.0955950884391,15.5110363957072,-75.6615435151467));
#48018=CARTESIAN_POINT('Ctrl Pts',(14.0955821654805,16.4807637197097,-77.4853390728469));
#48019=CARTESIAN_POINT('Ctrl Pts',(14.0955755061043,16.9172399919993,-78.3062334631458));
#48020=CARTESIAN_POINT('Ctrl Pts',(14.0955755061044,17.3537615793888,-79.127211165244));
#48021=CARTESIAN_POINT('Ctrl Pts',(16.9149146750659,4.07897667199088,24.8306334110303));
#48022=CARTESIAN_POINT('Ctrl Pts',(16.9149651977252,4.07897662056641,24.7817540574022));
#48023=CARTESIAN_POINT('Ctrl Pts',(16.9150181737118,4.0789765654222,24.7328757294337));
#48024=CARTESIAN_POINT('Ctrl Pts',(16.9156442730076,4.07897597177255,24.1822680919074));
#48025=CARTESIAN_POINT('Ctrl Pts',(16.9161269734332,4.07897518447184,23.1781399571955));
#48026=CARTESIAN_POINT('Ctrl Pts',(16.9172433640999,4.07897211690891,21.1695412597421));
#48027=CARTESIAN_POINT('Ctrl Pts',(16.9214155178135,4.07896883877421,19.6654077412023));
#48028=CARTESIAN_POINT('Ctrl Pts',(16.9302509496875,4.07896362085564,18.4143674188174));
#48029=CARTESIAN_POINT('Ctrl Pts',(16.9344872446245,4.07896071419103,17.911549791888));
#48030=CARTESIAN_POINT('Ctrl Pts',(16.9451259341652,4.07895312756752,16.9075638897551));
#48031=CARTESIAN_POINT('Ctrl Pts',(16.9679426050505,4.07893661648641,15.1537589849107));
#48032=CARTESIAN_POINT('Ctrl Pts',(16.9896349955101,4.0789273818902,13.652067309321));
#48033=CARTESIAN_POINT('Ctrl Pts',(17.003230380445,4.07892843819468,12.3976224720681));
#48034=CARTESIAN_POINT('Ctrl Pts',(17.0087877338512,4.0789296402581,11.8966775230641));
#48035=CARTESIAN_POINT('Ctrl Pts',(17.0201128766379,4.07893398003655,10.8948445658532));
#48036=CARTESIAN_POINT('Ctrl Pts',(17.0341306376338,4.07894601370972,9.6423540468266));
#48037=CARTESIAN_POINT('Ctrl Pts',(17.0489049863049,4.07896057755439,8.13790518564467));
#48038=CARTESIAN_POINT('Ctrl Pts',(17.056231342848,4.0789732683848,7.13321645454046));
#48039=CARTESIAN_POINT('Ctrl Pts',(17.0596285869194,4.07897831227912,6.50535580676845));
#48040=CARTESIAN_POINT('Ctrl Pts',(17.0612262769992,4.07917336989423,6.25763836117411));
#48041=CARTESIAN_POINT('Ctrl Pts',(17.0651710787483,4.08018959764778,5.7592455610475));
#48042=CARTESIAN_POINT('Ctrl Pts',(17.0734407068839,4.08324547128552,4.88428910557113));
#48043=CARTESIAN_POINT('Ctrl Pts',(17.0904584133639,4.09135539448048,3.1220081935595));
#48044=CARTESIAN_POINT('Ctrl Pts',(17.0891533677877,4.09145541777562,1.59973877304789));
#48045=CARTESIAN_POINT('Ctrl Pts',(17.0646709071443,4.07817954636044,0.522128338721078));
#48046=CARTESIAN_POINT('Ctrl Pts',(17.0614837486151,4.07644673010588,0.392785044077598));
#48047=CARTESIAN_POINT('Ctrl Pts',(17.0541257053017,4.0724504864719,0.135292485977696));
#48048=CARTESIAN_POINT('Ctrl Pts',(17.0388178453858,4.06413593022721,-0.314140200815017));
#48049=CARTESIAN_POINT('Ctrl Pts',(17.0110024464137,4.0489904422446,-0.951871992683431));
#48050=CARTESIAN_POINT('Ctrl Pts',(16.9709419512572,4.02715354110494,-1.71113231692929));
#48051=CARTESIAN_POINT('Ctrl Pts',(16.912684360406,3.99528529045317,-2.7160831512387));
#48052=CARTESIAN_POINT('Ctrl Pts',(16.8377628728703,3.95432262381237,-3.95990686830802));
#48053=CARTESIAN_POINT('Ctrl Pts',(16.7915419611338,3.92943076972257,-4.94437343056028));
#48054=CARTESIAN_POINT('Ctrl Pts',(16.772086427439,3.9194044335412,-5.55738411087098));
#48055=CARTESIAN_POINT('Ctrl Pts',(16.7648299758058,3.91568536083192,-5.80596409311825));
#48056=CARTESIAN_POINT('Ctrl Pts',(16.7521031374105,3.90937504184032,-6.30221922227335));
#48057=CARTESIAN_POINT('Ctrl Pts',(16.7342146873742,3.90103532864856,-7.17351055723086));
#48058=CARTESIAN_POINT('Ctrl Pts',(16.7188093989426,3.89544229392706,-8.42216908296638));
#48059=CARTESIAN_POINT('Ctrl Pts',(16.7105978259963,3.8942327556059,-9.6742176186002));
#48060=CARTESIAN_POINT('Ctrl Pts',(16.7052879353651,3.89351915368516,-10.5507039889754));
#48061=CARTESIAN_POINT('Ctrl Pts',(16.7019251356697,3.89283922134315,-11.0514122978929));
#48062=CARTESIAN_POINT('Ctrl Pts',(16.7000571407005,3.89235689075373,-11.3016868957108));
#48063=CARTESIAN_POINT('Ctrl Pts',(16.6985494828742,3.89192044803081,-11.4901024956647));
#48064=CARTESIAN_POINT('Ctrl Pts',(16.6975614038115,3.89164881404471,-11.6155271159647));
#48065=CARTESIAN_POINT('Ctrl Pts',(16.6956971873959,3.89118926092637,-11.8667984874337));
#48066=CARTESIAN_POINT('Ctrl Pts',(16.6927173666452,3.89059333721637,-12.305622960348));
#48067=CARTESIAN_POINT('Ctrl Pts',(16.6878322157708,3.89014397323601,-13.181630887958));
#48068=CARTESIAN_POINT('Ctrl Pts',(16.6834373461523,3.89110638138056,-14.4297904636907));
#48069=CARTESIAN_POINT('Ctrl Pts',(16.6816042897392,3.89263633585584,-15.5548111776018));
#48070=CARTESIAN_POINT('Ctrl Pts',(16.6808466165555,3.89341434739833,-16.3077059042397));
#48071=CARTESIAN_POINT('Ctrl Pts',(16.6804318274288,3.89383440847301,-16.8105532211299));
#48072=CARTESIAN_POINT('Ctrl Pts',(16.6802159758175,3.89399167832577,-17.1889053690298));
#48073=CARTESIAN_POINT('Ctrl Pts',(16.6800358900155,3.89399901650942,-17.5042315594726));
#48074=CARTESIAN_POINT('Ctrl Pts',(16.6799767886698,3.89401121920815,-17.628572830162));
#48075=CARTESIAN_POINT('Ctrl Pts',(16.6799068875002,3.89407032502083,-17.8777057176927));
#48076=CARTESIAN_POINT('Ctrl Pts',(16.679913398416,3.89417129025278,-18.1269066907719));
#48077=CARTESIAN_POINT('Ctrl Pts',(16.6799851027977,3.89430841468651,-18.3763595048988));
#48078=CARTESIAN_POINT('Ctrl Pts',(16.6800590290734,3.89440466408374,-18.5323341229066));
#48079=CARTESIAN_POINT('Ctrl Pts',(16.6801339494268,3.89448767657968,-18.6571673554093));
#48080=CARTESIAN_POINT('Ctrl Pts',(16.6801984108401,3.89455213286529,-18.7508154517068));
#48081=CARTESIAN_POINT('Ctrl Pts',(16.6802589473794,3.89460735325547,-18.8288767069996));
#48082=CARTESIAN_POINT('Ctrl Pts',(16.6803111947214,3.89465248203599,-18.8913377344271));
#48083=CARTESIAN_POINT('Ctrl Pts',(16.6807786103057,3.89503986621869,-19.4223275899097));
#48084=CARTESIAN_POINT('Ctrl Pts',(16.6824568240971,3.89575916697941,-20.439776571058));
#48085=CARTESIAN_POINT('Ctrl Pts',(16.6864874400154,3.89574282887653,-21.9492402018461));
#48086=CARTESIAN_POINT('Ctrl Pts',(16.6900714332117,3.89373179158201,-22.9605693115645));
#48087=CARTESIAN_POINT('Ctrl Pts',(16.6924571036858,3.89164348899801,-23.5925093952893));
#48088=CARTESIAN_POINT('Ctrl Pts',(16.6934692462877,3.89070366993123,-23.8431111230596));
#48089=CARTESIAN_POINT('Ctrl Pts',(16.6957568714141,3.88838138009332,-24.344487023896));
#48090=CARTESIAN_POINT('Ctrl Pts',(16.7003586297709,3.88334097133003,-25.2230673320503));
#48091=CARTESIAN_POINT('Ctrl Pts',(16.7081644394295,3.87406933870138,-26.479880505014));
#48092=CARTESIAN_POINT('Ctrl Pts',(16.7177935931692,3.86276510361262,-27.9870543427907));
#48093=CARTESIAN_POINT('Ctrl Pts',(16.7233193953658,3.85669854106861,-28.9885471470297));
#48094=CARTESIAN_POINT('Ctrl Pts',(16.7258535540266,3.85430623269711,-29.5503462654312));
#48095=CARTESIAN_POINT('Ctrl Pts',(16.7263168576138,3.85372101518925,-29.6770508651879));
#48096=CARTESIAN_POINT('Ctrl Pts',(16.7268790701398,3.85237600033726,-29.9292284771417));
#48097=CARTESIAN_POINT('Ctrl Pts',(16.7269982851966,3.84959656653962,-30.3706843069735));
#48098=CARTESIAN_POINT('Ctrl Pts',(16.7245363433686,3.84283451302849,-31.2514329399704));
#48099=CARTESIAN_POINT('Ctrl Pts',(16.7175349032075,3.83231245730799,-32.5042685138076));
#48100=CARTESIAN_POINT('Ctrl Pts',(16.7174964875878,3.82765847457322,-33.7475171559131));
#48101=CARTESIAN_POINT('Ctrl Pts',(16.7287497672298,3.83172266819031,-34.7351162525985));
#48102=CARTESIAN_POINT('Ctrl Pts',(16.7392901152939,3.83699566582681,-35.2264235346435));
#48103=CARTESIAN_POINT('Ctrl Pts',(16.7495253964372,3.84242433343839,-35.594735035358));
#48104=CARTESIAN_POINT('Ctrl Pts',(16.757597882556,3.84675307570527,-35.839518727925));
#48105=CARTESIAN_POINT('Ctrl Pts',(16.7777503546989,3.8577716135805,-36.3310864798155));
#48106=CARTESIAN_POINT('Ctrl Pts',(16.8218420325679,3.88242389109144,-37.1933485584074));
#48107=CARTESIAN_POINT('Ctrl Pts',(16.932759743038,3.94586133891672,-38.9293707178973));
#48108=CARTESIAN_POINT('Ctrl Pts',(17.0248342837548,4.00264192802993,-40.4465622192129));
#48109=CARTESIAN_POINT('Ctrl Pts',(17.0548534638343,4.02815505439204,-41.7334021407456));
#48110=CARTESIAN_POINT('Ctrl Pts',(17.0617900002719,4.0319026324534,-42.1316506025687));
#48111=CARTESIAN_POINT('Ctrl Pts',(17.0675846318347,4.03125442328988,-42.6479199311238));
#48112=CARTESIAN_POINT('Ctrl Pts',(17.0712609357292,4.02799382577384,-43.1619316799385));
#48113=CARTESIAN_POINT('Ctrl Pts',(17.0723042754547,4.02067663238492,-43.7952514515751));
#48114=CARTESIAN_POINT('Ctrl Pts',(17.0691441837673,4.01218212961586,-44.5420517787092));
#48115=CARTESIAN_POINT('Ctrl Pts',(17.0638977866498,4.00960088327479,-45.1523786175568));
#48116=CARTESIAN_POINT('Ctrl Pts',(17.0588510491071,4.01255629312146,-45.6331084565198));
#48117=CARTESIAN_POINT('Ctrl Pts',(17.0547671612117,4.01789369453871,-45.9899028044721));
#48118=CARTESIAN_POINT('Ctrl Pts',(17.0505511977916,4.02690254845307,-46.3428518603264));
#48119=CARTESIAN_POINT('Ctrl Pts',(17.0449963708357,4.0444916672167,-46.8082413517047));
#48120=CARTESIAN_POINT('Ctrl Pts',(17.0410653648893,4.06483665626451,-47.1513493295494));
#48121=CARTESIAN_POINT('Ctrl Pts',(17.0376999000655,4.09092409317607,-47.4917006453254));
#48122=CARTESIAN_POINT('Ctrl Pts',(17.0351503357226,4.11065377767826,-47.7400159897784));
#48123=CARTESIAN_POINT('Ctrl Pts',(17.0289836561659,4.15212670812739,-48.2235284994233));
#48124=CARTESIAN_POINT('Ctrl Pts',(17.0157609678126,4.23337229511935,-49.0717867229332));
#48125=CARTESIAN_POINT('Ctrl Pts',(16.9919464655623,4.37612993656612,-50.2688586222703));
#48126=CARTESIAN_POINT('Ctrl Pts',(16.9626550785882,4.60038614223337,-51.6886041014199));
#48127=CARTESIAN_POINT('Ctrl Pts',(16.9469695415295,4.79192210163469,-52.6222521044942));
#48128=CARTESIAN_POINT('Ctrl Pts',(16.9397627089671,4.92703807383931,-53.2035467307471));
#48129=CARTESIAN_POINT('Ctrl Pts',(16.9369146755773,4.98364117268894,-53.440722973793));
#48130=CARTESIAN_POINT('Ctrl Pts',(16.9314745786511,5.10264327431612,-53.9148837756041));
#48131=CARTESIAN_POINT('Ctrl Pts',(16.922607945119,5.32672256459404,-54.747790768806));
#48132=CARTESIAN_POINT('Ctrl Pts',(16.9076194942708,5.83458111882296,-56.4192674493408));
#48133=CARTESIAN_POINT('Ctrl Pts',(16.8999356945503,6.36284906266773,-57.8524303513783));
#48134=CARTESIAN_POINT('Ctrl Pts',(16.8974805636034,6.77168043251319,-58.8580127366239));
#48135=CARTESIAN_POINT('Ctrl Pts',(16.8972648103021,6.81915928483857,-58.9733155701948));
#48136=CARTESIAN_POINT('Ctrl Pts',(16.8969802126965,6.91846895958593,-59.2089983557977));
#48137=CARTESIAN_POINT('Ctrl Pts',(16.896917944298,7.09828865112667,-59.6220435374114));
#48138=CARTESIAN_POINT('Ctrl Pts',(16.8982412500171,7.48383323680778,-60.4592532906179));
#48139=CARTESIAN_POINT('Ctrl Pts',(16.9021949253572,7.97127227018086,-61.4324272317552));
#48140=CARTESIAN_POINT('Ctrl Pts',(16.9067378748187,8.48444954617013,-62.4167904717263));
#48141=CARTESIAN_POINT('Ctrl Pts',(16.9091943680861,8.77844615812734,-62.9736158842109));
#48142=CARTESIAN_POINT('Ctrl Pts',(16.9106594487652,8.97493743578547,-63.3459133746306));
#48143=CARTESIAN_POINT('Ctrl Pts',(16.911577598122,9.10595214562086,-63.5943917097937));
#48144=CARTESIAN_POINT('Ctrl Pts',(16.9124086561989,9.23676839272102,-63.8432182552755));
#48145=CARTESIAN_POINT('Ctrl Pts',(16.9130215853273,9.35080672825771,-64.0612843748139));
#48146=CARTESIAN_POINT('Ctrl Pts',(16.9133375675906,9.41579986074407,-64.1859854625765));
#48147=CARTESIAN_POINT('Ctrl Pts',(16.9137747317867,9.51309088246509,-64.3731159900114));
#48148=CARTESIAN_POINT('Ctrl Pts',(16.9140652969669,9.59371446454079,-64.529259559438));
#48149=CARTESIAN_POINT('Ctrl Pts',(16.9144167279272,9.72622726928115,-64.787754105224));
#48150=CARTESIAN_POINT('Ctrl Pts',(16.9147363867585,9.85549051025473,-65.0387769469754));
#48151=CARTESIAN_POINT('Ctrl Pts',(16.9152124179813,10.1188956091204,-65.5461829041274));
#48152=CARTESIAN_POINT('Ctrl Pts',(16.915685918939,10.5787468651793,-66.4222485940659));
#48153=CARTESIAN_POINT('Ctrl Pts',(16.9154868474475,11.5052148408086,-68.1572132791816));
#48154=CARTESIAN_POINT('Ctrl Pts',(16.914587493052,12.3063136758984,-69.6364416210659));
#48155=CARTESIAN_POINT('Ctrl Pts',(16.914633424635,12.9106480847908,-70.7731930265593));
#48156=CARTESIAN_POINT('Ctrl Pts',(16.9146383518857,13.0437985626505,-71.0236338700303));
#48157=CARTESIAN_POINT('Ctrl Pts',(16.9146470758778,13.3108863200786,-71.5259878708771));
#48158=CARTESIAN_POINT('Ctrl Pts',(16.9146570930598,13.6441973881165,-72.1528910927276));
#48159=CARTESIAN_POINT('Ctrl Pts',(16.9146600572098,14.0442047153699,-72.9052049952523));
#48160=CARTESIAN_POINT('Ctrl Pts',(16.9146582758106,14.8438344056538,-74.4090767084999));
#48161=CARTESIAN_POINT('Ctrl Pts',(16.9146627373669,15.5097822694014,-75.6615387328973));
#48162=CARTESIAN_POINT('Ctrl Pts',(16.9146737757476,16.4795080936937,-77.4853610045239));
#48163=CARTESIAN_POINT('Ctrl Pts',(16.9146794696564,16.9159645367713,-78.3062333142393));
#48164=CARTESIAN_POINT('Ctrl Pts',(16.9146794696565,17.3524861241607,-79.1272110163379));
#48165=CARTESIAN_POINT('Ctrl Pts',(19.7316905697294,4.07935448938162,24.830633935914));
#48166=CARTESIAN_POINT('Ctrl Pts',(19.731749408434,4.07935450933349,24.7817545980753));
#48167=CARTESIAN_POINT('Ctrl Pts',(19.73181113422,4.07935453691546,24.7328763236576));
#48168=CARTESIAN_POINT('Ctrl Pts',(19.7325392880933,4.07935456156444,24.1822676113171));
#48169=CARTESIAN_POINT('Ctrl Pts',(19.7330915102349,4.07935241872843,23.1781290371801));
#48170=CARTESIAN_POINT('Ctrl Pts',(19.734386066713,4.07935125552519,21.16952961444));
#48171=CARTESIAN_POINT('Ctrl Pts',(19.7392243248583,4.07934829382183,19.6653703770963));
#48172=CARTESIAN_POINT('Ctrl Pts',(19.7495130845821,4.0793521589517,18.4143189930037));
#48173=CARTESIAN_POINT('Ctrl Pts',(19.7544484885452,4.07935455477466,17.9115008539396));
#48174=CARTESIAN_POINT('Ctrl Pts',(19.766839498765,4.07935982008661,16.9075083417517));
#48175=CARTESIAN_POINT('Ctrl Pts',(19.7934209949296,4.07937279166992,15.1536950428428));
#48176=CARTESIAN_POINT('Ctrl Pts',(19.8186621736851,4.07937766165514,13.6519395529123));
#48177=CARTESIAN_POINT('Ctrl Pts',(19.834506757662,4.07938630977482,12.3974618327996));
#48178=CARTESIAN_POINT('Ctrl Pts',(19.8409870511261,4.07939063207221,11.896506822936));
#48179=CARTESIAN_POINT('Ctrl Pts',(19.8542109084696,4.07940376416714,10.8946632038776));
#48180=CARTESIAN_POINT('Ctrl Pts',(19.8705476717958,4.07941204516816,9.64212444575423));
#48181=CARTESIAN_POINT('Ctrl Pts',(19.887804112216,4.07942989188445,8.1376208453681));
#48182=CARTESIAN_POINT('Ctrl Pts',(19.8963059268321,4.07942448829874,7.13290173233056));
#48183=CARTESIAN_POINT('Ctrl Pts',(19.9002643271173,4.07942588898193,6.50490471479));
#48184=CARTESIAN_POINT('Ctrl Pts',(19.9018435195747,4.07940107803301,6.25434123804895));
#48185=CARTESIAN_POINT('Ctrl Pts',(19.9049508975073,4.07926731921548,5.75286295607368));
#48186=CARTESIAN_POINT('Ctrl Pts',(19.9100753780821,4.07884861781295,4.87399706060382));
#48187=CARTESIAN_POINT('Ctrl Pts',(19.9179299517214,4.07773750234611,3.11401396013838));
#48188=CARTESIAN_POINT('Ctrl Pts',(19.9160327000162,4.07760589988365,1.60935695765296));
#48189=CARTESIAN_POINT('Ctrl Pts',(19.9067271157157,4.07942683025897,0.552365774248749));
#48190=CARTESIAN_POINT('Ctrl Pts',(19.9055276056199,4.07967354567833,0.426638999775616));
#48191=CARTESIAN_POINT('Ctrl Pts',(19.9027400321877,4.08023663483943,0.175238431751414));
#48192=CARTESIAN_POINT('Ctrl Pts',(19.8969210328009,4.0814046752406,-0.264300184378953));
#48193=CARTESIAN_POINT('Ctrl Pts',(19.8861804513372,4.08348190805184,-0.891342867381702));
#48194=CARTESIAN_POINT('Ctrl Pts',(19.8707003983181,4.08640779973263,-1.64276387359526));
#48195=CARTESIAN_POINT('Ctrl Pts',(19.8478739867681,4.09051387445938,-2.64390761035535));
#48196=CARTESIAN_POINT('Ctrl Pts',(19.8184602098816,4.09548305738938,-3.89512046614111));
#48197=CARTESIAN_POINT('Ctrl Pts',(19.7995658555875,4.09828589820852,-4.8986886576812));
#48198=CARTESIAN_POINT('Ctrl Pts',(19.7910048215388,4.09935782538962,-5.52762127940719));
#48199=CARTESIAN_POINT('Ctrl Pts',(19.7876614372912,4.09974712809936,-5.77894874591882));
#48200=CARTESIAN_POINT('Ctrl Pts',(19.7813542100678,4.10035194775432,-6.28202511088013));
#48201=CARTESIAN_POINT('Ctrl Pts',(19.7712007143656,4.10100695113103,-7.16258996222176));
#48202=CARTESIAN_POINT('Ctrl Pts',(19.7590139140574,4.10104245326206,-8.42041961138705));
#48203=CARTESIAN_POINT('Ctrl Pts',(19.7493961943797,4.10061964535909,-9.67517807562287));
#48204=CARTESIAN_POINT('Ctrl Pts',(19.7437605557968,4.10047778183881,-10.5504750025485));
#48205=CARTESIAN_POINT('Ctrl Pts',(19.7407885077789,4.10049626661812,-11.0495578008507));
#48206=CARTESIAN_POINT('Ctrl Pts',(19.7393771920844,4.10054805882285,-11.2987018195911));
#48207=CARTESIAN_POINT('Ctrl Pts',(19.7383407909855,4.10060663713044,-11.4861849899995));
#48208=CARTESIAN_POINT('Ctrl Pts',(19.737667358513,4.10064799464512,-11.6122859436781));
#48209=CARTESIAN_POINT('Ctrl Pts',(19.7364020395687,4.10073774603204,-11.8641351428825));
#48210=CARTESIAN_POINT('Ctrl Pts',(19.7343937719702,4.10091189806865,-12.3042414007394));
#48211=CARTESIAN_POINT('Ctrl Pts',(19.7311318713114,4.10131291049498,-13.1821365759618));
#48212=CARTESIAN_POINT('Ctrl Pts',(19.7283662371774,4.10196984298857,-14.4319944615007));
#48213=CARTESIAN_POINT('Ctrl Pts',(19.7273504799056,4.10247530938435,-15.5570659964618));
#48214=CARTESIAN_POINT('Ctrl Pts',(19.7269580604332,4.10270448918149,-16.309427149594));
#48215=CARTESIAN_POINT('Ctrl Pts',(19.7267559570064,4.10282451667879,-16.8117648997344));
#48216=CARTESIAN_POINT('Ctrl Pts',(19.7266245428868,4.10286667409472,-17.1895525871661));
#48217=CARTESIAN_POINT('Ctrl Pts',(19.7265160857273,4.10287396504927,-17.5043370351011));
#48218=CARTESIAN_POINT('Ctrl Pts',(19.7265064163444,4.10288245535858,-17.6288438629665));
#48219=CARTESIAN_POINT('Ctrl Pts',(19.7266103048185,4.10291733055289,-17.8780646836674));
#48220=CARTESIAN_POINT('Ctrl Pts',(19.7268781409595,4.10297412970388,-18.1274070504594));
#48221=CARTESIAN_POINT('Ctrl Pts',(19.7272886495818,4.10304802339381,-18.3769304058717));
#48222=CARTESIAN_POINT('Ctrl Pts',(19.7275955378439,4.10309899866357,-18.5329468870759));
#48223=CARTESIAN_POINT('Ctrl Pts',(19.7278690490042,4.10314218015061,-18.6578030814957));
#48224=CARTESIAN_POINT('Ctrl Pts',(19.7280866533016,4.10317537676589,-18.7514657853085));
#48225=CARTESIAN_POINT('Ctrl Pts',(19.7282776058114,4.10320352312179,-18.8295358423443));
#48226=CARTESIAN_POINT('Ctrl Pts',(19.7284359336775,4.10322629604098,-18.8920023401028));
#48227=CARTESIAN_POINT('Ctrl Pts',(19.7298109404199,4.10342047933287,-19.4230282642657));
#48228=CARTESIAN_POINT('Ctrl Pts',(19.7331572114862,4.10377137295389,-20.4401908236404));
#48229=CARTESIAN_POINT('Ctrl Pts',(19.7369494432878,4.10344189876844,-21.9484042415267));
#48230=CARTESIAN_POINT('Ctrl Pts',(19.7358394579444,4.10198821210429,-22.9582963768966));
#48231=CARTESIAN_POINT('Ctrl Pts',(19.7333544804705,4.10053776327126,-23.5891593966175));
#48232=CARTESIAN_POINT('Ctrl Pts',(19.7321760621842,4.09988629850747,-23.8391695437685));
#48233=CARTESIAN_POINT('Ctrl Pts',(19.7290616593307,4.09829137473462,-24.339613135241));
#48234=CARTESIAN_POINT('Ctrl Pts',(19.7219239461885,4.09484772201759,-25.2168463500179));
#48235=CARTESIAN_POINT('Ctrl Pts',(19.7081538012807,4.08854495688428,-26.4727754554355));
#48236=CARTESIAN_POINT('Ctrl Pts',(19.6910680763066,4.08070275774671,-27.9803984717941));
#48237=CARTESIAN_POINT('Ctrl Pts',(19.682181615747,4.07644882190675,-28.9833847666746));
#48238=CARTESIAN_POINT('Ctrl Pts',(19.6789063358229,4.07474992627841,-29.5461747236964));
#48239=CARTESIAN_POINT('Ctrl Pts',(19.6781643290644,4.07439003395089,-29.6713449100555));
#48240=CARTESIAN_POINT('Ctrl Pts',(19.6765979656164,4.07370056899209,-29.9217094990869));
#48241=CARTESIAN_POINT('Ctrl Pts',(19.6736761126337,4.07257592588719,-30.3601050028827));
#48242=CARTESIAN_POINT('Ctrl Pts',(19.6674110815844,4.07062996206372,-31.2375938981368));
#48243=CARTESIAN_POINT('Ctrl Pts',(19.6589600545705,4.06853967488443,-32.4926327690216));
#48244=CARTESIAN_POINT('Ctrl Pts',(19.6554404212508,4.06698916538458,-33.7476184880732));
#48245=CARTESIAN_POINT('Ctrl Pts',(19.6580885878912,4.065868905903,-34.7503127027266));
#48246=CARTESIAN_POINT('Ctrl Pts',(19.6616531760529,4.06529455477844,-35.2511296095717));
#48247=CARTESIAN_POINT('Ctrl Pts',(19.665317861005,4.06485642982007,-35.6274105267477));
#48248=CARTESIAN_POINT('Ctrl Pts',(19.6682557022879,4.06452735058168,-35.8799831172533));
#48249=CARTESIAN_POINT('Ctrl Pts',(19.6759570604248,4.06377152046226,-36.3837372228955));
#48250=CARTESIAN_POINT('Ctrl Pts',(19.6938393828171,4.062297043252,-37.26353505748));
#48251=CARTESIAN_POINT('Ctrl Pts',(19.7419383911154,4.0591779187408,-39.014885353225));
#48252=CARTESIAN_POINT('Ctrl Pts',(19.787835736678,4.05803854631324,-40.5132616492215));
#48253=CARTESIAN_POINT('Ctrl Pts',(19.8076592637585,4.06081185444712,-41.7644661924603));
#48254=CARTESIAN_POINT('Ctrl Pts',(19.8127401621175,4.05882529185606,-42.1583425608284));
#48255=CARTESIAN_POINT('Ctrl Pts',(19.8182210067088,4.0527771384098,-42.6673496342845));
#48256=CARTESIAN_POINT('Ctrl Pts',(19.8229989227837,4.04528573324617,-43.1756057463211));
#48257=CARTESIAN_POINT('Ctrl Pts',(19.8278103195324,4.03460887261985,-43.8030097224572));
#48258=CARTESIAN_POINT('Ctrl Pts',(19.8323913480545,4.02410301328588,-44.545389174707));
#48259=CARTESIAN_POINT('Ctrl Pts',(19.8357640253749,4.02076109607437,-45.1540565174229));
#48260=CARTESIAN_POINT('Ctrl Pts',(19.8383792636965,4.02326144297558,-45.6346936020065));
#48261=CARTESIAN_POINT('Ctrl Pts',(19.8404448287581,4.02822588709096,-45.992036286084));
#48262=CARTESIAN_POINT('Ctrl Pts',(19.8426848273797,4.03673804444104,-46.3461583074312));
#48263=CARTESIAN_POINT('Ctrl Pts',(19.8459593924335,4.0534007785814,-46.8139160110249));
#48264=CARTESIAN_POINT('Ctrl Pts',(19.8490102862601,4.0725780024727,-47.1597454447569));
#48265=CARTESIAN_POINT('Ctrl Pts',(19.8524421822243,4.09707767505399,-47.5033352104608));
#48266=CARTESIAN_POINT('Ctrl Pts',(19.8549821621875,4.1154308208764,-47.7517883290858));
#48267=CARTESIAN_POINT('Ctrl Pts',(19.8609128581012,4.15406663927081,-48.2364844060615));
#48268=CARTESIAN_POINT('Ctrl Pts',(19.8730354455658,4.22979398838813,-49.0857137837747));
#48269=CARTESIAN_POINT('Ctrl Pts',(19.8928105255737,4.36366137946812,-50.2829982698093));
#48270=CARTESIAN_POINT('Ctrl Pts',(19.9110158584986,4.57797201329531,-51.7001736054087));
#48271=CARTESIAN_POINT('Ctrl Pts',(19.9140889565939,4.76458586101715,-52.6302330956112));
#48272=CARTESIAN_POINT('Ctrl Pts',(19.9113288594367,4.89772463046567,-53.2086743982499));
#48273=CARTESIAN_POINT('Ctrl Pts',(19.9097330121159,4.9537090997724,-53.4449852387809));
#48274=CARTESIAN_POINT('Ctrl Pts',(19.9047889632458,5.07187747957425,-53.917432226375));
#48275=CARTESIAN_POINT('Ctrl Pts',(19.8921640234306,5.29553920307492,-54.7478003303291));
#48276=CARTESIAN_POINT('Ctrl Pts',(19.8551417665773,5.8059701002291,-56.4156742081449));
#48277=CARTESIAN_POINT('Ctrl Pts',(19.8179048087849,6.33969776481573,-57.8484357420634));
#48278=CARTESIAN_POINT('Ctrl Pts',(19.8020555987685,6.75149430652742,-58.8550852625136));
#48279=CARTESIAN_POINT('Ctrl Pts',(19.8000495326012,6.79916648367612,-58.9701141739038));
#48280=CARTESIAN_POINT('Ctrl Pts',(19.7961289086579,6.89901093073692,-59.2055141726096));
#48281=CARTESIAN_POINT('Ctrl Pts',(19.7893504671894,7.07984491459817,-59.6180253267165));
#48282=CARTESIAN_POINT('Ctrl Pts',(19.7763661962944,7.46788194576182,-60.4545612854285));
#48283=CARTESIAN_POINT('Ctrl Pts',(19.7630048641413,7.95890168870625,-61.4275068436025));
#48284=CARTESIAN_POINT('Ctrl Pts',(19.7516453032531,8.47575416449995,-62.4121765161391));
#48285=CARTESIAN_POINT('Ctrl Pts',(19.7460529641767,8.77173687932521,-62.9693603278665));
#48286=CARTESIAN_POINT('Ctrl Pts',(19.7426787391143,8.96948177555833,-63.3419757199963));
#48287=CARTESIAN_POINT('Ctrl Pts',(19.7405303622212,9.10130626640622,-63.590688332912));
#48288=CARTESIAN_POINT('Ctrl Pts',(19.7385146449095,9.23290572032763,-63.8397804006721));
#48289=CARTESIAN_POINT('Ctrl Pts',(19.7368938568286,9.3475829472815,-64.0581101092336));
#48290=CARTESIAN_POINT('Ctrl Pts',(19.736006538874,9.41292900959727,-64.1829707544759));
#48291=CARTESIAN_POINT('Ctrl Pts',(19.734716083465,9.51073577429339,-64.370349741563));
#48292=CARTESIAN_POINT('Ctrl Pts',(19.7337155215584,9.59176751053624,-64.5267201302611));
#48293=CARTESIAN_POINT('Ctrl Pts',(19.7321833122377,9.72490590884203,-64.785616544752));
#48294=CARTESIAN_POINT('Ctrl Pts',(19.7307903414362,9.8546954230295,-65.0369589505087));
#48295=CARTESIAN_POINT('Ctrl Pts',(19.7287090777181,10.1189851698039,-65.5449893060533));
#48296=CARTESIAN_POINT('Ctrl Pts',(19.7266829189429,10.5798955165842,-66.4219623980084));
#48297=CARTESIAN_POINT('Ctrl Pts',(19.7276676576506,11.5068788766144,-68.1580753862004));
#48298=CARTESIAN_POINT('Ctrl Pts',(19.7318934421853,12.3068965513959,-69.6370766309225));
#48299=CARTESIAN_POINT('Ctrl Pts',(19.7317655953638,12.9109104740048,-70.7730753050621));
#48300=CARTESIAN_POINT('Ctrl Pts',(19.731747534186,13.0441058105992,-71.0235794241767));
#48301=CARTESIAN_POINT('Ctrl Pts',(19.7317183219463,13.3112072443434,-71.5259251673118));
#48302=CARTESIAN_POINT('Ctrl Pts',(19.7316918915079,13.6445569377086,-72.1528687312019));
#48303=CARTESIAN_POINT('Ctrl Pts',(19.7316858882025,14.0445750481121,-72.9051951966746));
#48304=CARTESIAN_POINT('Ctrl Pts',(19.731701553499,14.8442122836675,-74.4090975500849));
#48305=CARTESIAN_POINT('Ctrl Pts',(19.7317226301597,15.510148776986,-75.6615557162998));
#48306=CARTESIAN_POINT('Ctrl Pts',(19.7317044242158,16.479871690132,-77.4853474815518));
#48307=CARTESIAN_POINT('Ctrl Pts',(19.7316950307522,16.9163422836949,-78.3062335121641));
#48308=CARTESIAN_POINT('Ctrl Pts',(19.7316950307521,17.3528638710844,-79.1272112142626));
#48309=CARTESIAN_POINT('Ctrl Pts',(22.0806872581769,4.0817112774535,24.8306369402783));
#48310=CARTESIAN_POINT('Ctrl Pts',(22.0807531893061,4.08171138793248,24.7817576970255));
#48311=CARTESIAN_POINT('Ctrl Pts',(22.0808223364565,4.08171150089068,24.7328795140129));
#48312=CARTESIAN_POINT('Ctrl Pts',(22.0816389036773,4.08171296325905,24.1822720755345));
#48313=CARTESIAN_POINT('Ctrl Pts',(22.0822628297011,4.08171593727744,23.1781363452397));
#48314=CARTESIAN_POINT('Ctrl Pts',(22.0837134257396,4.0817218195251,21.1695390105029));
#48315=CARTESIAN_POINT('Ctrl Pts',(22.0891480761944,4.08173286928369,19.6653832895225));
#48316=CARTESIAN_POINT('Ctrl Pts',(22.1006837454411,4.0817473182421,18.4143332656791));
#48317=CARTESIAN_POINT('Ctrl Pts',(22.106215392913,4.08175442852641,17.9115211063208));
#48318=CARTESIAN_POINT('Ctrl Pts',(22.1201046843955,4.0817733584488,16.9075336614081));
#48319=CARTESIAN_POINT('Ctrl Pts',(22.1498965369521,4.08181298878673,15.1537211775948));
#48320=CARTESIAN_POINT('Ctrl Pts',(22.1782115772056,4.08184803808263,13.6519550007739));
#48321=CARTESIAN_POINT('Ctrl Pts',(22.1959821252523,4.08185640482049,12.3974562400484));
#48322=CARTESIAN_POINT('Ctrl Pts',(22.2032490945125,4.08185823625986,11.8964924068614));
#48323=CARTESIAN_POINT('Ctrl Pts',(22.2180712991417,4.08185590403518,10.8946345861558));
#48324=CARTESIAN_POINT('Ctrl Pts',(22.2364075742634,4.08185096497192,9.64209341000557));
#48325=CARTESIAN_POINT('Ctrl Pts',(22.2557598888455,4.08183561206296,8.13759363954354));
#48326=CARTESIAN_POINT('Ctrl Pts',(22.2653316985992,4.08183262212613,7.13289760894556));
#48327=CARTESIAN_POINT('Ctrl Pts',(22.2697798697298,4.08182891552378,6.50490839933043));
#48328=CARTESIAN_POINT('Ctrl Pts',(22.2714680039726,4.08179307578173,6.25425061006605));
#48329=CARTESIAN_POINT('Ctrl Pts',(22.2745101250835,4.08161068554481,5.75267104405992));
#48330=CARTESIAN_POINT('Ctrl Pts',(22.2789478637005,4.08107443746193,4.87368318059426));
#48331=CARTESIAN_POINT('Ctrl Pts',(22.2842233509257,4.07964539768461,3.11379727390321));
#48332=CARTESIAN_POINT('Ctrl Pts',(22.2823498152796,4.07968863300819,1.60985064855089));
#48333=CARTESIAN_POINT('Ctrl Pts',(22.2778081809785,4.08195512191518,0.553599358401225));
#48334=CARTESIAN_POINT('Ctrl Pts',(22.2772161841593,4.0822448224232,0.427984441741552));
#48335=CARTESIAN_POINT('Ctrl Pts',(22.275838864125,4.08291878036556,0.176781772273433));
#48336=CARTESIAN_POINT('Ctrl Pts',(22.2729491009355,4.08432382985036,-0.262431355723268));
#48337=CARTESIAN_POINT('Ctrl Pts',(22.2676105494159,4.08691133652606,-0.889101992934185));
#48338=CARTESIAN_POINT('Ctrl Pts',(22.2597610041138,4.09064398215328,-1.64029242724309));
#48339=CARTESIAN_POINT('Ctrl Pts',(22.2480116337292,4.09613028427393,-2.64145813674392));
#48340=CARTESIAN_POINT('Ctrl Pts',(22.2320940873357,4.10317395660869,-3.89327783208695));
#48341=CARTESIAN_POINT('Ctrl Pts',(22.2206681795821,4.10740367299369,-4.89747150057058));
#48342=CARTESIAN_POINT('Ctrl Pts',(22.2148552608892,4.10905808987711,-5.52672152324843));
#48343=CARTESIAN_POINT('Ctrl Pts',(22.2125378664224,4.10966736971728,-5.77793552878553));
#48344=CARTESIAN_POINT('Ctrl Pts',(22.2078972997522,4.11071887719346,-6.28095978966975));
#48345=CARTESIAN_POINT('Ctrl Pts',(22.1998362198795,4.11214569764531,-7.16146359659875));
#48346=CARTESIAN_POINT('Ctrl Pts',(22.1887604553002,4.11318625410649,-8.41957491079932));
#48347=CARTESIAN_POINT('Ctrl Pts',(22.1789920192977,4.11333851024897,-9.6750259227349));
#48348=CARTESIAN_POINT('Ctrl Pts',(22.1732201097211,4.11320661362161,-10.5510379086196));
#48349=CARTESIAN_POINT('Ctrl Pts',(22.1702828176501,4.11309903099946,-11.0505969687109));
#48350=CARTESIAN_POINT('Ctrl Pts',(22.1689438897613,4.11304030179607,-11.3000015048504));
#48351=CARTESIAN_POINT('Ctrl Pts',(22.1679877770531,4.11299599543326,-11.4876940375807));
#48352=CARTESIAN_POINT('Ctrl Pts',(22.1673581839659,4.11295442151722,-11.6141016365983));
#48353=CARTESIAN_POINT('Ctrl Pts',(22.1661543332355,4.11282692441663,-11.8664290867861));
#48354=CARTESIAN_POINT('Ctrl Pts',(22.1641885750189,4.1124961281729,-12.3073258727564));
#48355=CARTESIAN_POINT('Ctrl Pts',(22.1608085968938,4.11146884907708,-13.1863892779554));
#48356=CARTESIAN_POINT('Ctrl Pts',(22.1574251842106,4.10930348790506,-14.4367873212243));
#48357=CARTESIAN_POINT('Ctrl Pts',(22.1558729907192,4.10738504447621,-15.5609562570509));
#48358=CARTESIAN_POINT('Ctrl Pts',(22.155340060491,4.10648741718098,-16.3121472359132));
#48359=CARTESIAN_POINT('Ctrl Pts',(22.1551084149864,4.10601442669833,-16.8135559816661));
#48360=CARTESIAN_POINT('Ctrl Pts',(22.1550828627036,4.10582997028817,-17.1904736305975));
#48361=CARTESIAN_POINT('Ctrl Pts',(22.1551183195028,4.1058005333167,-17.5044814660014));
#48362=CARTESIAN_POINT('Ctrl Pts',(22.155179274139,4.10577633105441,-17.6294802209848));
#48363=CARTESIAN_POINT('Ctrl Pts',(22.1554734941708,4.10568791669081,-17.8791216720373));
#48364=CARTESIAN_POINT('Ctrl Pts',(22.1560114778335,4.10554739946089,-18.12893591468));
#48365=CARTESIAN_POINT('Ctrl Pts',(22.1567400996841,4.10537329353691,-18.3787108686903));
#48366=CARTESIAN_POINT('Ctrl Pts',(22.1572692425485,4.10525407920985,-18.5348529247192));
#48367=CARTESIAN_POINT('Ctrl Pts',(22.1577296457834,4.10515479122478,-18.6597699978175));
#48368=CARTESIAN_POINT('Ctrl Pts',(22.1580928061923,4.10507890335121,-18.7534645699545));
#48369=CARTESIAN_POINT('Ctrl Pts',(22.1584092338762,4.10501494381649,-18.8315471216055));
#48370=CARTESIAN_POINT('Ctrl Pts',(22.1586696170516,4.10496364273465,-18.8940160178554));
#48371=CARTESIAN_POINT('Ctrl Pts',(22.1609244923333,4.10452743167003,-19.4250166780277));
#48372=CARTESIAN_POINT('Ctrl Pts',(22.1666117086279,4.10371393162455,-20.4406887452964));
#48373=CARTESIAN_POINT('Ctrl Pts',(22.1728486493173,4.1048750925385,-21.9427050549345));
#48374=CARTESIAN_POINT('Ctrl Pts',(22.1721548195285,4.10870954669947,-22.9457918178194));
#48375=CARTESIAN_POINT('Ctrl Pts',(22.1689681366907,4.11250052261211,-23.5715577180345));
#48376=CARTESIAN_POINT('Ctrl Pts',(22.1674053242735,4.11420424041461,-23.8184716543449));
#48377=CARTESIAN_POINT('Ctrl Pts',(22.1632586022422,4.11833524471003,-24.3141483484936));
#48378=CARTESIAN_POINT('Ctrl Pts',(22.1536481125674,4.12720731324701,-25.184535378242));
#48379=CARTESIAN_POINT('Ctrl Pts',(22.135280394341,4.14306970300957,-26.4361733232101));
#48380=CARTESIAN_POINT('Ctrl Pts',(22.1119075504369,4.16259534336498,-27.9468610752968));
#48381=CARTESIAN_POINT('Ctrl Pts',(22.0998150320629,4.17286510122039,-28.9575801470414));
#48382=CARTESIAN_POINT('Ctrl Pts',(22.095134968522,4.1770426651094,-29.5262025538896));
#48383=CARTESIAN_POINT('Ctrl Pts',(22.0940862306972,4.17796210642411,-29.6513811403136));
#48384=CARTESIAN_POINT('Ctrl Pts',(22.0919769998257,4.17979334736485,-29.9025054603524));
#48385=CARTESIAN_POINT('Ctrl Pts',(22.0882790979027,4.18294814217091,-30.3419115460975));
#48386=CARTESIAN_POINT('Ctrl Pts',(22.0810018498695,4.18900722017071,-31.2218692521629));
#48387=CARTESIAN_POINT('Ctrl Pts',(22.0718693716956,4.19641679166098,-32.480798983417));
#48388=CARTESIAN_POINT('Ctrl Pts',(22.0669315823576,4.20090765113935,-33.7404563518645));
#48389=CARTESIAN_POINT('Ctrl Pts',(22.067020405947,4.20200039738248,-34.7472756017462));
#48390=CARTESIAN_POINT('Ctrl Pts',(22.0686865258567,4.20154261960756,-35.25032782635));
#48391=CARTESIAN_POINT('Ctrl Pts',(22.0706369822072,4.20079212635281,-35.6283477330854));
#48392=CARTESIAN_POINT('Ctrl Pts',(22.0722987978,4.20008504708062,-35.8822278341604));
#48393=CARTESIAN_POINT('Ctrl Pts',(22.0768288687233,4.19795632805282,-36.3884193841766));
#48394=CARTESIAN_POINT('Ctrl Pts',(22.0875114482299,4.19246069123774,-37.2723454492449));
#48395=CARTESIAN_POINT('Ctrl Pts',(22.1168195499966,4.17645376142218,-39.0309713117747));
#48396=CARTESIAN_POINT('Ctrl Pts',(22.1452208937072,4.15960897852894,-40.5324084559771));
#48397=CARTESIAN_POINT('Ctrl Pts',(22.160021497551,4.14994809813247,-41.7846755817295));
#48398=CARTESIAN_POINT('Ctrl Pts',(22.1640731974279,4.14408605348006,-42.1785184250812));
#48399=CARTESIAN_POINT('Ctrl Pts',(22.1689234073965,4.13301313193747,-42.688083469762));
#48400=CARTESIAN_POINT('Ctrl Pts',(22.1734502659695,4.12038747736818,-43.1970812016711));
#48401=CARTESIAN_POINT('Ctrl Pts',(22.1786439586059,4.10309924576169,-43.8258929583668));
#48402=CARTESIAN_POINT('Ctrl Pts',(22.184512600668,4.08404155036858,-44.5706823058272));
#48403=CARTESIAN_POINT('Ctrl Pts',(22.1894231114516,4.07286395725458,-45.1819851922531));
#48404=CARTESIAN_POINT('Ctrl Pts',(22.1936410112016,4.06864047791503,-45.665058999565));
#48405=CARTESIAN_POINT('Ctrl Pts',(22.1969596251638,4.06827562019768,-46.0244133809164));
#48406=CARTESIAN_POINT('Ctrl Pts',(22.2004867382473,4.07115636050592,-46.38071592816));
#48407=CARTESIAN_POINT('Ctrl Pts',(22.2055651893566,4.07990004759,-46.8516072133082));
#48408=CARTESIAN_POINT('Ctrl Pts',(22.2097599807653,4.09259101321018,-47.2000174156823));
#48409=CARTESIAN_POINT('Ctrl Pts',(22.2144340942165,4.11025304607408,-47.5464448219065));
#48410=CARTESIAN_POINT('Ctrl Pts',(22.2179845343943,4.1234000695629,-47.8012542930714));
#48411=CARTESIAN_POINT('Ctrl Pts',(22.2264508375367,4.14990942280532,-48.2941815322197));
#48412=CARTESIAN_POINT('Ctrl Pts',(22.2441171102791,4.2004838021227,-49.1547161665545));
#48413=CARTESIAN_POINT('Ctrl Pts',(22.2730861939326,4.29174641565724,-50.3543134049614));
#48414=CARTESIAN_POINT('Ctrl Pts',(22.3009319069203,4.45713611655791,-51.7546452965729));
#48415=CARTESIAN_POINT('Ctrl Pts',(22.3058715633566,4.62077825109781,-52.6609037956568));
#48416=CARTESIAN_POINT('Ctrl Pts',(22.3022024873703,4.74496293333649,-53.22130732141));
#48417=CARTESIAN_POINT('Ctrl Pts',(22.3000586188446,4.79829552597872,-53.4524280611144));
#48418=CARTESIAN_POINT('Ctrl Pts',(22.2931776516886,4.91313174392385,-53.91472992067));
#48419=CARTESIAN_POINT('Ctrl Pts',(22.27525507018,5.13638845677519,-54.7309787844978));
#48420=CARTESIAN_POINT('Ctrl Pts',(22.2225551369417,5.66344503276242,-56.3818257352234));
#48421=CARTESIAN_POINT('Ctrl Pts',(22.1709802552974,6.22850461206744,-57.8181758712166));
#48422=CARTESIAN_POINT('Ctrl Pts',(22.1514149325893,6.65724598612538,-58.8342802240781));
#48423=CARTESIAN_POINT('Ctrl Pts',(22.1489595264732,6.70600875414962,-58.9483090109368));
#48424=CARTESIAN_POINT('Ctrl Pts',(22.1442400202983,6.80879920661242,-59.1830571507315));
#48425=CARTESIAN_POINT('Ctrl Pts',(22.1363028643529,6.99498442952442,-59.5941165420173));
#48426=CARTESIAN_POINT('Ctrl Pts',(22.1217946990428,7.3956306795507,-60.4293377456673));
#48427=CARTESIAN_POINT('Ctrl Pts',(22.1082118821127,7.90372222660544,-61.4026487287963));
#48428=CARTESIAN_POINT('Ctrl Pts',(22.097131910433,8.43806063047352,-62.3895723906743));
#48429=CARTESIAN_POINT('Ctrl Pts',(22.091753128424,8.74353415108705,-62.9486874843298));
#48430=CARTESIAN_POINT('Ctrl Pts',(22.0885029341397,8.9472809575208,-63.3229122276346));
#48431=CARTESIAN_POINT('Ctrl Pts',(22.0864181423634,9.083002586351,-63.5727833041763));
#48432=CARTESIAN_POINT('Ctrl Pts',(22.0844775815037,9.21833703742369,-63.82317503393));
#48433=CARTESIAN_POINT('Ctrl Pts',(22.0828795252351,9.33609318052984,-64.0427690708459));
#48434=CARTESIAN_POINT('Ctrl Pts',(22.081997554122,9.40314135852388,-64.1683913455471));
#48435=CARTESIAN_POINT('Ctrl Pts',(22.0807043366672,9.50344054266713,-64.3569522702284));
#48436=CARTESIAN_POINT('Ctrl Pts',(22.079698989849,9.58642565845107,-64.5143969331008));
#48437=CARTESIAN_POINT('Ctrl Pts',(22.0781088241658,9.72258813692965,-64.7751907809016));
#48438=CARTESIAN_POINT('Ctrl Pts',(22.076697740684,9.85502070351906,-65.0282610850301));
#48439=CARTESIAN_POINT('Ctrl Pts',(22.0746378008923,10.1236397871968,-65.5395128310741));
#48440=CARTESIAN_POINT('Ctrl Pts',(22.0728859065854,10.5895145738863,-66.4212273936681));
#48441=CARTESIAN_POINT('Ctrl Pts',(22.0749234104754,11.5180077313772,-68.1632758098855));
#48442=CARTESIAN_POINT('Ctrl Pts',(22.0804594529303,12.3112391469442,-69.6409149901483));
#48443=CARTESIAN_POINT('Ctrl Pts',(22.0806257779101,12.9130724883053,-70.7727596451814));
#48444=CARTESIAN_POINT('Ctrl Pts',(22.0806527519314,13.0464178125152,-71.0235393205986));
#48445=CARTESIAN_POINT('Ctrl Pts',(22.0806944391854,13.3134515585615,-71.5257468364649));
#48446=CARTESIAN_POINT('Ctrl Pts',(22.0807296412911,13.6468658286295,-72.1527998158485));
#48447=CARTESIAN_POINT('Ctrl Pts',(22.0807366569763,14.0468732661696,-72.9051028689926));
#48448=CARTESIAN_POINT('Ctrl Pts',(22.0807103639373,14.8465315061039,-74.4090479193263));
#48449=CARTESIAN_POINT('Ctrl Pts',(22.0806660938293,15.5124783026127,-75.6615235028954));
#48450=CARTESIAN_POINT('Ctrl Pts',(22.0806849652143,16.4822164609512,-77.4853318752546));
#48451=CARTESIAN_POINT('Ctrl Pts',(22.0806947236768,16.9186987050899,-78.3062336020347));
#48452=CARTESIAN_POINT('Ctrl Pts',(22.0806947236768,17.3552202924793,-79.1272113041328));
#48453=CARTESIAN_POINT('Ctrl Pts',(23.9622955648791,4.08200208292847,24.8306372289488));
#48454=CARTESIAN_POINT('Ctrl Pts',(23.9623672448828,4.08200212320931,24.7817579944141));
#48455=CARTESIAN_POINT('Ctrl Pts',(23.9624424300683,4.08200216777709,24.7328798208572));
#48456=CARTESIAN_POINT('Ctrl Pts',(23.9633298985665,4.08200258379766,24.1822724635428));
#48457=CARTESIAN_POINT('Ctrl Pts',(23.9640073494789,4.08200366899808,23.1781369203715));
#48458=CARTESIAN_POINT('Ctrl Pts',(23.9655889010078,4.08200861120864,21.1695396264063));
#48459=CARTESIAN_POINT('Ctrl Pts',(23.9714912585163,4.08201016296143,19.6653829285451));
#48460=CARTESIAN_POINT('Ctrl Pts',(23.9840219927533,4.08200941516488,18.4143322408156));
#48461=CARTESIAN_POINT('Ctrl Pts',(23.9900323092972,4.08200976742032,17.9115202128027));
#48462=CARTESIAN_POINT('Ctrl Pts',(24.0051239731149,4.08201119176686,16.9075328742348));
#48463=CARTESIAN_POINT('Ctrl Pts',(24.037496132628,4.0820144081645,15.1537210085095));
#48464=CARTESIAN_POINT('Ctrl Pts',(24.068242343924,4.08200623174243,13.6519534556492));
#48465=CARTESIAN_POINT('Ctrl Pts',(24.0875228981722,4.08198831338579,12.3974529705996));
#48466=CARTESIAN_POINT('Ctrl Pts',(24.0954058032681,4.08197955514058,11.8964883932064));
#48467=CARTESIAN_POINT('Ctrl Pts',(24.1114809640743,4.08195780220778,10.8946300282762));
#48468=CARTESIAN_POINT('Ctrl Pts',(24.1313466678573,4.08191971253225,9.64208610714998));
#48469=CARTESIAN_POINT('Ctrl Pts',(24.1523116190628,4.08187527364994,8.1375880305666));
#48470=CARTESIAN_POINT('Ctrl Pts',(24.162661272085,4.08184505251405,7.13288645161328));
#48471=CARTESIAN_POINT('Ctrl Pts',(24.1674743487717,4.08183210280749,6.50490582828351));
#48472=CARTESIAN_POINT('Ctrl Pts',(24.1692799771994,4.0818096792317,6.25445557044036));
#48473=CARTESIAN_POINT('Ctrl Pts',(24.1724595365447,4.08170829787728,5.75310012246982));
#48474=CARTESIAN_POINT('Ctrl Pts',(24.1769118524244,4.08141173075345,4.87439057217338));
#48475=CARTESIAN_POINT('Ctrl Pts',(24.1816968570422,4.08064089883581,3.11432371976836));
#48476=CARTESIAN_POINT('Ctrl Pts',(24.1795300230087,4.08057722320863,1.60904293781249));
#48477=CARTESIAN_POINT('Ctrl Pts',(24.1759953565136,4.08176721012071,0.551230943523595));
#48478=CARTESIAN_POINT('Ctrl Pts',(24.1755386312866,4.08192464213912,0.425341023486164));
#48479=CARTESIAN_POINT('Ctrl Pts',(24.174466431991,4.08228588949836,0.173670854360428));
#48480=CARTESIAN_POINT('Ctrl Pts',(24.1722042923348,4.08303543284079,-0.266313863042626));
#48481=CARTESIAN_POINT('Ctrl Pts',(24.1679500685005,4.08438399185807,-0.893856249545121));
#48482=CARTESIAN_POINT('Ctrl Pts',(24.1616828022971,4.08630908814705,-1.64571238473509));
#48483=CARTESIAN_POINT('Ctrl Pts',(24.1521684529351,4.08906946798073,-2.6472116329457));
#48484=CARTESIAN_POINT('Ctrl Pts',(24.1392409619321,4.09252064208642,-3.89838880524634));
#48485=CARTESIAN_POINT('Ctrl Pts',(24.1296595937059,4.09456326651587,-4.90104830521301));
#48486=CARTESIAN_POINT('Ctrl Pts',(24.1245921150774,4.0953892226464,-5.52907006867696));
#48487=CARTESIAN_POINT('Ctrl Pts',(24.122543135074,4.09570581151499,-5.78005730609914));
#48488=CARTESIAN_POINT('Ctrl Pts',(24.1183711475979,4.09627961290835,-6.28254171768649));
#48489=CARTESIAN_POINT('Ctrl Pts',(24.110912934954,4.09713082267407,-7.162312337955));
#48490=CARTESIAN_POINT('Ctrl Pts',(24.1001218654103,4.09791704539196,-8.41971430174056));
#48491=CARTESIAN_POINT('Ctrl Pts',(24.0900005940753,4.09816054654107,-9.67499262570322));
#48492=CARTESIAN_POINT('Ctrl Pts',(24.0837261929461,4.09806168192696,-10.551155153125));
#48493=CARTESIAN_POINT('Ctrl Pts',(24.0804251175495,4.09793095582491,-11.0508803093238));
#48494=CARTESIAN_POINT('Ctrl Pts',(24.0788794798348,4.09784105346742,-11.3003946775157));
#48495=CARTESIAN_POINT('Ctrl Pts',(24.0777594081461,4.09776436119308,-11.4881778539406));
#48496=CARTESIAN_POINT('Ctrl Pts',(24.0770066256652,4.09770108469074,-11.6145632672188));
#48497=CARTESIAN_POINT('Ctrl Pts',(24.075502944022,4.09753197255658,-11.8668916405279));
#48498=CARTESIAN_POINT('Ctrl Pts',(24.072882864956,4.09713203653876,-12.3077631563438));
#48499=CARTESIAN_POINT('Ctrl Pts',(24.0677487709978,4.09597723281603,-13.1867776263164));
#48500=CARTESIAN_POINT('Ctrl Pts',(24.0611063576802,4.09369426111681,-14.4370753980823));
#48501=CARTESIAN_POINT('Ctrl Pts',(24.0568300528932,4.0917465099413,-15.5611346823936));
#48502=CARTESIAN_POINT('Ctrl Pts',(24.055047903523,4.09084877125918,-16.312237806251));
#48503=CARTESIAN_POINT('Ctrl Pts',(24.0541711416194,4.09038135679613,-16.8135860569128));
#48504=CARTESIAN_POINT('Ctrl Pts',(24.0538868311995,4.09020069604123,-17.1904517707465));
#48505=CARTESIAN_POINT('Ctrl Pts',(24.0538902418915,4.09017721932461,-17.504417356177));
#48506=CARTESIAN_POINT('Ctrl Pts',(24.0539261147657,4.09015693885285,-17.6294314542331));
#48507=CARTESIAN_POINT('Ctrl Pts',(24.0541305633638,4.09007310391961,-17.8790800058834));
#48508=CARTESIAN_POINT('Ctrl Pts',(24.0545220869184,4.08993459007116,-18.1289017837817));
#48509=CARTESIAN_POINT('Ctrl Pts',(24.055079936961,4.08976038112565,-18.3786753221093));
#48510=CARTESIAN_POINT('Ctrl Pts',(24.0554929637826,4.08964046612317,-18.534814836201));
#48511=CARTESIAN_POINT('Ctrl Pts',(24.0558594922731,4.08954025765299,-18.6597282953941));
#48512=CARTESIAN_POINT('Ctrl Pts',(24.0561516636267,4.08946354742096,-18.7534195243898));
#48513=CARTESIAN_POINT('Ctrl Pts',(24.0564089854875,4.08939881893064,-18.8314986568552));
#48514=CARTESIAN_POINT('Ctrl Pts',(24.0566228183052,4.08934683325637,-18.8939645198468));
#48515=CARTESIAN_POINT('Ctrl Pts',(24.0584852768486,4.08890451612297,-19.4249374335339));
#48516=CARTESIAN_POINT('Ctrl Pts',(24.0633643670787,4.08809475111636,-20.4404636917259));
#48517=CARTESIAN_POINT('Ctrl Pts',(24.0717452079226,4.08931496172151,-21.9421262926985));
#48518=CARTESIAN_POINT('Ctrl Pts',(24.0761460116141,4.09339376732741,-22.9448491109531));
#48519=CARTESIAN_POINT('Ctrl Pts',(24.0779762230367,4.0974562092785,-23.5703671053928));
#48520=CARTESIAN_POINT('Ctrl Pts',(24.0786796961305,4.09927817321484,-23.8170761770731));
#48521=CARTESIAN_POINT('Ctrl Pts',(24.0799760497679,4.10373186863751,-24.3124706455005));
#48522=CARTESIAN_POINT('Ctrl Pts',(24.0819970407477,4.11337074967939,-25.1824729583923));
#48523=CARTESIAN_POINT('Ctrl Pts',(24.0842021198426,4.1308454136294,-26.4339700730892));
#48524=CARTESIAN_POINT('Ctrl Pts',(24.0864078697437,4.15263365321005,-27.9450038672982));
#48525=CARTESIAN_POINT('Ctrl Pts',(24.0877812226619,4.16412692188707,-28.9562923588698));
#48526=CARTESIAN_POINT('Ctrl Pts',(24.0886514726177,4.1687482944764,-29.5253334387894));
#48527=CARTESIAN_POINT('Ctrl Pts',(24.0888326397504,4.16975911269941,-29.6506348041106));
#48528=CARTESIAN_POINT('Ctrl Pts',(24.0891409486858,4.17175142993273,-29.9019716591638));
#48529=CARTESIAN_POINT('Ctrl Pts',(24.0895498987179,4.17513461975883,-30.3417198488222));
#48530=CARTESIAN_POINT('Ctrl Pts',(24.0899602386112,4.18145381343337,-31.2221966398746));
#48531=CARTESIAN_POINT('Ctrl Pts',(24.0900269745172,4.18884650516548,-32.4813785165483));
#48532=CARTESIAN_POINT('Ctrl Pts',(24.0910174225162,4.19322095175136,-33.7405815354532));
#48533=CARTESIAN_POINT('Ctrl Pts',(24.0933253133805,4.19441944678141,-34.7466124020879));
#48534=CARTESIAN_POINT('Ctrl Pts',(24.0951479965203,4.19414850076315,-35.2491273596588));
#48535=CARTESIAN_POINT('Ctrl Pts',(24.0968191041055,4.1935978845164,-35.6266887560775));
#48536=CARTESIAN_POINT('Ctrl Pts',(24.0981285479769,4.19306099669884,-35.8801114343427));
#48537=CARTESIAN_POINT('Ctrl Pts',(24.1014087904296,4.19138300845976,-36.3856118091494));
#48538=CARTESIAN_POINT('Ctrl Pts',(24.1087164830883,4.18698244390804,-37.2685998966351));
#48539=CARTESIAN_POINT('Ctrl Pts',(24.1269844698749,4.17360041191136,-39.026696961175));
#48540=CARTESIAN_POINT('Ctrl Pts',(24.1415905609808,4.15823646272699,-40.530354778854));
#48541=CARTESIAN_POINT('Ctrl Pts',(24.143961339622,4.14796103186066,-41.7852242144327));
#48542=CARTESIAN_POINT('Ctrl Pts',(24.1443439544137,4.14179468730075,-42.1797011452874));
#48543=CARTESIAN_POINT('Ctrl Pts',(24.1442498711312,4.13010473975566,-42.6899536899554));
#48544=CARTESIAN_POINT('Ctrl Pts',(24.14378449886,4.11677123523734,-43.1995233294011));
#48545=CARTESIAN_POINT('Ctrl Pts',(24.1424974647182,4.09844750714945,-43.8288475600246));
#48546=CARTESIAN_POINT('Ctrl Pts',(24.139866251443,4.07803004113037,-44.5739413341453));
#48547=CARTESIAN_POINT('Ctrl Pts',(24.1367976109779,4.06571129506959,-45.18525201338));
#48548=CARTESIAN_POINT('Ctrl Pts',(24.133772595606,4.06058762318336,-45.6681760139594));
#48549=CARTESIAN_POINT('Ctrl Pts',(24.1312507499958,4.05958009324959,-46.0273487349289));
#48550=CARTESIAN_POINT('Ctrl Pts',(24.1284755233732,4.06185881345286,-46.38339949684));
#48551=CARTESIAN_POINT('Ctrl Pts',(24.1244252548433,4.06986374479445,-46.8538654027403));
#48552=CARTESIAN_POINT('Ctrl Pts',(24.1210589308145,4.08210270223804,-47.2018603071012));
#48553=CARTESIAN_POINT('Ctrl Pts',(24.1174132533512,4.0993842933789,-47.5478343049022));
#48554=CARTESIAN_POINT('Ctrl Pts',(24.1148393446767,4.11220700729379,-47.8032316024947));
#48555=CARTESIAN_POINT('Ctrl Pts',(24.1091958067937,4.13796629168275,-48.2966296675904));
#48556=CARTESIAN_POINT('Ctrl Pts',(24.0981441517371,4.1871107392127,-49.1577797770064));
#48557=CARTESIAN_POINT('Ctrl Pts',(24.0796951632445,4.27687296827978,-50.3567072681302));
#48558=CARTESIAN_POINT('Ctrl Pts',(24.0548574625172,4.44322788604528,-51.7533392942329));
#48559=CARTESIAN_POINT('Ctrl Pts',(24.0376307905872,4.60874279082569,-52.6550105143473));
#48560=CARTESIAN_POINT('Ctrl Pts',(24.0269167212642,4.73426592858213,-53.212210232132));
#48561=CARTESIAN_POINT('Ctrl Pts',(24.022261688763,4.78802914663047,-53.4409847524117));
#48562=CARTESIAN_POINT('Ctrl Pts',(24.011937980585,4.90444432727691,-53.899996095257));
#48563=CARTESIAN_POINT('Ctrl Pts',(23.9917197269347,5.13175954459855,-54.7119534677432));
#48564=CARTESIAN_POINT('Ctrl Pts',(23.946881494816,5.67152647254202,-56.3614849702221));
#48565=CARTESIAN_POINT('Ctrl Pts',(23.9149861796843,6.25065906002568,-57.8060061410901));
#48566=CARTESIAN_POINT('Ctrl Pts',(23.9082889999673,6.68463357757772,-58.8311245098676));
#48567=CARTESIAN_POINT('Ctrl Pts',(23.9077683667265,6.73386259900167,-58.9460129438745));
#48568=CARTESIAN_POINT('Ctrl Pts',(23.9070918607004,6.83745355958267,-59.1824653739889));
#48569=CARTESIAN_POINT('Ctrl Pts',(23.9070829160766,7.02450015525985,-59.5961205690869));
#48570=CARTESIAN_POINT('Ctrl Pts',(23.9109487883727,7.42501547924234,-60.4353539082253));
#48571=CARTESIAN_POINT('Ctrl Pts',(23.9216909852029,7.92938628651344,-61.4108375088605));
#48572=CARTESIAN_POINT('Ctrl Pts',(23.9340640848195,8.45818729151285,-62.3980996785296));
#48573=CARTESIAN_POINT('Ctrl Pts',(23.9408211940191,8.76022657679104,-62.9567360326512));
#48574=CARTESIAN_POINT('Ctrl Pts',(23.9448860238444,8.96170365245728,-63.3303615884543));
#48575=CARTESIAN_POINT('Ctrl Pts',(23.9474573707423,9.09592765324216,-63.5797569212499));
#48576=CARTESIAN_POINT('Ctrl Pts',(23.9497770282467,9.22980515457034,-63.8295558129152));
#48577=CARTESIAN_POINT('Ctrl Pts',(23.9515308576229,9.34634785666618,-64.0485240946921));
#48578=CARTESIAN_POINT('Ctrl Pts',(23.9524438717482,9.41272428541754,-64.1737568833352));
#48579=CARTESIAN_POINT('Ctrl Pts',(23.9537200122451,9.51203994843218,-64.361702149246));
#48580=CARTESIAN_POINT('Ctrl Pts',(23.9545752284772,9.59425793624058,-64.5185625171711));
#48581=CARTESIAN_POINT('Ctrl Pts',(23.9556701773485,9.72925393134929,-64.7783107806095));
#48582=CARTESIAN_POINT('Ctrl Pts',(23.9567284557211,9.86106264889938,-65.0312747707878));
#48583=CARTESIAN_POINT('Ctrl Pts',(23.9584683822691,10.1283193737384,-65.5418186150697));
#48584=CARTESIAN_POINT('Ctrl Pts',(23.9606501935929,10.5924204836096,-66.4227026698923));
#48585=CARTESIAN_POINT('Ctrl Pts',(23.9623055482788,11.5187962468744,-68.1634283976708));
#48586=CARTESIAN_POINT('Ctrl Pts',(23.9614773124919,12.3120252077534,-69.641062233731));
#48587=CARTESIAN_POINT('Ctrl Pts',(23.9621246704273,12.9136059543534,-70.773334928149));
#48588=CARTESIAN_POINT('Ctrl Pts',(23.9622527599848,13.0467770048231,-71.0239630352363));
#48589=CARTESIAN_POINT('Ctrl Pts',(23.9624420290191,13.3135967940574,-71.5260295392633));
#48590=CARTESIAN_POINT('Ctrl Pts',(23.9625647757318,13.6468141449215,-72.1528836114454));
#48591=CARTESIAN_POINT('Ctrl Pts',(23.9625770445063,14.0467309375321,-72.9050342749593));
#48592=CARTESIAN_POINT('Ctrl Pts',(23.962409408479,14.8463966744232,-74.4087646262313));
#48593=CARTESIAN_POINT('Ctrl Pts',(23.9620320808063,15.512652456629,-75.6613100284921));
#48594=CARTESIAN_POINT('Ctrl Pts',(23.9620255452841,16.4825593234147,-77.4854317343623));
#48595=CARTESIAN_POINT('Ctrl Pts',(23.9620221622173,16.9189893457455,-78.3062332078354));
#48596=CARTESIAN_POINT('Ctrl Pts',(23.9620221622173,17.355510933135,-79.1272109099336));
#48597=CARTESIAN_POINT('Ctrl Pts',(25.844570784284,4.08057977943501,24.8306353590067));
#48598=CARTESIAN_POINT('Ctrl Pts',(25.844648185704,4.08057966651517,24.7817560666017));
#48599=CARTESIAN_POINT('Ctrl Pts',(25.8447293650715,4.08057954730243,24.7328778289554));
#48600=CARTESIAN_POINT('Ctrl Pts',(25.8456878994455,4.08057817374023,24.1822699652252));
#48601=CARTESIAN_POINT('Ctrl Pts',(25.8464233826524,4.08057784177856,23.1781352323388));
#48602=CARTESIAN_POINT('Ctrl Pts',(25.8481374319039,4.08057692917578,21.1695367649276));
#48603=CARTESIAN_POINT('Ctrl Pts',(25.8545155933218,4.08056815801389,19.6653829487358));
#48604=CARTESIAN_POINT('Ctrl Pts',(25.8680382452856,4.08054600320532,18.4143333506094));
#48605=CARTESIAN_POINT('Ctrl Pts',(25.8745244558723,4.0805353149668,17.9115175621618));
#48606=CARTESIAN_POINT('Ctrl Pts',(25.8908129421233,4.0805085448771,16.907528530086));
#48607=CARTESIAN_POINT('Ctrl Pts',(25.925750354669,4.08045059698757,15.1537187688109));
#48608=CARTESIAN_POINT('Ctrl Pts',(25.9589300071752,4.08039564964573,13.6519725049998));
#48609=CARTESIAN_POINT('Ctrl Pts',(25.9797127722873,4.08035898548116,12.3974923061763));
#48610=CARTESIAN_POINT('Ctrl Pts',(25.9882070772645,4.08034368966931,11.8965356241494));
#48611=CARTESIAN_POINT('Ctrl Pts',(26.005518572936,4.08031121874985,10.8946878428175));
#48612=CARTESIAN_POINT('Ctrl Pts',(26.0269097431622,4.08027143363959,9.64215699732804));
#48613=CARTESIAN_POINT('Ctrl Pts',(26.0494661062327,4.08022743379009,8.13766358558484));
#48614=CARTESIAN_POINT('Ctrl Pts',(26.0606095379075,4.08020777316334,7.13296163855839));
#48615=CARTESIAN_POINT('Ctrl Pts',(26.0657868554483,4.08019818971332,6.50498953783284));
#48616=CARTESIAN_POINT('Ctrl Pts',(26.0677293368991,4.08019860392813,6.254821542523));
#48617=CARTESIAN_POINT('Ctrl Pts',(26.0711518004003,4.08021363683779,5.75377060631554));
#48618=CARTESIAN_POINT('Ctrl Pts',(26.0759579026102,4.08027080938024,4.87544910775995));
#48619=CARTESIAN_POINT('Ctrl Pts',(26.081128793862,4.08043695841909,3.11515403116237));
#48620=CARTESIAN_POINT('Ctrl Pts',(26.0788518154024,4.08045581336314,1.60815971006337));
#48621=CARTESIAN_POINT('Ctrl Pts',(26.0749837526961,4.08017495077629,0.548307353526776));
#48622=CARTESIAN_POINT('Ctrl Pts',(26.0744793339419,4.08013714720592,0.422056861710988));
#48623=CARTESIAN_POINT('Ctrl Pts',(26.0732989455254,4.08005053177588,0.169779472383307));
#48624=CARTESIAN_POINT('Ctrl Pts',(26.0708087506696,4.07987008450307,-0.271193576271456));
#48625=CARTESIAN_POINT('Ctrl Pts',(26.0661614568501,4.07954941719884,-0.899809220006871));
#48626=CARTESIAN_POINT('Ctrl Pts',(26.0592820344404,4.07909382231187,-1.65246885411488));
#48627=CARTESIAN_POINT('Ctrl Pts',(26.0488932000221,4.07846206268153,-2.65438880624532));
#48628=CARTESIAN_POINT('Ctrl Pts',(26.0346923351045,4.07769375101536,-3.9048842466606));
#48629=CARTESIAN_POINT('Ctrl Pts',(26.024217932681,4.07729272551322,-4.90564261911502));
#48630=CARTESIAN_POINT('Ctrl Pts',(26.0186988348058,4.07714577043534,-5.53205833177433));
#48631=CARTESIAN_POINT('Ctrl Pts',(26.0164949451559,4.07709446937418,-5.78287146791138));
#48632=CARTESIAN_POINT('Ctrl Pts',(26.0120848108843,4.07702655552691,-6.28477858997372));
#48633=CARTESIAN_POINT('Ctrl Pts',(26.0043862149626,4.0769874486626,-7.16375641765298));
#48634=CARTESIAN_POINT('Ctrl Pts',(25.9935479321394,4.07709939533413,-8.4201770232055));
#48635=CARTESIAN_POINT('Ctrl Pts',(25.9832001785983,4.07725903384453,-9.67481503127917));
#48636=CARTESIAN_POINT('Ctrl Pts',(25.9763642186198,4.07730127796632,-10.5506640151661));
#48637=CARTESIAN_POINT('Ctrl Pts',(25.9725930924616,4.07729366717744,-11.050257032386));
#48638=CARTESIAN_POINT('Ctrl Pts',(25.9707563537227,4.07727728154854,-11.2997214865617));
#48639=CARTESIAN_POINT('Ctrl Pts',(25.9693926551822,4.07725920620956,-11.4874662439065));
#48640=CARTESIAN_POINT('Ctrl Pts',(25.9684619723602,4.07724603910095,-11.6135983416455));
#48641=CARTESIAN_POINT('Ctrl Pts',(25.9665527693782,4.07721311695757,-11.8655778154556));
#48642=CARTESIAN_POINT('Ctrl Pts',(25.9631025382659,4.07714069706844,-12.3058419391744));
#48643=CARTESIAN_POINT('Ctrl Pts',(25.9559122008311,4.07694519975544,-13.1839670337358));
#48644=CARTESIAN_POINT('Ctrl Pts',(25.9456061675272,4.07655137577511,-14.4337708179989));
#48645=CARTESIAN_POINT('Ctrl Pts',(25.9382627210243,4.07618719946379,-15.5583998491895));
#48646=CARTESIAN_POINT('Ctrl Pts',(25.9349787321692,4.07603124892372,-16.3103112660927));
#48647=CARTESIAN_POINT('Ctrl Pts',(25.9332708395799,4.07595705010926,-16.8123083898932));
#48648=CARTESIAN_POINT('Ctrl Pts',(25.9326014082205,4.07593777072971,-17.1897929762814));
#48649=CARTESIAN_POINT('Ctrl Pts',(25.9324422746817,4.07595254629577,-17.5043122449826));
#48650=CARTESIAN_POINT('Ctrl Pts',(25.9323909876488,4.0759529390079,-17.6290107968246));
#48651=CARTESIAN_POINT('Ctrl Pts',(25.9323335197263,4.07595072339627,-17.8784039971533));
#48652=CARTESIAN_POINT('Ctrl Pts',(25.9323539449517,4.0759394659283,-18.1279353152333));
#48653=CARTESIAN_POINT('Ctrl Pts',(25.9324598599516,4.07592737655612,-18.377562269577));
#48654=CARTESIAN_POINT('Ctrl Pts',(25.9325656989019,4.07591881813072,-18.5336303782332));
#48655=CARTESIAN_POINT('Ctrl Pts',(25.9326749957718,4.07591254453843,-18.6585121522346));
#48656=CARTESIAN_POINT('Ctrl Pts',(25.9327699231852,4.07590797996094,-18.7521884498438));
#48657=CARTESIAN_POINT('Ctrl Pts',(25.9328601637811,4.07590438461883,-18.8302641974303));
#48658=CARTESIAN_POINT('Ctrl Pts',(25.9329390907671,4.07590182294606,-18.8927321535059));
#48659=CARTESIAN_POINT('Ctrl Pts',(25.9336501455939,4.07588108238224,-19.4237516127014));
#48660=CARTESIAN_POINT('Ctrl Pts',(25.9363009371823,4.07583341441431,-20.4403475109291));
#48661=CARTESIAN_POINT('Ctrl Pts',(25.9453630178633,4.07641698035684,-21.9459502231633));
#48662=CARTESIAN_POINT('Ctrl Pts',(25.9558794513379,4.07731497584596,-22.9529656912019));
#48663=CARTESIAN_POINT('Ctrl Pts',(25.9642086520499,4.07805728208967,-23.5817432715613));
#48664=CARTESIAN_POINT('Ctrl Pts',(25.9678540602757,4.07839867495163,-23.8304233353386));
#48665=CARTESIAN_POINT('Ctrl Pts',(25.9764013443531,4.07915865200955,-24.3288588433319));
#48666=CARTESIAN_POINT('Ctrl Pts',(25.9942301597475,4.0806592216352,-25.2032646909985));
#48667=CARTESIAN_POINT('Ctrl Pts',(26.025221328115,4.082732631673,-26.4576901759554));
#48668=CARTESIAN_POINT('Ctrl Pts',(26.0630445990899,4.08449353718692,-27.967094636833));
#48669=CARTESIAN_POINT('Ctrl Pts',(26.0829726200033,4.08489425524181,-28.9734406960325));
#48670=CARTESIAN_POINT('Ctrl Pts',(26.0913002227101,4.08499781220332,-29.5386707502503));
#48671=CARTESIAN_POINT('Ctrl Pts',(26.0931251317467,4.08502743350306,-29.6641131002139));
#48672=CARTESIAN_POINT('Ctrl Pts',(26.0966334094344,4.08507488495586,-29.9151404576258));
#48673=CARTESIAN_POINT('Ctrl Pts',(26.1024148737267,4.08512341588005,-30.3545438582529));
#48674=CARTESIAN_POINT('Ctrl Pts',(26.1126395490258,4.08512931616553,-31.233781402742));
#48675=CARTESIAN_POINT('Ctrl Pts',(26.1238689000862,4.08484171664707,-32.4903335546092));
#48676=CARTESIAN_POINT('Ctrl Pts',(26.1318887243776,4.08432971989877,-33.7454848406989));
#48677=CARTESIAN_POINT('Ctrl Pts',(26.1372094940222,4.08391397588549,-34.7474837791314));
#48678=CARTESIAN_POINT('Ctrl Pts',(26.1396084872277,4.08363675797948,-35.247707527111));
#48679=CARTESIAN_POINT('Ctrl Pts',(26.141371220675,4.08344203936742,-35.623440510749));
#48680=CARTESIAN_POINT('Ctrl Pts',(26.1426337835212,4.08327341585163,-35.8753722067299));
#48681=CARTESIAN_POINT('Ctrl Pts',(26.1453549329869,4.08282791481109,-36.3783044765536));
#48682=CARTESIAN_POINT('Ctrl Pts',(26.1503980487191,4.08171475754224,-37.257313806696));
#48683=CARTESIAN_POINT('Ctrl Pts',(26.1593188077099,4.07897427874934,-39.01007237833));
#48684=CARTESIAN_POINT('Ctrl Pts',(26.1581117957454,4.07706675221868,-40.5130850563031));
#48685=CARTESIAN_POINT('Ctrl Pts',(26.1442318739232,4.07761140540693,-41.7694461876314));
#48686=CARTESIAN_POINT('Ctrl Pts',(26.1397782129226,4.07464958837052,-42.1647424202513));
#48687=CARTESIAN_POINT('Ctrl Pts',(26.1330493969374,4.06699950959388,-42.6753154763828));
#48688=CARTESIAN_POINT('Ctrl Pts',(26.1257350602188,4.05768397496789,-43.1849413640208));
#48689=CARTESIAN_POINT('Ctrl Pts',(26.115365164687,4.04442739625451,-43.8136832824334));
#48690=CARTESIAN_POINT('Ctrl Pts',(26.1005460918204,4.03055517689925,-44.5570878496065));
#48691=CARTESIAN_POINT('Ctrl Pts',(26.0858584399693,4.02434764341965,-45.1661285977057));
#48692=CARTESIAN_POINT('Ctrl Pts',(26.0724650863366,4.02463040301721,-45.646760157016));
#48693=CARTESIAN_POINT('Ctrl Pts',(26.0615494470953,4.02797252451459,-46.003952285481));
#48694=CARTESIAN_POINT('Ctrl Pts',(26.0497046656066,4.03492112593504,-46.3577693998032));
#48695=CARTESIAN_POINT('Ctrl Pts',(26.0325958430163,4.04959367855714,-46.8249245878478));
#48696=CARTESIAN_POINT('Ctrl Pts',(26.0182065832668,4.06739629210528,-47.1700518562479));
#48697=CARTESIAN_POINT('Ctrl Pts',(26.0026297402098,4.09061053940423,-47.5128689033931));
#48698=CARTESIAN_POINT('Ctrl Pts',(25.9912336674935,4.10813287081449,-47.7635943609639));
#48699=CARTESIAN_POINT('Ctrl Pts',(25.9649865045349,4.14438276814989,-48.2503889637481));
#48700=CARTESIAN_POINT('Ctrl Pts',(25.9113335131762,4.214496021023,-49.1021605184574));
#48701=CARTESIAN_POINT('Ctrl Pts',(25.8199243549994,4.33678677328201,-50.2966447803426));
#48702=CARTESIAN_POINT('Ctrl Pts',(25.7129189353006,4.53530999157483,-51.7027703341965));
#48703=CARTESIAN_POINT('Ctrl Pts',(25.6623982059248,4.71624948069983,-52.621419873122));
#48704=CARTESIAN_POINT('Ctrl Pts',(25.6428686247225,4.84960861203734,-53.1915163476384));
#48705=CARTESIAN_POINT('Ctrl Pts',(25.6354037440851,4.90561734273628,-53.4216810401192));
#48706=CARTESIAN_POINT('Ctrl Pts',(25.622450587021,5.02663649475412,-53.8855341814151));
#48707=CARTESIAN_POINT('Ctrl Pts',(25.6045455906359,5.26086402238474,-54.7045799538225));
#48708=CARTESIAN_POINT('Ctrl Pts',(25.5859152122443,5.8106038398779,-56.3677207273517));
#48709=CARTESIAN_POINT('Ctrl Pts',(25.5936609389522,6.38981330126379,-57.8204867428421));
#48710=CARTESIAN_POINT('Ctrl Pts',(25.6082771767271,6.81852440848565,-58.8514652972658));
#48711=CARTESIAN_POINT('Ctrl Pts',(25.6108235337001,6.86784699759766,-58.9686583326326));
#48712=CARTESIAN_POINT('Ctrl Pts',(25.6164812962558,6.97062005327531,-59.2083923499976));
#48713=CARTESIAN_POINT('Ctrl Pts',(25.628647620426,7.15515134191995,-59.627341287499));
#48714=CARTESIAN_POINT('Ctrl Pts',(25.6599824454046,7.54546138682434,-60.4734127225068));
#48715=CARTESIAN_POINT('Ctrl Pts',(25.7063620960752,8.02861820652914,-61.4508681824153));
#48716=CARTESIAN_POINT('Ctrl Pts',(25.7526341951128,8.53156286551664,-62.435681976523));
#48717=CARTESIAN_POINT('Ctrl Pts',(25.7767943793768,8.81850578713554,-62.9913328103881));
#48718=CARTESIAN_POINT('Ctrl Pts',(25.7913328807926,9.01016007811373,-63.3622459744139));
#48719=CARTESIAN_POINT('Ctrl Pts',(25.8005534938435,9.13793802959155,-63.6096298946428));
#48720=CARTESIAN_POINT('Ctrl Pts',(25.8089946376101,9.26556868353528,-63.8571080587124));
#48721=CARTESIAN_POINT('Ctrl Pts',(25.8155491309342,9.37691360542288,-64.0737428963701));
#48722=CARTESIAN_POINT('Ctrl Pts',(25.8190373561112,9.44040887490913,-64.1975514715952));
#48723=CARTESIAN_POINT('Ctrl Pts',(25.8240016713012,9.53549980173153,-64.383268720066));
#48724=CARTESIAN_POINT('Ctrl Pts',(25.8275621499168,9.61440570071669,-64.538068934009));
#48725=CARTESIAN_POINT('Ctrl Pts',(25.8325698248521,9.74429868510807,-64.7941471789633));
#48726=CARTESIAN_POINT('Ctrl Pts',(25.8372188246519,9.87232665433277,-65.0452157696068));
#48727=CARTESIAN_POINT('Ctrl Pts',(25.8444371392966,10.1327681425613,-65.5513457195204));
#48728=CARTESIAN_POINT('Ctrl Pts',(25.8522523448846,10.5886367494958,-66.4260858166688));
#48729=CARTESIAN_POINT('Ctrl Pts',(25.8529704258499,11.5096169214689,-68.1585107930789));
#48730=CARTESIAN_POINT('Ctrl Pts',(25.8427466506853,12.3095608914108,-69.6375099740252));
#48731=CARTESIAN_POINT('Ctrl Pts',(25.84405505498,12.9128106186317,-70.7746794958561));
#48732=CARTESIAN_POINT('Ctrl Pts',(25.844306964925,13.0455079725974,-71.024753629924));
#48733=CARTESIAN_POINT('Ctrl Pts',(25.8446814868113,13.3119932674773,-71.5266931920502));
#48734=CARTESIAN_POINT('Ctrl Pts',(25.8449316978369,13.6447800575678,-72.153072250218));
#48735=CARTESIAN_POINT('Ctrl Pts',(25.8449597858347,14.0445382927846,-72.9049624655928));
#48736=CARTESIAN_POINT('Ctrl Pts',(25.844637678253,14.8441994652986,-74.4082520428641));
#48737=CARTESIAN_POINT('Ctrl Pts',(25.8439279150842,15.511032583249,-75.6609274498486));
#48738=CARTESIAN_POINT('Ctrl Pts',(25.8439346315324,16.4812454805264,-77.4856308339518));
#48739=CARTESIAN_POINT('Ctrl Pts',(25.8439377293388,16.9175685704731,-78.306234354275));
#48740=CARTESIAN_POINT('Ctrl Pts',(25.843937729339,17.3540901578626,-79.1272120563734));
#48741=CARTESIAN_POINT('Ctrl Pts',(27.7252597652467,4.07604430203363,24.830629906652));
#48742=CARTESIAN_POINT('Ctrl Pts',(27.725342633422,4.07604398489538,24.7817504395661));
#48743=CARTESIAN_POINT('Ctrl Pts',(27.7254295486928,4.07604365338282,24.7328720248872));
#48744=CARTESIAN_POINT('Ctrl Pts',(27.7264557041567,4.07603969724442,24.1822620861588));
#48745=CARTESIAN_POINT('Ctrl Pts',(27.7272430738068,4.07603395588985,23.1781243249467));
#48746=CARTESIAN_POINT('Ctrl Pts',(27.7290798647343,4.07601957377584,21.1695223025744));
#48747=CARTESIAN_POINT('Ctrl Pts',(27.7359069292677,4.07599287934245,19.6653679592558));
#48748=CARTESIAN_POINT('Ctrl Pts',(27.7503810766268,4.07594970932461,18.4143185095723));
#48749=CARTESIAN_POINT('Ctrl Pts',(27.757323963104,4.07592802362061,17.9114919920945));
#48750=CARTESIAN_POINT('Ctrl Pts',(27.7747592655169,4.07587160380069,16.9074951083392));
#48751=CARTESIAN_POINT('Ctrl Pts',(27.8121566969761,4.07575137527824,15.1536852342599));
#48752=CARTESIAN_POINT('Ctrl Pts',(27.8476686036972,4.07565137525816,13.6519715739283));
#48753=CARTESIAN_POINT('Ctrl Pts',(27.8699096323763,4.07561802498269,12.3975366392587));
#48754=CARTESIAN_POINT('Ctrl Pts',(27.8789999249988,4.07560775093695,11.8965984778399));
#48755=CARTESIAN_POINT('Ctrl Pts',(27.8975261319994,4.07559790364118,10.8947777778399));
#48756=CARTESIAN_POINT('Ctrl Pts',(27.92041464346,4.07559964500799,9.64226446740739));
#48757=CARTESIAN_POINT('Ctrl Pts',(27.9445489060284,4.07561795275291,8.13776813910616));
#48758=CARTESIAN_POINT('Ctrl Pts',(27.956465467892,4.07563038589341,7.13304469504194));
#48759=CARTESIAN_POINT('Ctrl Pts',(27.9620013880069,4.07563792059547,6.50505993209809));
#48760=CARTESIAN_POINT('Ctrl Pts',(27.9640898945436,4.07565339079377,6.2549958595789));
#48761=CARTESIAN_POINT('Ctrl Pts',(27.9678091802326,4.07572482436653,5.75405417771761));
#48762=CARTESIAN_POINT('Ctrl Pts',(27.9731241294107,4.07592958460531,4.8758699093757));
#48763=CARTESIAN_POINT('Ctrl Pts',(27.9791216548069,4.07647638005503,3.11547842572566));
#48764=CARTESIAN_POINT('Ctrl Pts',(27.9766408448158,4.07649656028921,1.60780894281924));
#48765=CARTESIAN_POINT('Ctrl Pts',(27.9716927842217,4.07569812473195,0.547187709820962));
#48766=CARTESIAN_POINT('Ctrl Pts',(27.9710490981585,4.0755954385535,0.420807592805693));
#48767=CARTESIAN_POINT('Ctrl Pts',(27.969544237905,4.07535654929588,0.168308988144524));
#48768=CARTESIAN_POINT('Ctrl Pts',(27.9663754136284,4.07485760897021,-0.273024725269034));
#48769=CARTESIAN_POINT('Ctrl Pts',(27.9604721629123,4.07394173010837,-0.902038225881202));
#48770=CARTESIAN_POINT('Ctrl Pts',(27.951789048622,4.07262501270999,-1.65498593663574));
#48771=CARTESIAN_POINT('Ctrl Pts',(27.9387566627383,4.07070977393899,-2.65703120096997));
#48772=CARTESIAN_POINT('Ctrl Pts',(27.9212160850017,4.06827102583396,-3.90721016180692));
#48773=CARTESIAN_POINT('Ctrl Pts',(27.9087198935433,4.06683898836998,-4.90728724033103));
#48774=CARTESIAN_POINT('Ctrl Pts',(27.9023452962071,4.06627680295807,-5.53318228176463));
#48775=CARTESIAN_POINT('Ctrl Pts',(27.8998132638848,4.06605006258839,-5.78420215251212));
#48776=CARTESIAN_POINT('Ctrl Pts',(27.8948169833875,4.06559904063942,-6.28620637550023));
#48777=CARTESIAN_POINT('Ctrl Pts',(27.8862467391115,4.06484014153083,-7.16528954655609));
#48778=CARTESIAN_POINT('Ctrl Pts',(27.8745228455075,4.06397616282331,-8.42123471706821));
#48779=CARTESIAN_POINT('Ctrl Pts',(27.8635486779871,4.06376894206732,-9.67470205018876));
#48780=CARTESIAN_POINT('Ctrl Pts',(27.8562974748696,4.06415849215986,-10.5493253285242));
#48781=CARTESIAN_POINT('Ctrl Pts',(27.8522752578299,4.06456154596584,-11.0481047440172));
#48782=CARTESIAN_POINT('Ctrl Pts',(27.8503056619078,4.06482741062643,-11.2971266153811));
#48783=CARTESIAN_POINT('Ctrl Pts',(27.8488380948691,4.06505369206006,-11.4845136170205));
#48784=CARTESIAN_POINT('Ctrl Pts',(27.8478387225673,4.06522635783411,-11.6100666615064));
#48785=CARTESIAN_POINT('Ctrl Pts',(27.8457949913781,4.06565345729717,-11.8611571983129));
#48786=CARTESIAN_POINT('Ctrl Pts',(27.8421172256742,4.06659833553217,-12.2999491112108));
#48787=CARTESIAN_POINT('Ctrl Pts',(27.83450473203,4.06914670333787,-13.1759408515894));
#48788=CARTESIAN_POINT('Ctrl Pts',(27.8236949615891,4.07399139474701,-14.4248681628644));
#48789=CARTESIAN_POINT('Ctrl Pts',(27.8159716061492,4.07805125044414,-15.5513490835192));
#48790=CARTESIAN_POINT('Ctrl Pts',(27.8124463356609,4.07987178138328,-16.3055406475485));
#48791=CARTESIAN_POINT('Ctrl Pts',(27.8105826109813,4.08079914276608,-16.8093285996371));
#48792=CARTESIAN_POINT('Ctrl Pts',(27.809806805342,4.08110792252154,-17.188491092894));
#48793=CARTESIAN_POINT('Ctrl Pts',(27.8095628641991,4.08109372160537,-17.5045006498987));
#48794=CARTESIAN_POINT('Ctrl Pts',(27.8094599355081,4.08111817749354,-17.6283252589352));
#48795=CARTESIAN_POINT('Ctrl Pts',(27.8092512127343,4.08124060372734,-17.8769952578661));
#48796=CARTESIAN_POINT('Ctrl Pts',(27.8090537139309,4.08146137275893,-18.1257048811657));
#48797=CARTESIAN_POINT('Ctrl Pts',(27.8088922868064,4.08174129213902,-18.3749058438896));
#48798=CARTESIAN_POINT('Ctrl Pts',(27.8088138483126,4.08193318914977,-18.5307639459064));
#48799=CARTESIAN_POINT('Ctrl Pts',(27.8087675428498,4.08209203328318,-18.6555488900249));
#48800=CARTESIAN_POINT('Ctrl Pts',(27.8087421554227,4.08221266043367,-18.7491773194674));
#48801=CARTESIAN_POINT('Ctrl Pts',(27.8087295957166,4.08231343946583,-18.8272385283061));
#48802=CARTESIAN_POINT('Ctrl Pts',(27.8087249750729,4.08239359400097,-18.8897085260827));
#48803=CARTESIAN_POINT('Ctrl Pts',(27.808720773895,4.08307069487227,-19.4208291291356));
#48804=CARTESIAN_POINT('Ctrl Pts',(27.809766220267,4.08419888503665,-20.440153362845));
#48805=CARTESIAN_POINT('Ctrl Pts',(27.8182931588619,4.08046837024067,-21.9572999985565));
#48806=CARTESIAN_POINT('Ctrl Pts',(27.8311639841231,4.07136164873529,-22.9768965828833));
#48807=CARTESIAN_POINT('Ctrl Pts',(27.8421249121948,4.06268008158841,-23.6149629631284));
#48808=CARTESIAN_POINT('Ctrl Pts',(27.8470036316719,4.05875847852701,-23.8695454397219));
#48809=CARTESIAN_POINT('Ctrl Pts',(27.8585771754437,4.0492928372162,-24.3769158141936));
#48810=CARTESIAN_POINT('Ctrl Pts',(27.8829116671664,4.02899651239132,-25.2639735759599));
#48811=CARTESIAN_POINT('Ctrl Pts',(27.9251515127041,3.99244565770101,-26.5254803374876));
#48812=CARTESIAN_POINT('Ctrl Pts',(27.975597257599,3.94679410327626,-28.0273674093273));
#48813=CARTESIAN_POINT('Ctrl Pts',(28.001404566098,3.92264214621878,-29.0184171325543));
#48814=CARTESIAN_POINT('Ctrl Pts',(28.011633827728,3.9131270121333,-29.5724349601575));
#48815=CARTESIAN_POINT('Ctrl Pts',(28.0138570161614,3.91102844849041,-29.6977826106848));
#48816=CARTESIAN_POINT('Ctrl Pts',(28.018141578614,3.90693672684914,-29.9472368861018));
#48817=CARTESIAN_POINT('Ctrl Pts',(28.0252029585086,3.90004491183638,-30.3844944289742));
#48818=CARTESIAN_POINT('Ctrl Pts',(28.0376368063003,3.88743466921074,-31.2586216643811));
#48819=CARTESIAN_POINT('Ctrl Pts',(28.0508118216071,3.87324243377045,-32.5073230373447));
#48820=CARTESIAN_POINT('Ctrl Pts',(28.058464528192,3.86541237630078,-33.7532405839383));
#48821=CARTESIAN_POINT('Ctrl Pts',(28.061598007007,3.8636961549409,-34.7471057905053));
#48822=CARTESIAN_POINT('Ctrl Pts',(28.0622160983558,3.86446398961727,-35.24299923233));
#48823=CARTESIAN_POINT('Ctrl Pts',(28.0623363568929,3.86569332284622,-35.6153653883871));
#48824=CARTESIAN_POINT('Ctrl Pts',(28.0624084040805,3.86672772959505,-35.8648400903879));
#48825=CARTESIAN_POINT('Ctrl Pts',(28.0624249857157,3.86960165717128,-36.3632178233884));
#48826=CARTESIAN_POINT('Ctrl Pts',(28.0619088716433,3.87670634631738,-37.234748718342));
#48827=CARTESIAN_POINT('Ctrl Pts',(28.0565239559215,3.89862226927546,-38.974858080016));
#48828=CARTESIAN_POINT('Ctrl Pts',(28.0375516851198,3.9288465415769,-40.4707855447929));
#48829=CARTESIAN_POINT('Ctrl Pts',(28.0058950939431,3.95825344195036,-41.7230304683817));
#48830=CARTESIAN_POINT('Ctrl Pts',(27.9961949133861,3.96418821564324,-42.1192273100256));
#48831=CARTESIAN_POINT('Ctrl Pts',(27.9822576273785,3.96804481463516,-42.6287445473197));
#48832=CARTESIAN_POINT('Ctrl Pts',(27.96755666201,3.97036276216118,-43.1369109547469));
#48833=CARTESIAN_POINT('Ctrl Pts',(27.9474881920418,3.97195109531181,-43.7623681408787));
#48834=CARTESIAN_POINT('Ctrl Pts',(27.9199217600844,3.97701783601881,-44.4997356664036));
#48835=CARTESIAN_POINT('Ctrl Pts',(27.8933868124384,3.98789191040196,-45.1018732863831));
#48836=CARTESIAN_POINT('Ctrl Pts',(27.8696213174653,4.00280086222066,-45.5759985059116));
#48837=CARTESIAN_POINT('Ctrl Pts',(27.8504479695429,4.01761013346641,-45.927772180604));
#48838=CARTESIAN_POINT('Ctrl Pts',(27.8298393555229,4.03654503788735,-46.2756787441312));
#48839=CARTESIAN_POINT('Ctrl Pts',(27.8003406194524,4.06792328209229,-46.7343239196486));
#48840=CARTESIAN_POINT('Ctrl Pts',(27.7758603434497,4.0990316860175,-47.072428902339));
#48841=CARTESIAN_POINT('Ctrl Pts',(27.7496222602011,4.13616544021014,-47.4076655151877));
#48842=CARTESIAN_POINT('Ctrl Pts',(27.7300808308059,4.16404867107337,-47.6433623245972));
#48843=CARTESIAN_POINT('Ctrl Pts',(27.6850539923559,4.22426306029349,-48.1101929853665));
#48844=CARTESIAN_POINT('Ctrl Pts',(27.593116066249,4.34318408401633,-48.9343820357971));
#48845=CARTESIAN_POINT('Ctrl Pts',(27.4408114174443,4.54500317820541,-50.122975463761));
#48846=CARTESIAN_POINT('Ctrl Pts',(27.2755250705735,4.83476078856946,-51.5727845981512));
#48847=CARTESIAN_POINT('Ctrl Pts',(27.2061907388541,5.06456125557638,-52.5505534801801));
#48848=CARTESIAN_POINT('Ctrl Pts',(27.183551494855,5.22154654919903,-53.1641767504487));
#48849=CARTESIAN_POINT('Ctrl Pts',(27.1763563639251,5.28455046882595,-53.4037136252652));
#48850=CARTESIAN_POINT('Ctrl Pts',(27.1666283628491,5.4182927063964,-53.8883422138275));
#48851=CARTESIAN_POINT('Ctrl Pts',(27.161798484126,5.66792564631842,-54.7358199162023));
#48852=CARTESIAN_POINT('Ctrl Pts',(27.1916742338282,6.22480761952307,-56.4369091352207));
#48853=CARTESIAN_POINT('Ctrl Pts',(27.2592709585012,6.770416555555,-57.893854841528));
#48854=CARTESIAN_POINT('Ctrl Pts',(27.3024918086758,7.16866025819872,-58.9208359710296));
#48855=CARTESIAN_POINT('Ctrl Pts',(27.308267792042,7.21667437315079,-59.0431743753317));
#48856=CARTESIAN_POINT('Ctrl Pts',(27.3208610029625,7.31419109541403,-59.2892156770369));
#48857=CARTESIAN_POINT('Ctrl Pts',(27.3458092890061,7.48742213377067,-59.7190455675896));
#48858=CARTESIAN_POINT('Ctrl Pts',(27.4054139778381,7.84408431333284,-60.578846302573));
#48859=CARTESIAN_POINT('Ctrl Pts',(27.4882088196579,8.26968443491987,-61.5593398063424));
#48860=CARTESIAN_POINT('Ctrl Pts',(27.5695998286669,8.70647993816199,-62.5358329011113));
#48861=CARTESIAN_POINT('Ctrl Pts',(27.611788194642,8.95561345643034,-63.0827825152622));
#48862=CARTESIAN_POINT('Ctrl Pts',(27.6371741472353,9.12285524300534,-63.4461212682437));
#48863=CARTESIAN_POINT('Ctrl Pts',(27.6532879455544,9.23465279481759,-63.68797698079));
#48864=CARTESIAN_POINT('Ctrl Pts',(27.6680588741092,9.34685836197186,-63.9291967606));
#48865=CARTESIAN_POINT('Ctrl Pts',(27.6796050030846,9.44538682052386,-64.1396796035441));
#48866=CARTESIAN_POINT('Ctrl Pts',(27.6857786186791,9.50178161071815,-64.2597736386839));
#48867=CARTESIAN_POINT('Ctrl Pts',(27.694600528921,9.58646123109406,-64.4397203232055));
#48868=CARTESIAN_POINT('Ctrl Pts',(27.7010045164677,9.6572128452808,-64.589276980363));
#48869=CARTESIAN_POINT('Ctrl Pts',(27.7101987626557,9.77449673083689,-64.8361386585405));
#48870=CARTESIAN_POINT('Ctrl Pts',(27.7186300515028,9.89251261724371,-65.0813968670931));
#48871=CARTESIAN_POINT('Ctrl Pts',(27.7315080399507,10.135523604251,-65.5752676778135));
#48872=CARTESIAN_POINT('Ctrl Pts',(27.7447877706368,10.5706174643503,-66.4328510835051));
#48873=CARTESIAN_POINT('Ctrl Pts',(27.7435062478646,11.48013096566,-68.1432586929741));
#48874=CARTESIAN_POINT('Ctrl Pts',(27.7229022051548,12.3005800439645,-69.6263475279766));
#48875=CARTESIAN_POINT('Ctrl Pts',(27.7246885000752,12.9095176561353,-70.7774414900148));
#48876=CARTESIAN_POINT('Ctrl Pts',(27.7250295580969,13.0411787435169,-71.0261772935901));
#48877=CARTESIAN_POINT('Ctrl Pts',(27.7255384777638,13.3071441815651,-71.5280548752207));
#48878=CARTESIAN_POINT('Ctrl Pts',(27.7258701397283,13.6390881555502,-72.1534463363424));
#48879=CARTESIAN_POINT('Ctrl Pts',(27.7259037645158,14.038578087583,-72.9048957167522));
#48880=CARTESIAN_POINT('Ctrl Pts',(27.7254557241049,14.8382159491145,-74.4073405563225));
#48881=CARTESIAN_POINT('Ctrl Pts',(27.7244616541709,15.5061273143185,-75.6602517422099));
#48882=CARTESIAN_POINT('Ctrl Pts',(27.7244571580331,16.4769049386683,-77.4860026540351));
#48883=CARTESIAN_POINT('Ctrl Pts',(27.7244524507195,16.9130347404094,-78.3062352076152));
#48884=CARTESIAN_POINT('Ctrl Pts',(27.7244524507195,17.3495563277989,-79.1272129097137));
#48885=CARTESIAN_POINT('Ctrl Pts',(29.5993149956237,4.07429432543499,24.8306289799893));
#48886=CARTESIAN_POINT('Ctrl Pts',(29.5994030211458,4.07429420375214,24.7817494857571));
#48887=CARTESIAN_POINT('Ctrl Pts',(29.59949534349,4.07429407638746,24.7328710442847));
#48888=CARTESIAN_POINT('Ctrl Pts',(29.6005854466145,4.07429257198405,24.1822607664862));
#48889=CARTESIAN_POINT('Ctrl Pts',(29.6014191999821,4.07428801440418,23.1781214006778));
#48890=CARTESIAN_POINT('Ctrl Pts',(29.6033606044468,4.07427518556936,21.169519334596));
#48891=CARTESIAN_POINT('Ctrl Pts',(29.610614365,4.07426533445962,19.6653671077297));
#48892=CARTESIAN_POINT('Ctrl Pts',(29.6260068844141,4.07426137190018,18.4143195377649));
#48893=CARTESIAN_POINT('Ctrl Pts',(29.6333886063572,4.07425835334317,17.9114922155898));
#48894=CARTESIAN_POINT('Ctrl Pts',(29.6519236564938,4.074248997782,16.9074941482145));
#48895=CARTESIAN_POINT('Ctrl Pts',(29.6916804235764,4.07422988477827,15.1536809080577));
#48896=CARTESIAN_POINT('Ctrl Pts',(29.7294577809132,4.0742302222938,13.6519679097109));
#48897=CARTESIAN_POINT('Ctrl Pts',(29.7531561761526,4.07426282133815,12.397538380551));
#48898=CARTESIAN_POINT('Ctrl Pts',(29.7628464015737,4.07427993524369,11.8966022439376));
#48899=CARTESIAN_POINT('Ctrl Pts',(29.7826085546186,4.07432680774722,10.894784447323));
#48900=CARTESIAN_POINT('Ctrl Pts',(29.8070480979797,4.07440292614643,9.64227387939513));
#48901=CARTESIAN_POINT('Ctrl Pts',(29.8328361859105,4.07449964963566,8.13777685229673));
#48902=CARTESIAN_POINT('Ctrl Pts',(29.8455822861327,4.07455385603853,7.13305293157917));
#48903=CARTESIAN_POINT('Ctrl Pts',(29.8515040877241,4.07457966189139,6.50506371904686));
#48904=CARTESIAN_POINT('Ctrl Pts',(29.8537404124718,4.07459708884447,6.25493787721224));
#48905=CARTESIAN_POINT('Ctrl Pts',(29.8577314727171,4.07465518968221,5.75392922686311));
#48906=CARTESIAN_POINT('Ctrl Pts',(29.8634595996021,4.07480340043025,4.87566199267245));
#48907=CARTESIAN_POINT('Ctrl Pts',(29.8699965156647,4.07517020734333,3.11532288435605));
#48908=CARTESIAN_POINT('Ctrl Pts',(29.8674400947039,4.07520573399403,1.60804732713263));
#48909=CARTESIAN_POINT('Ctrl Pts',(29.8620878347049,4.07472089968938,0.547889031456945));
#48910=CARTESIAN_POINT('Ctrl Pts',(29.8613895600481,4.07465767536286,0.421591316014558));
#48911=CARTESIAN_POINT('Ctrl Pts',(29.8597571396638,4.07451115277002,0.169232318339714));
#48912=CARTESIAN_POINT('Ctrl Pts',(29.856317121489,4.07420506061204,-0.271871253606398));
#48913=CARTESIAN_POINT('Ctrl Pts',(29.8499161122282,4.07364689547312,-0.900625008197283));
#48914=CARTESIAN_POINT('Ctrl Pts',(29.8404860937258,4.07284305568233,-1.65337249707067));
#48915=CARTESIAN_POINT('Ctrl Pts',(29.8263547165861,4.07168110269093,-2.65530752368736));
#48916=CARTESIAN_POINT('Ctrl Pts',(29.807320426347,4.07020206040575,-3.90565497565007));
#48917=CARTESIAN_POINT('Ctrl Pts',(29.7938144989464,4.06932573664757,-4.90618427242206));
#48918=CARTESIAN_POINT('Ctrl Pts',(29.7869485492971,4.06896712283885,-5.53245729202235));
#48919=CARTESIAN_POINT('Ctrl Pts',(29.7841978202766,4.06880921526131,-5.78358305763091));
#48920=CARTESIAN_POINT('Ctrl Pts',(29.778691800741,4.06845493287361,-6.2857910547242));
#48921=CARTESIAN_POINT('Ctrl Pts',(29.7690983039301,4.0677711656481,-7.1651450030849));
#48922=CARTESIAN_POINT('Ctrl Pts',(29.7558289847445,4.06683005027031,-8.42127075077741));
#48923=CARTESIAN_POINT('Ctrl Pts',(29.7439734570452,4.06650837692734,-9.67464607355679));
#48924=CARTESIAN_POINT('Ctrl Pts',(29.7368599281075,4.06690769772748,-10.5490660751661));
#48925=CARTESIAN_POINT('Ctrl Pts',(29.7331933528798,4.06735782533445,-11.0476884332829));
#48926=CARTESIAN_POINT('Ctrl Pts',(29.7315036662616,4.06766424952826,-11.2966188177246));
#48927=CARTESIAN_POINT('Ctrl Pts',(29.7302888303135,4.06792828189808,-11.4839285689021));
#48928=CARTESIAN_POINT('Ctrl Pts',(29.7294870043292,4.06813502516679,-11.6093235894704));
#48929=CARTESIAN_POINT('Ctrl Pts',(29.7279421809126,4.06865423676777,-11.8601860900761));
#48930=CARTESIAN_POINT('Ctrl Pts',(29.725389826179,4.06981981355778,-12.2986108981964));
#48931=CARTESIAN_POINT('Ctrl Pts',(29.7208768841446,4.07300452507182,-13.1741417640586));
#48932=CARTESIAN_POINT('Ctrl Pts',(29.7159894535552,4.07896435358632,-14.4230614670945));
#48933=CARTESIAN_POINT('Ctrl Pts',(29.713271253966,4.08361336207818,-15.5504015677926));
#48934=CARTESIAN_POINT('Ctrl Pts',(29.7120630728298,4.08547635296668,-16.3055682087937));
#48935=CARTESIAN_POINT('Ctrl Pts',(29.7114079961759,4.08632655897303,-16.810110543954));
#48936=CARTESIAN_POINT('Ctrl Pts',(29.711085673268,4.08644238934912,-17.1899505619475));
#48937=CARTESIAN_POINT('Ctrl Pts',(29.7108944071852,4.08617666123501,-17.5065808020651));
#48938=CARTESIAN_POINT('Ctrl Pts',(29.7108576273923,4.08607793182161,-17.630606021894));
#48939=CARTESIAN_POINT('Ctrl Pts',(29.7109134653549,4.0859388067722,-17.8796884198289));
#48940=CARTESIAN_POINT('Ctrl Pts',(29.7111542199351,4.08585618358414,-18.1287794582781));
#48941=CARTESIAN_POINT('Ctrl Pts',(29.7115472674956,4.08580725212287,-18.3783404698916));
#48942=CARTESIAN_POINT('Ctrl Pts',(29.711851431493,4.08578080996527,-18.5344117625362));
#48943=CARTESIAN_POINT('Ctrl Pts',(29.7121258668272,4.08575951266777,-18.6593604015799));
#48944=CARTESIAN_POINT('Ctrl Pts',(29.7123464933354,4.08574189092715,-18.7531080428038));
#48945=CARTESIAN_POINT('Ctrl Pts',(29.7125419244913,4.0857249533818,-18.8312657442226));
#48946=CARTESIAN_POINT('Ctrl Pts',(29.712704719546,4.0857098145209,-18.8938109813415));
#48947=CARTESIAN_POINT('Ctrl Pts',(29.7141245567445,4.08556846233154,-19.4255598315393));
#48948=CARTESIAN_POINT('Ctrl Pts',(29.7179165159392,4.08477473745439,-20.4459195671905));
#48949=CARTESIAN_POINT('Ctrl Pts',(29.7227947595283,4.07813595568139,-21.9631847030267));
#48950=CARTESIAN_POINT('Ctrl Pts',(29.7228197405083,4.06656944330437,-22.9821417896511));
#48951=CARTESIAN_POINT('Ctrl Pts',(29.7212855264258,4.05610940139834,-23.6197858299393));
#48952=CARTESIAN_POINT('Ctrl Pts',(29.7206006154444,4.05132379121746,-23.8755233732632));
#48953=CARTESIAN_POINT('Ctrl Pts',(29.7189966927731,4.03971846009631,-24.384080615756));
#48954=CARTESIAN_POINT('Ctrl Pts',(29.7156823742808,4.01487967422658,-25.2728408188628));
#48955=CARTESIAN_POINT('Ctrl Pts',(29.7096529350652,3.97135847452742,-26.5344569657397));
#48956=CARTESIAN_POINT('Ctrl Pts',(29.7011660287891,3.92207482840445,-28.0330195389327));
#48957=CARTESIAN_POINT('Ctrl Pts',(29.6937877062663,3.90004084220167,-29.0183931840762));
#48958=CARTESIAN_POINT('Ctrl Pts',(29.6892079956831,3.89304817141064,-29.5681789460954));
#48959=CARTESIAN_POINT('Ctrl Pts',(29.6882027168309,3.89146670769311,-29.6935042542137));
#48960=CARTESIAN_POINT('Ctrl Pts',(29.6861323114497,3.88849456448362,-29.9423467419571));
#48961=CARTESIAN_POINT('Ctrl Pts',(29.6823614333076,3.88366439358369,-30.3786763102188));
#48962=CARTESIAN_POINT('Ctrl Pts',(29.6742460534377,3.87579628390308,-31.2502924258845));
#48963=CARTESIAN_POINT('Ctrl Pts',(29.6609144555033,3.87026071660242,-32.4942654758644));
#48964=CARTESIAN_POINT('Ctrl Pts',(29.6451304702306,3.87442122751028,-33.7338440750293));
#48965=CARTESIAN_POINT('Ctrl Pts',(29.6310400941273,3.88480360350046,-34.7218015165097));
#48966=CARTESIAN_POINT('Ctrl Pts',(29.6234327027725,3.89240511171261,-35.2144370370806));
#48967=CARTESIAN_POINT('Ctrl Pts',(29.6175189787847,3.8991544760285,-35.5842589899869));
#48968=CARTESIAN_POINT('Ctrl Pts',(29.6136224179486,3.90400477355977,-35.8322093983451));
#48969=CARTESIAN_POINT('Ctrl Pts',(29.6059853898096,3.91498514479027,-36.3275547496979));
#48970=CARTESIAN_POINT('Ctrl Pts',(29.5928447866597,3.9372613712976,-37.1940447974019));
#48971=CARTESIAN_POINT('Ctrl Pts',(29.5651743675474,3.99332949963186,-38.925059677524));
#48972=CARTESIAN_POINT('Ctrl Pts',(29.5330583057904,4.05686719182932,-40.414463461334));
#48973=CARTESIAN_POINT('Ctrl Pts',(29.4939991631395,4.11458157887276,-41.6622338145054));
#48974=CARTESIAN_POINT('Ctrl Pts',(29.481999865542,4.1296577793405,-42.0586700846136));
#48975=CARTESIAN_POINT('Ctrl Pts',(29.4654870958894,4.14506807273594,-42.5669781608281));
#48976=CARTESIAN_POINT('Ctrl Pts',(29.4485009083319,4.15895663671303,-43.0737203583354));
#48977=CARTESIAN_POINT('Ctrl Pts',(29.4262500169145,4.17491366446097,-43.6965311392603));
#48978=CARTESIAN_POINT('Ctrl Pts',(29.3974965002966,4.19753376495065,-44.4296641893549));
#48979=CARTESIAN_POINT('Ctrl Pts',(29.3715705382284,4.22356199850653,-45.0274643139234));
#48980=CARTESIAN_POINT('Ctrl Pts',(29.3494795130514,4.25108923091108,-45.4979018229268));
#48981=CARTESIAN_POINT('Ctrl Pts',(29.3322638627556,4.27568310557469,-45.846778881379));
#48982=CARTESIAN_POINT('Ctrl Pts',(29.314392778617,4.30479313323617,-46.1917374920439));
#48983=CARTESIAN_POINT('Ctrl Pts',(29.2896832385308,4.35032906285243,-46.6464347261138));
#48984=CARTESIAN_POINT('Ctrl Pts',(29.2702566246333,4.39295370510534,-46.9816704378597));
#48985=CARTESIAN_POINT('Ctrl Pts',(29.2501760994589,4.4422994607737,-47.3139071855016));
#48986=CARTESIAN_POINT('Ctrl Pts',(29.2351822739187,4.47751987988122,-47.5356590347669));
#48987=CARTESIAN_POINT('Ctrl Pts',(29.2002771765164,4.55768479882917,-47.9870237659329));
#48988=CARTESIAN_POINT('Ctrl Pts',(29.1288193456356,4.72142273984953,-48.7928463859593));
#48989=CARTESIAN_POINT('Ctrl Pts',(29.0117058666492,5.01407715242886,-49.9892916781006));
#48990=CARTESIAN_POINT('Ctrl Pts',(28.8869853863707,5.42531794347212,-51.4870056708363));
#48991=CARTESIAN_POINT('Ctrl Pts',(28.8383531646819,5.71474040591769,-52.5218188230081));
#48992=CARTESIAN_POINT('Ctrl Pts',(28.8272637315404,5.892048266746,-53.1805071735208));
#48993=CARTESIAN_POINT('Ctrl Pts',(28.825826739766,5.9609963501372,-53.4337737250127));
#48994=CARTESIAN_POINT('Ctrl Pts',(28.8288000690768,6.10127380632862,-53.9449231453492));
#48995=CARTESIAN_POINT('Ctrl Pts',(28.8502088233308,6.34808337843803,-54.8299403145687));
#48996=CARTESIAN_POINT('Ctrl Pts',(28.9443258702338,6.85206468914668,-56.5772621940024));
#48997=CARTESIAN_POINT('Ctrl Pts',(29.0743550579446,7.29956809649302,-58.0245962648194));
#48998=CARTESIAN_POINT('Ctrl Pts',(29.142362196496,7.63396361850681,-59.025759487261));
#48999=CARTESIAN_POINT('Ctrl Pts',(29.150368314908,7.67645094579754,-59.1530718934086));
#49000=CARTESIAN_POINT('Ctrl Pts',(29.1674383162613,7.76052935149197,-59.403928184714));
#49001=CARTESIAN_POINT('Ctrl Pts',(29.1991223274621,7.9085528314483,-59.8431987406454));
#49002=CARTESIAN_POINT('Ctrl Pts',(29.2690812034583,8.20600540902721,-60.7147381602923));
#49003=CARTESIAN_POINT('Ctrl Pts',(29.3577344780619,8.55148910181861,-61.6969370343437));
#49004=CARTESIAN_POINT('Ctrl Pts',(29.4418444288282,8.90699328456685,-62.6614155249426));
#49005=CARTESIAN_POINT('Ctrl Pts',(29.4848798671639,9.11213719381989,-63.1968645443645));
#49006=CARTESIAN_POINT('Ctrl Pts',(29.5107875800078,9.25161829540371,-63.5505543400145));
#49007=CARTESIAN_POINT('Ctrl Pts',(29.5272502284902,9.34538419914306,-63.7854673786848));
#49008=CARTESIAN_POINT('Ctrl Pts',(29.5424086917862,9.44035300080261,-64.0189839127288));
#49009=CARTESIAN_POINT('Ctrl Pts',(29.5543617511136,9.52464115379926,-64.2220783195799));
#49010=CARTESIAN_POINT('Ctrl Pts',(29.5607958107896,9.57315913640717,-64.3377676283452));
#49011=CARTESIAN_POINT('Ctrl Pts',(29.5700392154857,9.64629549385839,-64.5109277939624));
#49012=CARTESIAN_POINT('Ctrl Pts',(29.5768712110625,9.70800834440408,-64.6544478555143));
#49013=CARTESIAN_POINT('Ctrl Pts',(29.5869086511977,9.81123656178933,-64.8908706102067));
#49014=CARTESIAN_POINT('Ctrl Pts',(29.5960573924192,9.91696695876116,-65.1275057385619));
#49015=CARTESIAN_POINT('Ctrl Pts',(29.609872181182,10.1392905384201,-65.6052501796801));
#49016=CARTESIAN_POINT('Ctrl Pts',(29.6236975019776,10.5494798153022,-66.4401818001343));
#49017=CARTESIAN_POINT('Ctrl Pts',(29.6208255037327,11.4459753092593,-68.123924432973));
#49018=CARTESIAN_POINT('Ctrl Pts',(29.597720877929,12.2927174915538,-69.6119030654474));
#49019=CARTESIAN_POINT('Ctrl Pts',(29.5992865022612,12.9092073399133,-70.780618733348));
#49020=CARTESIAN_POINT('Ctrl Pts',(29.5995928254283,13.0396901616617,-71.0277553580473));
#49021=CARTESIAN_POINT('Ctrl Pts',(29.600045825416,13.305178885112,-71.5296772981996));
#49022=CARTESIAN_POINT('Ctrl Pts',(29.6003457225441,13.6362082664364,-72.1539563517124));
#49023=CARTESIAN_POINT('Ctrl Pts',(29.6003778189031,14.0354313024268,-72.9049693850447));
#49024=CARTESIAN_POINT('Ctrl Pts',(29.5999843874973,14.8350251245033,-74.4065089551867));
#49025=CARTESIAN_POINT('Ctrl Pts',(29.5991125426097,15.5040220823233,-75.6596150039117));
#49026=CARTESIAN_POINT('Ctrl Pts',(29.5991128528511,16.4753612997457,-77.4864029689));
#49027=CARTESIAN_POINT('Ctrl Pts',(29.5991129894343,16.9112819153692,-78.3062324169441));
#49028=CARTESIAN_POINT('Ctrl Pts',(29.5991129894343,17.3478035027587,-79.1272101190426));
#49029=CARTESIAN_POINT('Ctrl Pts',(31.4687069735213,4.07784582772364,24.830632914927));
#49030=CARTESIAN_POINT('Ctrl Pts',(31.4688000635425,4.07784624467808,24.7817535405126));
#49031=CARTESIAN_POINT('Ctrl Pts',(31.4688976979175,4.07784668242652,24.7328752241303));
#49032=CARTESIAN_POINT('Ctrl Pts',(31.4700505243162,4.07785183613015,24.1822662583626));
#49033=CARTESIAN_POINT('Ctrl Pts',(31.4709279702857,4.07785362025415,23.178126478299));
#49034=CARTESIAN_POINT('Ctrl Pts',(31.4729683211627,4.07785665699013,21.169527575308));
#49035=CARTESIAN_POINT('Ctrl Pts',(31.4806396876406,4.07789079203985,19.6653772917441));
#49036=CARTESIAN_POINT('Ctrl Pts',(31.4969397650137,4.07797400571134,18.4143316530787));
#49037=CARTESIAN_POINT('Ctrl Pts',(31.5047549575706,4.07801375969669,17.9115124513854));
#49038=CARTESIAN_POINT('Ctrl Pts',(31.5243755589964,4.07811333944882,16.9075189304788));
#49039=CARTESIAN_POINT('Ctrl Pts',(31.5664619580017,4.07832811607674,15.1537000124256));
#49040=CARTESIAN_POINT('Ctrl Pts',(31.6064806007486,4.07853723942291,13.6519540876285));
#49041=CARTESIAN_POINT('Ctrl Pts',(31.6316328890473,4.07867877911592,12.3974905146125));
#49042=CARTESIAN_POINT('Ctrl Pts',(31.6419227892459,4.07873805562588,11.8965403339566));
#49043=CARTESIAN_POINT('Ctrl Pts',(31.662924688753,4.07886351330506,10.8947024710264));
#49044=CARTESIAN_POINT('Ctrl Pts',(31.6889231294956,4.07902358553982,9.64217598858967));
#49045=CARTESIAN_POINT('Ctrl Pts',(31.7163820564252,4.07919813160548,8.13767926649671));
#49046=CARTESIAN_POINT('Ctrl Pts',(31.7299663429113,4.07928360551118,7.13296679681987));
#49047=CARTESIAN_POINT('Ctrl Pts',(31.7362807752421,4.07932315893059,6.50498407946279));
#49048=CARTESIAN_POINT('Ctrl Pts',(31.7386607704019,4.07933720918986,6.25474989933836));
#49049=CARTESIAN_POINT('Ctrl Pts',(31.7428928314146,4.07935913196592,5.75362660739471));
#49050=CARTESIAN_POINT('Ctrl Pts',(31.748931792919,4.07938196538265,4.8752133773194));
#49051=CARTESIAN_POINT('Ctrl Pts',(31.7557359412242,4.07938753101485,3.11496826331555));
#49052=CARTESIAN_POINT('Ctrl Pts',(31.7530991072807,4.07936570054024,1.60835609825969));
#49053=CARTESIAN_POINT('Ctrl Pts',(31.747831202818,4.07940105300397,0.548987428145391));
#49054=CARTESIAN_POINT('Ctrl Pts',(31.7471431370894,4.07940625482527,0.422828438854361));
#49055=CARTESIAN_POINT('Ctrl Pts',(31.7455308102498,4.07941788807958,0.170703857723262));
#49056=CARTESIAN_POINT('Ctrl Pts',(31.7421250519014,4.0794418507879,-0.27001683645575));
#49057=CARTESIAN_POINT('Ctrl Pts',(31.7357664534412,4.07948298217841,-0.898351856990242));
#49058=CARTESIAN_POINT('Ctrl Pts',(31.7263746716039,4.07954010204105,-1.65078035668601));
#49059=CARTESIAN_POINT('Ctrl Pts',(31.7122659162751,4.0796168459856,-2.65254930057485));
#49060=CARTESIAN_POINT('Ctrl Pts',(31.6932033012039,4.07969634396477,-3.90315909986217));
#49061=CARTESIAN_POINT('Ctrl Pts',(31.6795777768752,4.07971951734305,-4.90443422286743));
#49062=CARTESIAN_POINT('Ctrl Pts',(31.6725906366524,4.07970971933928,-5.5313148080553));
#49063=CARTESIAN_POINT('Ctrl Pts',(31.6697485046803,4.07969691159586,-5.78231976151824));
#49064=CARTESIAN_POINT('Ctrl Pts',(31.6639217657505,4.079640700228,-6.28454501781444));
#49065=CARTESIAN_POINT('Ctrl Pts',(31.6534779552804,4.07947905658651,-7.16394174025885));
#49066=CARTESIAN_POINT('Ctrl Pts',(31.6386066476219,4.07915577397756,-8.42056430436979));
#49067=CARTESIAN_POINT('Ctrl Pts',(31.6257945049036,4.07895378579147,-9.67488459875914));
#49068=CARTESIAN_POINT('Ctrl Pts',(31.618960078523,4.07900247231926,-10.5502342652491));
#49069=CARTESIAN_POINT('Ctrl Pts',(31.6158110476425,4.07910303501304,-11.0494586612985));
#49070=CARTESIAN_POINT('Ctrl Pts',(31.6145143722234,4.0791799694181,-11.2987140498463));
#49071=CARTESIAN_POINT('Ctrl Pts',(31.6136515985956,4.07924915509268,-11.4862856583363));
#49072=CARTESIAN_POINT('Ctrl Pts',(31.6131274815052,4.07930249851795,-11.6121482637079));
#49073=CARTESIAN_POINT('Ctrl Pts',(31.6122901367677,4.07944550038625,-11.8637173726598));
#49074=CARTESIAN_POINT('Ctrl Pts',(31.6113447622238,4.07978032212702,-12.3033175014865));
#49075=CARTESIAN_POINT('Ctrl Pts',(31.6112783421474,4.08071914839239,-13.1805656977755));
#49076=CARTESIAN_POINT('Ctrl Pts',(31.6148523621694,4.08257692351233,-14.4303175338137));
#49077=CARTESIAN_POINT('Ctrl Pts',(31.6187202822993,4.08401670864369,-15.5562589293961));
#49078=CARTESIAN_POINT('Ctrl Pts',(31.6199776863949,4.08441232747168,-16.3094955671417));
#49079=CARTESIAN_POINT('Ctrl Pts',(31.6203606822337,4.08449522846437,-16.8124947920013));
#49080=CARTESIAN_POINT('Ctrl Pts',(31.620050118909,4.08431569993787,-17.1908997106453));
#49081=CARTESIAN_POINT('Ctrl Pts',(31.619310512475,4.08400162739168,-17.5062483640748));
#49082=CARTESIAN_POINT('Ctrl Pts',(31.6190954350977,4.0838836770891,-17.6311496466164));
#49083=CARTESIAN_POINT('Ctrl Pts',(31.6189782372705,4.08356741764711,-17.8809905469006));
#49084=CARTESIAN_POINT('Ctrl Pts',(31.6192751513199,4.08316160710082,-18.1309141329983));
#49085=CARTESIAN_POINT('Ctrl Pts',(31.6198655894181,4.08266314623051,-18.3809095800197));
#49086=CARTESIAN_POINT('Ctrl Pts',(31.6203368834378,4.08231761180404,-18.5371934816371));
#49087=CARTESIAN_POINT('Ctrl Pts',(31.6207596883997,4.08202049119935,-18.6622410423212));
#49088=CARTESIAN_POINT('Ctrl Pts',(31.6210967681186,4.08178802013735,-18.7560379646719));
#49089=CARTESIAN_POINT('Ctrl Pts',(31.6213915535343,4.08158651687251,-18.8342116652941));
#49090=CARTESIAN_POINT('Ctrl Pts',(31.6216335004812,4.08142051212769,-18.8967560255184));
#49091=CARTESIAN_POINT('Ctrl Pts',(31.6237261069884,4.07998516218906,-19.4284203111848));
#49092=CARTESIAN_POINT('Ctrl Pts',(31.6285980996611,4.0765381756599,-20.4459114336292));
#49093=CARTESIAN_POINT('Ctrl Pts',(31.6245096349564,4.07053585147111,-21.9527148393062));
#49094=CARTESIAN_POINT('Ctrl Pts',(31.6054527654478,4.06783851514021,-22.9604284739142));
#49095=CARTESIAN_POINT('Ctrl Pts',(31.5851502219919,4.06703322930736,-23.5894247381428));
#49096=CARTESIAN_POINT('Ctrl Pts',(31.5761557495189,4.06655258278944,-23.8414590433909));
#49097=CARTESIAN_POINT('Ctrl Pts',(31.5544793458723,4.06506216304023,-24.3436418296724));
#49098=CARTESIAN_POINT('Ctrl Pts',(31.5078634265954,4.0612182643314,-25.2229432881163));
#49099=CARTESIAN_POINT('Ctrl Pts',(31.4220683331932,4.05296711392328,-26.4759183308666));
#49100=CARTESIAN_POINT('Ctrl Pts',(31.3083228675675,4.04194537238345,-27.9716356437027));
#49101=CARTESIAN_POINT('Ctrl Pts',(31.241208833653,4.03900947809416,-28.9617904982848));
#49102=CARTESIAN_POINT('Ctrl Pts',(31.2102909779811,4.04093054226757,-29.5163696380308));
#49103=CARTESIAN_POINT('Ctrl Pts',(31.2034300134135,4.04147801988664,-29.6416653102345));
#49104=CARTESIAN_POINT('Ctrl Pts',(31.189882917682,4.04255656273384,-29.8910246976545));
#49105=CARTESIAN_POINT('Ctrl Pts',(31.166602866815,4.0446452051083,-30.3278701302552));
#49106=CARTESIAN_POINT('Ctrl Pts',(31.1217485478009,4.04968077060979,-31.2004186275354));
#49107=CARTESIAN_POINT('Ctrl Pts',(31.0625616532806,4.06093324452965,-32.4447029374165));
#49108=CARTESIAN_POINT('Ctrl Pts',(31.0097944727872,4.08113968644785,-33.6836095292349));
#49109=CARTESIAN_POINT('Ctrl Pts',(30.9713218638268,4.10469684596768,-34.6704253479765));
#49110=CARTESIAN_POINT('Ctrl Pts',(30.9533849362174,4.11934855872571,-35.1623178497854));
#49111=CARTESIAN_POINT('Ctrl Pts',(30.9403650528998,4.13152953971904,-35.5315351808384));
#49112=CARTESIAN_POINT('Ctrl Pts',(30.931962014745,4.14013412429074,-35.7797086367032));
#49113=CARTESIAN_POINT('Ctrl Pts',(30.9163631552964,4.1588670841948,-36.2752055194683));
#49114=CARTESIAN_POINT('Ctrl Pts',(30.8918999880386,4.1956918462424,-37.1421567095371));
#49115=CARTESIAN_POINT('Ctrl Pts',(30.8520875761949,4.28367231496665,-38.8741422979402));
#49116=CARTESIAN_POINT('Ctrl Pts',(30.824585745144,4.37976812029803,-40.3635451829372));
#49117=CARTESIAN_POINT('Ctrl Pts',(30.795647337687,4.4659231753878,-41.6110017876324));
#49118=CARTESIAN_POINT('Ctrl Pts',(30.7861469487672,4.48985586971024,-42.0060413061234));
#49119=CARTESIAN_POINT('Ctrl Pts',(30.7739391456391,4.51690834540139,-42.5137074529757));
#49120=CARTESIAN_POINT('Ctrl Pts',(30.7616615007434,4.54256551313821,-43.0199495146523));
#49121=CARTESIAN_POINT('Ctrl Pts',(30.7464969580757,4.57345561727011,-43.6428716432487));
#49122=CARTESIAN_POINT('Ctrl Pts',(30.7287732714005,4.61477282839475,-44.377217515882));
#49123=CARTESIAN_POINT('Ctrl Pts',(30.7147709802563,4.65741603609451,-44.977016357536));
#49124=CARTESIAN_POINT('Ctrl Pts',(30.704346797177,4.69924303580619,-45.4497221191383));
#49125=CARTESIAN_POINT('Ctrl Pts',(30.6969679517773,4.73509707802723,-45.8005692897468));
#49126=CARTESIAN_POINT('Ctrl Pts',(30.690109753667,4.77608970526089,-46.1477696955023));
#49127=CARTESIAN_POINT('Ctrl Pts',(30.6817966335565,4.83845043678961,-46.6057570928931));
#49128=CARTESIAN_POINT('Ctrl Pts',(30.6765542601007,4.89475954321947,-46.9437642923097));
#49129=CARTESIAN_POINT('Ctrl Pts',(30.6722371976059,4.95880011563281,-47.2786017031431));
#49130=CARTESIAN_POINT('Ctrl Pts',(30.6697139007788,5.00309856561159,-47.4923421202682));
#49131=CARTESIAN_POINT('Ctrl Pts',(30.6614671304962,5.10626565674607,-47.9366598900565));
#49132=CARTESIAN_POINT('Ctrl Pts',(30.6411558365244,5.31864108263074,-48.7344018720708));
#49133=CARTESIAN_POINT('Ctrl Pts',(30.5988468763563,5.69851407103839,-49.9380115029223));
#49134=CARTESIAN_POINT('Ctrl Pts',(30.5487314548176,6.20918068978983,-51.4657504505471));
#49135=CARTESIAN_POINT('Ctrl Pts',(30.5360732835478,6.53535513791848,-52.5416398339894));
#49136=CARTESIAN_POINT('Ctrl Pts',(30.5436070090105,6.71763690250309,-53.2362337071639));
#49137=CARTESIAN_POINT('Ctrl Pts',(30.5499302831122,6.78717803372439,-53.5040512714113));
#49138=CARTESIAN_POINT('Ctrl Pts',(30.5696211270458,6.92150899013218,-54.0411043082594));
#49139=CARTESIAN_POINT('Ctrl Pts',(30.6230773435729,7.14154958243025,-54.9641411305007));
#49140=CARTESIAN_POINT('Ctrl Pts',(30.7912110839135,7.5404246546231,-56.7578792993563));
#49141=CARTESIAN_POINT('Ctrl Pts',(30.9860329592378,7.84676198898512,-58.1861024721125));
#49142=CARTESIAN_POINT('Ctrl Pts',(31.0752271371353,8.09892223662111,-59.1454725131373));
#49143=CARTESIAN_POINT('Ctrl Pts',(31.0853218009868,8.13314032704081,-59.2761377230917));
#49144=CARTESIAN_POINT('Ctrl Pts',(31.1058757443481,8.1990465314762,-59.5286092028247));
#49145=CARTESIAN_POINT('Ctrl Pts',(31.1414352880725,8.31446356687814,-59.9722776557029));
#49146=CARTESIAN_POINT('Ctrl Pts',(31.2113800066628,8.54226303971064,-60.8472925910589));
#49147=CARTESIAN_POINT('Ctrl Pts',(31.2857763710018,8.80550296428891,-61.8258299092601));
#49148=CARTESIAN_POINT('Ctrl Pts',(31.3507242714438,9.08534203953185,-62.7766992498672));
#49149=CARTESIAN_POINT('Ctrl Pts',(31.3830181518182,9.25156079466651,-63.3011287796442));
#49150=CARTESIAN_POINT('Ctrl Pts',(31.4025052137197,9.36699878875882,-63.6460583027522));
#49151=CARTESIAN_POINT('Ctrl Pts',(31.4149352565952,9.44526104167027,-63.8747808577239));
#49152=CARTESIAN_POINT('Ctrl Pts',(31.4264914430533,9.52554998192621,-64.1015753771454));
#49153=CARTESIAN_POINT('Ctrl Pts',(31.4357981005218,9.59776145502393,-64.2983655263945));
#49154=CARTESIAN_POINT('Ctrl Pts',(31.440879219036,9.63960551034226,-64.4103355604511));
#49155=CARTESIAN_POINT('Ctrl Pts',(31.44826118774,9.70296125674408,-64.5778027379595));
#49156=CARTESIAN_POINT('Ctrl Pts',(31.4539039935886,9.75701258305106,-64.7163456025992));
#49157=CARTESIAN_POINT('Ctrl Pts',(31.4625469125157,9.84823769697998,-64.9442418696047));
#49158=CARTESIAN_POINT('Ctrl Pts',(31.4704018060749,9.94247260813082,-65.1716937489053));
#49159=CARTESIAN_POINT('Ctrl Pts',(31.482138511333,10.1459603455991,-65.6337942490935));
#49160=CARTESIAN_POINT('Ctrl Pts',(31.4935293569103,10.5331942370106,-66.4464679478753));
#49161=CARTESIAN_POINT('Ctrl Pts',(31.489739600742,11.4180616192753,-68.1055723847549));
#49162=CARTESIAN_POINT('Ctrl Pts',(31.4689354929894,12.2901135094031,-69.5979852881751));
#49163=CARTESIAN_POINT('Ctrl Pts',(31.4697806871723,12.9140139982325,-70.7834972100309));
#49164=CARTESIAN_POINT('Ctrl Pts',(31.469989039785,13.0434440655494,-71.0291593677387));
#49165=CARTESIAN_POINT('Ctrl Pts',(31.470277045121,13.3085758311122,-71.5311884003762));
#49166=CARTESIAN_POINT('Ctrl Pts',(31.4704734126682,13.6388199643196,-72.1544788905691));
#49167=CARTESIAN_POINT('Ctrl Pts',(31.4704957141681,14.0378297615307,-72.9051396997616));
#49168=CARTESIAN_POINT('Ctrl Pts',(31.4702487463697,14.8373791344158,-74.4059019368014));
#49169=CARTESIAN_POINT('Ctrl Pts',(31.4696762369953,15.5072839216342,-75.6591361257847));
#49170=CARTESIAN_POINT('Ctrl Pts',(31.4696585255378,16.4790900577772,-77.4867586602277));
#49171=CARTESIAN_POINT('Ctrl Pts',(31.4696575427394,16.9148362784751,-78.3062378482243));
#49172=CARTESIAN_POINT('Ctrl Pts',(31.4696575427393,17.3513578658645,-79.1272155503226));
#49173=CARTESIAN_POINT('Ctrl Pts',(33.7970285977012,4.09821853641055,24.8306494002684));
#49174=CARTESIAN_POINT('Ctrl Pts',(33.7971282050739,4.09822036764379,24.781770541049));
#49175=CARTESIAN_POINT('Ctrl Pts',(33.7972326733307,4.09822228839506,24.7328927512991));
#49176=CARTESIAN_POINT('Ctrl Pts',(33.7984662721378,4.09824493829563,24.1822897741847));
#49177=CARTESIAN_POINT('Ctrl Pts',(33.7994033543667,4.09826758173109,23.1781553718533));
#49178=CARTESIAN_POINT('Ctrl Pts',(33.8015798097595,4.09832432028853,21.1695681394724));
#49179=CARTESIAN_POINT('Ctrl Pts',(33.809789540473,4.09847426299123,19.6654230517925));
#49180=CARTESIAN_POINT('Ctrl Pts',(33.8272430182452,4.09876605720855,18.4143804676529));
#49181=CARTESIAN_POINT('Ctrl Pts',(33.8356105809491,4.09890898968022,17.911592099575));
#49182=CARTESIAN_POINT('Ctrl Pts',(33.8566174432594,4.09927273294534,16.9076192478544));
#49183=CARTESIAN_POINT('Ctrl Pts',(33.9016781945664,4.10005254213659,15.1537923232443));
#49184=CARTESIAN_POINT('Ctrl Pts',(33.9445372161864,4.10075015715253,13.6519415878471));
#49185=CARTESIAN_POINT('Ctrl Pts',(33.9714908584138,4.10111414654576,12.3973491179456));
#49186=CARTESIAN_POINT('Ctrl Pts',(33.9825187974683,4.10125490028183,11.8963456467522));
#49187=CARTESIAN_POINT('Ctrl Pts',(34.0050307592515,4.10151625570471,10.8944298036317));
#49188=CARTESIAN_POINT('Ctrl Pts',(34.0329083871325,4.10179725385752,9.64184755920691));
#49189=CARTESIAN_POINT('Ctrl Pts',(34.0623629492985,4.10205582204821,8.13735768627829));
#49190=CARTESIAN_POINT('Ctrl Pts',(34.0769482549485,4.10216300191832,7.13269822728231));
#49191=CARTESIAN_POINT('Ctrl Pts',(34.0837323382561,4.10220971726014,6.50475899129787));
#49192=CARTESIAN_POINT('Ctrl Pts',(34.0862739652426,4.10221810797943,6.25443092752143));
#49193=CARTESIAN_POINT('Ctrl Pts',(34.0907407487412,4.1021998457707,5.75321624620991));
#49194=CARTESIAN_POINT('Ctrl Pts',(34.0969930980285,4.1020905575295,4.8746861490407));
#49195=CARTESIAN_POINT('Ctrl Pts',(34.103685094322,4.10170822554426,3.11454451952558));
#49196=CARTESIAN_POINT('Ctrl Pts',(34.1009489428922,4.1015395669589,1.60853147061917));
#49197=CARTESIAN_POINT('Ctrl Pts',(34.0964395095961,4.10194657169397,0.549856156660557));
#49198=CARTESIAN_POINT('Ctrl Pts',(34.0958477606116,4.10200085509198,0.423813583599584));
#49199=CARTESIAN_POINT('Ctrl Pts',(34.0944545982225,4.1021276108948,0.171887827235955));
#49200=CARTESIAN_POINT('Ctrl Pts',(34.0914952451723,4.10239545883754,-0.268508702835578));
#49201=CARTESIAN_POINT('Ctrl Pts',(34.0859339137065,4.10288703977165,-0.896487986774876));
#49202=CARTESIAN_POINT('Ctrl Pts',(34.0776481013222,4.10360530012229,-1.64864637123662));
#49203=CARTESIAN_POINT('Ctrl Pts',(34.0651183943709,4.10464258775604,-2.65027867683541));
#49204=CARTESIAN_POINT('Ctrl Pts',(34.0479680651029,4.10595923985949,-3.90110177373963));
#49205=CARTESIAN_POINT('Ctrl Pts',(34.0353734908973,4.10670070469566,-4.90298322940253));
#49206=CARTESIAN_POINT('Ctrl Pts',(34.0287148154635,4.10697788756576,-5.53030604893786));
#49207=CARTESIAN_POINT('Ctrl Pts',(34.0259683562906,4.10713807836924,-5.78050396910268));
#49208=CARTESIAN_POINT('Ctrl Pts',(34.020212265199,4.1076119846857,-6.28196993185703));
#49209=CARTESIAN_POINT('Ctrl Pts',(34.0096219631666,4.10873822584859,-7.16041794032691));
#49210=CARTESIAN_POINT('Ctrl Pts',(33.9940490444314,4.11055545053572,-8.41785751623567));
#49211=CARTESIAN_POINT('Ctrl Pts',(33.9805692707932,4.11102346648838,-9.67551174623761));
#49212=CARTESIAN_POINT('Ctrl Pts',(33.9736569921043,4.10977984028363,-10.5546102028952));
#49213=CARTESIAN_POINT('Ctrl Pts',(33.9706278463524,4.10849838473789,-11.0563763144717));
#49214=CARTESIAN_POINT('Ctrl Pts',(33.9694562894734,4.10764406600035,-11.3070255162176));
#49215=CARTESIAN_POINT('Ctrl Pts',(33.9687138816181,4.10691458550222,-11.4957406859376));
#49216=CARTESIAN_POINT('Ctrl Pts',(33.9683305005745,4.10635066232301,-11.623881277403));
#49217=CARTESIAN_POINT('Ctrl Pts',(33.9679941469379,4.10492260948579,-11.8788305489746));
#49218=CARTESIAN_POINT('Ctrl Pts',(33.9684435458204,4.1017019555296,-12.324027240282));
#49219=CARTESIAN_POINT('Ctrl Pts',(33.9728128464778,4.09283721169593,-13.2090959126564));
#49220=CARTESIAN_POINT('Ctrl Pts',(33.9847244786488,4.07593321409288,-14.4608181274448));
#49221=CARTESIAN_POINT('Ctrl Pts',(33.9926489282834,4.06270791099737,-15.5773441815626));
#49222=CARTESIAN_POINT('Ctrl Pts',(33.9926559322855,4.05823257350317,-16.3199250450109));
#49223=CARTESIAN_POINT('Ctrl Pts',(33.9909580318512,4.05665527841438,-16.8146719247331));
#49224=CARTESIAN_POINT('Ctrl Pts',(33.9875228023187,4.05725463110933,-17.1855451243572));
#49225=CARTESIAN_POINT('Ctrl Pts',(33.9830696704345,4.05905098401968,-17.4941735460199));
#49226=CARTESIAN_POINT('Ctrl Pts',(33.9814056436223,4.05963041847793,-17.6215761453741));
#49227=CARTESIAN_POINT('Ctrl Pts',(33.9783372416422,4.0605977981083,-17.8728790271971));
#49228=CARTESIAN_POINT('Ctrl Pts',(33.9756133255376,4.06127516748637,-18.1247044351465));
#49229=CARTESIAN_POINT('Ctrl Pts',(33.973037750308,4.06185452718477,-18.375286557969));
#49230=CARTESIAN_POINT('Ctrl Pts',(33.9714660496556,4.0621965310781,-18.5317727670195));
#49231=CARTESIAN_POINT('Ctrl Pts',(33.9702063188726,4.06248084755737,-18.6567506225113));
#49232=CARTESIAN_POINT('Ctrl Pts',(33.9692570300578,4.06270263149698,-18.7504177013163));
#49233=CARTESIAN_POINT('Ctrl Pts',(33.968457893804,4.06289856079581,-18.8284017384575));
#49234=CARTESIAN_POINT('Ctrl Pts',(33.9678105003257,4.06306458795975,-18.8907509910024));
#49235=CARTESIAN_POINT('Ctrl Pts',(33.9622595988739,4.06452886023594,-19.4204906348209));
#49236=CARTESIAN_POINT('Ctrl Pts',(33.9501447783641,4.06940351449382,-20.4259725248278));
#49237=CARTESIAN_POINT('Ctrl Pts',(33.9049300086482,4.09926664542524,-21.8905015715613));
#49238=CARTESIAN_POINT('Ctrl Pts',(33.8412587973299,4.14138642964727,-22.8524069521049));
#49239=CARTESIAN_POINT('Ctrl Pts',(33.7871591392881,4.17532867843808,-23.4478026640479));
#49240=CARTESIAN_POINT('Ctrl Pts',(33.7635278638142,4.18995873126553,-23.6803950602424));
#49241=CARTESIAN_POINT('Ctrl Pts',(33.7090682763451,4.22238043752065,-24.1517312196106));
#49242=CARTESIAN_POINT('Ctrl Pts',(33.5973815953313,4.28598348845388,-24.985690223896));
#49243=CARTESIAN_POINT('Ctrl Pts',(33.4076798001897,4.38631421939129,-26.2072358071185));
#49244=CARTESIAN_POINT('Ctrl Pts',(33.1821937759443,4.50076189696166,-27.7182987079329));
#49245=CARTESIAN_POINT('Ctrl Pts',(33.0624190729428,4.56821605762625,-28.7530471474503));
#49246=CARTESIAN_POINT('Ctrl Pts',(33.0096393889443,4.60295930013888,-29.3408905338608));
#49247=CARTESIAN_POINT('Ctrl Pts',(32.9980607975317,4.61041835741825,-29.4669949640881));
#49248=CARTESIAN_POINT('Ctrl Pts',(32.9754196679533,4.6252360792123,-29.7216007220453));
#49249=CARTESIAN_POINT('Ctrl Pts',(32.9371999997291,4.65065906069946,-30.1655944655998));
#49250=CARTESIAN_POINT('Ctrl Pts',(32.8660890777854,4.70016473201003,-31.0531853689413));
#49251=CARTESIAN_POINT('Ctrl Pts',(32.7790451317061,4.76997238849969,-32.3164739882917));
#49252=CARTESIAN_POINT('Ctrl Pts',(32.7095781231124,4.84516280801569,-33.5733152642523));
#49253=CARTESIAN_POINT('Ctrl Pts',(32.6637818788412,4.9118723010392,-34.5737015394328));
#49254=CARTESIAN_POINT('Ctrl Pts',(32.6442194323323,4.94810389547688,-35.0721798075551));
#49255=CARTESIAN_POINT('Ctrl Pts',(32.6306781266863,4.97656239475885,-35.4463068277234));
#49256=CARTESIAN_POINT('Ctrl Pts',(32.6221171787377,4.99614191803143,-35.6988034335822));
#49257=CARTESIAN_POINT('Ctrl Pts',(32.6071741780158,5.03671215964242,-36.202030201179));
#49258=CARTESIAN_POINT('Ctrl Pts',(32.5861604767153,5.11152796365657,-37.0819022504336));
#49259=CARTESIAN_POINT('Ctrl Pts',(32.5609699932313,5.27390711956672,-38.8361707540274));
#49260=CARTESIAN_POINT('Ctrl Pts',(32.554981900109,5.42853889027826,-40.3382427694044));
#49261=CARTESIAN_POINT('Ctrl Pts',(32.5459371475621,5.55790806072204,-41.5936066720029));
#49262=CARTESIAN_POINT('Ctrl Pts',(32.5420138658918,5.59421486056015,-41.984174813383));
#49263=CARTESIAN_POINT('Ctrl Pts',(32.5373730788485,5.6380683728732,-42.4923196178453));
#49264=CARTESIAN_POINT('Ctrl Pts',(32.5327641984067,5.68031193203146,-42.9997665311057));
#49265=CARTESIAN_POINT('Ctrl Pts',(32.5276504291001,5.7315365234597,-43.627710232422));
#49266=CARTESIAN_POINT('Ctrl Pts',(32.5232803629278,5.79608129494499,-44.3725340641912));
#49267=CARTESIAN_POINT('Ctrl Pts',(32.5219296485828,5.85686717131584,-44.9847842771367));
#49268=CARTESIAN_POINT('Ctrl Pts',(32.5228946316512,5.91237385605236,-45.4693743176206));
#49269=CARTESIAN_POINT('Ctrl Pts',(32.5247246540156,5.95805395638314,-45.8300154304055));
#49270=CARTESIAN_POINT('Ctrl Pts',(32.5278247101902,6.00842253105358,-46.1877882470674));
#49271=CARTESIAN_POINT('Ctrl Pts',(32.5339569753228,6.08265565062642,-46.6607371758016));
#49272=CARTESIAN_POINT('Ctrl Pts',(32.5408734284837,6.14715785201562,-47.0107614030028));
#49273=CARTESIAN_POINT('Ctrl Pts',(32.5500619378399,6.21885511206134,-47.3576960899547));
#49274=CARTESIAN_POINT('Ctrl Pts',(32.5581144745922,6.26895137514107,-47.575578936988));
#49275=CARTESIAN_POINT('Ctrl Pts',(32.5744820127434,6.38404756662234,-48.0281094073996));
#49276=CARTESIAN_POINT('Ctrl Pts',(32.6060226061346,6.61689911901625,-48.8347242072648));
#49277=CARTESIAN_POINT('Ctrl Pts',(32.6558408667422,7.01549898084816,-50.044478682879));
#49278=CARTESIAN_POINT('Ctrl Pts',(32.7274054405778,7.51367808139426,-51.5865810358887));
#49279=CARTESIAN_POINT('Ctrl Pts',(32.7906493652785,7.79578840821404,-52.6881528625075));
#49280=CARTESIAN_POINT('Ctrl Pts',(32.8386819868785,7.93232635462115,-53.4058345890841));
#49281=CARTESIAN_POINT('Ctrl Pts',(32.8597479739066,7.9842516044768,-53.6958302088392));
#49282=CARTESIAN_POINT('Ctrl Pts',(32.9108190532738,8.07144100511394,-54.2663327052882));
#49283=CARTESIAN_POINT('Ctrl Pts',(33.019547085727,8.18761287487766,-55.2415234092912));
#49284=CARTESIAN_POINT('Ctrl Pts',(33.2931164552012,8.31125407880594,-57.0871404591677));
#49285=CARTESIAN_POINT('Ctrl Pts',(33.5358997999199,8.36694047219133,-58.4509986593335));
#49286=CARTESIAN_POINT('Ctrl Pts',(33.629766996932,8.5000635463776,-59.318605589913));
#49287=CARTESIAN_POINT('Ctrl Pts',(33.640526434217,8.51993120779359,-59.4460956936651));
#49288=CARTESIAN_POINT('Ctrl Pts',(33.6605628283255,8.55836196716042,-59.6880631583425));
#49289=CARTESIAN_POINT('Ctrl Pts',(33.6915063919367,8.6285990716164,-60.1163445282915));
#49290=CARTESIAN_POINT('Ctrl Pts',(33.7386558114479,8.77755295787295,-60.9619250812387));
#49291=CARTESIAN_POINT('Ctrl Pts',(33.7653691776996,8.97465054982133,-61.9147245541562));
#49292=CARTESIAN_POINT('Ctrl Pts',(33.7783381708424,9.2056620343217,-62.8462653352938));
#49293=CARTESIAN_POINT('Ctrl Pts',(33.7829177528305,9.34955005789062,-63.3624432207782));
#49294=CARTESIAN_POINT('Ctrl Pts',(33.7858406170772,9.4517420062381,-63.702857887243));
#49295=CARTESIAN_POINT('Ctrl Pts',(33.7878203178101,9.52157568263138,-63.9288452877205));
#49296=CARTESIAN_POINT('Ctrl Pts',(33.7899354442175,9.59399559459775,-64.153275087536));
#49297=CARTESIAN_POINT('Ctrl Pts',(33.7920791446143,9.65972535332635,-64.3483419885931));
#49298=CARTESIAN_POINT('Ctrl Pts',(33.7934095898122,9.69797055378872,-64.4594218829255));
#49299=CARTESIAN_POINT('Ctrl Pts',(33.7955226256635,9.75602384276808,-64.6256403883808));
#49300=CARTESIAN_POINT('Ctrl Pts',(33.7975472234733,9.80585938053793,-64.7633453371639));
#49301=CARTESIAN_POINT('Ctrl Pts',(33.8013790957159,9.89023306448245,-64.9899273901492));
#49302=CARTESIAN_POINT('Ctrl Pts',(33.8049049794753,9.97508253817971,-65.2076712376803));
#49303=CARTESIAN_POINT('Ctrl Pts',(33.810078935351,10.164584800907,-65.6573965312079));
#49304=CARTESIAN_POINT('Ctrl Pts',(33.814875131772,10.5341174610181,-66.4507763384098));
#49305=CARTESIAN_POINT('Ctrl Pts',(33.8119694278541,11.4112563331564,-68.0910591200175));
#49306=CARTESIAN_POINT('Ctrl Pts',(33.8009691673892,12.3048066618138,-69.5863841076439));
#49307=CARTESIAN_POINT('Ctrl Pts',(33.8003410766881,12.9352837166494,-70.7856886607226));
#49308=CARTESIAN_POINT('Ctrl Pts',(33.8003831704564,13.0639995479544,-71.0302511003522));
#49309=CARTESIAN_POINT('Ctrl Pts',(33.8003672239512,13.3290522508635,-71.5325143948912));
#49310=CARTESIAN_POINT('Ctrl Pts',(33.8003895503051,13.658830490243,-72.1551409816205));
#49311=CARTESIAN_POINT('Ctrl Pts',(33.8004007241132,14.0577532219815,-72.9056498879106));
#49312=CARTESIAN_POINT('Ctrl Pts',(33.8004378474102,14.857255052155,-74.4059521057206));
#49313=CARTESIAN_POINT('Ctrl Pts',(33.8004407127823,15.5275910160368,-75.6591109780893));
#49314=CARTESIAN_POINT('Ctrl Pts',(33.8003969455338,16.4996040288826,-77.4870418399451));
#49315=CARTESIAN_POINT('Ctrl Pts',(33.8004049519044,16.9352520962529,-78.3062943979546));
#49316=CARTESIAN_POINT('Ctrl Pts',(33.8004049519044,17.3717736836423,-79.1272721000527));
#49317=CARTESIAN_POINT('Ctrl Pts',(36.1186449350266,4.15213573292229,24.8306479566142));
#49318=CARTESIAN_POINT('Ctrl Pts',(36.118751955118,4.15213910516501,24.7817690707861));
#49319=CARTESIAN_POINT('Ctrl Pts',(36.1188641989714,4.1521426412137,24.7328912549376));
#49320=CARTESIAN_POINT('Ctrl Pts',(36.1201895134702,4.15218440716461,24.1822879344031));
#49321=CARTESIAN_POINT('Ctrl Pts',(36.1212095746272,4.15222197704974,23.1781532987238));
#49322=CARTESIAN_POINT('Ctrl Pts',(36.1235891875911,4.15231267361934,21.1695652709454));
#49323=CARTESIAN_POINT('Ctrl Pts',(36.1324076246725,4.15259078195511,19.6654195537376));
#49324=CARTESIAN_POINT('Ctrl Pts',(36.1510886615449,4.15315263302483,18.4143757893904));
#49325=CARTESIAN_POINT('Ctrl Pts',(36.1600511061703,4.15342376468628,17.9115794728721));
#49326=CARTESIAN_POINT('Ctrl Pts',(36.1825617524411,4.15410772118649,16.9076013119465));
#49327=CARTESIAN_POINT('Ctrl Pts',(36.2308457613202,4.15557255720582,15.1537769141764));
#49328=CARTESIAN_POINT('Ctrl Pts',(36.2766768526778,4.15693796052261,13.6519512351655));
#49329=CARTESIAN_POINT('Ctrl Pts',(36.3053368834683,4.15774125966134,12.3973909479109));
#49330=CARTESIAN_POINT('Ctrl Pts',(36.3170450031152,4.15806369848647,11.8963997715426));
#49331=CARTESIAN_POINT('Ctrl Pts',(36.34088818551,4.1587014714145,10.894499728827));
#49332=CARTESIAN_POINT('Ctrl Pts',(36.3703244215625,4.15946462904555,9.64192212646858));
#49333=CARTESIAN_POINT('Ctrl Pts',(36.4013422084235,4.16024013195097,8.13742396783722));
#49334=CARTESIAN_POINT('Ctrl Pts',(36.416660456582,4.16061455607174,7.13274788009381));
#49335=CARTESIAN_POINT('Ctrl Pts',(36.4237783626832,4.16078504527602,6.5048016068737));
#49336=CARTESIAN_POINT('Ctrl Pts',(36.4264294595897,4.16084483231786,6.25454567739911));
#49337=CARTESIAN_POINT('Ctrl Pts',(36.4310320312793,4.16093593632228,5.75340726173014));
#49338=CARTESIAN_POINT('Ctrl Pts',(36.4373308648874,4.16102908765525,4.87497226920453));
#49339=CARTESIAN_POINT('Ctrl Pts',(36.4436051613166,4.16100828955505,3.11477173871754));
#49340=CARTESIAN_POINT('Ctrl Pts',(36.4404304587637,4.16085273295468,1.60829703065008));
#49341=CARTESIAN_POINT('Ctrl Pts',(36.4363722249507,4.16087269744914,0.54908913247953));
#49342=CARTESIAN_POINT('Ctrl Pts',(36.435841044003,4.16087513362729,0.422954290450214));
#49343=CARTESIAN_POINT('Ctrl Pts',(36.434589295354,4.16088144845133,0.170871541684232));
#49344=CARTESIAN_POINT('Ctrl Pts',(36.4319292680497,4.16089522631591,-0.26978215410378));
#49345=CARTESIAN_POINT('Ctrl Pts',(36.4269131718644,4.16092325537722,-0.898055013797758));
#49346=CARTESIAN_POINT('Ctrl Pts',(36.4194217572928,4.1609582606988,-1.65043323512625));
#49347=CARTESIAN_POINT('Ctrl Pts',(36.4080166493647,4.16100822936559,-2.6522040911542));
#49348=CARTESIAN_POINT('Ctrl Pts',(36.392266008259,4.16104373891537,-3.90286135663219));
#49349=CARTESIAN_POINT('Ctrl Pts',(36.3803636434912,4.16103146254835,-4.90429019119771));
#49350=CARTESIAN_POINT('Ctrl Pts',(36.3739116299766,4.1609871795194,-5.53120786050771));
#49351=CARTESIAN_POINT('Ctrl Pts',(36.3713606906984,4.16102356994971,-5.78138723335569));
#49352=CARTESIAN_POINT('Ctrl Pts',(36.366345718637,4.16127637656656,-6.28274353426383));
#49353=CARTESIAN_POINT('Ctrl Pts',(36.3577443463334,4.16207694741307,-7.16105813208124));
#49354=CARTESIAN_POINT('Ctrl Pts',(36.3456034160075,4.16363296143633,-8.41833001284824));
#49355=CARTESIAN_POINT('Ctrl Pts',(36.3328233994175,4.16400016903126,-9.67581570986639));
#49356=CARTESIAN_POINT('Ctrl Pts',(36.3230878338691,4.1627189089989,-10.5547256151369));
#49357=CARTESIAN_POINT('Ctrl Pts',(36.3172349488834,4.16141560307,-11.0563995665472));
#49358=CARTESIAN_POINT('Ctrl Pts',(36.3141976241003,4.1605546972218,-11.3069518728839));
#49359=CARTESIAN_POINT('Ctrl Pts',(36.311867463079,4.15981617321664,-11.4957297272532));
#49360=CARTESIAN_POINT('Ctrl Pts',(36.3104545978921,4.15901797692348,-11.628471241393));
#49361=CARTESIAN_POINT('Ctrl Pts',(36.3081772327842,4.15649951043857,-11.8892616158524));
#49362=CARTESIAN_POINT('Ctrl Pts',(36.3054764271753,4.14986400164058,-12.344182579232));
#49363=CARTESIAN_POINT('Ctrl Pts',(36.3039001418369,4.12976492006611,-13.2403168618754));
#49364=CARTESIAN_POINT('Ctrl Pts',(36.3055860448045,4.09306418891023,-14.4874973759583));
#49365=CARTESIAN_POINT('Ctrl Pts',(36.2942146040001,4.07651301036016,-15.5739312984285));
#49366=CARTESIAN_POINT('Ctrl Pts',(36.2740467355084,4.08175161671561,-16.2857592940339));
#49367=CARTESIAN_POINT('Ctrl Pts',(36.2567923498229,4.09007842869138,-16.7572189427173));
#49368=CARTESIAN_POINT('Ctrl Pts',(36.2389427433258,4.10244261181981,-17.1074548236883));
#49369=CARTESIAN_POINT('Ctrl Pts',(36.2208664629216,4.11665826718186,-17.3974452542242));
#49370=CARTESIAN_POINT('Ctrl Pts',(36.2133730769138,4.12288760773508,-17.5193584165972));
#49371=CARTESIAN_POINT('Ctrl Pts',(36.1972619311317,4.13573594543672,-17.7590957322682));
#49372=CARTESIAN_POINT('Ctrl Pts',(36.1794845836868,4.14963289799397,-18.0004187229686));
#49373=CARTESIAN_POINT('Ctrl Pts',(36.1602453247373,4.16435807034453,-18.2410234719111));
#49374=CARTESIAN_POINT('Ctrl Pts',(36.1476322300781,4.17393530170251,-18.3916144026914));
#49375=CARTESIAN_POINT('Ctrl Pts',(36.1372149370081,4.1818007370874,-18.5120405738868));
#49376=CARTESIAN_POINT('Ctrl Pts',(36.1292414811277,4.1878046265628,-18.6023874548805));
#49377=CARTESIAN_POINT('Ctrl Pts',(36.1224677615594,4.1928926133522,-18.677676965247));
#49378=CARTESIAN_POINT('Ctrl Pts',(36.1169744232355,4.19701302310448,-18.7379164308516));
#49379=CARTESIAN_POINT('Ctrl Pts',(36.0698644414276,4.23232318293373,-19.2499674852621));
#49380=CARTESIAN_POINT('Ctrl Pts',(35.9665612554792,4.30865010297181,-20.2294585309346));
#49381=CARTESIAN_POINT('Ctrl Pts',(35.8007022817384,4.44338771065726,-21.6777249613799));
#49382=CARTESIAN_POINT('Ctrl Pts',(35.6985474547797,4.55366109792194,-22.6436070310028));
#49383=CARTESIAN_POINT('Ctrl Pts',(35.6409616397526,4.63295243003527,-23.2440179530984));
#49384=CARTESIAN_POINT('Ctrl Pts',(35.6184001316968,4.66404898478509,-23.4651075012263));
#49385=CARTESIAN_POINT('Ctrl Pts',(35.5714930887105,4.73609875981253,-23.9253851652744));
#49386=CARTESIAN_POINT('Ctrl Pts',(35.4866210875483,4.88180845890605,-24.7451776075493));
#49387=CARTESIAN_POINT('Ctrl Pts',(35.3607305332135,5.13770232629307,-25.9708121318986));
#49388=CARTESIAN_POINT('Ctrl Pts',(35.2142276066228,5.47503752153702,-27.51013784333));
#49389=CARTESIAN_POINT('Ctrl Pts',(35.1287204298902,5.68300225352559,-28.579818117116));
#49390=CARTESIAN_POINT('Ctrl Pts',(35.0878448026781,5.78365285372853,-29.1926592172269));
#49391=CARTESIAN_POINT('Ctrl Pts',(35.0795921412154,5.804619458885,-29.3207592382003));
#49392=CARTESIAN_POINT('Ctrl Pts',(35.0630934440586,5.84649147906714,-29.5812104390111));
#49393=CARTESIAN_POINT('Ctrl Pts',(35.0354683041597,5.91754668256178,-30.0340522643875));
#49394=CARTESIAN_POINT('Ctrl Pts',(34.9841364638804,6.053064873335,-30.9387119821918));
#49395=CARTESIAN_POINT('Ctrl Pts',(34.9215988790561,6.23029214907037,-32.2219964317856));
#49396=CARTESIAN_POINT('Ctrl Pts',(34.8720796920368,6.39500510705853,-33.4942535933966));
#49397=CARTESIAN_POINT('Ctrl Pts',(34.8401758497231,6.52454157318325,-34.5043398338357));
#49398=CARTESIAN_POINT('Ctrl Pts',(34.8267142376718,6.589363786187,-35.0066684959514));
#49399=CARTESIAN_POINT('Ctrl Pts',(34.8175695011411,6.63850023499951,-35.3834627780651));
#49400=CARTESIAN_POINT('Ctrl Pts',(34.8116941048461,6.67171062801112,-35.6396028924226));
#49401=CARTESIAN_POINT('Ctrl Pts',(34.802022989597,6.73752943798291,-36.1488028995589));
#49402=CARTESIAN_POINT('Ctrl Pts',(34.7896756969634,6.85162363355519,-37.0388907733161));
#49403=CARTESIAN_POINT('Ctrl Pts',(34.780419785692,7.07415792333669,-38.8113317003373));
#49404=CARTESIAN_POINT('Ctrl Pts',(34.7885680474133,7.25240420099761,-40.3262000688208));
#49405=CARTESIAN_POINT('Ctrl Pts',(34.7922929384013,7.39024155720927,-41.591498175899));
#49406=CARTESIAN_POINT('Ctrl Pts',(34.7924068356153,7.42924402972164,-41.9789634900419));
#49407=CARTESIAN_POINT('Ctrl Pts',(34.7924493108881,7.47677005399358,-42.4886835116074));
#49408=CARTESIAN_POINT('Ctrl Pts',(34.7924820473252,7.52221413824149,-42.9983713480713));
#49409=CARTESIAN_POINT('Ctrl Pts',(34.7930507774722,7.57594601810967,-43.6322878904797));
#49410=CARTESIAN_POINT('Ctrl Pts',(34.7960381341315,7.63892333195803,-44.3884882496669));
#49411=CARTESIAN_POINT('Ctrl Pts',(34.8017725228489,7.69286318487468,-45.0139962663783));
#49412=CARTESIAN_POINT('Ctrl Pts',(34.8089999595259,7.73851263582959,-45.511382337068));
#49413=CARTESIAN_POINT('Ctrl Pts',(34.8160222362676,7.77439227005541,-45.882785120485));
#49414=CARTESIAN_POINT('Ctrl Pts',(34.824860917934,7.81230831042121,-46.2524957987966));
#49415=CARTESIAN_POINT('Ctrl Pts',(34.8393386173542,7.86608982182046,-46.742960460993));
#49416=CARTESIAN_POINT('Ctrl Pts',(34.8537455518391,7.91061328612196,-47.1080553302964));
#49417=CARTESIAN_POINT('Ctrl Pts',(34.8709410861411,7.95875254430267,-47.4714358673103));
#49418=CARTESIAN_POINT('Ctrl Pts',(34.8839834705516,7.99243680465684,-47.7022779156774));
#49419=CARTESIAN_POINT('Ctrl Pts',(34.9133572479211,8.06898230823606,-48.1772108814288));
#49420=CARTESIAN_POINT('Ctrl Pts',(34.9738217220953,8.22144382015883,-49.0185420321587));
#49421=CARTESIAN_POINT('Ctrl Pts',(35.0820820293093,8.47148089508071,-50.2647952395676));
#49422=CARTESIAN_POINT('Ctrl Pts',(35.2351526769321,8.75014012826034,-51.8333470205335));
#49423=CARTESIAN_POINT('Ctrl Pts',(35.3427326291523,8.86951422265271,-52.9349741093424));
#49424=CARTESIAN_POINT('Ctrl Pts',(35.4078923821326,8.90587288905447,-53.6436700502769));
#49425=CARTESIAN_POINT('Ctrl Pts',(35.4353624911882,8.91551702527776,-53.9526639891302));
#49426=CARTESIAN_POINT('Ctrl Pts',(35.4947913587344,8.91260207054687,-54.5419025239566));
#49427=CARTESIAN_POINT('Ctrl Pts',(35.6072519093414,8.86279590946284,-55.5418424448288));
#49428=CARTESIAN_POINT('Ctrl Pts',(35.8424450750142,8.65493143604865,-57.3800614358869));
#49429=CARTESIAN_POINT('Ctrl Pts',(36.0149308588584,8.5351779208891,-58.6759953288372));
#49430=CARTESIAN_POINT('Ctrl Pts',(36.0809952548126,8.60043152813387,-59.451695379221));
#49431=CARTESIAN_POINT('Ctrl Pts',(36.0885407153967,8.61075055262764,-59.5692306619767));
#49432=CARTESIAN_POINT('Ctrl Pts',(36.1020277936,8.63293407448938,-59.791773774123));
#49433=CARTESIAN_POINT('Ctrl Pts',(36.1215461055886,8.67887213429191,-60.189018935145));
#49434=CARTESIAN_POINT('Ctrl Pts',(36.1459574663463,8.79631439142916,-60.9828849793252));
#49435=CARTESIAN_POINT('Ctrl Pts',(36.1481729065539,8.98695572450133,-61.9000917036662));
#49436=CARTESIAN_POINT('Ctrl Pts',(36.1396454278851,9.22658847892513,-62.8181111290303));
#49437=CARTESIAN_POINT('Ctrl Pts',(36.1335264055312,9.37842901981253,-63.3346872065385));
#49438=CARTESIAN_POINT('Ctrl Pts',(36.1300114391582,9.48621884888992,-63.6785588611986));
#49439=CARTESIAN_POINT('Ctrl Pts',(36.127885752017,9.55979649333591,-63.9076897706352));
#49440=CARTESIAN_POINT('Ctrl Pts',(36.1262122462846,9.63586865333346,-64.1364782842017));
#49441=CARTESIAN_POINT('Ctrl Pts',(36.1253141932307,9.70455338622023,-64.3364143671117));
#49442=CARTESIAN_POINT('Ctrl Pts',(36.124991351822,9.74439272579184,-64.4505712574178));
#49443=CARTESIAN_POINT('Ctrl Pts',(36.1247099153703,9.80472639043459,-64.6216853401157));
#49444=CARTESIAN_POINT('Ctrl Pts',(36.124932073824,9.85621713484614,-64.7640878246856));
#49445=CARTESIAN_POINT('Ctrl Pts',(36.1260402834046,9.94277504210635,-64.9989547811454));
#49446=CARTESIAN_POINT('Ctrl Pts',(36.1273229909198,10.0254902169591,-65.2126141431759));
#49447=CARTESIAN_POINT('Ctrl Pts',(36.1291758847748,10.2137505174887,-65.6617087684228));
#49448=CARTESIAN_POINT('Ctrl Pts',(36.1311833869412,10.5810170945027,-66.4511101943034));
#49449=CARTESIAN_POINT('Ctrl Pts',(36.130738160053,11.4591355370609,-68.0894113511506));
#49450=CARTESIAN_POINT('Ctrl Pts',(36.126345375064,12.3572615261994,-69.5843476939743));
#49451=CARTESIAN_POINT('Ctrl Pts',(36.1249006423819,12.9894425233202,-70.7860628595763));
#49452=CARTESIAN_POINT('Ctrl Pts',(36.1249374217901,13.118205570479,-71.0305629313097));
#49453=CARTESIAN_POINT('Ctrl Pts',(36.1248379255275,13.3834907027566,-71.5330384800975));
#49454=CARTESIAN_POINT('Ctrl Pts',(36.1248501107365,13.7133832691705,-72.1557180082116));
#49455=CARTESIAN_POINT('Ctrl Pts',(36.1248713979155,14.1123888014151,-72.9063590020337));
#49456=CARTESIAN_POINT('Ctrl Pts',(36.1250136146553,14.911861549032,-74.4067848331667));
#49457=CARTESIAN_POINT('Ctrl Pts',(36.1252094628775,15.5818687416089,-75.6597056091058));
#49458=CARTESIAN_POINT('Ctrl Pts',(36.1251645924201,16.5536865502446,-77.4872413901607));
#49459=CARTESIAN_POINT('Ctrl Pts',(36.1251960907172,16.9893579083434,-78.306521149624));
#49460=CARTESIAN_POINT('Ctrl Pts',(36.1251960907173,17.4258794957329,-79.1274988517223));
#49461=CARTESIAN_POINT('Ctrl Pts',(37.9743793938247,4.21863409729416,24.8306267144035));
#49462=CARTESIAN_POINT('Ctrl Pts',(37.974492258943,4.21863841245639,24.78174714051));
#49463=CARTESIAN_POINT('Ctrl Pts',(37.9746106306985,4.21864293872577,24.7328686303977));
#49464=CARTESIAN_POINT('Ctrl Pts',(37.9760083865885,4.21869637434015,24.1822570212595));
#49465=CARTESIAN_POINT('Ctrl Pts',(37.9770915843225,4.21873200165046,23.178111074583));
#49466=CARTESIAN_POINT('Ctrl Pts',(37.9796217625982,4.21881175633108,21.1695081088091));
#49467=CARTESIAN_POINT('Ctrl Pts',(37.9889227535691,4.21916723227851,19.6653538966312));
#49468=CARTESIAN_POINT('Ctrl Pts',(38.0085894948983,4.21994781539465,18.4143063459505));
#49469=CARTESIAN_POINT('Ctrl Pts',(38.0180268333167,4.22031950377046,17.9114656680587));
#49470=CARTESIAN_POINT('Ctrl Pts',(38.0417338295989,4.22124783985785,16.9074551401735));
#49471=CARTESIAN_POINT('Ctrl Pts',(38.0925813872245,4.22323994665397,15.1536342494888));
#49472=CARTESIAN_POINT('Ctrl Pts',(38.1408117825693,4.22516867420997,13.6519382550817));
#49473=CARTESIAN_POINT('Ctrl Pts',(38.1709079604311,4.22644869451557,12.3975578235691));
#49474=CARTESIAN_POINT('Ctrl Pts',(38.1831964689025,4.22698016482334,11.8966405663243));
#49475=CARTESIAN_POINT('Ctrl Pts',(38.2082001178775,4.2280900923784,10.89484911608));
#49476=CARTESIAN_POINT('Ctrl Pts',(38.2390387632422,4.22949823370161,9.64233663567765));
#49477=CARTESIAN_POINT('Ctrl Pts',(38.2714937740577,4.23102035728818,8.13782020555378));
#49478=CARTESIAN_POINT('Ctrl Pts',(38.2875020804209,4.23178261123858,7.13305418257719));
#49479=CARTESIAN_POINT('Ctrl Pts',(38.2949304559688,4.23213921574379,6.50504097441828));
#49480=CARTESIAN_POINT('Ctrl Pts',(38.2976902518413,4.23227629394518,6.25486333187328));
#49481=CARTESIAN_POINT('Ctrl Pts',(38.3024566847348,4.23252931044664,5.75379505782952));
#49482=CARTESIAN_POINT('Ctrl Pts',(38.3089192082696,4.23291193377536,4.87544297152401));
#49483=CARTESIAN_POINT('Ctrl Pts',(38.3151336323395,4.23342810905955,3.11513770009187));
#49484=CARTESIAN_POINT('Ctrl Pts',(38.3116765402784,4.23335441307545,1.60808221958763));
#49485=CARTESIAN_POINT('Ctrl Pts',(38.3076705606032,4.23301392086635,0.548265115589204));
#49486=CARTESIAN_POINT('Ctrl Pts',(38.3071452992699,4.23296996296405,0.422036119001589));
#49487=CARTESIAN_POINT('Ctrl Pts',(38.3059091966356,4.23286482875268,0.169788232924755));
#49488=CARTESIAN_POINT('Ctrl Pts',(38.3032833893307,4.23263987593515,-0.271134839049098));
#49489=CARTESIAN_POINT('Ctrl Pts',(38.2983399003467,4.23220915338293,-0.899734170126479));
#49490=CARTESIAN_POINT('Ctrl Pts',(38.2909381042811,4.23157615514907,-1.65235304049793));
#49491=CARTESIAN_POINT('Ctrl Pts',(38.279665745071,4.23061740452919,-2.65432268665193));
#49492=CARTESIAN_POINT('Ctrl Pts',(38.2640282182585,4.22933803030512,-3.90490507972187));
#49493=CARTESIAN_POINT('Ctrl Pts',(38.2521329820479,4.22844215333868,-4.90599788327314));
#49494=CARTESIAN_POINT('Ctrl Pts',(38.2456115546156,4.22801160713605,-5.53266954474732));
#49495=CARTESIAN_POINT('Ctrl Pts',(38.2432139048281,4.22773560300612,-5.78506890425695));
#49496=CARTESIAN_POINT('Ctrl Pts',(38.2391023217651,4.22684064921901,-6.28876410275137));
#49497=CARTESIAN_POINT('Ctrl Pts',(38.2332760101616,4.22458816124566,-7.17007490241801));
#49498=CARTESIAN_POINT('Ctrl Pts',(38.226456056922,4.22056665615865,-8.42601796915756));
#49499=CARTESIAN_POINT('Ctrl Pts',(38.2151634607775,4.21878579347824,-9.67536092665477));
#49500=CARTESIAN_POINT('Ctrl Pts',(38.201510169486,4.22046816872256,-10.5446395981229));
#49501=CARTESIAN_POINT('Ctrl Pts',(38.1915776224637,4.22250384649015,-11.0397541416357));
#49502=CARTESIAN_POINT('Ctrl Pts',(38.1858209942656,4.22391321247,-11.2866020505556));
#49503=CARTESIAN_POINT('Ctrl Pts',(38.1811561945481,4.22513990252829,-11.4725955114208));
#49504=CARTESIAN_POINT('Ctrl Pts',(38.1781231817478,4.2256673507536,-11.6084095583563));
#49505=CARTESIAN_POINT('Ctrl Pts',(38.172416962679,4.22535403168541,-11.8719247327729));
#49506=CARTESIAN_POINT('Ctrl Pts',(38.1632101925206,4.22178743142648,-12.3315588082072));
#49507=CARTESIAN_POINT('Ctrl Pts',(38.1466521359241,4.20573495068469,-13.2300179665428));
#49508=CARTESIAN_POINT('Ctrl Pts',(38.1208998504696,4.17589084567263,-14.4631736218846));
#49509=CARTESIAN_POINT('Ctrl Pts',(38.0783845247824,4.17896862737656,-15.5157856111138));
#49510=CARTESIAN_POINT('Ctrl Pts',(38.0351280575023,4.20667903991865,-16.1974410314374));
#49511=CARTESIAN_POINT('Ctrl Pts',(38.0018870091212,4.23260587197108,-16.6468058390751));
#49512=CARTESIAN_POINT('Ctrl Pts',(37.9715402958889,4.26115653272591,-16.9784979407005));
#49513=CARTESIAN_POINT('Ctrl Pts',(37.9428822522154,4.29068437333013,-17.2519506004831));
#49514=CARTESIAN_POINT('Ctrl Pts',(37.9309121166235,4.30320748052913,-17.3618749444117));
#49515=CARTESIAN_POINT('Ctrl Pts',(37.9047576019355,4.33028450196241,-17.5826112593404));
#49516=CARTESIAN_POINT('Ctrl Pts',(37.8755045401449,4.3604750146577,-17.8060117972872));
#49517=CARTESIAN_POINT('Ctrl Pts',(37.843661785628,4.39334406374891,-18.031718943508));
#49518=CARTESIAN_POINT('Ctrl Pts',(37.8227909946016,4.41493560327634,-18.1738267243772));
#49519=CARTESIAN_POINT('Ctrl Pts',(37.8055778985813,4.43279175427115,-18.2881138433063));
#49520=CARTESIAN_POINT('Ctrl Pts',(37.7924268084728,4.44646428185898,-18.3741363191589));
#49521=CARTESIAN_POINT('Ctrl Pts',(37.7812809907889,4.45808321172109,-18.4460723317931));
#49522=CARTESIAN_POINT('Ctrl Pts',(37.7722595951433,4.46750766486995,-18.5037759979881));
#49523=CARTESIAN_POINT('Ctrl Pts',(37.695022708878,4.54835904189559,-18.9950878850114));
#49524=CARTESIAN_POINT('Ctrl Pts',(37.5305819780222,4.72434670681134,-19.9610964749048));
#49525=CARTESIAN_POINT('Ctrl Pts',(37.3051029479327,5.01823596921909,-21.4586235781379));
#49526=CARTESIAN_POINT('Ctrl Pts',(37.1955939026535,5.23122815130101,-22.4917581243808));
#49527=CARTESIAN_POINT('Ctrl Pts',(37.1455073222649,5.36711897314608,-23.1435640254773));
#49528=CARTESIAN_POINT('Ctrl Pts',(37.1296059114069,5.41770838498506,-23.3745708513876));
#49529=CARTESIAN_POINT('Ctrl Pts',(37.0991677184359,5.53041814804529,-23.8572987491716));
#49530=CARTESIAN_POINT('Ctrl Pts',(37.0535693526703,5.74525965546662,-24.7061348664269));
#49531=CARTESIAN_POINT('Ctrl Pts',(37.0012890967258,6.09156617222418,-25.9554051399712));
#49532=CARTESIAN_POINT('Ctrl Pts',(36.9473976697968,6.51348748988546,-27.499250671943));
#49533=CARTESIAN_POINT('Ctrl Pts',(36.9133313107658,6.76467422120613,-28.5625661281727));
#49534=CARTESIAN_POINT('Ctrl Pts',(36.8939524645289,6.88631594558857,-29.1702997742256));
#49535=CARTESIAN_POINT('Ctrl Pts',(36.8901953539948,6.91224581145836,-29.3008098254207));
#49536=CARTESIAN_POINT('Ctrl Pts',(36.8827996560842,6.96324100593501,-29.5639684519698));
#49537=CARTESIAN_POINT('Ctrl Pts',(36.8709931285117,7.04906085338863,-30.0222918894149));
#49538=CARTESIAN_POINT('Ctrl Pts',(36.851060722126,7.20889062551895,-30.9359618354406));
#49539=CARTESIAN_POINT('Ctrl Pts',(36.8328740793196,7.40877289976207,-32.2289515952689));
#49540=CARTESIAN_POINT('Ctrl Pts',(36.8263100628016,7.5850490148669,-33.5044476393165));
#49541=CARTESIAN_POINT('Ctrl Pts',(36.8265592325707,7.71975151448663,-34.5125815020699));
#49542=CARTESIAN_POINT('Ctrl Pts',(36.8284007726567,7.78649502690822,-35.0123003094323));
#49543=CARTESIAN_POINT('Ctrl Pts',(36.8302422030198,7.83687505870679,-35.3865350342881));
#49544=CARTESIAN_POINT('Ctrl Pts',(36.8315120391773,7.87101044252364,-35.6440496199976));
#49545=CARTESIAN_POINT('Ctrl Pts',(36.8358568082861,7.93751800985704,-36.1542445699149));
#49546=CARTESIAN_POINT('Ctrl Pts',(36.847237669633,8.05062893861643,-37.0470229512314));
#49547=CARTESIAN_POINT('Ctrl Pts',(36.8824480260088,8.26236414082339,-38.8243606250119));
#49548=CARTESIAN_POINT('Ctrl Pts',(36.9234642151751,8.41889131363091,-40.3443424816412));
#49549=CARTESIAN_POINT('Ctrl Pts',(36.9517860700139,8.53484591648929,-41.614030993031));
#49550=CARTESIAN_POINT('Ctrl Pts',(36.9592376200307,8.56764734381142,-41.9992090889243));
#49551=CARTESIAN_POINT('Ctrl Pts',(36.9683476045283,8.60760114210068,-42.50904350848));
#49552=CARTESIAN_POINT('Ctrl Pts',(36.9770403748266,8.6454975835139,-43.0191781457652));
#49553=CARTESIAN_POINT('Ctrl Pts',(36.9876403346379,8.68944332364214,-43.655405806571));
#49554=CARTESIAN_POINT('Ctrl Pts',(37.0013381840815,8.73840883574967,-44.4167461203277));
#49555=CARTESIAN_POINT('Ctrl Pts',(37.0147952319846,8.77741565667612,-45.0486963300423));
#49556=CARTESIAN_POINT('Ctrl Pts',(37.027632614232,8.80842154980143,-45.5525006513341));
#49557=CARTESIAN_POINT('Ctrl Pts',(37.038440488472,8.83172909652937,-45.929386688973));
#49558=CARTESIAN_POINT('Ctrl Pts',(37.0506250140234,8.85528687507259,-46.3052579784331));
#49559=CARTESIAN_POINT('Ctrl Pts',(37.0690074575453,8.88730474900626,-46.8048669254791));
#49560=CARTESIAN_POINT('Ctrl Pts',(37.0853542896548,8.91217988455291,-47.1779259422816));
#49561=CARTESIAN_POINT('Ctrl Pts',(37.1040005222447,8.93812390306473,-47.5500917536217));
#49562=CARTESIAN_POINT('Ctrl Pts',(37.1174893861852,8.95620812618262,-47.7877040574019));
#49563=CARTESIAN_POINT('Ctrl Pts',(37.1471749698849,8.99716486633686,-48.2747490401855));
#49564=CARTESIAN_POINT('Ctrl Pts',(37.2056971608678,9.07764006184513,-49.135329879993));
#49565=CARTESIAN_POINT('Ctrl Pts',(37.3028492188309,9.20328040460516,-50.4016484218929));
#49566=CARTESIAN_POINT('Ctrl Pts',(37.426850198214,9.32122267562777,-51.9762540942031));
#49567=CARTESIAN_POINT('Ctrl Pts',(37.5047710024866,9.34257078545175,-53.0651446979514));
#49568=CARTESIAN_POINT('Ctrl Pts',(37.5493822799248,9.32608751006771,-53.7605712583107));
#49569=CARTESIAN_POINT('Ctrl Pts',(37.5681824068605,9.3119219865871,-54.0737087055534));
#49570=CARTESIAN_POINT('Ctrl Pts',(37.6069862512297,9.26334418068316,-54.6630166434402));
#49571=CARTESIAN_POINT('Ctrl Pts',(37.6770765329605,9.13669869620959,-55.6608709574235));
#49572=CARTESIAN_POINT('Ctrl Pts',(37.8159387231878,8.79827935854848,-57.4834792507308));
#49573=CARTESIAN_POINT('Ctrl Pts',(37.913486645184,8.62006744396071,-58.7608746719867));
#49574=CARTESIAN_POINT('Ctrl Pts',(37.9535058005589,8.6630413573171,-59.5032113087664));
#49575=CARTESIAN_POINT('Ctrl Pts',(37.9580719704498,8.67021106909296,-59.6160263902128));
#49576=CARTESIAN_POINT('Ctrl Pts',(37.9662511317454,8.6870295365958,-59.8299975680421));
#49577=CARTESIAN_POINT('Ctrl Pts',(37.9781030159931,8.72491997924004,-60.2131778620392));
#49578=CARTESIAN_POINT('Ctrl Pts',(37.9929764021785,8.83200747034294,-60.9839274746279));
#49579=CARTESIAN_POINT('Ctrl Pts',(37.9943767493591,9.0221597655985,-61.8859344504134));
#49580=CARTESIAN_POINT('Ctrl Pts',(37.9893344013422,9.26865925501439,-62.7991904173723));
#49581=CARTESIAN_POINT('Ctrl Pts',(37.9857174720035,9.42598099805474,-63.3166639671887));
#49582=CARTESIAN_POINT('Ctrl Pts',(37.9836469546191,9.53759795275649,-63.6625454370981));
#49583=CARTESIAN_POINT('Ctrl Pts',(37.9824006145624,9.61372962915768,-63.8933931853993));
#49584=CARTESIAN_POINT('Ctrl Pts',(37.9814213750252,9.69231282634275,-64.1244361994236));
#49585=CARTESIAN_POINT('Ctrl Pts',(37.9809106222791,9.76304704436886,-64.326833963689));
#49586=CARTESIAN_POINT('Ctrl Pts',(37.9807337431088,9.80400196055581,-64.442535573146));
#49587=CARTESIAN_POINT('Ctrl Pts',(37.9805919097837,9.86594338959743,-64.6161004856718));
#49588=CARTESIAN_POINT('Ctrl Pts',(37.9807463369306,9.91863581785843,-64.7608413565679));
#49589=CARTESIAN_POINT('Ctrl Pts',(37.9814622524679,10.006859705651,-64.9998595182745));
#49590=CARTESIAN_POINT('Ctrl Pts',(37.9826301558853,10.0892520642219,-65.2123223473177));
#49591=CARTESIAN_POINT('Ctrl Pts',(37.984346930264,10.2780325969123,-65.6621174689531));
#49592=CARTESIAN_POINT('Ctrl Pts',(37.986642528923,10.6456486560468,-66.4511350626474));
#49593=CARTESIAN_POINT('Ctrl Pts',(37.9879108841636,11.524912009961,-68.0899328486106));
#49594=CARTESIAN_POINT('Ctrl Pts',(37.985066779144,12.4235874158634,-69.5844828536149));
#49595=CARTESIAN_POINT('Ctrl Pts',(37.9833104983342,13.056073118225,-70.7862662061612));
#49596=CARTESIAN_POINT('Ctrl Pts',(37.9834152527383,13.1849143669782,-71.0308187122585));
#49597=CARTESIAN_POINT('Ctrl Pts',(37.9833545435611,13.4503155154178,-71.5333720275582));
#49598=CARTESIAN_POINT('Ctrl Pts',(37.983414746917,13.7803064517032,-72.1561248389429));
#49599=CARTESIAN_POINT('Ctrl Pts',(37.9834440827621,14.1793606209594,-72.9068371922368));
#49600=CARTESIAN_POINT('Ctrl Pts',(37.983560394376,14.9788300444199,-74.4073549057964));
#49601=CARTESIAN_POINT('Ctrl Pts',(37.9836464209878,15.6486817082044,-75.6601782849562));
#49602=CARTESIAN_POINT('Ctrl Pts',(37.9835707570307,16.6204131422508,-77.487514078272));
#49603=CARTESIAN_POINT('Ctrl Pts',(37.9836041227838,17.0561121018744,-78.3068237760512));
#49604=CARTESIAN_POINT('Ctrl Pts',(37.9836041227839,17.4926336892639,-79.1278014781496));
#49605=CARTESIAN_POINT('Ctrl Pts',(39.8297890978139,4.30089180200322,24.8306033519864));
#49606=CARTESIAN_POINT('Ctrl Pts',(39.8299074020901,4.30089711404966,24.7817230525328));
#49607=CARTESIAN_POINT('Ctrl Pts',(39.830031479274,4.3009026866052,24.7328438116444));
#49608=CARTESIAN_POINT('Ctrl Pts',(39.8314965764819,4.30096848600841,24.1822234222506));
#49609=CARTESIAN_POINT('Ctrl Pts',(39.8326291542074,4.30100164232867,23.1780643674514));
#49610=CARTESIAN_POINT('Ctrl Pts',(39.8352733292624,4.30106760982009,21.1694460455231));
#49611=CARTESIAN_POINT('Ctrl Pts',(39.8450224013784,4.3015063259998,19.6652841373055));
#49612=CARTESIAN_POINT('Ctrl Pts',(39.8656503854775,4.30252264560954,18.4142343890651));
#49613=CARTESIAN_POINT('Ctrl Pts',(39.8755468785802,4.30300312909193,17.911351654955));
#49614=CARTESIAN_POINT('Ctrl Pts',(39.9004034153351,4.30419822099428,16.9073098440472));
#49615=CARTESIAN_POINT('Ctrl Pts',(39.953716293508,4.30676554786842,15.153489091752));
#49616=CARTESIAN_POINT('Ctrl Pts',(40.0043125451533,4.30931090977232,13.6519156262175));
#49617=CARTESIAN_POINT('Ctrl Pts',(40.0359355901385,4.31109503698416,12.3977077797573));
#49618=CARTESIAN_POINT('Ctrl Pts',(40.0488540424933,4.31184611138178,11.896861536915));
#49619=CARTESIAN_POINT('Ctrl Pts',(40.0751597988642,4.31344670334409,10.8951765808069));
#49620=CARTESIAN_POINT('Ctrl Pts',(40.1076330240833,4.31553018183121,9.64272890374985));
#49621=CARTESIAN_POINT('Ctrl Pts',(40.1418302072307,4.31782592199948,8.13819823380099));
#49622=CARTESIAN_POINT('Ctrl Pts',(40.158699490557,4.31899908471942,7.13334121701694));
#49623=CARTESIAN_POINT('Ctrl Pts',(40.1665241376599,4.31954936256452,6.5052603902337));
#49624=CARTESIAN_POINT('Ctrl Pts',(40.1694302788948,4.31976414814769,6.2551379681381));
#49625=CARTESIAN_POINT('Ctrl Pts',(40.174446373827,4.3201742172438,5.7541147994796));
#49626=CARTESIAN_POINT('Ctrl Pts',(40.1812395059384,4.32083073673609,4.87581090564104));
#49627=CARTESIAN_POINT('Ctrl Pts',(40.1877539016281,4.32182649441906,3.11541238522877));
#49628=CARTESIAN_POINT('Ctrl Pts',(40.1841301313211,4.32187206126619,1.60788760759156));
#49629=CARTESIAN_POINT('Ctrl Pts',(40.180007725456,4.3212798572179,0.547615075927073));
#49630=CARTESIAN_POINT('Ctrl Pts',(40.1794671788892,4.32120140318382,0.421323426395065));
#49631=CARTESIAN_POINT('Ctrl Pts',(40.1781932213731,4.32101446375644,0.168961732958732));
#49632=CARTESIAN_POINT('Ctrl Pts',(40.1754837625236,4.32061298834142,-0.272146661512237));
#49633=CARTESIAN_POINT('Ctrl Pts',(40.1703722396646,4.31985173574526,-0.900986822677657));
#49634=CARTESIAN_POINT('Ctrl Pts',(40.1627145970043,4.31872192159838,-1.65378076716345));
#49635=CARTESIAN_POINT('Ctrl Pts',(40.1510375361638,4.31703143200427,-2.65592708254926));
#49636=CARTESIAN_POINT('Ctrl Pts',(40.1348310495129,4.3147720923205,-3.90653507224137));
#49637=CARTESIAN_POINT('Ctrl Pts',(40.1224731624672,4.31322379578241,-4.90747430946853));
#49638=CARTESIAN_POINT('Ctrl Pts',(40.1156951883021,4.31246287247062,-5.53414030084685));
#49639=CARTESIAN_POINT('Ctrl Pts',(40.1134265827715,4.31174306157199,-5.79061969698076));
#49640=CARTESIAN_POINT('Ctrl Pts',(40.1103207508345,4.30897225982735,-6.29871002733814));
#49641=CARTESIAN_POINT('Ctrl Pts',(40.107764830051,4.30145627816816,-7.18564143430966));
#49642=CARTESIAN_POINT('Ctrl Pts',(40.1073129445978,4.28775474082735,-8.43927035199998));
#49643=CARTESIAN_POINT('Ctrl Pts',(40.0977448736392,4.28253710202282,-9.67381183084355));
#49644=CARTESIAN_POINT('Ctrl Pts',(40.0792095436937,4.28966756715249,-10.5256145598245));
#49645=CARTESIAN_POINT('Ctrl Pts',(40.0642320282913,4.29763772232685,-11.0088039007234));
#49646=CARTESIAN_POINT('Ctrl Pts',(40.0551153157523,4.30304169912288,-11.2489656079416));
#49647=CARTESIAN_POINT('Ctrl Pts',(40.0475753584296,4.30770081209947,-11.4298114982365));
#49648=CARTESIAN_POINT('Ctrl Pts',(40.0424649739259,4.31079842987331,-11.5667670080804));
#49649=CARTESIAN_POINT('Ctrl Pts',(40.0321283015705,4.31535000812646,-11.8295432782458));
#49650=CARTESIAN_POINT('Ctrl Pts',(40.0136236246797,4.32023439713232,-12.2882344186287));
#49651=CARTESIAN_POINT('Ctrl Pts',(39.9742697126271,4.32108683590219,-13.1798275768615));
#49652=CARTESIAN_POINT('Ctrl Pts',(39.9075680371124,4.32104910385571,-14.3935305465639));
#49653=CARTESIAN_POINT('Ctrl Pts',(39.8245515951701,4.36404624239605,-15.4144192264781));
#49654=CARTESIAN_POINT('Ctrl Pts',(39.7569601952596,4.42364867697426,-16.0701224672648));
#49655=CARTESIAN_POINT('Ctrl Pts',(39.7087610954069,4.4723153808393,-16.5012837962032));
#49656=CARTESIAN_POINT('Ctrl Pts',(39.6690529117656,4.51981795229302,-16.8187798291709));
#49657=CARTESIAN_POINT('Ctrl Pts',(39.6342883707279,4.56646918211518,-17.0802410219354));
#49658=CARTESIAN_POINT('Ctrl Pts',(39.6199984966607,4.58472515057873,-17.1762538452768));
#49659=CARTESIAN_POINT('Ctrl Pts',(39.5889265892873,4.62599416228208,-17.3771298804896));
#49660=CARTESIAN_POINT('Ctrl Pts',(39.554651239453,4.67288333425478,-17.5819569012756));
#49661=CARTESIAN_POINT('Ctrl Pts',(39.517836729212,4.72543655859869,-17.7935001323825));
#49662=CARTESIAN_POINT('Ctrl Pts',(39.4939152441966,4.76046599000218,-17.9278381161626));
#49663=CARTESIAN_POINT('Ctrl Pts',(39.4743069681511,4.78977534427916,-18.0367841617068));
#49664=CARTESIAN_POINT('Ctrl Pts',(39.4593852950562,4.81237727141882,-18.1191591592661));
#49665=CARTESIAN_POINT('Ctrl Pts',(39.4467851989995,4.83171899173353,-18.1883791438491));
#49666=CARTESIAN_POINT('Ctrl Pts',(39.4366168539807,4.84748950267596,-18.2440920040423));
#49667=CARTESIAN_POINT('Ctrl Pts',(39.3496791578271,4.98316553995294,-18.7195275406655));
#49668=CARTESIAN_POINT('Ctrl Pts',(39.1696125978185,5.29476671855043,-19.6872826769249));
#49669=CARTESIAN_POINT('Ctrl Pts',(38.9254391201082,5.8260446390497,-21.2538055525673));
#49670=CARTESIAN_POINT('Ctrl Pts',(38.8091730810157,6.16624702587357,-22.3689791879353));
#49671=CARTESIAN_POINT('Ctrl Pts',(38.7609438346582,6.35633355146274,-23.0827727912001));
#49672=CARTESIAN_POINT('Ctrl Pts',(38.7488279482753,6.42508837087025,-23.329659703437));
#49673=CARTESIAN_POINT('Ctrl Pts',(38.7278858800121,6.5693101036196,-23.8434439852938));
#49674=CARTESIAN_POINT('Ctrl Pts',(38.7073568571337,6.82482364374566,-24.7329543374407));
#49675=CARTESIAN_POINT('Ctrl Pts',(38.7112017822482,7.19631750331981,-26.0144237229354));
#49676=CARTESIAN_POINT('Ctrl Pts',(38.7502041664417,7.61697021007329,-27.5653952969295));
#49677=CARTESIAN_POINT('Ctrl Pts',(38.7794787848461,7.85707833808124,-28.6136653389407));
#49678=CARTESIAN_POINT('Ctrl Pts',(38.7890382182912,7.97473470366522,-29.2064710004707));
#49679=CARTESIAN_POINT('Ctrl Pts',(38.7909034054849,8.00090786122559,-29.3403315551717));
#49680=CARTESIAN_POINT('Ctrl Pts',(38.7953101761858,8.0511770518412,-29.606341355115));
#49681=CARTESIAN_POINT('Ctrl Pts',(38.8041101311858,8.13469272707989,-30.0712812851529));
#49682=CARTESIAN_POINT('Ctrl Pts',(38.8262952957626,8.28461802010922,-30.9955386075008));
#49683=CARTESIAN_POINT('Ctrl Pts',(38.8690901302992,8.45752449381605,-32.2998439063812));
#49684=CARTESIAN_POINT('Ctrl Pts',(38.9213026202173,8.59554440185858,-33.5769673036543));
#49685=CARTESIAN_POINT('Ctrl Pts',(38.9649646296608,8.69785473195649,-34.5798586006522));
#49686=CARTESIAN_POINT('Ctrl Pts',(38.9867947953882,8.74832837595039,-35.0744900763109));
#49687=CARTESIAN_POINT('Ctrl Pts',(39.0029788553092,8.7869259048607,-35.4441031748303));
#49688=CARTESIAN_POINT('Ctrl Pts',(39.0137851816264,8.81332284709096,-35.7023542144892));
#49689=CARTESIAN_POINT('Ctrl Pts',(39.0363669701529,8.86363270877695,-36.2118091976656));
#49690=CARTESIAN_POINT('Ctrl Pts',(39.0775623106058,8.94696765931663,-37.1041976637785));
#49691=CARTESIAN_POINT('Ctrl Pts',(39.1642231201606,9.09472486839895,-38.8796940426679));
#49692=CARTESIAN_POINT('Ctrl Pts',(39.2358830961913,9.19261049889707,-40.3979192073547));
#49693=CARTESIAN_POINT('Ctrl Pts',(39.2832491197789,9.26213510924688,-41.6660593258461));
#49694=CARTESIAN_POINT('Ctrl Pts',(39.2963609311839,9.28162753281898,-42.0486332010792));
#49695=CARTESIAN_POINT('Ctrl Pts',(39.3122407852406,9.30498530969422,-42.5567449806013));
#49696=CARTESIAN_POINT('Ctrl Pts',(39.3272012842619,9.32679323766449,-43.0652703573797));
#49697=CARTESIAN_POINT('Ctrl Pts',(39.3444391257118,9.3513141849052,-43.7003677520274));
#49698=CARTESIAN_POINT('Ctrl Pts',(39.3636542466282,9.37707891605137,-44.4615057370672));
#49699=CARTESIAN_POINT('Ctrl Pts',(39.3791663659872,9.39605873195574,-45.0943593321814));
#49700=CARTESIAN_POINT('Ctrl Pts',(39.3916724839035,9.41007620651285,-45.5995359708631));
#49701=CARTESIAN_POINT('Ctrl Pts',(39.4012261438507,9.42009333262994,-45.9777897987432));
#49702=CARTESIAN_POINT('Ctrl Pts',(39.4110598971786,9.42969807933419,-46.3553745961967));
#49703=CARTESIAN_POINT('Ctrl Pts',(39.4246721994116,9.4420605604787,-46.8577539520659));
#49704=CARTESIAN_POINT('Ctrl Pts',(39.4356599382094,9.45097650435408,-47.2334521355618));
#49705=CARTESIAN_POINT('Ctrl Pts',(39.4473515344133,9.45982361763867,-47.6087025243231));
#49706=CARTESIAN_POINT('Ctrl Pts',(39.455337067446,9.4663017968158,-47.8489229908066));
#49707=CARTESIAN_POINT('Ctrl Pts',(39.4718790872392,9.48214615291164,-48.3402938738331));
#49708=CARTESIAN_POINT('Ctrl Pts',(39.5020923450511,9.51513391225086,-49.2072285291987));
#49709=CARTESIAN_POINT('Ctrl Pts',(39.5475557172048,9.56722915901666,-50.4780205381822));
#49710=CARTESIAN_POINT('Ctrl Pts',(39.6016890568396,9.60042591580183,-52.0487581356094));
#49711=CARTESIAN_POINT('Ctrl Pts',(39.6347305365777,9.57525937165125,-53.1273923993307));
#49712=CARTESIAN_POINT('Ctrl Pts',(39.6535137749267,9.53479531567369,-53.8138129076782));
#49713=CARTESIAN_POINT('Ctrl Pts',(39.661169940129,9.51015686831468,-54.1263920717817));
#49714=CARTESIAN_POINT('Ctrl Pts',(39.6764625795126,9.44253409843686,-54.7125978515887));
#49715=CARTESIAN_POINT('Ctrl Pts',(39.7028639675253,9.28571205301212,-55.7058062339899));
#49716=CARTESIAN_POINT('Ctrl Pts',(39.7530011338049,8.89889291572278,-57.5194444827078));
#49717=CARTESIAN_POINT('Ctrl Pts',(39.7835032645467,8.69962611761777,-58.7903065084076));
#49718=CARTESIAN_POINT('Ctrl Pts',(39.8000150983343,8.73424237255801,-59.5232704936248));
#49719=CARTESIAN_POINT('Ctrl Pts',(39.8019222250902,8.74013864044067,-59.6338670314763));
#49720=CARTESIAN_POINT('Ctrl Pts',(39.8055094403312,8.75489037257384,-59.8442120746572));
#49721=CARTESIAN_POINT('Ctrl Pts',(39.8111544726665,8.78982528331435,-60.2212344718915));
#49722=CARTESIAN_POINT('Ctrl Pts',(39.8201591891876,8.89384559283988,-60.9820397452859));
#49723=CARTESIAN_POINT('Ctrl Pts',(39.8261140542061,9.08579366933095,-61.8776392676396));
#49724=CARTESIAN_POINT('Ctrl Pts',(39.829586958919,9.33715620879876,-62.7891644282645));
#49725=CARTESIAN_POINT('Ctrl Pts',(39.8310001436177,9.49778490900772,-63.3072282738974));
#49726=CARTESIAN_POINT('Ctrl Pts',(39.8318821730951,9.61161725883178,-63.6541416261478));
#49727=CARTESIAN_POINT('Ctrl Pts',(39.8324646653385,9.68921063017446,-63.8858427380399));
#49728=CARTESIAN_POINT('Ctrl Pts',(39.833062788756,9.76920095439907,-64.1179849789079));
#49729=CARTESIAN_POINT('Ctrl Pts',(39.8336228250072,9.84108231145926,-64.3215618361683));
#49730=CARTESIAN_POINT('Ctrl Pts',(39.8339584908655,9.88266127202547,-64.4379995134357));
#49731=CARTESIAN_POINT('Ctrl Pts',(39.8344801499524,9.94550363394761,-64.6127287338887));
#49732=CARTESIAN_POINT('Ctrl Pts',(39.8349578956891,9.99886501999364,-64.758571954533));
#49733=CARTESIAN_POINT('Ctrl Pts',(39.8358402435902,10.0880420096664,-64.9995450483702));
#49734=CARTESIAN_POINT('Ctrl Pts',(39.8373877044086,10.1705358382447,-65.2116971529894));
#49735=CARTESIAN_POINT('Ctrl Pts',(39.8397091263091,10.359927845254,-65.6621240062535));
#49736=CARTESIAN_POINT('Ctrl Pts',(39.8430289812638,10.7281424458995,-66.4514330159084));
#49737=CARTESIAN_POINT('Ctrl Pts',(39.8457928929032,11.6080654311873,-68.0909050412643));
#49738=CARTESIAN_POINT('Ctrl Pts',(39.8432888149172,12.5062750279481,-69.5851588058513));
#49739=CARTESIAN_POINT('Ctrl Pts',(39.841321185353,13.1386526418442,-70.7865926005885));
#49740=CARTESIAN_POINT('Ctrl Pts',(39.8415070828448,13.2675448732065,-71.0311925039694));
#49741=CARTESIAN_POINT('Ctrl Pts',(39.8415070337952,13.5329907597079,-71.5337671071248));
#49742=CARTESIAN_POINT('Ctrl Pts',(39.8416367901604,13.8630247881417,-72.1565594092134));
#49743=CARTESIAN_POINT('Ctrl Pts',(39.8416800538061,14.262096492683,-72.9073007263981));
#49744=CARTESIAN_POINT('Ctrl Pts',(39.8417621362322,15.0615590344823,-74.4078623733623));
#49745=CARTESIAN_POINT('Ctrl Pts',(39.841731405234,15.7313091343584,-75.6606358759336));
#49746=CARTESIAN_POINT('Ctrl Pts',(39.8416414731529,16.7029833477083,-77.4878768425244));
#49747=CARTESIAN_POINT('Ctrl Pts',(39.8416862517014,17.138686967236,-78.3071986448441));
#49748=CARTESIAN_POINT('Ctrl Pts',(39.8416862517014,17.5752085546255,-79.1281763469426));
#49749=CARTESIAN_POINT('Ctrl Pts',(42.1495473044919,4.43306139937208,24.8306020121279));
#49750=CARTESIAN_POINT('Ctrl Pts',(42.1496711288007,4.43306863677417,24.7817216606101));
#49751=CARTESIAN_POINT('Ctrl Pts',(42.1498009969792,4.43307622975196,24.7328423838449));
#49752=CARTESIAN_POINT('Ctrl Pts',(42.1513345113838,4.43316584953248,24.1822208256038));
#49753=CARTESIAN_POINT('Ctrl Pts',(42.1524899114227,4.43321285195566,23.1780525968573));
#49754=CARTESIAN_POINT('Ctrl Pts',(42.155167291499,4.43330892962013,21.1694346333917));
#49755=CARTESIAN_POINT('Ctrl Pts',(42.1653737847785,4.43390567942966,19.6652685471539));
#49756=CARTESIAN_POINT('Ctrl Pts',(42.1871192153285,4.43527922967145,18.4142216147178));
#49757=CARTESIAN_POINT('Ctrl Pts',(42.1975377622187,4.43593271204772,17.9113503761067));
#49758=CARTESIAN_POINT('Ctrl Pts',(42.2236822241422,4.43756527475675,16.9073116829106));
#49759=CARTESIAN_POINT('Ctrl Pts',(42.2797628188204,4.44107469922938,15.1534730382367));
#49760=CARTESIAN_POINT('Ctrl Pts',(42.3331943604571,4.44450509135218,13.651831009471));
#49761=CARTESIAN_POINT('Ctrl Pts',(42.3669550198508,4.44682915128521,12.3975686439851));
#49762=CARTESIAN_POINT('Ctrl Pts',(42.3807873604139,4.44779989493999,11.8967018737848));
#49763=CARTESIAN_POINT('Ctrl Pts',(42.4090840801753,4.44984468734248,10.8949964356632));
#49764=CARTESIAN_POINT('Ctrl Pts',(42.4442171196688,4.45246607212628,9.64252335981429));
#49765=CARTESIAN_POINT('Ctrl Pts',(42.4814072821943,4.45531901001824,8.13800024039924));
#49766=CARTESIAN_POINT('Ctrl Pts',(42.4998434201269,4.45675508843371,7.13312595518398));
#49767=CARTESIAN_POINT('Ctrl Pts',(42.5084122685094,4.45742537182735,6.50504551612233));
#49768=CARTESIAN_POINT('Ctrl Pts',(42.51160778917,4.45768189011103,6.2548761461837));
#49769=CARTESIAN_POINT('Ctrl Pts',(42.5171741324758,4.45815132839053,5.75380286805977));
#49770=CARTESIAN_POINT('Ctrl Pts',(42.5248501417164,4.45885435824313,4.87541295252293));
#49771=CARTESIAN_POINT('Ctrl Pts',(42.53273812315,4.45978601263875,3.11501628858445));
#49772=CARTESIAN_POINT('Ctrl Pts',(42.5294330916105,4.45970186585179,1.60755532665802));
#49773=CARTESIAN_POINT('Ctrl Pts',(42.5249151043497,4.45921098674461,0.547538475444217));
#49774=CARTESIAN_POINT('Ctrl Pts',(42.5243183972503,4.45914818259243,0.42131908384523));
#49775=CARTESIAN_POINT('Ctrl Pts',(42.5229020237262,4.45899935226643,0.169067490081134));
#49776=CARTESIAN_POINT('Ctrl Pts',(42.5198669424298,4.45868324002639,-0.271858993253347));
#49777=CARTESIAN_POINT('Ctrl Pts',(42.5141026079898,4.45807762005991,-0.9005622772302));
#49778=CARTESIAN_POINT('Ctrl Pts',(42.5054293061842,4.45717146798543,-1.65322810939649));
#49779=CARTESIAN_POINT('Ctrl Pts',(42.4922134460657,4.4557594557389,-2.65543993302332));
#49780=CARTESIAN_POINT('Ctrl Pts',(42.4739066559715,4.45377219520505,-3.90642746118527));
#49781=CARTESIAN_POINT('Ctrl Pts',(42.4601455997033,4.45218440214942,-4.90801081744749));
#49782=CARTESIAN_POINT('Ctrl Pts',(42.4526907229684,4.45130677983019,-5.53552450617664));
#49783=CARTESIAN_POINT('Ctrl Pts',(42.4505153709451,4.44981089037036,-5.80126348319439));
#49784=CARTESIAN_POINT('Ctrl Pts',(42.4487840037071,4.44317745383545,-6.31951543703047));
#49785=CARTESIAN_POINT('Ctrl Pts',(42.4510303132461,4.42430589539898,-7.21941478754799));
#49786=CARTESIAN_POINT('Ctrl Pts',(42.4602303355477,4.3893349439202,-8.46815781427861));
#49787=CARTESIAN_POINT('Ctrl Pts',(42.4532219858788,4.37685621361606,-9.66956937468799));
#49788=CARTESIAN_POINT('Ctrl Pts',(42.4271817651349,4.39590747938916,-10.4822054214672));
#49789=CARTESIAN_POINT('Ctrl Pts',(42.4044716210716,4.41668070021709,-10.9386148174557));
#49790=CARTESIAN_POINT('Ctrl Pts',(42.3902153921439,4.43063517945358,-11.1638416979877));
#49791=CARTESIAN_POINT('Ctrl Pts',(42.3782722056273,4.44263468939651,-11.3329536164645));
#49792=CARTESIAN_POINT('Ctrl Pts',(42.3697703806089,4.4519500151394,-11.4646692583993));
#49793=CARTESIAN_POINT('Ctrl Pts',(42.351321649476,4.46934048245381,-11.7159121980543));
#49794=CARTESIAN_POINT('Ctrl Pts',(42.3152439548395,4.49925129058086,-12.1560887373164));
#49795=CARTESIAN_POINT('Ctrl Pts',(42.2297056224542,4.55754971709465,-13.0140184699734));
#49796=CARTESIAN_POINT('Ctrl Pts',(42.0773240096532,4.64888468816603,-14.1882274322353));
#49797=CARTESIAN_POINT('Ctrl Pts',(41.9325191738719,4.77050106757277,-15.1912635102137));
#49798=CARTESIAN_POINT('Ctrl Pts',(41.8452918440761,4.88692134853426,-15.8482707091843));
#49799=CARTESIAN_POINT('Ctrl Pts',(41.7901431054233,4.97564273781242,-16.2835631550585));
#49800=CARTESIAN_POINT('Ctrl Pts',(41.7528864837405,5.05632896224043,-16.608048811206));
#49801=CARTESIAN_POINT('Ctrl Pts',(41.7246967815049,5.13293672777087,-16.8762028627259));
#49802=CARTESIAN_POINT('Ctrl Pts',(41.715396332616,5.15873444698128,-16.9612142112661));
#49803=CARTESIAN_POINT('Ctrl Pts',(41.6944040117279,5.22161590569571,-17.1514437495934));
#49804=CARTESIAN_POINT('Ctrl Pts',(41.672161523455,5.29428393728964,-17.3463288379007));
#49805=CARTESIAN_POINT('Ctrl Pts',(41.6479517267108,5.37832437641012,-17.552483703133));
#49806=CARTESIAN_POINT('Ctrl Pts',(41.6321781699855,5.43491908494667,-17.6841062705179));
#49807=CARTESIAN_POINT('Ctrl Pts',(41.6191255756403,5.48268422564165,-17.7915446933069));
#49808=CARTESIAN_POINT('Ctrl Pts',(41.6091394464926,5.51966990717561,-17.8729907465177));
#49809=CARTESIAN_POINT('Ctrl Pts',(41.600650421912,5.55144709136434,-17.9416361362078));
#49810=CARTESIAN_POINT('Ctrl Pts',(41.5937611144038,5.57742449020185,-17.996981410194));
#49811=CARTESIAN_POINT('Ctrl Pts',(41.5346675293466,5.80122879970189,-18.4699284319811));
#49812=CARTESIAN_POINT('Ctrl Pts',(41.4045373278031,6.32571973585028,-19.4466039091188));
#49813=CARTESIAN_POINT('Ctrl Pts',(41.1873260294732,7.19197459488153,-21.0465699183824));
#49814=CARTESIAN_POINT('Ctrl Pts',(41.0595608408375,7.70110568021989,-22.2372870473665));
#49815=CARTESIAN_POINT('Ctrl Pts',(41.0098926459178,7.95033509171429,-23.0367194728072));
#49816=CARTESIAN_POINT('Ctrl Pts',(40.9997427846034,8.03481830193072,-23.3111939636317));
#49817=CARTESIAN_POINT('Ctrl Pts',(40.9877047371297,8.1971669377381,-23.8792071216224));
#49818=CARTESIAN_POINT('Ctrl Pts',(40.9971528699687,8.44713220264407,-24.8513408873681));
#49819=CARTESIAN_POINT('Ctrl Pts',(41.0781879173059,8.72716793635427,-26.2183255071894));
#49820=CARTESIAN_POINT('Ctrl Pts',(41.232085897233,8.9607472408925,-27.7992151801498));
#49821=CARTESIAN_POINT('Ctrl Pts',(41.3275733968445,9.07279975647791,-28.8084262738872));
#49822=CARTESIAN_POINT('Ctrl Pts',(41.3663199668624,9.13284859687676,-29.3629560207209));
#49823=CARTESIAN_POINT('Ctrl Pts',(41.374418954637,9.14740642213019,-29.502410456033));
#49824=CARTESIAN_POINT('Ctrl Pts',(41.3910015401214,9.17309908398007,-29.7712916311122));
#49825=CARTESIAN_POINT('Ctrl Pts',(41.4200465535244,9.21262050656757,-30.2443705780784));
#49826=CARTESIAN_POINT('Ctrl Pts',(41.4785475784755,9.26973374039164,-31.178128557866));
#49827=CARTESIAN_POINT('Ctrl Pts',(41.5608973985288,9.30357052903612,-32.4869538878879));
#49828=CARTESIAN_POINT('Ctrl Pts',(41.6385333838955,9.30801153630281,-33.7540908153341));
#49829=CARTESIAN_POINT('Ctrl Pts',(41.6970645298839,9.31307806614043,-34.7421863638859));
#49830=CARTESIAN_POINT('Ctrl Pts',(41.725145340962,9.31904280747962,-35.2271388313623));
#49831=CARTESIAN_POINT('Ctrl Pts',(41.7457972589986,9.32585891497254,-35.5887587531886));
#49832=CARTESIAN_POINT('Ctrl Pts',(41.7596279291193,9.33040802484349,-35.8452562293953));
#49833=CARTESIAN_POINT('Ctrl Pts',(41.7870666252456,9.33854391595455,-36.3491403525278));
#49834=CARTESIAN_POINT('Ctrl Pts',(41.8343110804492,9.35083950840714,-37.2328678954738));
#49835=CARTESIAN_POINT('Ctrl Pts',(41.9242318227127,9.36875964061655,-38.9902018452413));
#49836=CARTESIAN_POINT('Ctrl Pts',(41.9877472130835,9.3773882204503,-40.4935747403769));
#49837=CARTESIAN_POINT('Ctrl Pts',(42.0272574366068,9.38538630372938,-41.7492890543106));
#49838=CARTESIAN_POINT('Ctrl Pts',(42.0381644075537,9.38721236589782,-42.1286435688507));
#49839=CARTESIAN_POINT('Ctrl Pts',(42.0511232360393,9.38880216746414,-42.6319389127963));
#49840=CARTESIAN_POINT('Ctrl Pts',(42.0630576969637,9.38997229832213,-43.1355830201978));
#49841=CARTESIAN_POINT('Ctrl Pts',(42.0761701660747,9.39088764188186,-43.7642917648869));
#49842=CARTESIAN_POINT('Ctrl Pts',(42.0893241462601,9.39189107665992,-44.5173903243411));
#49843=CARTESIAN_POINT('Ctrl Pts',(42.0983983816962,9.39329188039546,-45.1432207338739));
#49844=CARTESIAN_POINT('Ctrl Pts',(42.1047279826398,9.3951652624769,-45.6425970992607));
#49845=CARTESIAN_POINT('Ctrl Pts',(42.1090298863024,9.39702639675693,-46.0164087043907));
#49846=CARTESIAN_POINT('Ctrl Pts',(42.1129296314231,9.39943973181789,-46.3894634288434));
#49847=CARTESIAN_POINT('Ctrl Pts',(42.1176583956564,9.40352647135289,-46.8856896438178));
#49848=CARTESIAN_POINT('Ctrl Pts',(42.1206949411916,9.40767304516513,-47.2566448321986));
#49849=CARTESIAN_POINT('Ctrl Pts',(42.1235199090029,9.41276160489034,-47.6270477559909));
#49850=CARTESIAN_POINT('Ctrl Pts',(42.1250877992718,9.4172418231088,-47.8629849085641));
#49851=CARTESIAN_POINT('Ctrl Pts',(42.1270615745575,9.43060438525352,-48.3469638310146));
#49852=CARTESIAN_POINT('Ctrl Pts',(42.1277850714073,9.46312836091267,-49.2019780343514));
#49853=CARTESIAN_POINT('Ctrl Pts',(42.1229160656678,9.5238508496721,-50.4596868135424));
#49854=CARTESIAN_POINT('Ctrl Pts',(42.1133957123464,9.5772391955778,-52.0205213259128));
#49855=CARTESIAN_POINT('Ctrl Pts',(42.1084948227126,9.56874892174017,-53.0965359880168));
#49856=CARTESIAN_POINT('Ctrl Pts',(42.1073149193619,9.53893199127567,-53.7823908590073));
#49857=CARTESIAN_POINT('Ctrl Pts',(42.1068070481075,9.52000368930904,-54.0890497549449));
#49858=CARTESIAN_POINT('Ctrl Pts',(42.1057800418371,9.46508757911363,-54.6685113050492));
#49859=CARTESIAN_POINT('Ctrl Pts',(42.1038697439046,9.33357303918558,-55.6522294188415));
#49860=CARTESIAN_POINT('Ctrl Pts',(42.1014299978837,9.00154770075439,-57.4608506741487));
#49861=CARTESIAN_POINT('Ctrl Pts',(42.0981196164158,8.83054051958777,-58.7441892388778));
#49862=CARTESIAN_POINT('Ctrl Pts',(42.102473629823,8.87389154790522,-59.5018847710551));
#49863=CARTESIAN_POINT('Ctrl Pts',(42.1029927927764,8.88102566132885,-59.6144631853288));
#49864=CARTESIAN_POINT('Ctrl Pts',(42.1042902056847,8.89787525908731,-59.8290965989406));
#49865=CARTESIAN_POINT('Ctrl Pts',(42.1070771307108,8.93590705043286,-60.2127458185008));
#49866=CARTESIAN_POINT('Ctrl Pts',(42.1145055180033,9.04366772762629,-60.9845447964307));
#49867=CARTESIAN_POINT('Ctrl Pts',(42.1256720654178,9.23499438509171,-61.8869276390296));
#49868=CARTESIAN_POINT('Ctrl Pts',(42.1367429007561,9.48260508362316,-62.8003515442931));
#49869=CARTESIAN_POINT('Ctrl Pts',(42.14250105984,9.64046459144008,-63.3177835092151));
#49870=CARTESIAN_POINT('Ctrl Pts',(42.1459717192686,9.75238155687925,-63.6636132991502));
#49871=CARTESIAN_POINT('Ctrl Pts',(42.1481777795587,9.82869851579108,-63.8944172718737));
#49872=CARTESIAN_POINT('Ctrl Pts',(42.1502082497363,9.90743557445359,-64.1254062764649));
#49873=CARTESIAN_POINT('Ctrl Pts',(42.1518026560732,9.9782825312177,-64.3277498871866));
#49874=CARTESIAN_POINT('Ctrl Pts',(42.1526581514894,10.0192943221162,-64.4434190207101));
#49875=CARTESIAN_POINT('Ctrl Pts',(42.1538847500963,10.0813139802647,-64.616934095387));
#49876=CARTESIAN_POINT('Ctrl Pts',(42.1547828775597,10.1340519497849,-64.7616293724365));
#49877=CARTESIAN_POINT('Ctrl Pts',(42.1561038287678,10.2223350366598,-65.0005771275026));
#49878=CARTESIAN_POINT('Ctrl Pts',(42.1582105074284,10.3048934440516,-65.2131820487537));
#49879=CARTESIAN_POINT('Ctrl Pts',(42.1614148903209,10.4938853814907,-65.6631041403599));
#49880=CARTESIAN_POINT('Ctrl Pts',(42.1659317372334,10.8617557144184,-66.4523321841232));
#49881=CARTESIAN_POINT('Ctrl Pts',(42.1697446831104,11.7410172575913,-68.0912718937255));
#49882=CARTESIAN_POINT('Ctrl Pts',(42.1665941544893,12.6391474445693,-69.585738936787));
#49883=CARTESIAN_POINT('Ctrl Pts',(42.164216736395,13.2713485701069,-70.7872900881665));
#49884=CARTESIAN_POINT('Ctrl Pts',(42.1644755981786,13.4001883022114,-71.031839329675));
#49885=CARTESIAN_POINT('Ctrl Pts',(42.1645103319829,13.6655586906436,-71.5343623900713));
#49886=CARTESIAN_POINT('Ctrl Pts',(42.1646955444271,13.9955320466049,-72.1570933130439));
#49887=CARTESIAN_POINT('Ctrl Pts',(42.1647527808815,14.3945740389569,-72.9077835335904));
#49888=CARTESIAN_POINT('Ctrl Pts',(42.1648264840299,15.1940437661561,-74.4082770771058));
#49889=CARTESIAN_POINT('Ctrl Pts',(42.1647109721311,15.8639134512714,-75.6611090767548));
#49890=CARTESIAN_POINT('Ctrl Pts',(42.1645878003007,16.8356533223413,-77.4884825573361));
#49891=CARTESIAN_POINT('Ctrl Pts',(42.164642108565,17.2713436057313,-78.3077784929303));
#49892=CARTESIAN_POINT('Ctrl Pts',(42.1646421085649,17.7078651931207,-79.1287561950287));
#49893=CARTESIAN_POINT('Ctrl Pts',(44.9333669821193,4.63587816982636,24.8307041888048));
#49894=CARTESIAN_POINT('Ctrl Pts',(44.9334979023578,4.63589034715466,24.7818270640558));
#49895=CARTESIAN_POINT('Ctrl Pts',(44.9336352132025,4.63590311675132,24.7329510937676));
#49896=CARTESIAN_POINT('Ctrl Pts',(44.9352566680075,4.63605389014306,24.1823667254701));
#49897=CARTESIAN_POINT('Ctrl Pts',(44.9364556490902,4.63619612515483,23.1782347087865));
#49898=CARTESIAN_POINT('Ctrl Pts',(44.9392184572998,4.63654477111558,21.1696867815275));
#49899=CARTESIAN_POINT('Ctrl Pts',(44.9500110013522,4.63754679539249,19.6655321882608));
#49900=CARTESIAN_POINT('Ctrl Pts',(44.9731189460185,4.63953900490499,18.4144926058473));
#49901=CARTESIAN_POINT('Ctrl Pts',(44.984185233339,4.64050938219707,17.9118227013444));
#49902=CARTESIAN_POINT('Ctrl Pts',(45.0119472070561,4.64297264048472,16.9079214810503));
#49903=CARTESIAN_POINT('Ctrl Pts',(45.0715072955918,4.64825356183551,15.1540495788374));
#49904=CARTESIAN_POINT('Ctrl Pts',(45.1283478334055,4.65306438840288,13.6517227532813));
#49905=CARTESIAN_POINT('Ctrl Pts',(45.1644336381274,4.65570009337017,12.3966002597124));
#49906=CARTESIAN_POINT('Ctrl Pts',(45.1792335941515,4.65673530413848,11.895383592665));
#49907=CARTESIAN_POINT('Ctrl Pts',(45.2095615747859,4.6587103195502,10.8931727060101));
#49908=CARTESIAN_POINT('Ctrl Pts',(45.2472949754295,4.66094941471739,9.64032070536151));
#49909=CARTESIAN_POINT('Ctrl Pts',(45.2873515969718,4.66311480069243,8.13584259206917));
#49910=CARTESIAN_POINT('Ctrl Pts',(45.3072846050537,4.66410108210267,7.13126553200396));
#49911=CARTESIAN_POINT('Ctrl Pts',(45.3165865636776,4.66454211847491,6.50346922286369));
#49912=CARTESIAN_POINT('Ctrl Pts',(45.3200619051891,4.66468562275181,6.25304880874878));
#49913=CARTESIAN_POINT('Ctrl Pts',(45.3261392327148,4.66486046820295,5.75176838221114));
#49914=CARTESIAN_POINT('Ctrl Pts',(45.3345868607911,4.66490596131958,4.87307865335014));
#49915=CARTESIAN_POINT('Ctrl Pts',(45.343562651372,4.66426069244295,3.11300099070761));
#49916=CARTESIAN_POINT('Ctrl Pts',(45.3405430703049,4.66342578091586,1.60687954862173));
#49917=CARTESIAN_POINT('Ctrl Pts',(45.3360427857126,4.66366032599448,0.548605170266317));
#49918=CARTESIAN_POINT('Ctrl Pts',(45.3354519489155,4.66369145735315,0.422590875695751));
#49919=CARTESIAN_POINT('Ctrl Pts',(45.3340608597991,4.66376449726404,0.170728951294827));
#49920=CARTESIAN_POINT('Ctrl Pts',(45.3310991987033,4.66392039122531,-0.26956437068448));
#49921=CARTESIAN_POINT('Ctrl Pts',(45.325492148662,4.66421182722607,-0.897571164468606));
#49922=CARTESIAN_POINT('Ctrl Pts',(45.3169761097054,4.66466508037382,-1.64953651843115));
#49923=CARTESIAN_POINT('Ctrl Pts',(45.3037963714485,4.66535305212888,-2.65122580347224));
#49924=CARTESIAN_POINT('Ctrl Pts',(45.2849366378433,4.66632617957509,-3.90218803647896));
#49925=CARTESIAN_POINT('Ctrl Pts',(45.2695380422325,4.66700510860821,-4.90425811297242));
#49926=CARTESIAN_POINT('Ctrl Pts',(45.2605037636271,4.6673525618632,-5.53292392344991));
#49927=CARTESIAN_POINT('Ctrl Pts',(45.2579511424781,4.66497636398758,-5.81475951906011));
#49928=CARTESIAN_POINT('Ctrl Pts',(45.25626273268,4.65221408575269,-6.35050785645233));
#49929=CARTESIAN_POINT('Ctrl Pts',(45.2600538878317,4.61439141343846,-7.27242908556972));
#49930=CARTESIAN_POINT('Ctrl Pts',(45.2723247521635,4.54589500426883,-8.51158077669593));
#49931=CARTESIAN_POINT('Ctrl Pts',(45.2615711141445,4.52686668740426,-9.65381276654877));
#49932=CARTESIAN_POINT('Ctrl Pts',(45.225449036529,4.56656545267834,-10.3973910987338));
#49933=CARTESIAN_POINT('Ctrl Pts',(45.1944970405879,4.60700490521411,-10.8072424755639));
#49934=CARTESIAN_POINT('Ctrl Pts',(45.175294273951,4.63349787943198,-11.0070600284335));
#49935=CARTESIAN_POINT('Ctrl Pts',(45.1593270749882,4.65598440875296,-11.1560398985103));
#49936=CARTESIAN_POINT('Ctrl Pts',(45.1475104260899,4.67364615357786,-11.2648315375785));
#49937=CARTESIAN_POINT('Ctrl Pts',(45.1206604029663,4.7107868069394,-11.4784866796688));
#49938=CARTESIAN_POINT('Ctrl Pts',(45.0656450549295,4.78318112797988,-11.8572625762786));
#49939=CARTESIAN_POINT('Ctrl Pts',(44.9291075434275,4.95228012845482,-12.6240386706489));
#49940=CARTESIAN_POINT('Ctrl Pts',(44.6929466638584,5.24814367801828,-13.7657020756945));
#49941=CARTESIAN_POINT('Ctrl Pts',(44.5043923325839,5.57416245985198,-14.8524096422358));
#49942=CARTESIAN_POINT('Ctrl Pts',(44.4075739601456,5.82140209288632,-15.5941629233189));
#49943=CARTESIAN_POINT('Ctrl Pts',(44.3512027368814,5.99428860812313,-16.0922118718401));
#49944=CARTESIAN_POINT('Ctrl Pts',(44.3190745151794,6.13339619520395,-16.4694384969807));
#49945=CARTESIAN_POINT('Ctrl Pts',(44.299226354482,6.25379420494699,-16.7826337520401));
#49946=CARTESIAN_POINT('Ctrl Pts',(44.2969229064794,6.29291565417392,-16.8764705598309));
#49947=CARTESIAN_POINT('Ctrl Pts',(44.2902827333537,6.38480407787161,-17.0866420639222));
#49948=CARTESIAN_POINT('Ctrl Pts',(44.2860475637416,6.48497231549507,-17.2959799360825));
#49949=CARTESIAN_POINT('Ctrl Pts',(44.2820535485249,6.59558853274627,-17.5143805077403));
#49950=CARTESIAN_POINT('Ctrl Pts',(44.2799827571647,6.66801192718192,-17.6522587472907));
#49951=CARTESIAN_POINT('Ctrl Pts',(44.2784147873834,6.72802588610404,-17.7641449538538));
#49952=CARTESIAN_POINT('Ctrl Pts',(44.2773150161733,6.77395220332713,-17.8486085072498));
#49953=CARTESIAN_POINT('Ctrl Pts',(44.2764425517342,6.81298585885999,-17.919542477742));
#49954=CARTESIAN_POINT('Ctrl Pts',(44.2757697912063,6.84463869239768,-17.9765872337853));
#49955=CARTESIAN_POINT('Ctrl Pts',(44.2702372924635,7.11608657359585,-18.4632195255323));
#49956=CARTESIAN_POINT('Ctrl Pts',(44.2630045039821,7.7074245624471,-19.4457608820307));
#49957=CARTESIAN_POINT('Ctrl Pts',(44.2611419814737,8.6222707657364,-21.0521041695837));
#49958=CARTESIAN_POINT('Ctrl Pts',(44.2725461051462,9.13292987135093,-22.2730506947804));
#49959=CARTESIAN_POINT('Ctrl Pts',(44.2816142769132,9.35867008260939,-23.099799003702));
#49960=CARTESIAN_POINT('Ctrl Pts',(44.2876325887398,9.43432231200718,-23.4010860497399));
#49961=CARTESIAN_POINT('Ctrl Pts',(44.3058999069322,9.56020964037718,-24.0113613345034));
#49962=CARTESIAN_POINT('Ctrl Pts',(44.3525560292799,9.71031473239032,-25.0527674960325));
#49963=CARTESIAN_POINT('Ctrl Pts',(44.4443173329707,9.77268873266039,-26.4730277999505));
#49964=CARTESIAN_POINT('Ctrl Pts',(44.55190239764,9.73690379055372,-28.044254216766));
#49965=CARTESIAN_POINT('Ctrl Pts',(44.6030629052135,9.71526496697493,-29.0043367489214));
#49966=CARTESIAN_POINT('Ctrl Pts',(44.6217562968118,9.71971469691473,-29.5208988965381));
#49967=CARTESIAN_POINT('Ctrl Pts',(44.6257907026183,9.72052246806346,-29.6585948864942));
#49968=CARTESIAN_POINT('Ctrl Pts',(44.6330315310391,9.72062718334552,-29.9202917581488));
#49969=CARTESIAN_POINT('Ctrl Pts',(44.6437898559616,9.71741656585746,-30.3829589911478));
#49970=CARTESIAN_POINT('Ctrl Pts',(44.6583278615562,9.69897448965321,-31.2959284016156));
#49971=CARTESIAN_POINT('Ctrl Pts',(44.6639992263246,9.64838030429391,-32.5818848810449));
#49972=CARTESIAN_POINT('Ctrl Pts',(44.662053705329,9.58931415476959,-33.8363371428099));
#49973=CARTESIAN_POINT('Ctrl Pts',(44.6631620352193,9.54999353886839,-34.8212887515721));
#49974=CARTESIAN_POINT('Ctrl Pts',(44.665816383274,9.53502460744065,-35.3070035254001));
#49975=CARTESIAN_POINT('Ctrl Pts',(44.6690383588918,9.52628046901086,-35.6699624300507));
#49976=CARTESIAN_POINT('Ctrl Pts',(44.6712928845314,9.52019431481522,-35.9233658300565));
#49977=CARTESIAN_POINT('Ctrl Pts',(44.6760911582724,9.50849652247419,-36.4234977421827));
#49978=CARTESIAN_POINT('Ctrl Pts',(44.685147460511,9.48876679621087,-37.2999188157056));
#49979=CARTESIAN_POINT('Ctrl Pts',(44.7046283752818,9.45311685214669,-39.0448048665985));
#49980=CARTESIAN_POINT('Ctrl Pts',(44.7197705753507,9.43012322769321,-40.5386959198999));
#49981=CARTESIAN_POINT('Ctrl Pts',(44.7269699252603,9.41682046044001,-41.7869668791111));
#49982=CARTESIAN_POINT('Ctrl Pts',(44.7286300530116,9.41246364758171,-42.164811723922));
#49983=CARTESIAN_POINT('Ctrl Pts',(44.730085289389,9.40654236583585,-42.6653424239963));
#49984=CARTESIAN_POINT('Ctrl Pts',(44.7311163037048,9.40067534306281,-43.1661034760371));
#49985=CARTESIAN_POINT('Ctrl Pts',(44.7317465398154,9.39377152228866,-43.7907628656876));
#49986=CARTESIAN_POINT('Ctrl Pts',(44.7319011558653,9.38713394939372,-44.5384113611807));
#49987=CARTESIAN_POINT('Ctrl Pts',(44.7319043098671,9.38377476804963,-45.1591833277389));
#49988=CARTESIAN_POINT('Ctrl Pts',(44.7320495731726,9.38287360366303,-45.6542337605805));
#49989=CARTESIAN_POINT('Ctrl Pts',(44.7322894649879,9.38320418990688,-46.0246454874006));
#49990=CARTESIAN_POINT('Ctrl Pts',(44.7327160627022,9.38465971037982,-46.3941481905926));
#49991=CARTESIAN_POINT('Ctrl Pts',(44.7336068540788,9.3882586426597,-46.8854311103639));
#49992=CARTESIAN_POINT('Ctrl Pts',(44.734728483665,9.39299139524036,-47.2524296398557));
#49993=CARTESIAN_POINT('Ctrl Pts',(44.7362621756588,9.3993314064098,-47.6186566589199));
#49994=CARTESIAN_POINT('Ctrl Pts',(44.7372683747344,9.40488441682722,-47.8500549667319));
#49995=CARTESIAN_POINT('Ctrl Pts',(44.7391923515483,9.42160812051236,-48.3268142682009));
#49996=CARTESIAN_POINT('Ctrl Pts',(44.7424819869383,9.46295827084018,-49.1706486727884));
#49997=CARTESIAN_POINT('Ctrl Pts',(44.7476480509491,9.54397160623419,-50.4182362572702));
#49998=CARTESIAN_POINT('Ctrl Pts',(44.7572798693228,9.62975168477225,-51.9754036097172));
#49999=CARTESIAN_POINT('Ctrl Pts',(44.7679244366479,9.64388643626604,-53.0551856218759));
#50000=CARTESIAN_POINT('Ctrl Pts',(44.7766541899908,9.62670923029403,-53.7452837511029));
#50001=CARTESIAN_POINT('Ctrl Pts',(44.7806492307899,9.61386186366492,-54.0487471333629));
#50002=CARTESIAN_POINT('Ctrl Pts',(44.7899635506518,9.57141967994042,-54.6254954386526));
#50003=CARTESIAN_POINT('Ctrl Pts',(44.8090369070717,9.46305212497968,-55.6049996912444));
#50004=CARTESIAN_POINT('Ctrl Pts',(44.8535080186623,9.17796813642923,-57.4128116283892));
#50005=CARTESIAN_POINT('Ctrl Pts',(44.8871058615105,9.03482251140912,-58.7066364139985));
#50006=CARTESIAN_POINT('Ctrl Pts',(44.9025681610021,9.08815669291933,-59.4823187154555));
#50007=CARTESIAN_POINT('Ctrl Pts',(44.9043036643419,9.09661811168106,-59.5969035133632));
#50008=CARTESIAN_POINT('Ctrl Pts',(44.9076457910595,9.11571979425487,-59.8154200625901));
#50009=CARTESIAN_POINT('Ctrl Pts',(44.9130012877661,9.15698333644756,-60.2052869646091));
#50010=CARTESIAN_POINT('Ctrl Pts',(44.9220063838328,9.26828364727815,-60.987323531218));
#50011=CARTESIAN_POINT('Ctrl Pts',(44.9289888871208,9.45792877534444,-61.8962934745214));
#50012=CARTESIAN_POINT('Ctrl Pts',(44.9340057627777,9.70063939087671,-62.8116504337714));
#50013=CARTESIAN_POINT('Ctrl Pts',(44.9363590175526,9.85513792044804,-63.3285348517037));
#50014=CARTESIAN_POINT('Ctrl Pts',(44.9378449419104,9.96480529890248,-63.673351095806));
#50015=CARTESIAN_POINT('Ctrl Pts',(44.9388207088418,10.0396397863523,-63.9033067107434));
#50016=CARTESIAN_POINT('Ctrl Pts',(44.9397905035546,10.1169431330247,-64.1331971180868));
#50017=CARTESIAN_POINT('Ctrl Pts',(44.9406491940526,10.1866267537447,-64.3343557746241));
#50018=CARTESIAN_POINT('Ctrl Pts',(44.9411462012543,10.2270060089222,-64.4492842746316));
#50019=CARTESIAN_POINT('Ctrl Pts',(44.9419002284174,10.2881135621904,-64.6216269443045));
#50020=CARTESIAN_POINT('Ctrl Pts',(44.9425480773535,10.3401695449471,-64.7652089194153));
#50021=CARTESIAN_POINT('Ctrl Pts',(44.9436808820581,10.4274889561099,-65.002183647395));
#50022=CARTESIAN_POINT('Ctrl Pts',(44.9457296368594,10.5100058197732,-65.2151434701464));
#50023=CARTESIAN_POINT('Ctrl Pts',(44.9488563346992,10.6984555106575,-65.6644707635653));
#50024=CARTESIAN_POINT('Ctrl Pts',(44.9534691872529,11.0658192309505,-66.4534539136408));
#50025=CARTESIAN_POINT('Ctrl Pts',(44.9578122690832,11.9444667864977,-68.0917160342065));
#50026=CARTESIAN_POINT('Ctrl Pts',(44.9547060432961,12.842828120554,-69.5864114707208));
#50027=CARTESIAN_POINT('Ctrl Pts',(44.951532773924,13.4749122379537,-70.7882465589457));
#50028=CARTESIAN_POINT('Ctrl Pts',(44.9518124352172,13.6037024593924,-71.0327438068155));
#50029=CARTESIAN_POINT('Ctrl Pts',(44.9517934305402,13.8690078572436,-71.5352327466239));
#50030=CARTESIAN_POINT('Ctrl Pts',(44.9519840675579,14.1989254473966,-72.1579099499273));
#50031=CARTESIAN_POINT('Ctrl Pts',(44.9520529495098,14.597943036186,-72.9085592690338));
#50032=CARTESIAN_POINT('Ctrl Pts',(44.9522036988278,15.3974222066628,-74.4089927823421));
#50033=CARTESIAN_POINT('Ctrl Pts',(44.9521854715562,16.0673918589498,-75.6618676901378));
#50034=CARTESIAN_POINT('Ctrl Pts',(44.952029847549,17.0391786068487,-77.4893496207617));
#50035=CARTESIAN_POINT('Ctrl Pts',(44.9520993138037,17.4748560812393,-78.3086236045963));
#50036=CARTESIAN_POINT('Ctrl Pts',(44.9520993138036,17.9113776686288,-79.1296013066945));
#50037=CARTESIAN_POINT('Ctrl Pts',(47.7140540990422,4.88276541972323,24.8307163556754));
#50038=CARTESIAN_POINT('Ctrl Pts',(47.7141971173369,4.88278120060972,24.7818396449418));
#50039=CARTESIAN_POINT('Ctrl Pts',(47.7143471136432,4.88279775286369,24.7329641087686));
#50040=CARTESIAN_POINT('Ctrl Pts',(47.7161182130505,4.88299298383964,24.1823841333583));
#50041=CARTESIAN_POINT('Ctrl Pts',(47.7175115582471,4.8831861471748,23.1782641182978));
#50042=CARTESIAN_POINT('Ctrl Pts',(47.7207801503277,4.8836674491671,21.1697193937816));
#50043=CARTESIAN_POINT('Ctrl Pts',(47.7325651987108,4.88496318581718,19.6655383093397));
#50044=CARTESIAN_POINT('Ctrl Pts',(47.757378839843,4.88749314359155,18.4144737796136));
#50045=CARTESIAN_POINT('Ctrl Pts',(47.7693014564166,4.88871928109935,17.9117784514982));
#50046=CARTESIAN_POINT('Ctrl Pts',(47.7992812031425,4.89181749989893,16.9078631888763));
#50047=CARTESIAN_POINT('Ctrl Pts',(47.8635810010464,4.89844697175688,15.1540271445886));
#50048=CARTESIAN_POINT('Ctrl Pts',(47.9243824440423,4.90452675243611,13.6517624151243));
#50049=CARTESIAN_POINT('Ctrl Pts',(47.9619455787172,4.90795802124528,12.3967075962964));
#50050=CARTESIAN_POINT('Ctrl Pts',(47.9772376973858,4.90931662958083,11.8955151113586));
#50051=CARTESIAN_POINT('Ctrl Pts',(48.0082082808038,4.91194454293002,10.8933262319668));
#50052=CARTESIAN_POINT('Ctrl Pts',(48.046211838742,4.91498035507158,9.64042959022222));
#50053=CARTESIAN_POINT('Ctrl Pts',(48.0860185467446,4.91797824695313,8.13589047411817));
#50054=CARTESIAN_POINT('Ctrl Pts',(48.1056098351614,4.91937625239819,7.13124158256873));
#50055=CARTESIAN_POINT('Ctrl Pts',(48.1146981889812,4.92001433792512,6.50342636458933));
#50056=CARTESIAN_POINT('Ctrl Pts',(48.1180371737479,4.92023305876676,6.25306617747529));
#50057=CARTESIAN_POINT('Ctrl Pts',(48.1236727259873,4.92054064178157,5.75184956235704));
#50058=CARTESIAN_POINT('Ctrl Pts',(48.1309872142257,4.92077098009341,4.87322641890403));
#50059=CARTESIAN_POINT('Ctrl Pts',(48.1369265441169,4.92033171306085,3.11310955178566));
#50060=CARTESIAN_POINT('Ctrl Pts',(48.1322764461187,4.91940466989494,1.60646990766414));
#50061=CARTESIAN_POINT('Ctrl Pts',(48.129245719316,4.91953876976763,0.547621487047117));
#50062=CARTESIAN_POINT('Ctrl Pts',(48.1288783623415,4.9195368662062,0.420854514195474));
#50063=CARTESIAN_POINT('Ctrl Pts',(48.1281131888024,4.91945090085748,0.167995994665409));
#50064=CARTESIAN_POINT('Ctrl Pts',(48.126678129514,4.91911460500282,-0.273960982828218));
#50065=CARTESIAN_POINT('Ctrl Pts',(48.1242588428073,4.91820359136341,-0.903463341764215));
#50066=CARTESIAN_POINT('Ctrl Pts',(48.1204801725179,4.91687631511617,-1.65588634714346));
#50067=CARTESIAN_POINT('Ctrl Pts',(48.1138698310929,4.91526522898741,-2.65644975655062));
#50068=CARTESIAN_POINT('Ctrl Pts',(48.1019227893584,4.91469403605023,-3.90268697487727));
#50069=CARTESIAN_POINT('Ctrl Pts',(48.0868609972421,4.91793322355432,-4.89715028181298));
#50070=CARTESIAN_POINT('Ctrl Pts',(48.0752321103946,4.92190940017826,-5.52055922497928));
#50071=CARTESIAN_POINT('Ctrl Pts',(48.0712633898345,4.92005083458062,-5.81518377909426));
#50072=CARTESIAN_POINT('Ctrl Pts',(48.0655015626684,4.90450636863208,-6.36312763586707));
#50073=CARTESIAN_POINT('Ctrl Pts',(48.0592168020764,4.85552961531939,-7.29939475139431));
#50074=CARTESIAN_POINT('Ctrl Pts',(48.0511976567384,4.76958316060189,-8.52471463285954));
#50075=CARTESIAN_POINT('Ctrl Pts',(48.0199164246137,4.75932888021026,-9.61059960005426));
#50076=CARTESIAN_POINT('Ctrl Pts',(47.9752816089115,4.82181429860099,-10.2929408967411));
#50077=CARTESIAN_POINT('Ctrl Pts',(47.9424979225489,4.87987419509223,-10.6643694086282));
#50078=CARTESIAN_POINT('Ctrl Pts',(47.9236288796491,4.91691909256987,-10.8445900060882));
#50079=CARTESIAN_POINT('Ctrl Pts',(47.9084971204255,4.94799809250737,-10.9784412427892));
#50080=CARTESIAN_POINT('Ctrl Pts',(47.8976355795159,4.96884528601334,-11.0610698453323));
#50081=CARTESIAN_POINT('Ctrl Pts',(47.8727229773347,5.01818225658932,-11.2371677963152));
#50082=CARTESIAN_POINT('Ctrl Pts',(47.8218781901417,5.12167551518096,-11.5580728652217));
#50083=CARTESIAN_POINT('Ctrl Pts',(47.6967732133967,5.39744374854651,-12.2606177190604));
#50084=CARTESIAN_POINT('Ctrl Pts',(47.4805558259505,5.96971223774114,-13.4089363387501));
#50085=CARTESIAN_POINT('Ctrl Pts',(47.2864638625924,6.59347980095187,-14.5733310719199));
#50086=CARTESIAN_POINT('Ctrl Pts',(47.1773736182701,7.00141160295155,-15.4007988051126));
#50087=CARTESIAN_POINT('Ctrl Pts',(47.1122976380426,7.26794126587674,-15.9669900830333));
#50088=CARTESIAN_POINT('Ctrl Pts',(47.0741237010702,7.45793602346966,-16.4088688151826));
#50089=CARTESIAN_POINT('Ctrl Pts',(47.0518022747637,7.6058210314354,-16.7857958495628));
#50090=CARTESIAN_POINT('Ctrl Pts',(47.0489742060024,7.65345793122167,-16.9020873872941));
#50091=CARTESIAN_POINT('Ctrl Pts',(47.043384940024,7.7572671761431,-17.154408557878));
#50092=CARTESIAN_POINT('Ctrl Pts',(47.0433955158451,7.86100386175213,-17.4003654293072));
#50093=CARTESIAN_POINT('Ctrl Pts',(47.0469238435683,7.96774815158817,-17.6512767660494));
#50094=CARTESIAN_POINT('Ctrl Pts',(47.0509092928993,8.0347187919395,-17.8077901965876));
#50095=CARTESIAN_POINT('Ctrl Pts',(47.0549903822185,8.08864548775169,-17.9336983160115));
#50096=CARTESIAN_POINT('Ctrl Pts',(47.0585259276304,8.12915788199319,-18.0282424756206));
#50097=CARTESIAN_POINT('Ctrl Pts',(47.0618417665668,8.16298950947656,-18.1072348211177));
#50098=CARTESIAN_POINT('Ctrl Pts',(47.0647166611982,8.1900763342476,-18.1705263139997));
#50099=CARTESIAN_POINT('Ctrl Pts',(47.0903610767103,8.42040249669643,-18.7091546133712));
#50100=CARTESIAN_POINT('Ctrl Pts',(47.1782761053397,8.86342262799073,-19.7591085302407));
#50101=CARTESIAN_POINT('Ctrl Pts',(47.3622945182627,9.42369471265307,-21.4015509469075));
#50102=CARTESIAN_POINT('Ctrl Pts',(47.4614748893442,9.67809115965601,-22.556175004692));
#50103=CARTESIAN_POINT('Ctrl Pts',(47.4939758264104,9.79163368355877,-23.2884768894686));
#50104=CARTESIAN_POINT('Ctrl Pts',(47.5058241833002,9.83393921132415,-23.5903433667823));
#50105=CARTESIAN_POINT('Ctrl Pts',(47.527080293437,9.89432197909471,-24.1776719661128));
#50106=CARTESIAN_POINT('Ctrl Pts',(47.5570667969751,9.95034896451951,-25.1861886156599));
#50107=CARTESIAN_POINT('Ctrl Pts',(47.5813189919887,9.92692150286911,-26.5544701327999));
#50108=CARTESIAN_POINT('Ctrl Pts',(47.5907919954819,9.84487695116789,-28.0872067810766));
#50109=CARTESIAN_POINT('Ctrl Pts',(47.5895961217043,9.81034388656042,-29.0326355854953));
#50110=CARTESIAN_POINT('Ctrl Pts',(47.5878944989112,9.8094997328447,-29.543045756842));
#50111=CARTESIAN_POINT('Ctrl Pts',(47.5872811789768,9.80921610815855,-29.6731667034628));
#50112=CARTESIAN_POINT('Ctrl Pts',(47.5853766864156,9.80848681579351,-29.9239474618171));
#50113=CARTESIAN_POINT('Ctrl Pts',(47.5802903111877,9.80670231759085,-30.3674344249167));
#50114=CARTESIAN_POINT('Ctrl Pts',(47.5640056156477,9.80132977906479,-31.2501910378675));
#50115=CARTESIAN_POINT('Ctrl Pts',(47.5279973552059,9.78911979854965,-32.510888638707));
#50116=CARTESIAN_POINT('Ctrl Pts',(47.4878923241183,9.77377649988443,-33.7647088759262));
#50117=CARTESIAN_POINT('Ctrl Pts',(47.4612495425572,9.76236532583633,-34.7634274753251));
#50118=CARTESIAN_POINT('Ctrl Pts',(47.4510763748714,9.75745732390579,-35.2610383747428));
#50119=CARTESIAN_POINT('Ctrl Pts',(47.4451123721182,9.75431432208389,-35.6345701057286));
#50120=CARTESIAN_POINT('Ctrl Pts',(47.4413196822235,9.75228836524071,-35.8865342472504));
#50121=CARTESIAN_POINT('Ctrl Pts',(47.4344830515908,9.74825789205966,-36.388694212146));
#50122=CARTESIAN_POINT('Ctrl Pts',(47.4242868162918,9.74134624202967,-37.2664093733548));
#50123=CARTESIAN_POINT('Ctrl Pts',(47.4098208967714,9.72862251883125,-39.01646234273));
#50124=CARTESIAN_POINT('Ctrl Pts',(47.4029054140399,9.72041099201589,-40.5149166685421));
#50125=CARTESIAN_POINT('Ctrl Pts',(47.3954184588552,9.71639541728355,-41.7677554829351));
#50126=CARTESIAN_POINT('Ctrl Pts',(47.3928919742263,9.71475439976693,-42.1459791643895));
#50127=CARTESIAN_POINT('Ctrl Pts',(47.3892407582933,9.71214425217703,-42.6477286125353));
#50128=CARTESIAN_POINT('Ctrl Pts',(47.3854959843847,9.70939409226986,-43.1497036668692));
#50129=CARTESIAN_POINT('Ctrl Pts',(47.3808428311234,9.70599285160254,-43.7761834401676));
#50130=CARTESIAN_POINT('Ctrl Pts',(47.3759290165794,9.70289100421383,-44.5263946243753));
#50131=CARTESIAN_POINT('Ctrl Pts',(47.3729163064396,9.70188685186302,-45.1496679134366));
#50132=CARTESIAN_POINT('Ctrl Pts',(47.3714890385956,9.70250109054733,-45.6469583727039));
#50133=CARTESIAN_POINT('Ctrl Pts',(47.3709808369827,9.70377682246791,-46.0191617072633));
#50134=CARTESIAN_POINT('Ctrl Pts',(47.3711155244775,9.70598203671017,-46.3905676980616));
#50135=CARTESIAN_POINT('Ctrl Pts',(47.3722619960134,9.71030876625392,-46.8845459369719));
#50136=CARTESIAN_POINT('Ctrl Pts',(47.3743161765341,9.71528383058321,-47.2537195147694));
#50137=CARTESIAN_POINT('Ctrl Pts',(47.3773474890592,9.72163710347664,-47.6222653452682));
#50138=CARTESIAN_POINT('Ctrl Pts',(47.3796952654116,9.72714144142203,-47.8557565540428));
#50139=CARTESIAN_POINT('Ctrl Pts',(47.3853842139194,9.74340970086942,-48.335995883122));
#50140=CARTESIAN_POINT('Ctrl Pts',(47.3977916480236,9.78303804553009,-49.185160534592));
#50141=CARTESIAN_POINT('Ctrl Pts',(47.4212746322405,9.85897715801594,-50.4376674203479));
#50142=CARTESIAN_POINT('Ctrl Pts',(47.4556152568079,9.93497304216505,-51.9969760966932));
#50143=CARTESIAN_POINT('Ctrl Pts',(47.4811676044814,9.94145679742741,-53.0756574316043));
#50144=CARTESIAN_POINT('Ctrl Pts',(47.4976840347983,9.91961192914167,-53.7643743698396));
#50145=CARTESIAN_POINT('Ctrl Pts',(47.5049960739062,9.90437362808324,-54.069643578578));
#50146=CARTESIAN_POINT('Ctrl Pts',(47.5212002501635,9.85692668755594,-54.6481425932325));
#50147=CARTESIAN_POINT('Ctrl Pts',(47.5528019510802,9.73903591069576,-55.6302471286004));
#50148=CARTESIAN_POINT('Ctrl Pts',(47.6217691433342,9.43396909243672,-57.4389214989051));
#50149=CARTESIAN_POINT('Ctrl Pts',(47.6715736591803,9.27964416172965,-58.7268771422535));
#50150=CARTESIAN_POINT('Ctrl Pts',(47.6929289382822,9.32914414065638,-59.4924758815156));
#50151=CARTESIAN_POINT('Ctrl Pts',(47.6953084223224,9.33706414622836,-59.6060262207789));
#50152=CARTESIAN_POINT('Ctrl Pts',(47.6997399955762,9.35525736429222,-59.8224955049814));
#50153=CARTESIAN_POINT('Ctrl Pts',(47.7064814914924,9.39520989700813,-60.2091296542782));
#50154=CARTESIAN_POINT('Ctrl Pts',(47.7164083821879,9.50508439961949,-60.9858984347427));
#50155=CARTESIAN_POINT('Ctrl Pts',(47.7212347723481,9.69553200767656,-61.8916620069962));
#50156=CARTESIAN_POINT('Ctrl Pts',(47.7229811173075,9.94053973412928,-62.8062931149944));
#50157=CARTESIAN_POINT('Ctrl Pts',(47.7234538904886,10.0966356011433,-63.3236293982551));
#50158=CARTESIAN_POINT('Ctrl Pts',(47.7238251783761,10.2073953196583,-63.6690819228632));
#50159=CARTESIAN_POINT('Ctrl Pts',(47.7241044339201,10.2829556096916,-63.8995499207142));
#50160=CARTESIAN_POINT('Ctrl Pts',(47.7244634116366,10.3609734614794,-64.1300807060567));
#50161=CARTESIAN_POINT('Ctrl Pts',(47.7248880865451,10.4312491867597,-64.3319116549294));
#50162=CARTESIAN_POINT('Ctrl Pts',(47.7251694617457,10.471954805787,-64.4472559420996));
#50163=CARTESIAN_POINT('Ctrl Pts',(47.7256344500065,10.5335378042138,-64.6202526824162));
#50164=CARTESIAN_POINT('Ctrl Pts',(47.7261158818515,10.5859602740694,-64.7644468421099));
#50165=CARTESIAN_POINT('Ctrl Pts',(47.7270972701321,10.6738182258527,-65.0024966791782));
#50166=CARTESIAN_POINT('Ctrl Pts',(47.7292412577957,10.7564493085798,-65.2153400389283));
#50167=CARTESIAN_POINT('Ctrl Pts',(47.7324899373616,10.9453278605935,-65.6650772708215));
#50168=CARTESIAN_POINT('Ctrl Pts',(47.7374964661587,11.3131995151145,-66.4543190474403));
#50169=CARTESIAN_POINT('Ctrl Pts',(47.7426980816088,12.1924759235898,-68.0930375920078));
#50170=CARTESIAN_POINT('Ctrl Pts',(47.7397237287679,13.0906640581855,-69.587602268803));
#50171=CARTESIAN_POINT('Ctrl Pts',(47.7358536354079,13.7226246763649,-70.7892368292671));
#50172=CARTESIAN_POINT('Ctrl Pts',(47.7361736204316,13.8514600454724,-71.0337711059821));
#50173=CARTESIAN_POINT('Ctrl Pts',(47.7361291960693,14.1168018249454,-71.536283784416));
#50174=CARTESIAN_POINT('Ctrl Pts',(47.7363418421861,14.4467634673457,-72.158998942125));
#50175=CARTESIAN_POINT('Ctrl Pts',(47.7364213613972,14.8458003853794,-72.9096754717041));
#50176=CARTESIAN_POINT('Ctrl Pts',(47.7366172482031,15.6452858065704,-74.4101476191509));
#50177=CARTESIAN_POINT('Ctrl Pts',(47.7366332425202,16.315198688152,-75.662993732331));
#50178=CARTESIAN_POINT('Ctrl Pts',(47.7364484008569,17.2869467086366,-77.4904063862681));
#50179=CARTESIAN_POINT('Ctrl Pts',(47.7365301978728,17.7226365160067,-78.3096957673099));
#50180=CARTESIAN_POINT('Ctrl Pts',(47.7365301978729,18.1591581033962,-79.1306734694082));
#50181=CARTESIAN_POINT('Ctrl Pts',(50.4917922817391,5.17568235489026,24.8304882420805));
#50182=CARTESIAN_POINT('Ctrl Pts',(50.4919463673591,5.17569630217301,24.7816042480269));
#50183=CARTESIAN_POINT('Ctrl Pts',(50.4921079653614,5.17571093355396,24.7327213068017));
#50184=CARTESIAN_POINT('Ctrl Pts',(50.49401610954,5.17588375084432,24.1820554369562));
#50185=CARTESIAN_POINT('Ctrl Pts',(50.4955757902885,5.17595412085274,23.1778367254635));
#50186=CARTESIAN_POINT('Ctrl Pts',(50.4992711998872,5.17607766572335,21.1691325217455));
#50187=CARTESIAN_POINT('Ctrl Pts',(50.5119648081948,5.17722942219756,19.6648866682171));
#50188=CARTESIAN_POINT('Ctrl Pts',(50.5384011514674,5.17998292067282,18.413787630287));
#50189=CARTESIAN_POINT('Ctrl Pts',(50.5511164369398,5.18126936488514,17.910627519419));
#50190=CARTESIAN_POINT('Ctrl Pts',(50.5831063438728,5.18443886028894,16.9063830670091));
#50191=CARTESIAN_POINT('Ctrl Pts',(50.6516956130457,5.19124688005388,15.1526043614716));
#50192=CARTESIAN_POINT('Ctrl Pts',(50.7162903435254,5.19817646025032,13.6518036614801));
#50193=CARTESIAN_POINT('Ctrl Pts',(50.7557685599339,5.20338627675366,12.3986765425074));
#50194=CARTESIAN_POINT('Ctrl Pts',(50.7718008519029,5.20561383787571,11.8982690533153));
#50195=CARTESIAN_POINT('Ctrl Pts',(50.8041363870134,5.21047180505797,10.8972275154556));
#50196=CARTESIAN_POINT('Ctrl Pts',(50.8435837667984,5.21693603644432,9.64510071597907));
#50197=CARTESIAN_POINT('Ctrl Pts',(50.8846203402977,5.22422122892856,8.14041717856539));
#50198=CARTESIAN_POINT('Ctrl Pts',(50.9046159556434,5.22799629709726,7.13495554102581));
#50199=CARTESIAN_POINT('Ctrl Pts',(50.9138114954878,5.22978915534201,6.50646180185706));
#50200=CARTESIAN_POINT('Ctrl Pts',(50.9171497614407,5.23049291660771,6.25664748473695));
#50201=CARTESIAN_POINT('Ctrl Pts',(50.9226288259833,5.23185331422438,5.75587063687534));
#50202=CARTESIAN_POINT('Ctrl Pts',(50.9293284936965,5.23406903617317,4.87782255222184));
#50203=CARTESIAN_POINT('Ctrl Pts',(50.9331844612803,5.23762107699015,3.11689522340721));
#50204=CARTESIAN_POINT('Ctrl Pts',(50.9270757237267,5.23819298900028,1.60668800491269));
#50205=CARTESIAN_POINT('Ctrl Pts',(50.9248587722347,5.23662161216685,0.543497413880909));
#50206=CARTESIAN_POINT('Ctrl Pts',(50.9246333912762,5.23632273157213,0.414409441866805));
#50207=CARTESIAN_POINT('Ctrl Pts',(50.9243176736549,5.23531986251075,0.158287120738933));
#50208=CARTESIAN_POINT('Ctrl Pts',(50.9240633982016,5.23260278305952,-0.289084873984695));
#50209=CARTESIAN_POINT('Ctrl Pts',(50.924236551002,5.22653184322983,-0.923623408987164));
#50210=CARTESIAN_POINT('Ctrl Pts',(50.9242820186088,5.21760812954524,-1.6783329718768));
#50211=CARTESIAN_POINT('Ctrl Pts',(50.9227938318951,5.20583640270268,-2.67667968195561));
#50212=CARTESIAN_POINT('Ctrl Pts',(50.9155087270415,5.19591695372494,-3.91037106297294));
#50213=CARTESIAN_POINT('Ctrl Pts',(50.8985916819313,5.20214475796566,-4.8841803612588));
#50214=CARTESIAN_POINT('Ctrl Pts',(50.8828868788886,5.21330954430444,-5.49180684910913));
#50215=CARTESIAN_POINT('Ctrl Pts',(50.8764673354544,5.215033553012,-5.78755078053324));
#50216=CARTESIAN_POINT('Ctrl Pts',(50.8633859905258,5.20611621322098,-6.33245979971984));
#50217=CARTESIAN_POINT('Ctrl Pts',(50.8389770566919,5.16928155482403,-7.26301720700937));
#50218=CARTESIAN_POINT('Ctrl Pts',(50.7964827697425,5.10491128967598,-8.47107721615394));
#50219=CARTESIAN_POINT('Ctrl Pts',(50.7377218755804,5.12502850707293,-9.52925017206961));
#50220=CARTESIAN_POINT('Ctrl Pts',(50.6901697495722,5.2137233758942,-10.1916827055123));
#50221=CARTESIAN_POINT('Ctrl Pts',(50.662118172762,5.28912141861767,-10.5536869186764));
#50222=CARTESIAN_POINT('Ctrl Pts',(50.6478921279656,5.33596910600582,-10.7302411105224));
#50223=CARTESIAN_POINT('Ctrl Pts',(50.6371826404424,5.37485343867045,-10.8614554100438));
#50224=CARTESIAN_POINT('Ctrl Pts',(50.6307159721729,5.39705801614812,-10.9310818960025));
#50225=CARTESIAN_POINT('Ctrl Pts',(50.6154401332022,5.45490626609664,-11.0921354556276));
#50226=CARTESIAN_POINT('Ctrl Pts',(50.5846981114416,5.58090977361102,-11.3924344636096));
#50227=CARTESIAN_POINT('Ctrl Pts',(50.5066630577099,5.94058212465662,-12.0842817249592));
#50228=CARTESIAN_POINT('Ctrl Pts',(50.3578490121105,6.71358458556874,-13.2416724689023));
#50229=CARTESIAN_POINT('Ctrl Pts',(50.2065835518162,7.53232603473581,-14.4259820552415));
#50230=CARTESIAN_POINT('Ctrl Pts',(50.1139611608556,8.04584711163632,-15.2949612559555));
#50231=CARTESIAN_POINT('Ctrl Pts',(50.0564719102312,8.37311379279236,-15.900095054076));
#50232=CARTESIAN_POINT('Ctrl Pts',(50.0201438075105,8.59438581664167,-16.3873359291976));
#50233=CARTESIAN_POINT('Ctrl Pts',(49.9978240510594,8.75337087316149,-16.8152614588801));
#50234=CARTESIAN_POINT('Ctrl Pts',(49.9932719239137,8.80394733204392,-16.9530270287384));
#50235=CARTESIAN_POINT('Ctrl Pts',(49.9851495296652,8.90696100792097,-17.2462322364938));
#50236=CARTESIAN_POINT('Ctrl Pts',(49.9821302379449,9.00073505208439,-17.5314704398829));
#50237=CARTESIAN_POINT('Ctrl Pts',(49.9826393962094,9.08938550147516,-17.819049666724));
#50238=CARTESIAN_POINT('Ctrl Pts',(49.9845954418485,9.14189286236218,-17.9974335107659));
#50239=CARTESIAN_POINT('Ctrl Pts',(49.9869978917432,9.18249029971152,-18.1401049509871));
#50240=CARTESIAN_POINT('Ctrl Pts',(49.9892307552561,9.21215923530497,-18.2468571894993));
#50241=CARTESIAN_POINT('Ctrl Pts',(49.9914268319859,9.23627677705772,-18.3357024376677));
#50242=CARTESIAN_POINT('Ctrl Pts',(49.9933821403262,9.25520325252199,-18.4066777428617));
#50243=CARTESIAN_POINT('Ctrl Pts',(50.0110680129098,9.41401883658551,-19.0094610531942));
#50244=CARTESIAN_POINT('Ctrl Pts',(50.0792682289136,9.65255491121305,-20.1462575189252));
#50245=CARTESIAN_POINT('Ctrl Pts',(50.2091332895172,9.86433688529703,-21.7595264968037));
#50246=CARTESIAN_POINT('Ctrl Pts',(50.2674574528492,9.95568369829372,-22.7869865090925));
#50247=CARTESIAN_POINT('Ctrl Pts',(50.2825760832839,10.0117450467348,-23.4161246816041));
#50248=CARTESIAN_POINT('Ctrl Pts',(50.2875272443829,10.0339899843054,-23.705844706264));
#50249=CARTESIAN_POINT('Ctrl Pts',(50.2950269110892,10.0637741588356,-24.2559959869773));
#50250=CARTESIAN_POINT('Ctrl Pts',(50.3019274865117,10.0876891524349,-25.2161934049187));
#50251=CARTESIAN_POINT('Ctrl Pts',(50.297668864508,10.060160953794,-26.5368336469249));
#50252=CARTESIAN_POINT('Ctrl Pts',(50.2806400399388,9.99541428276367,-28.051138637435));
#50253=CARTESIAN_POINT('Ctrl Pts',(50.2704192293568,9.97068968221786,-29.0068078119763));
#50254=CARTESIAN_POINT('Ctrl Pts',(50.2680902577453,9.97170400042531,-29.5297903668874));
#50255=CARTESIAN_POINT('Ctrl Pts',(50.2675633128472,9.97203436851492,-29.6556098830141));
#50256=CARTESIAN_POINT('Ctrl Pts',(50.266354914397,9.97294138056059,-29.9020947112043));
#50257=CARTESIAN_POINT('Ctrl Pts',(50.2639105114052,9.9752324211205,-30.3367763830376));
#50258=CARTESIAN_POINT('Ctrl Pts',(50.2578839994032,9.98226236368177,-31.206406783758));
#50259=CARTESIAN_POINT('Ctrl Pts',(50.2473409278746,9.99796157371762,-32.4559954984309));
#50260=CARTESIAN_POINT('Ctrl Pts',(50.2376092948052,10.0167119816908,-33.7110935550376));
#50261=CARTESIAN_POINT('Ctrl Pts',(50.2322499145794,10.0303674776112,-34.7178088980314));
#50262=CARTESIAN_POINT('Ctrl Pts',(50.2306931834636,10.0362754548982,-35.2218816182731));
#50263=CARTESIAN_POINT('Ctrl Pts',(50.2300612982916,10.040109748401,-35.6010456515645));
#50264=CARTESIAN_POINT('Ctrl Pts',(50.2298010525293,10.042602014251,-35.8526947068551));
#50265=CARTESIAN_POINT('Ctrl Pts',(50.2298747170317,10.0474750052036,-36.356536925899));
#50266=CARTESIAN_POINT('Ctrl Pts',(50.2313887377468,10.0557642612372,-37.2361004289692));
#50267=CARTESIAN_POINT('Ctrl Pts',(50.2385455068631,10.0711028262601,-38.9908386578714));
#50268=CARTESIAN_POINT('Ctrl Pts',(50.2469303887032,10.0828908266136,-40.4936351840155));
#50269=CARTESIAN_POINT('Ctrl Pts',(50.2497861673699,10.0921244140975,-41.7505068669631));
#50270=CARTESIAN_POINT('Ctrl Pts',(50.2502702105738,10.0943027208078,-42.1293448835941));
#50271=CARTESIAN_POINT('Ctrl Pts',(50.2504294326418,10.0964052575757,-42.6323665495166));
#50272=CARTESIAN_POINT('Ctrl Pts',(50.250343076812,10.0981278236175,-43.1356412571861));
#50273=CARTESIAN_POINT('Ctrl Pts',(50.2499257473924,10.0997965195295,-43.7639609947201));
#50274=CARTESIAN_POINT('Ctrl Pts',(50.2494101467874,10.1017974964918,-44.5166494128688));
#50275=CARTESIAN_POINT('Ctrl Pts',(50.2493693574037,10.104099340921,-45.1422356819985));
#50276=CARTESIAN_POINT('Ctrl Pts',(50.249809185912,10.1066909341734,-45.6414808722959));
#50277=CARTESIAN_POINT('Ctrl Pts',(50.2504362280452,10.1091078188008,-46.0152243453922));
#50278=CARTESIAN_POINT('Ctrl Pts',(50.2514206232568,10.1120908343596,-46.3882409659662));
#50279=CARTESIAN_POINT('Ctrl Pts',(50.2532886632006,10.116950507721,-46.8844528098358));
#50280=CARTESIAN_POINT('Ctrl Pts',(50.25540923241,10.1217198984019,-47.2554383503514));
#50281=CARTESIAN_POINT('Ctrl Pts',(50.2581326010481,10.1274453409439,-47.6258728234225));
#50282=CARTESIAN_POINT('Ctrl Pts',(50.260107818025,10.1323681022638,-47.8613165863601));
#50283=CARTESIAN_POINT('Ctrl Pts',(50.2645300652927,10.1467153951326,-48.3447111522187));
#50284=CARTESIAN_POINT('Ctrl Pts',(50.2734586190813,10.1812210666923,-49.1988048899799));
#50285=CARTESIAN_POINT('Ctrl Pts',(50.289096735195,10.2454476087941,-50.4559708789396));
#50286=CARTESIAN_POINT('Ctrl Pts',(50.3113907758592,10.303771222499,-52.0172078681521));
#50287=CARTESIAN_POINT('Ctrl Pts',(50.3281951747258,10.2982140031211,-53.0944242249086));
#50288=CARTESIAN_POINT('Ctrl Pts',(50.3393348837964,10.2697154417897,-53.7813599592998));
#50289=CARTESIAN_POINT('Ctrl Pts',(50.3443475620727,10.2513279326554,-54.0881085257841));
#50290=CARTESIAN_POINT('Ctrl Pts',(50.3553654244131,10.1974224725376,-54.6678121480108));
#50291=CARTESIAN_POINT('Ctrl Pts',(50.3766105335714,10.0676138959923,-55.6516135370779));
#50292=CARTESIAN_POINT('Ctrl Pts',(50.422106002006,9.73901083306247,-57.4599799614481));
#50293=CARTESIAN_POINT('Ctrl Pts',(50.4518300690914,9.57152298929059,-58.7435487630709));
#50294=CARTESIAN_POINT('Ctrl Pts',(50.4673832424493,9.61678452934807,-59.5016760542654));
#50295=CARTESIAN_POINT('Ctrl Pts',(50.4691068208339,9.62413422649098,-59.6143692132953));
#50296=CARTESIAN_POINT('Ctrl Pts',(50.4724291890576,9.64137717775314,-59.8291956689248));
#50297=CARTESIAN_POINT('Ctrl Pts',(50.4777228802664,9.67998341820928,-60.2131942201998));
#50298=CARTESIAN_POINT('Ctrl Pts',(50.4865192303076,9.78848071124649,-60.9856468420894));
#50299=CARTESIAN_POINT('Ctrl Pts',(50.4930473652507,9.97985667703256,-61.8886735318654));
#50300=CARTESIAN_POINT('Ctrl Pts',(50.4975022393909,10.2272159581485,-62.8025747644526));
#50301=CARTESIAN_POINT('Ctrl Pts',(50.4995370799862,10.3849065774803,-63.3202082920092));
#50302=CARTESIAN_POINT('Ctrl Pts',(50.5008259755392,10.4967281288771,-63.6661400994148));
#50303=CARTESIAN_POINT('Ctrl Pts',(50.5016757912382,10.5729894359012,-63.8970034947931));
#50304=CARTESIAN_POINT('Ctrl Pts',(50.5025302150233,10.6516802926323,-64.1280375685076));
#50305=CARTESIAN_POINT('Ctrl Pts',(50.5032997606616,10.7225048544593,-64.3304078852364));
#50306=CARTESIAN_POINT('Ctrl Pts',(50.5037496849033,10.7635089449926,-64.4460882768762));
#50307=CARTESIAN_POINT('Ctrl Pts',(50.5044376473356,10.8255229325307,-64.6196163397289));
#50308=CARTESIAN_POINT('Ctrl Pts',(50.5050386966279,10.8782661361981,-64.7643128204007));
#50309=CARTESIAN_POINT('Ctrl Pts',(50.5061186304834,10.9665827412417,-65.0032530382309));
#50310=CARTESIAN_POINT('Ctrl Pts',(50.5086173349253,11.0493399786139,-65.2159941551862));
#50311=CARTESIAN_POINT('Ctrl Pts',(50.5123997427753,11.2386175512069,-65.6660613795346));
#50312=CARTESIAN_POINT('Ctrl Pts',(50.5183140141763,11.6069672647648,-66.4554986583973));
#50313=CARTESIAN_POINT('Ctrl Pts',(50.5247445762517,12.4868156446073,-68.0945711191323));
#50314=CARTESIAN_POINT('Ctrl Pts',(50.5217226319143,13.3848139405268,-69.5890289196084));
#50315=CARTESIAN_POINT('Ctrl Pts',(50.5172916352365,14.0166193126202,-70.7904864793872));
#50316=CARTESIAN_POINT('Ctrl Pts',(50.5176801339045,14.1454947301235,-71.0350483232966));
#50317=CARTESIAN_POINT('Ctrl Pts',(50.5176510909301,14.4108641406723,-71.5375759377691));
#50318=CARTESIAN_POINT('Ctrl Pts',(50.5179137443909,14.7408610844172,-72.1603179590527));
#50319=CARTESIAN_POINT('Ctrl Pts',(50.5180070923177,15.1399124031108,-72.9110139550441));
#50320=CARTESIAN_POINT('Ctrl Pts',(50.5182133876732,15.9394012467424,-74.4115156055686));
#50321=CARTESIAN_POINT('Ctrl Pts',(50.5181871982642,16.6092606723113,-75.6643418622959));
#50322=CARTESIAN_POINT('Ctrl Pts',(50.5179743581026,17.5809735969016,-77.4917026704339));
#50323=CARTESIAN_POINT('Ctrl Pts',(50.5180692026081,18.0166713543046,-78.3110028352501));
#50324=CARTESIAN_POINT('Ctrl Pts',(50.5180692026081,18.4531929416941,-79.1319805373485));
#50325=CARTESIAN_POINT('Ctrl Pts',(53.2695150563835,5.51412939726847,24.8304328418027));
#50326=CARTESIAN_POINT('Ctrl Pts',(53.2696688996589,5.51414443491013,24.7815471085002));
#50327=CARTESIAN_POINT('Ctrl Pts',(53.2698302575749,5.51416021237113,24.7326624174752));
#50328=CARTESIAN_POINT('Ctrl Pts',(53.2717355537201,5.51434666388,24.1819755549638));
#50329=CARTESIAN_POINT('Ctrl Pts',(53.2731190076681,5.51436686877321,23.1777004112197));
#50330=CARTESIAN_POINT('Ctrl Pts',(53.2762916814244,5.51433243053149,21.1689727072072));
#50331=CARTESIAN_POINT('Ctrl Pts',(53.2889745454163,5.51557857626836,19.6647602554609));
#50332=CARTESIAN_POINT('Ctrl Pts',(53.3162554220489,5.51883379753054,18.4137109770533));
#50333=CARTESIAN_POINT('Ctrl Pts',(53.3292888081772,5.52036031567856,17.9105682256386));
#50334=CARTESIAN_POINT('Ctrl Pts',(53.3619273956867,5.5241382069799,16.906316579728));
#50335=CARTESIAN_POINT('Ctrl Pts',(53.4319377194389,5.53228173032549,15.1524341677222));
#50336=CARTESIAN_POINT('Ctrl Pts',(53.4991258124589,5.54061652432534,13.6515381980859));
#50337=CARTESIAN_POINT('Ctrl Pts',(53.542473052396,5.54691456357747,12.3983966193952));
#50338=CARTESIAN_POINT('Ctrl Pts',(53.5603356607081,5.54961471051331,11.8979916029755));
#50339=CARTESIAN_POINT('Ctrl Pts',(53.5972024234654,5.55551879936049,10.897002135347));
#50340=CARTESIAN_POINT('Ctrl Pts',(53.6434512927629,5.56339708348542,9.64498895261323));
#50341=CARTESIAN_POINT('Ctrl Pts',(53.6928466346801,5.57224995798774,8.14041909589305));
#50342=CARTESIAN_POINT('Ctrl Pts',(53.7174864608606,5.57681098769189,7.13493855585078));
#50343=CARTESIAN_POINT('Ctrl Pts',(53.7289543784969,5.57895594316898,6.50639606605512));
#50344=CARTESIAN_POINT('Ctrl Pts',(53.7332399397066,5.57979684436249,6.25649768591037));
#50345=CARTESIAN_POINT('Ctrl Pts',(53.7407452387018,5.58140432867308,5.75560963473447));
#50346=CARTESIAN_POINT('Ctrl Pts',(53.7512130755125,5.58398764420394,4.87740710564012));
#50347=CARTESIAN_POINT('Ctrl Pts',(53.7625281946993,5.58799309354047,3.11630623138076));
#50348=CARTESIAN_POINT('Ctrl Pts',(53.7593283490689,5.58854306639946,1.60645823396047));
#50349=CARTESIAN_POINT('Ctrl Pts',(53.7543081104693,5.58680996580961,0.543452997857882));
#50350=CARTESIAN_POINT('Ctrl Pts',(53.7537151315514,5.58639943788977,0.412134805246649));
#50351=CARTESIAN_POINT('Ctrl Pts',(53.7525325840066,5.58484495007707,0.153207505278396));
#50352=CARTESIAN_POINT('Ctrl Pts',(53.7504298130056,5.58039238195928,-0.298852280230459));
#50353=CARTESIAN_POINT('Ctrl Pts',(53.7470896429771,5.57016836597694,-0.937114284333558));
#50354=CARTESIAN_POINT('Ctrl Pts',(53.7417739290271,5.55522922952095,-1.69238531231437));
#50355=CARTESIAN_POINT('Ctrl Pts',(53.7319395136192,5.53612531939417,-2.68582112449248));
#50356=CARTESIAN_POINT('Ctrl Pts',(53.7125866640681,5.52212017796381,-3.90307577254729));
#50357=CARTESIAN_POINT('Ctrl Pts',(53.6857013004841,5.53767860315604,-4.85280065205426));
#50358=CARTESIAN_POINT('Ctrl Pts',(53.6641830043257,5.56063240290011,-5.4420691309824));
#50359=CARTESIAN_POINT('Ctrl Pts',(53.6548139721549,5.56923331041967,-5.72862576373523));
#50360=CARTESIAN_POINT('Ctrl Pts',(53.6345170377436,5.57633161305388,-6.25852599704844));
#50361=CARTESIAN_POINT('Ctrl Pts',(53.5945971078396,5.57376225487845,-7.16757755734756));
#50362=CARTESIAN_POINT('Ctrl Pts',(53.5267535273497,5.56521492908129,-8.35957486081496));
#50363=CARTESIAN_POINT('Ctrl Pts',(53.4528066784746,5.63535903843469,-9.42461767107299));
#50364=CARTESIAN_POINT('Ctrl Pts',(53.4063264448625,5.75708558941193,-10.1070935533807));
#50365=CARTESIAN_POINT('Ctrl Pts',(53.3825855207646,5.85168431987466,-10.4839013761504));
#50366=CARTESIAN_POINT('Ctrl Pts',(53.3717711260772,5.9082780831659,-10.668762921667));
#50367=CARTESIAN_POINT('Ctrl Pts',(53.3641296138183,5.95448120662286,-10.8062514828049));
#50368=CARTESIAN_POINT('Ctrl Pts',(53.3609415101037,5.97947895554171,-10.8749525154684));
#50369=CARTESIAN_POINT('Ctrl Pts',(53.3525810895759,6.04538013200624,-11.037626473064));
#50370=CARTESIAN_POINT('Ctrl Pts',(53.3360567052155,6.18737340870044,-11.3401483424015));
#50371=CARTESIAN_POINT('Ctrl Pts',(53.2907506871901,6.5872514651254,-12.038539433205));
#50372=CARTESIAN_POINT('Ctrl Pts',(53.1925941608831,7.4250140432066,-13.204191553958));
#50373=CARTESIAN_POINT('Ctrl Pts',(53.0844762977564,8.2944695138769,-14.3991185169526));
#50374=CARTESIAN_POINT('Ctrl Pts',(53.0153923437052,8.83248777688499,-15.2830661152328));
#50375=CARTESIAN_POINT('Ctrl Pts',(52.9713518406644,9.17256455491026,-15.9017788862587));
#50376=CARTESIAN_POINT('Ctrl Pts',(52.9418943846209,9.3983203173646,-16.404501877126));
#50377=CARTESIAN_POINT('Ctrl Pts',(52.9220952320653,9.55509675497589,-16.8497512860891));
#50378=CARTESIAN_POINT('Ctrl Pts',(52.9170744783204,9.60547714751073,-16.9975381492885));
#50379=CARTESIAN_POINT('Ctrl Pts',(52.9076225110184,9.70397423114619,-17.3085087168662));
#50380=CARTESIAN_POINT('Ctrl Pts',(52.9014675276002,9.78896003877269,-17.6113587023661));
#50381=CARTESIAN_POINT('Ctrl Pts',(52.8975565743096,9.86463741111705,-17.9149028633213));
#50382=CARTESIAN_POINT('Ctrl Pts',(52.8961535288958,9.90755567793999,-18.1027394279948));
#50383=CARTESIAN_POINT('Ctrl Pts',(52.8955575391207,9.93964041294108,-18.2525370193699));
#50384=CARTESIAN_POINT('Ctrl Pts',(52.8953805694132,9.96253980574399,-18.3644296399647));
#50385=CARTESIAN_POINT('Ctrl Pts',(52.8954426432911,9.98071066858224,-18.4573752883049));
#50386=CARTESIAN_POINT('Ctrl Pts',(52.8956146345115,9.99470785692181,-18.5315144188974));
#50387=CARTESIAN_POINT('Ctrl Pts',(52.8977576515523,10.1107050642191,-19.1606209446941));
#50388=CARTESIAN_POINT('Ctrl Pts',(52.9225110046152,10.2395131612953,-20.3255595047088));
#50389=CARTESIAN_POINT('Ctrl Pts',(52.9776218232643,10.3008802158238,-21.9155284337944));
#50390=CARTESIAN_POINT('Ctrl Pts',(53.0035666335813,10.3301100096998,-22.889124084334));
#50391=CARTESIAN_POINT('Ctrl Pts',(53.0091514507972,10.3629588112806,-23.4703857380265));
#50392=CARTESIAN_POINT('Ctrl Pts',(53.0104509066303,10.376737772715,-23.7499115442637));
#50393=CARTESIAN_POINT('Ctrl Pts',(53.0116951558073,10.3951370917517,-24.2773902817673));
#50394=CARTESIAN_POINT('Ctrl Pts',(53.0098989792996,10.4107927229111,-25.2064856843808));
#50395=CARTESIAN_POINT('Ctrl Pts',(52.9996437044208,10.3962853899997,-26.5001577634974));
#50396=CARTESIAN_POINT('Ctrl Pts',(52.985573495527,10.3597651429066,-28.0151589056756));
#50397=CARTESIAN_POINT('Ctrl Pts',(52.9819354673514,10.3456237566901,-28.9932105392826));
#50398=CARTESIAN_POINT('Ctrl Pts',(52.9831672495963,10.3468226651521,-29.5345252208753));
#50399=CARTESIAN_POINT('Ctrl Pts',(52.9834618339309,10.3471246017814,-29.6607033909021));
#50400=CARTESIAN_POINT('Ctrl Pts',(52.984230858734,10.3478558390306,-29.9098655917076));
#50401=CARTESIAN_POINT('Ctrl Pts',(52.9859997430256,10.3494395327631,-30.3479071016356));
#50402=CARTESIAN_POINT('Ctrl Pts',(52.9910877275921,10.3536760394939,-31.2238536192905));
#50403=CARTESIAN_POINT('Ctrl Pts',(53.0018824045189,10.3617839853935,-32.4784261786044));
#50404=CARTESIAN_POINT('Ctrl Pts',(53.0150250933224,10.3703255534356,-33.7335695625717));
#50405=CARTESIAN_POINT('Ctrl Pts',(53.0255660425261,10.3763103895585,-34.7369580744697));
#50406=CARTESIAN_POINT('Ctrl Pts',(53.0306459750937,10.3788278479069,-35.2382903705776));
#50407=CARTESIAN_POINT('Ctrl Pts',(53.0343022880532,10.3804941335955,-35.6150223923661));
#50408=CARTESIAN_POINT('Ctrl Pts',(53.0368565578212,10.3816043729998,-35.8668683882239));
#50409=CARTESIAN_POINT('Ctrl Pts',(53.0423077317458,10.3837181513364,-36.3700419506216));
#50410=CARTESIAN_POINT('Ctrl Pts',(53.0526095271317,10.3872088831648,-37.2488784517629));
#50411=CARTESIAN_POINT('Ctrl Pts',(53.0749370713191,10.3934870690784,-39.0015781343972));
#50412=CARTESIAN_POINT('Ctrl Pts',(53.0927598271231,10.3985586653117,-40.5025012708411));
#50413=CARTESIAN_POINT('Ctrl Pts',(53.1020300932996,10.4033133844909,-41.7577923907435));
#50414=CARTESIAN_POINT('Ctrl Pts',(53.1043831419616,10.4041975940086,-42.1364495264179));
#50415=CARTESIAN_POINT('Ctrl Pts',(53.1068797929176,10.4046926600718,-42.6390036081494));
#50416=CARTESIAN_POINT('Ctrl Pts',(53.1090095338086,10.4048832049801,-43.1417926508615));
#50417=CARTESIAN_POINT('Ctrl Pts',(53.1110939742423,10.4048002178397,-43.7693855463974));
#50418=CARTESIAN_POINT('Ctrl Pts',(53.1130264615959,10.4050139698953,-44.5210345694311));
#50419=CARTESIAN_POINT('Ctrl Pts',(53.1144597922811,10.4061338634531,-45.1455962156924));
#50420=CARTESIAN_POINT('Ctrl Pts',(53.1156782935419,10.4079880616497,-45.6439451432393));
#50421=CARTESIAN_POINT('Ctrl Pts',(53.1166730225603,10.4099636011234,-46.0169683327606));
#50422=CARTESIAN_POINT('Ctrl Pts',(53.1177930906092,10.4126234963977,-46.3892183421306));
#50423=CARTESIAN_POINT('Ctrl Pts',(53.1195148227816,10.4172117803271,-46.884351859571));
#50424=CARTESIAN_POINT('Ctrl Pts',(53.1211258301745,10.4219833473072,-47.2544467632722));
#50425=CARTESIAN_POINT('Ctrl Pts',(53.1230500401165,10.4278371853805,-47.6239517433574));
#50426=CARTESIAN_POINT('Ctrl Pts',(53.12436166703,10.4328837420489,-47.8585839056701));
#50427=CARTESIAN_POINT('Ctrl Pts',(53.1269691023571,10.4477019749082,-48.3406195988866));
#50428=CARTESIAN_POINT('Ctrl Pts',(53.1315663929496,10.4835510487732,-49.1926272070234));
#50429=CARTESIAN_POINT('Ctrl Pts',(53.1383655351001,10.5511152764054,-50.4478347798509));
#50430=CARTESIAN_POINT('Ctrl Pts',(53.1479873645481,10.6147793240272,-52.0081718671275));
#50431=CARTESIAN_POINT('Ctrl Pts',(53.156447028726,10.6131912573835,-53.085717286359));
#50432=CARTESIAN_POINT('Ctrl Pts',(53.1629214165293,10.5870339863162,-53.7731140291621));
#50433=CARTESIAN_POINT('Ctrl Pts',(53.1659430409037,10.569810273764,-54.0790421421878));
#50434=CARTESIAN_POINT('Ctrl Pts',(53.1727564436081,10.5183244985191,-54.6579397162002));
#50435=CARTESIAN_POINT('Ctrl Pts',(53.1861233058401,10.3930525906094,-55.6406122873643));
#50436=CARTESIAN_POINT('Ctrl Pts',(53.2151846217902,10.0735258751026,-57.4487369102697));
#50437=CARTESIAN_POINT('Ctrl Pts',(53.2321543938323,9.91029533040072,-58.7350396653802));
#50438=CARTESIAN_POINT('Ctrl Pts',(53.243740090883,9.95716979747392,-59.4978810552022));
#50439=CARTESIAN_POINT('Ctrl Pts',(53.2449955793885,9.96473625601748,-59.6110245270641));
#50440=CARTESIAN_POINT('Ctrl Pts',(53.2475290643299,9.98235390960118,-59.8267667743487));
#50441=CARTESIAN_POINT('Ctrl Pts',(53.2517715992568,10.0215218737307,-60.2122127364834));
#50442=CARTESIAN_POINT('Ctrl Pts',(53.2596750196581,10.1307331248798,-60.9870643607676));
#50443=CARTESIAN_POINT('Ctrl Pts',(53.2672475158084,10.3220678340727,-61.8916255159988));
#50444=CARTESIAN_POINT('Ctrl Pts',(53.2735156455831,10.5687928930795,-62.8059939918394));
#50445=CARTESIAN_POINT('Ctrl Pts',(53.2766296476069,10.725990345077,-63.3235215809714));
#50446=CARTESIAN_POINT('Ctrl Pts',(53.2785685614647,10.8374653545796,-63.6692431125138));
#50447=CARTESIAN_POINT('Ctrl Pts',(53.2798277969375,10.9134935847789,-63.8999288216261));
#50448=CARTESIAN_POINT('Ctrl Pts',(53.2810447796835,10.9919538773434,-64.1307332047518));
#50449=CARTESIAN_POINT('Ctrl Pts',(53.2820765328361,11.0625855046011,-64.3328556288104));
#50450=CARTESIAN_POINT('Ctrl Pts',(53.2826580617144,11.103483121932,-64.4483814182979));
#50451=CARTESIAN_POINT('Ctrl Pts',(53.2835243590464,11.1653419503189,-64.6216651084278));
#50452=CARTESIAN_POINT('Ctrl Pts',(53.2842304329407,11.2179656495935,-64.7661305998104));
#50453=CARTESIAN_POINT('Ctrl Pts',(53.2854197490363,11.3061095226125,-65.0046642293767));
#50454=CARTESIAN_POINT('Ctrl Pts',(53.2882010693798,11.3889417772137,-65.2175224478048));
#50455=CARTESIAN_POINT('Ctrl Pts',(53.2924322715541,11.5782293927932,-65.6675133191105));
#50456=CARTESIAN_POINT('Ctrl Pts',(53.2991034786861,11.9466707796868,-66.4569647096837));
#50457=CARTESIAN_POINT('Ctrl Pts',(53.3065741614853,12.8266141431145,-68.0959329977427));
#50458=CARTESIAN_POINT('Ctrl Pts',(53.3034446514179,13.7246015455025,-69.5904384484924));
#50459=CARTESIAN_POINT('Ctrl Pts',(53.298454824434,14.3562318857571,-70.7919083359163));
#50460=CARTESIAN_POINT('Ctrl Pts',(53.2989019228725,14.4851096068852,-71.0364613092679));
#50461=CARTESIAN_POINT('Ctrl Pts',(53.2988790606072,14.7504636827547,-71.5389789626792));
#50462=CARTESIAN_POINT('Ctrl Pts',(53.2991825568548,15.0804570737878,-72.1617099472991));
#50463=CARTESIAN_POINT('Ctrl Pts',(53.2992890687305,15.4795056637326,-72.9123966172817));
#50464=CARTESIAN_POINT('Ctrl Pts',(53.2995141435576,16.2790023715052,-74.4128863212949));
#50465=CARTESIAN_POINT('Ctrl Pts',(53.2994612948345,16.9488827995346,-75.665724538253));
#50466=CARTESIAN_POINT('Ctrl Pts',(53.2992163810433,17.9206005062072,-77.4931099187158));
#50467=CARTESIAN_POINT('Ctrl Pts',(53.2993229371201,18.3562984860772,-78.312405584784));
#50468=CARTESIAN_POINT('Ctrl Pts',(53.29932293712,18.7928200734667,-79.1333832868824));
#50469=CARTESIAN_POINT('Ctrl Pts',(56.0538562954074,5.89165024012153,24.8309604003465));
#50470=CARTESIAN_POINT('Ctrl Pts',(56.0540116122581,5.89167990068842,24.7820913765585));
#50471=CARTESIAN_POINT('Ctrl Pts',(56.0541745295879,5.89171100104421,24.7332236978053));
#50472=CARTESIAN_POINT('Ctrl Pts',(56.0560981536171,5.89207817320162,24.1827331219404));
#50473=CARTESIAN_POINT('Ctrl Pts',(56.0573325828393,5.89247415459224,23.1786732167898));
#50474=CARTESIAN_POINT('Ctrl Pts',(56.0600534426369,5.89347092643402,21.1703130802733));
#50475=CARTESIAN_POINT('Ctrl Pts',(56.0728655050755,5.89590937649389,19.6662395446907));
#50476=CARTESIAN_POINT('Ctrl Pts',(56.1012316964193,5.90050969960956,18.4152728983411));
#50477=CARTESIAN_POINT('Ctrl Pts',(56.1147462351096,5.90279076485921,17.9132184233166));
#50478=CARTESIAN_POINT('Ctrl Pts',(56.1485361667684,5.90865570090384,16.9097331713725));
#50479=CARTESIAN_POINT('Ctrl Pts',(56.2210741679537,5.92123378561505,15.1557059965571));
#50480=CARTESIAN_POINT('Ctrl Pts',(56.2914134914659,5.93219694281183,13.6513343348583));
#50481=CARTESIAN_POINT('Ctrl Pts',(56.3380030057963,5.93721154809562,12.3936612477077));
#50482=CARTESIAN_POINT('Ctrl Pts',(56.3573126810151,5.93905485776692,11.8914244071032));
#50483=CARTESIAN_POINT('Ctrl Pts',(56.3975338417983,5.94215013443676,10.8877608718657));
#50484=CARTESIAN_POINT('Ctrl Pts',(56.4485948421275,5.94499428155967,9.63392266712354));
#50485=CARTESIAN_POINT('Ctrl Pts',(56.5038398846024,5.94702902649836,8.12966702503623));
#50486=CARTESIAN_POINT('Ctrl Pts',(56.5318786656771,5.9476348093116,7.12601654617415));
#50487=CARTESIAN_POINT('Ctrl Pts',(56.5451175184381,5.94783223170847,6.49903193976296));
#50488=CARTESIAN_POINT('Ctrl Pts',(56.5501450376796,5.94780846348296,6.24785780611247));
#50489=CARTESIAN_POINT('Ctrl Pts',(56.559241836301,5.94742736952047,5.74592863375821));
#50490=CARTESIAN_POINT('Ctrl Pts',(56.5726916525748,5.94601618318316,4.86637215456344));
#50491=CARTESIAN_POINT('Ctrl Pts',(56.5900048654683,5.94140601423123,3.10700589583077));
#50492=CARTESIAN_POINT('Ctrl Pts',(56.5895364791801,5.93821116463739,1.60556132597426));
#50493=CARTESIAN_POINT('Ctrl Pts',(56.5830907738242,5.94004214238158,0.551599771432738));
#50494=CARTESIAN_POINT('Ctrl Pts',(56.5823266484986,5.94002565977373,0.419000497013813));
#50495=CARTESIAN_POINT('Ctrl Pts',(56.580800409802,5.93910290897433,0.159135480437789));
#50496=CARTESIAN_POINT('Ctrl Pts',(56.5780725440921,5.93545041037213,-0.294580316420769));
#50497=CARTESIAN_POINT('Ctrl Pts',(56.5736645749159,5.9259217675061,-0.932794948601504));
#50498=CARTESIAN_POINT('Ctrl Pts',(56.5665312144104,5.91241497683955,-1.68514145248478));
#50499=CARTESIAN_POINT('Ctrl Pts',(56.5531776577419,5.8974933877812,-2.67026599152044));
#50500=CARTESIAN_POINT('Ctrl Pts',(56.5268416837315,5.8955788205326,-3.8692129523913));
#50501=CARTESIAN_POINT('Ctrl Pts',(56.4905108680574,5.93209099269583,-4.7958388535266));
#50502=CARTESIAN_POINT('Ctrl Pts',(56.4617001919105,5.9726109612883,-5.36829607916485));
#50503=CARTESIAN_POINT('Ctrl Pts',(56.4486050965068,5.99077468133528,-5.63962112151592));
#50504=CARTESIAN_POINT('Ctrl Pts',(56.4191070337447,6.02059082861141,-6.14825994930089));
#50505=CARTESIAN_POINT('Ctrl Pts',(56.3591906683692,6.06666028449872,-7.02774061874815));
#50506=CARTESIAN_POINT('Ctrl Pts',(56.258052074709,6.13755199903919,-8.20747819042182));
#50507=CARTESIAN_POINT('Ctrl Pts',(56.1585914012276,6.27717374595974,-9.30110347227688));
#50508=CARTESIAN_POINT('Ctrl Pts',(56.1031552157466,6.44038894773047,-10.0253563145223));
#50509=CARTESIAN_POINT('Ctrl Pts',(56.0772042357272,6.55677929476102,-10.4300198957996));
#50510=CARTESIAN_POINT('Ctrl Pts',(56.0663272930536,6.62350555199865,-10.6297806744373));
#50511=CARTESIAN_POINT('Ctrl Pts',(56.0590858017011,6.67694705514598,-10.7785470815969));
#50512=CARTESIAN_POINT('Ctrl Pts',(56.0572086293456,6.70556680595851,-10.8519969666275));
#50513=CARTESIAN_POINT('Ctrl Pts',(56.0515097738636,6.77914116439054,-11.0244233656895));
#50514=CARTESIAN_POINT('Ctrl Pts',(56.0411420905104,6.93302431413149,-11.3403871917385));
#50515=CARTESIAN_POINT('Ctrl Pts',(56.0119010310503,7.34960202239872,-12.0564238150741));
#50516=CARTESIAN_POINT('Ctrl Pts',(55.9423555314455,8.18633570232788,-13.2319459356605));
#50517=CARTESIAN_POINT('Ctrl Pts',(55.8606989766534,9.03446775281861,-14.4335826317914));
#50518=CARTESIAN_POINT('Ctrl Pts',(55.8078274105936,9.55305661363961,-15.323359668899));
#50519=CARTESIAN_POINT('Ctrl Pts',(55.773954709464,9.87868797757358,-15.9461193665655));
#50520=CARTESIAN_POINT('Ctrl Pts',(55.7512012634347,10.0918611128973,-16.4517402495332));
#50521=CARTESIAN_POINT('Ctrl Pts',(55.7358945084929,10.2373229525384,-16.8986727031992));
#50522=CARTESIAN_POINT('Ctrl Pts',(55.7320628041124,10.2851229032075,-17.0516780663757));
#50523=CARTESIAN_POINT('Ctrl Pts',(55.7251547347841,10.3759936592405,-17.3701166203036));
#50524=CARTESIAN_POINT('Ctrl Pts',(55.7211712881152,10.452196872169,-17.6808812380487));
#50525=CARTESIAN_POINT('Ctrl Pts',(55.7192131230406,10.5174898046456,-17.9910785587738));
#50526=CARTESIAN_POINT('Ctrl Pts',(55.7188977552019,10.5534715834494,-18.1828543478442));
#50527=CARTESIAN_POINT('Ctrl Pts',(55.7191039651392,10.5797214166711,-18.335541325308));
#50528=CARTESIAN_POINT('Ctrl Pts',(55.7194909678605,10.5981271124705,-18.4495004887757));
#50529=CARTESIAN_POINT('Ctrl Pts',(55.7199933559332,10.6124551659916,-18.5440686785368));
#50530=CARTESIAN_POINT('Ctrl Pts',(55.7204990192675,10.6233275116171,-18.6194481036827));
#50531=CARTESIAN_POINT('Ctrl Pts',(55.7253758088147,10.7124575844002,-19.2587758680929));
#50532=CARTESIAN_POINT('Ctrl Pts',(55.7522532141264,10.7815477183789,-20.4323773216303));
#50533=CARTESIAN_POINT('Ctrl Pts',(55.8031397938585,10.7627377228799,-22.0035158978069));
#50534=CARTESIAN_POINT('Ctrl Pts',(55.825737099881,10.7601510570931,-22.9452881163495));
#50535=CARTESIAN_POINT('Ctrl Pts',(55.8320950066742,10.782137854408,-23.5023779715933));
#50536=CARTESIAN_POINT('Ctrl Pts',(55.8340909980986,10.7915560371222,-23.7741616782038));
#50537=CARTESIAN_POINT('Ctrl Pts',(55.8372505969795,10.8051833217901,-24.2872868683742));
#50538=CARTESIAN_POINT('Ctrl Pts',(55.8404568442515,10.8197269207645,-25.1966898642464));
#50539=CARTESIAN_POINT('Ctrl Pts',(55.840087827842,10.8182318448034,-26.4760574343302));
#50540=CARTESIAN_POINT('Ctrl Pts',(55.8361433026693,10.8008785329893,-27.9945641694956));
#50541=CARTESIAN_POINT('Ctrl Pts',(55.834658027917,10.7916788201452,-28.9883692486796));
#50542=CARTESIAN_POINT('Ctrl Pts',(55.8352464030336,10.7906484334464,-29.5423588314564));
#50543=CARTESIAN_POINT('Ctrl Pts',(55.8353820157119,10.790377577361,-29.6692929526829));
#50544=CARTESIAN_POINT('Ctrl Pts',(55.8356247541215,10.7897068203214,-29.9209660665385));
#50545=CARTESIAN_POINT('Ctrl Pts',(55.8360007361368,10.7882119503876,-30.3624654127209));
#50546=CARTESIAN_POINT('Ctrl Pts',(55.8366037897902,10.7841005645739,-31.244305047108));
#50547=CARTESIAN_POINT('Ctrl Pts',(55.837392886965,10.7760252301369,-32.5030227351694));
#50548=CARTESIAN_POINT('Ctrl Pts',(55.8390037271353,10.7674769785333,-33.7573647708467));
#50549=CARTESIAN_POINT('Ctrl Pts',(55.8413101586343,10.7616974971422,-34.757077179787));
#50550=CARTESIAN_POINT('Ctrl Pts',(55.8428821540519,10.7594012798126,-35.255571422185));
#50551=CARTESIAN_POINT('Ctrl Pts',(55.8442554464811,10.7579659520475,-35.6298265937764));
#50552=CARTESIAN_POINT('Ctrl Pts',(55.8452792618007,10.7570014739844,-35.8817691950047));
#50553=CARTESIAN_POINT('Ctrl Pts',(55.8476951430184,10.7551262457876,-36.3841441827128));
#50554=CARTESIAN_POINT('Ctrl Pts',(55.8527414112041,10.7520089029467,-37.2620968637788));
#50555=CARTESIAN_POINT('Ctrl Pts',(55.8650741952096,10.7465773910564,-39.0126066758738));
#50556=CARTESIAN_POINT('Ctrl Pts',(55.8757055265642,10.744014883842,-40.5117095275918));
#50557=CARTESIAN_POINT('Ctrl Pts',(55.8804952904426,10.7437768053537,-41.7652712592726));
#50558=CARTESIAN_POINT('Ctrl Pts',(55.8815884039341,10.7432126106914,-42.1436772152057));
#50559=CARTESIAN_POINT('Ctrl Pts',(55.88255132219,10.7419325483112,-42.6456830734003));
#50560=CARTESIAN_POINT('Ctrl Pts',(55.8832415078542,10.7404472301093,-43.1479172097817));
#50561=CARTESIAN_POINT('Ctrl Pts',(55.883706560662,10.7384823465718,-43.7747209678689));
#50562=CARTESIAN_POINT('Ctrl Pts',(55.883986249836,10.736826384147,-44.5253077456604));
#50563=CARTESIAN_POINT('Ctrl Pts',(55.8842868961193,10.7367553253355,-45.1488783480515));
#50564=CARTESIAN_POINT('Ctrl Pts',(55.884752108554,10.7379140664082,-45.6463700676859));
#50565=CARTESIAN_POINT('Ctrl Pts',(55.8852567982933,10.7394977503655,-46.018718261597));
#50566=CARTESIAN_POINT('Ctrl Pts',(55.8859628356709,10.7419030693311,-46.3902611435584));
#50567=CARTESIAN_POINT('Ctrl Pts',(55.8872334971622,10.746345637622,-46.8844064295826));
#50568=CARTESIAN_POINT('Ctrl Pts',(55.888623767356,10.7512297242423,-47.2537105345762));
#50569=CARTESIAN_POINT('Ctrl Pts',(55.8904027456091,10.7573645699308,-47.6223775744809));
#50570=CARTESIAN_POINT('Ctrl Pts',(55.8916673641002,10.7626624185279,-47.8561843315716));
#50571=CARTESIAN_POINT('Ctrl Pts',(55.8943401260785,10.7782720818847,-48.3368618427273));
#50572=CARTESIAN_POINT('Ctrl Pts',(55.8994324357348,10.8161943746587,-49.1867388598945));
#50573=CARTESIAN_POINT('Ctrl Pts',(55.9078041596401,10.8884371599938,-50.4398661540837));
#50574=CARTESIAN_POINT('Ctrl Pts',(55.9200415336857,10.9593650678926,-51.9991864771287));
#50575=CARTESIAN_POINT('Ctrl Pts',(55.9304302925427,10.9627888364534,-53.077198113757));
#50576=CARTESIAN_POINT('Ctrl Pts',(55.9380573192689,10.9394594388728,-53.7652386011573));
#50577=CARTESIAN_POINT('Ctrl Pts',(55.9416089204399,10.9236075077244,-54.0703683356401));
#50578=CARTESIAN_POINT('Ctrl Pts',(55.9496284188782,10.8749406335218,-54.6485336841008));
#50579=CARTESIAN_POINT('Ctrl Pts',(55.9654007718481,10.7548844414289,-55.6301796463693));
#50580=CARTESIAN_POINT('Ctrl Pts',(55.9994801597755,10.4457295905618,-57.4383006955636));
#50581=CARTESIAN_POINT('Ctrl Pts',(56.0199751665574,10.2882719987063,-58.7271513010342));
#50582=CARTESIAN_POINT('Ctrl Pts',(56.0326904842793,10.337278922736,-59.4940543988374));
#50583=CARTESIAN_POINT('Ctrl Pts',(56.0340506213543,10.3451246445082,-59.6076251738527));
#50584=CARTESIAN_POINT('Ctrl Pts',(56.0367530445702,10.3632182368054,-59.8242094536169));
#50585=CARTESIAN_POINT('Ctrl Pts',(56.0411613373998,10.4030689516349,-60.210995835283));
#50586=CARTESIAN_POINT('Ctrl Pts',(56.0489566094561,10.5130336455672,-60.9880642774255));
#50587=CARTESIAN_POINT('Ctrl Pts',(56.0556887402585,10.7040394482772,-61.8940772156641));
#50588=CARTESIAN_POINT('Ctrl Pts',(56.0609545274981,10.9497688546937,-62.8089348476284));
#50589=CARTESIAN_POINT('Ctrl Pts',(56.063535498526,11.1062828232157,-63.3263977789393));
#50590=CARTESIAN_POINT('Ctrl Pts',(56.0651702598499,11.2173018665274,-63.6719400847196));
#50591=CARTESIAN_POINT('Ctrl Pts',(56.0662420948641,11.2930299821967,-63.9024701228049));
#50592=CARTESIAN_POINT('Ctrl Pts',(56.0673002598306,11.3712018859427,-64.133065809692));
#50593=CARTESIAN_POINT('Ctrl Pts',(56.0682223046878,11.4416005196807,-64.3349582563029));
#50594=CARTESIAN_POINT('Ctrl Pts',(56.0687505834134,11.4823719787838,-64.4503390882157));
#50595=CARTESIAN_POINT('Ctrl Pts',(56.0695468750535,11.5440494636025,-64.6233922442467));
#50596=CARTESIAN_POINT('Ctrl Pts',(56.07021642282,11.5965393493742,-64.7676365408963));
#50597=CARTESIAN_POINT('Ctrl Pts',(56.0713798269483,11.6844972675633,-65.0057761335482));
#50598=CARTESIAN_POINT('Ctrl Pts',(56.0742481638648,11.7673725945197,-65.2187440765607));
#50599=CARTESIAN_POINT('Ctrl Pts',(56.0786225888353,11.956626223471,-65.6686583942398));
#50600=CARTESIAN_POINT('Ctrl Pts',(56.0856207299876,12.325098293157,-66.4581217256169));
#50601=CARTESIAN_POINT('Ctrl Pts',(56.0937062273164,13.2050901989332,-68.0969928591841));
#50602=CARTESIAN_POINT('Ctrl Pts',(56.090624203504,14.1031075892701,-69.5915435266453));
#50603=CARTESIAN_POINT('Ctrl Pts',(56.0851893463343,14.7345980789755,-70.7930388880355));
#50604=CARTESIAN_POINT('Ctrl Pts',(56.0856673076515,14.8634752982914,-71.0375841108356));
#50605=CARTESIAN_POINT('Ctrl Pts',(56.0856335044423,15.1288146941014,-71.5400944851322));
#50606=CARTESIAN_POINT('Ctrl Pts',(56.0859568478666,15.4588035842588,-72.1628165081728));
#50607=CARTESIAN_POINT('Ctrl Pts',(56.0860723465189,15.8578497406362,-72.9134953028285));
#50608=CARTESIAN_POINT('Ctrl Pts',(56.0863258673364,16.657354734975,-74.4139738685058));
#50609=CARTESIAN_POINT('Ctrl Pts',(56.0862888584833,17.3272584591274,-75.6668214801239));
#50610=CARTESIAN_POINT('Ctrl Pts',(56.0860232991955,18.298981737646,-77.4942288106584));
#50611=CARTESIAN_POINT('Ctrl Pts',(56.0861395828494,18.7346801636112,-78.3135207979159));
#50612=CARTESIAN_POINT('Ctrl Pts',(56.0861395828494,19.1712017510007,-79.1344985000142));
#50613=CARTESIAN_POINT('Ctrl Pts',(58.8531048919552,6.29126117034768,24.8311270138471));
#50614=CARTESIAN_POINT('Ctrl Pts',(58.853288783423,6.29129935584637,24.7822631366728));
#50615=CARTESIAN_POINT('Ctrl Pts',(58.8534816497087,6.2913393689017,24.7334006343834));
#50616=CARTESIAN_POINT('Ctrl Pts',(58.8557584618987,6.29181245235756,24.1829722163064));
#50617=CARTESIAN_POINT('Ctrl Pts',(58.8576410777844,6.2924661188456,23.1790742508252));
#50618=CARTESIAN_POINT('Ctrl Pts',(58.8621221486529,6.29416752032691,21.1707865278706));
#50619=CARTESIAN_POINT('Ctrl Pts',(58.8772641083492,6.29730728170481,19.6666193118639));
#50620=CARTESIAN_POINT('Ctrl Pts',(58.9086867192454,6.30251976314054,18.4155160354777));
#50621=CARTESIAN_POINT('Ctrl Pts',(58.9238681411952,6.30510263301061,17.9134655130762));
#50622=CARTESIAN_POINT('Ctrl Pts',(58.9621931814769,6.31171912254366,16.9100353472743));
#50623=CARTESIAN_POINT('Ctrl Pts',(59.044403541375,6.32581484340266,15.1562873808193));
#50624=CARTESIAN_POINT('Ctrl Pts',(59.1211061781268,6.33775411577698,13.6520094580886));
#50625=CARTESIAN_POINT('Ctrl Pts',(59.1665661184318,6.3427083323814,12.3941538441954));
#50626=CARTESIAN_POINT('Ctrl Pts',(59.1848509216029,6.34443693178228,11.8918021760891));
#50627=CARTESIAN_POINT('Ctrl Pts',(59.2211705479974,6.347012855465,10.8878709549565));
#50628=CARTESIAN_POINT('Ctrl Pts',(59.2646739973078,6.34878292287888,9.63367636155125));
#50629=CARTESIAN_POINT('Ctrl Pts',(59.3092425919531,6.34933180168931,8.1292129060296));
#50630=CARTESIAN_POINT('Ctrl Pts',(59.3308039810503,6.34911032516135,7.12575148040342));
#50631=CARTESIAN_POINT('Ctrl Pts',(59.3407582844956,6.34895254139073,6.49900156323555));
#50632=CARTESIAN_POINT('Ctrl Pts',(59.3443009479904,6.3487870308239,6.2480976285954));
#50633=CARTESIAN_POINT('Ctrl Pts',(59.349863835633,6.34809587935646,5.74652248908033));
#50634=CARTESIAN_POINT('Ctrl Pts',(59.3559914845584,6.34610427421115,4.86750836522151));
#50635=CARTESIAN_POINT('Ctrl Pts',(59.3569458990738,6.34027728789477,3.10835172779085));
#50636=CARTESIAN_POINT('Ctrl Pts',(59.3490635616926,6.33670075767835,1.60628918930064));
#50637=CARTESIAN_POINT('Ctrl Pts',(59.3492784094883,6.33905879792391,0.550302612753713));
#50638=CARTESIAN_POINT('Ctrl Pts',(59.3495243001637,6.33896196490088,0.412614894001366));
#50639=CARTESIAN_POINT('Ctrl Pts',(59.3508389109231,6.33723377320785,0.146161885443116));
#50640=CARTESIAN_POINT('Ctrl Pts',(59.3550532176265,6.33072390632153,-0.318553477805038));
#50641=CARTESIAN_POINT('Ctrl Pts',(59.3652297576622,6.31399897839904,-0.965908052840755));
#50642=CARTESIAN_POINT('Ctrl Pts',(59.3798741113377,6.29000761912293,-1.72062652108147));
#50643=CARTESIAN_POINT('Ctrl Pts',(59.3971807795463,6.26259249771466,-2.69621161988787));
#50644=CARTESIAN_POINT('Ctrl Pts',(59.4043414085574,6.25497826476023,-3.85975006748727));
#50645=CARTESIAN_POINT('Ctrl Pts',(59.3733146100403,6.3105312327679,-4.73293165960504));
#50646=CARTESIAN_POINT('Ctrl Pts',(59.3363575784456,6.37295188297166,-5.26473353177676));
#50647=CARTESIAN_POINT('Ctrl Pts',(59.3183418149714,6.40289994227644,-5.50595486139798));
#50648=CARTESIAN_POINT('Ctrl Pts',(59.2730388009056,6.46480431714097,-5.97081755510265));
#50649=CARTESIAN_POINT('Ctrl Pts',(59.1724422888517,6.58535278710391,-6.78943021470857));
#50650=CARTESIAN_POINT('Ctrl Pts',(58.9912262531475,6.7868229657027,-7.94612904489456));
#50651=CARTESIAN_POINT('Ctrl Pts',(58.8223317891728,7.04771908873206,-9.10212973186673));
#50652=CARTESIAN_POINT('Ctrl Pts',(58.735697291889,7.28300208313501,-9.90635004105204));
#50653=CARTESIAN_POINT('Ctrl Pts',(58.6977351168525,7.43540237400419,-10.3634058429054));
#50654=CARTESIAN_POINT('Ctrl Pts',(58.6830346418896,7.51810068114256,-10.591111217551));
#50655=CARTESIAN_POINT('Ctrl Pts',(58.6738634777459,7.58260836432584,-10.761190612064));
#50656=CARTESIAN_POINT('Ctrl Pts',(58.6723346369094,7.6173239321139,-10.8453845146161));
#50657=CARTESIAN_POINT('Ctrl Pts',(58.6676689607852,7.70233593977603,-11.0379844018061));
#50658=CARTESIAN_POINT('Ctrl Pts',(58.6622876768978,7.87158105335511,-11.3815342433213));
#50659=CARTESIAN_POINT('Ctrl Pts',(58.6531725345026,8.29795340172989,-12.1307881868699));
#50660=CARTESIAN_POINT('Ctrl Pts',(58.6343507387422,9.0888204052782,-13.3224315637315));
#50661=CARTESIAN_POINT('Ctrl Pts',(58.6088503070498,9.85801911386535,-14.5331952917628));
#50662=CARTESIAN_POINT('Ctrl Pts',(58.5920713303508,10.3189685137634,-15.4243151261943));
#50663=CARTESIAN_POINT('Ctrl Pts',(58.5810899924814,10.6052359649885,-16.0452514748664));
#50664=CARTESIAN_POINT('Ctrl Pts',(58.5733938621257,10.7885227068715,-16.5448452975907));
#50665=CARTESIAN_POINT('Ctrl Pts',(58.5676247829872,10.911110806863,-16.9819314237086));
#50666=CARTESIAN_POINT('Ctrl Pts',(58.566515134249,10.9530822623337,-17.1389501191447));
#50667=CARTESIAN_POINT('Ctrl Pts',(58.5650823700106,11.0297845914177,-17.4602983187608));
#50668=CARTESIAN_POINT('Ctrl Pts',(58.5655994643091,11.0918640608194,-17.7749969970167));
#50669=CARTESIAN_POINT('Ctrl Pts',(58.567479755255,11.1421871122659,-18.0874443318188));
#50670=CARTESIAN_POINT('Ctrl Pts',(58.5692257607602,11.1687651072572,-18.2805138718139));
#50671=CARTESIAN_POINT('Ctrl Pts',(58.5709066006215,11.1874061276119,-18.4339668965554));
#50672=CARTESIAN_POINT('Ctrl Pts',(58.5723068416036,11.2000958147659,-18.5484262892516));
#50673=CARTESIAN_POINT('Ctrl Pts',(58.5735810792346,11.2096476662046,-18.6433263639815));
#50674=CARTESIAN_POINT('Ctrl Pts',(58.5746599324514,11.2166987397609,-18.7189271165951));
#50675=CARTESIAN_POINT('Ctrl Pts',(58.5841803354795,11.2733312266439,-19.3598937336237));
#50676=CARTESIAN_POINT('Ctrl Pts',(58.6120243623537,11.2811438472495,-20.5284346164844));
#50677=CARTESIAN_POINT('Ctrl Pts',(58.6548556526593,11.1940216759872,-22.0799936426061));
#50678=CARTESIAN_POINT('Ctrl Pts',(58.6749787296748,11.1632014021287,-23.0022998186139));
#50679=CARTESIAN_POINT('Ctrl Pts',(58.6826373505566,11.1724781990788,-23.5437147825256));
#50680=CARTESIAN_POINT('Ctrl Pts',(58.6852936633433,11.1764569534577,-23.8091597735434));
#50681=CARTESIAN_POINT('Ctrl Pts',(58.6897313102728,11.1821520504571,-24.3109583800983));
#50682=CARTESIAN_POINT('Ctrl Pts',(58.6951496568698,11.18811730114,-25.2033062990913));
#50683=CARTESIAN_POINT('Ctrl Pts',(58.6975113593674,11.1872479676171,-26.4667513104716));
#50684=CARTESIAN_POINT('Ctrl Pts',(58.6954851864191,11.1799618969185,-27.9801788785804));
#50685=CARTESIAN_POINT('Ctrl Pts',(58.6933663086165,11.1760448864423,-28.9802073808478));
#50686=CARTESIAN_POINT('Ctrl Pts',(58.6925291563035,11.1756400017411,-29.54013772036));
#50687=CARTESIAN_POINT('Ctrl Pts',(58.6922950590304,11.1755342273211,-29.6661205159246));
#50688=CARTESIAN_POINT('Ctrl Pts',(58.6916838214696,11.175261758783,-29.9172281844278));
#50689=CARTESIAN_POINT('Ctrl Pts',(58.6902528492363,11.1746278716065,-30.3572248042373));
#50690=CARTESIAN_POINT('Ctrl Pts',(58.686156011812,11.1728135218474,-31.237075055171));
#50691=CARTESIAN_POINT('Ctrl Pts',(58.6779244362639,11.1690434128148,-32.4940740070076));
#50692=CARTESIAN_POINT('Ctrl Pts',(58.6696380838126,11.1648456735736,-33.7486968816292));
#50693=CARTESIAN_POINT('Ctrl Pts',(58.6648548738614,11.162001808617,-34.7497098307469));
#50694=CARTESIAN_POINT('Ctrl Pts',(58.6633983437453,11.1608703557711,-35.2492405539033));
#50695=CARTESIAN_POINT('Ctrl Pts',(58.6627726971019,11.1601841652618,-35.6244027444587));
#50696=CARTESIAN_POINT('Ctrl Pts',(58.6624681048258,11.1597282059655,-35.8763034515194));
#50697=CARTESIAN_POINT('Ctrl Pts',(58.662267318025,11.1588190707973,-36.3789711970892));
#50698=CARTESIAN_POINT('Ctrl Pts',(58.6628639022804,11.1572820747005,-37.2572499766015));
#50699=CARTESIAN_POINT('Ctrl Pts',(58.6668824890188,11.1545806575703,-39.0086150002578));
#50700=CARTESIAN_POINT('Ctrl Pts',(58.6718031114793,11.1537637365605,-40.508386452936));
#50701=CARTESIAN_POINT('Ctrl Pts',(58.6730165686399,11.1546710008935,-41.7625412307252));
#50702=CARTESIAN_POINT('Ctrl Pts',(58.6731074510399,11.1544438395403,-42.1409999055361));
#50703=CARTESIAN_POINT('Ctrl Pts',(58.6728673574289,11.1535770440756,-42.6431794169131));
#50704=CARTESIAN_POINT('Ctrl Pts',(58.6724461101439,11.1524856555828,-43.1455918732114));
#50705=CARTESIAN_POINT('Ctrl Pts',(58.6716936934682,11.1509666828279,-43.7726690093924));
#50706=CARTESIAN_POINT('Ctrl Pts',(58.6707929708391,11.1497603315992,-44.52365118088));
#50707=CARTESIAN_POINT('Ctrl Pts',(58.6703480265652,11.1499817126121,-45.147614397289));
#50708=CARTESIAN_POINT('Ctrl Pts',(58.670359448683,11.1513089229432,-45.6454614270176));
#50709=CARTESIAN_POINT('Ctrl Pts',(58.6705970894054,11.152989107669,-46.018095499028));
#50710=CARTESIAN_POINT('Ctrl Pts',(58.6711096924726,11.1554586142605,-46.3899437030966));
#50711=CARTESIAN_POINT('Ctrl Pts',(58.6722217573552,11.1599390035811,-46.8845233225911));
#50712=CARTESIAN_POINT('Ctrl Pts',(58.6736050980711,11.1648026318779,-47.2541803983589));
#50713=CARTESIAN_POINT('Ctrl Pts',(58.6754544191834,11.1708724187996,-47.6232252559624));
#50714=CARTESIAN_POINT('Ctrl Pts',(58.6768261977709,11.1761194371953,-47.8573849835496));
#50715=CARTESIAN_POINT('Ctrl Pts',(58.6799052267683,11.1915668487932,-48.3386403067271));
#50716=CARTESIAN_POINT('Ctrl Pts',(58.6861582569438,11.2290588435075,-49.1893944317329));
#50717=CARTESIAN_POINT('Ctrl Pts',(58.6971032883846,11.3002628695192,-50.4432920806055));
#50718=CARTESIAN_POINT('Ctrl Pts',(58.7128620077876,11.3693893217062,-52.0028627018444));
#50719=CARTESIAN_POINT('Ctrl Pts',(58.7252444156214,11.3714512484384,-53.0805961140929));
#50720=CARTESIAN_POINT('Ctrl Pts',(58.7338153696161,11.347301218749,-53.76834192412));
#50721=CARTESIAN_POINT('Ctrl Pts',(58.7377766840328,11.3310354824593,-54.0737103110201));
#50722=CARTESIAN_POINT('Ctrl Pts',(58.7466284819545,11.2815142239099,-54.6520866627448));
#50723=CARTESIAN_POINT('Ctrl Pts',(58.7638687059199,11.1598471258297,-55.6340650974073));
#50724=CARTESIAN_POINT('Ctrl Pts',(58.800567281988,10.8473227536876,-57.4423158425765));
#50725=CARTESIAN_POINT('Ctrl Pts',(58.8224426358845,10.6879399518963,-58.7303538545682));
#50726=CARTESIAN_POINT('Ctrl Pts',(58.8355451088492,10.7362905625105,-59.4957112097895));
#50727=CARTESIAN_POINT('Ctrl Pts',(58.8369437008818,10.7440442698396,-59.6091146653755));
#50728=CARTESIAN_POINT('Ctrl Pts',(58.8396933622305,10.7619811815525,-59.8253728659405));
#50729=CARTESIAN_POINT('Ctrl Pts',(58.8441090309769,10.8015995672414,-60.2116412498697));
#50730=CARTESIAN_POINT('Ctrl Pts',(58.8516532452224,10.9112843858518,-60.9878681974567));
#50731=CARTESIAN_POINT('Ctrl Pts',(58.8576498131029,11.1023498914853,-61.8933793937477));
#50732=CARTESIAN_POINT('Ctrl Pts',(58.862065588882,11.348390653275,-62.8081425766873));
#50733=CARTESIAN_POINT('Ctrl Pts',(58.8641851331624,11.5051348146818,-63.3256911177079));
#50734=CARTESIAN_POINT('Ctrl Pts',(58.8655431183583,11.6163140515013,-63.6713440824319));
#50735=CARTESIAN_POINT('Ctrl Pts',(58.8664403305124,11.6921494967269,-63.9019619108394));
#50736=CARTESIAN_POINT('Ctrl Pts',(58.8673404322247,11.7704270793534,-64.1326656001653));
#50737=CARTESIAN_POINT('Ctrl Pts',(58.8681432316335,11.8409141347406,-64.3346702081786));
#50738=CARTESIAN_POINT('Ctrl Pts',(58.8686092840971,11.881734392604,-64.4501200906322));
#50739=CARTESIAN_POINT('Ctrl Pts',(58.869318507385,11.9434830759097,-64.6232815853475));
#50740=CARTESIAN_POINT('Ctrl Pts',(58.8699286517978,11.9960274978391,-64.7676265626046));
#50741=CARTESIAN_POINT('Ctrl Pts',(58.8710157569687,12.0840658209306,-65.0059424367529));
#50742=CARTESIAN_POINT('Ctrl Pts',(58.8738589421922,12.1669604684609,-65.2188979516415));
#50743=CARTESIAN_POINT('Ctrl Pts',(58.8781893104489,12.3562843388777,-65.6688870066509));
#50744=CARTESIAN_POINT('Ctrl Pts',(58.8851906494169,12.7248466273555,-66.4584035251456));
#50745=CARTESIAN_POINT('Ctrl Pts',(58.8934443763777,13.6049670574308,-68.0973570342353));
#50746=CARTESIAN_POINT('Ctrl Pts',(58.8905062211977,14.5029656194648,-69.5918838038918));
#50747=CARTESIAN_POINT('Ctrl Pts',(58.8849459593989,15.1344155593395,-70.7933399329592));
#50748=CARTESIAN_POINT('Ctrl Pts',(58.8854298430313,15.2633013275615,-71.0378917525492));
#50749=CARTESIAN_POINT('Ctrl Pts',(58.8853901310312,15.5286459532577,-71.540405931102));
#50750=CARTESIAN_POINT('Ctrl Pts',(58.8857159790617,15.8586422053525,-72.163134336603));
#50751=CARTESIAN_POINT('Ctrl Pts',(58.885832972894,16.2576915358115,-72.9138175400082));
#50752=CARTESIAN_POINT('Ctrl Pts',(58.8860950426403,17.0571981277039,-74.4143023315381));
#50753=CARTESIAN_POINT('Ctrl Pts',(58.8860657223544,17.7270914913872,-75.6671445469792));
#50754=CARTESIAN_POINT('Ctrl Pts',(58.8857948969183,18.6988067501922,-77.4945402056233));
#50755=CARTESIAN_POINT('Ctrl Pts',(58.8859129594251,19.1345069619474,-78.3138346232385));
#50756=CARTESIAN_POINT('Ctrl Pts',(58.8859129594252,19.5710285493368,-79.1348123253369));
#50757=CARTESIAN_POINT('Ctrl Pts',(61.1951430599348,6.62459351860839,24.8301566171112));
#50758=CARTESIAN_POINT('Ctrl Pts',(61.1953495829341,6.62461118340833,24.7812622509577));
#50759=CARTESIAN_POINT('Ctrl Pts',(61.1955661714496,6.62462972912612,24.7323686772253));
#50760=CARTESIAN_POINT('Ctrl Pts',(61.1981226275006,6.62484834924031,24.1815830296665));
#50761=CARTESIAN_POINT('Ctrl Pts',(61.200552546657,6.62487504513224,23.1773159143136));
#50762=CARTESIAN_POINT('Ctrl Pts',(61.2065289204206,6.62485044255725,21.1683500346935));
#50763=CARTESIAN_POINT('Ctrl Pts',(61.2235206228691,6.6263073739822,19.6639179088845));
#50764=CARTESIAN_POINT('Ctrl Pts',(61.2571976857159,6.63009622317173,18.4126432827115));
#50765=CARTESIAN_POINT('Ctrl Pts',(61.2735402762306,6.63178859409188,17.9085730154883));
#50766=CARTESIAN_POINT('Ctrl Pts',(61.3149072476585,6.63580631603488,16.9037326109381));
#50767=CARTESIAN_POINT('Ctrl Pts',(61.4035013072067,6.6443874466591,15.1503002603318));
#50768=CARTESIAN_POINT('Ctrl Pts',(61.4848249365008,6.65408168458786,13.6525508282425));
#50769=CARTESIAN_POINT('Ctrl Pts',(61.5305594648357,6.66308696916894,12.4031116832484));
#50770=CARTESIAN_POINT('Ctrl Pts',(61.5486814066148,6.66709153838059,11.9041991676416));
#50771=CARTESIAN_POINT('Ctrl Pts',(61.5837588738223,6.67629259873839,10.9052363266201));
#50772=CARTESIAN_POINT('Ctrl Pts',(61.6244364766192,6.68920666605379,9.65440342433843));
#50773=CARTESIAN_POINT('Ctrl Pts',(61.6644897802702,6.7043024031215,8.14923390352158));
#50774=CARTESIAN_POINT('Ctrl Pts',(61.6830749181458,6.71236791277641,7.14232597420164));
#50775=CARTESIAN_POINT('Ctrl Pts',(61.6913383718123,6.71624608706999,6.51262594167426));
#50776=CARTESIAN_POINT('Ctrl Pts',(61.69414610316,6.71780214827397,6.26370524403605));
#50777=CARTESIAN_POINT('Ctrl Pts',(61.6980214561424,6.72094132003559,5.76362531772536));
#50778=CARTESIAN_POINT('Ctrl Pts',(61.7007450863805,6.72636327795744,4.8866659505902));
#50779=CARTESIAN_POINT('Ctrl Pts',(61.6938174291058,6.73605603354009,3.12445746403));
#50780=CARTESIAN_POINT('Ctrl Pts',(61.6803461765711,6.73881989834997,1.61004654781063));
#50781=CARTESIAN_POINT('Ctrl Pts',(61.6804493960782,6.73532109511675,0.538275827822303));
#50782=CARTESIAN_POINT('Ctrl Pts',(61.6808101793117,6.73401731235922,0.391744046227261));
#50783=CARTESIAN_POINT('Ctrl Pts',(61.6827543160363,6.72849797514263,0.11292533490665));
#50784=CARTESIAN_POINT('Ctrl Pts',(61.6890248659479,6.71203304004211,-0.372274787302301));
#50785=CARTESIAN_POINT('Ctrl Pts',(61.7040904305426,6.67419733781364,-1.03825243668594));
#50786=CARTESIAN_POINT('Ctrl Pts',(61.7258780777276,6.62118416234288,-1.80127297542329));
#50787=CARTESIAN_POINT('Ctrl Pts',(61.7520928872156,6.55737622968081,-2.76765400835207));
#50788=CARTESIAN_POINT('Ctrl Pts',(61.7660952010983,6.52136939127453,-3.8821518154703));
#50789=CARTESIAN_POINT('Ctrl Pts',(61.729067495728,6.58516251664634,-4.67513771827723));
#50790=CARTESIAN_POINT('Ctrl Pts',(61.6839343104004,6.66311971581696,-5.14899657540951));
#50791=CARTESIAN_POINT('Ctrl Pts',(61.6617387075409,6.70034156427653,-5.35025911829331));
#50792=CARTESIAN_POINT('Ctrl Pts',(61.6046402242691,6.78918160908311,-5.75878526406458));
#50793=CARTESIAN_POINT('Ctrl Pts',(61.4765501720259,6.98331289136561,-6.50476976133261));
#50794=CARTESIAN_POINT('Ctrl Pts',(61.2474997672193,7.35403276894785,-7.64853950979505));
#50795=CARTESIAN_POINT('Ctrl Pts',(61.0315326652427,7.812434998521,-8.88214138951066));
#50796=CARTESIAN_POINT('Ctrl Pts',(60.9164087838436,8.15957649757144,-9.77875658120804));
#50797=CARTESIAN_POINT('Ctrl Pts',(60.8649434387047,8.36254780943143,-10.2990968288097));
#50798=CARTESIAN_POINT('Ctrl Pts',(60.8446861618763,8.46524558357949,-10.5620869355828));
#50799=CARTESIAN_POINT('Ctrl Pts',(60.8319717937481,8.54250760013033,-10.7601063274006));
#50800=CARTESIAN_POINT('Ctrl Pts',(60.8294620303259,8.5844566328175,-10.8601436322418));
#50801=CARTESIAN_POINT('Ctrl Pts',(60.8233921158387,8.68113683502462,-11.0820780579105));
#50802=CARTESIAN_POINT('Ctrl Pts',(60.8191540441179,8.86227482615309,-11.4680942275968));
#50803=CARTESIAN_POINT('Ctrl Pts',(60.8257513025041,9.27903522043605,-12.2748548396355));
#50804=CARTESIAN_POINT('Ctrl Pts',(60.8668397300883,9.97140776595471,-13.5004881682362));
#50805=CARTESIAN_POINT('Ctrl Pts',(60.91809750942,10.5941498479321,-14.7188381694371));
#50806=CARTESIAN_POINT('Ctrl Pts',(60.9479629679688,10.953166600623,-15.5959303525026));
#50807=CARTESIAN_POINT('Ctrl Pts',(60.9654273466163,11.1726390509724,-16.1995991182255));
#50808=CARTESIAN_POINT('Ctrl Pts',(60.9746817698278,11.3095967394032,-16.674774647252));
#50809=CARTESIAN_POINT('Ctrl Pts',(60.9784785963746,11.4012776811817,-17.082927036861));
#50810=CARTESIAN_POINT('Ctrl Pts',(60.9801506660244,11.4345556346319,-17.2394288135314));
#50811=CARTESIAN_POINT('Ctrl Pts',(60.9835902396351,11.493131799317,-17.5529833462735));
#50812=CARTESIAN_POINT('Ctrl Pts',(60.9872151786763,11.5395393577809,-17.8619373863565));
#50813=CARTESIAN_POINT('Ctrl Pts',(60.9908320118966,11.57551979552,-18.1673014652789));
#50814=CARTESIAN_POINT('Ctrl Pts',(60.9930796103776,11.5938996693051,-18.3562408564781));
#50815=CARTESIAN_POINT('Ctrl Pts',(60.9948531119313,11.6063443310479,-18.5063169153956));
#50816=CARTESIAN_POINT('Ctrl Pts',(60.9961699597551,11.6145865427258,-18.6182943335112));
#50817=CARTESIAN_POINT('Ctrl Pts',(60.9972543385166,11.6205841104154,-18.7111372183144));
#50818=CARTESIAN_POINT('Ctrl Pts',(60.9981121879651,11.6248839498187,-18.7851145838485));
#50819=CARTESIAN_POINT('Ctrl Pts',(61.0053617468449,11.6586247888096,-19.4123376454189));
#50820=CARTESIAN_POINT('Ctrl Pts',(61.0172652635169,11.638506103459,-20.5587287497834));
#50821=CARTESIAN_POINT('Ctrl Pts',(61.0268712384702,11.5302675454384,-22.0960102293423));
#50822=CARTESIAN_POINT('Ctrl Pts',(61.0305990851216,11.4890734836909,-23.0203699506435));
#50823=CARTESIAN_POINT('Ctrl Pts',(61.0339916227849,11.4918641686232,-23.5668462678014));
#50824=CARTESIAN_POINT('Ctrl Pts',(61.0351944413737,11.4929251983715,-23.8277092582862));
#50825=CARTESIAN_POINT('Ctrl Pts',(61.037153140714,11.4943502477889,-24.3247189869738));
#50826=CARTESIAN_POINT('Ctrl Pts',(61.0394974963756,11.4954093598254,-25.2082732613028));
#50827=CARTESIAN_POINT('Ctrl Pts',(61.040290778228,11.4936881528447,-26.4644309696059));
#50828=CARTESIAN_POINT('Ctrl Pts',(61.0387579071437,11.4898327101281,-27.9743589344223));
#50829=CARTESIAN_POINT('Ctrl Pts',(61.0372909646032,11.4884279010678,-28.9761098417619));
#50830=CARTESIAN_POINT('Ctrl Pts',(61.0367222294322,11.4886071465497,-29.5380249988527));
#50831=CARTESIAN_POINT('Ctrl Pts',(61.0365763771857,11.4886536420874,-29.6633057425343));
#50832=CARTESIAN_POINT('Ctrl Pts',(61.036197723935,11.4887692768465,-29.9137065824811));
#50833=CARTESIAN_POINT('Ctrl Pts',(61.0353289370354,11.4890318207177,-30.3522566304998));
#50834=CARTESIAN_POINT('Ctrl Pts',(61.0328937905285,11.4897738835658,-31.2299465515799));
#50835=CARTESIAN_POINT('Ctrl Pts',(61.0281756870949,11.4913506436747,-32.4851072083748));
#50836=CARTESIAN_POINT('Ctrl Pts',(61.0238079284518,11.493284065832,-33.7399112197011));
#50837=CARTESIAN_POINT('Ctrl Pts',(61.0217143885294,11.4948093702616,-34.7422387719057));
#50838=CARTESIAN_POINT('Ctrl Pts',(61.0213301291716,11.4955280787965,-35.2428220670568));
#50839=CARTESIAN_POINT('Ctrl Pts',(61.021365193341,11.4960345422261,-35.6189094102041));
#50840=CARTESIAN_POINT('Ctrl Pts',(61.0214880534992,11.4963594205114,-35.8707605975974));
#50841=CARTESIAN_POINT('Ctrl Pts',(61.022091923799,11.4969726153639,-36.3737127464358));
#50842=CARTESIAN_POINT('Ctrl Pts',(61.0239682927916,11.4979686662637,-37.2522956319764));
#50843=CARTESIAN_POINT('Ctrl Pts',(61.030118867598,11.4998855199777,-39.0044637620451));
#50844=CARTESIAN_POINT('Ctrl Pts',(61.0363540626141,11.5020954232287,-40.5049067899921));
#50845=CARTESIAN_POINT('Ctrl Pts',(61.038646816702,11.5050744859075,-41.7596996292913));
#50846=CARTESIAN_POINT('Ctrl Pts',(61.0390752697443,11.5054585796329,-42.1382540029348));
#50847=CARTESIAN_POINT('Ctrl Pts',(61.0392956115982,11.5053604416316,-42.6406423496876));
#50848=CARTESIAN_POINT('Ctrl Pts',(61.0393322346442,11.5049977022042,-43.1432669810382));
#50849=CARTESIAN_POINT('Ctrl Pts',(61.0391335617917,11.5043074977545,-43.7706467352822));
#50850=CARTESIAN_POINT('Ctrl Pts',(61.0388191356084,11.5039312905533,-44.5220374744878));
#50851=CARTESIAN_POINT('Ctrl Pts',(61.0387575897355,11.5046808017656,-45.1463820923632));
#50852=CARTESIAN_POINT('Ctrl Pts',(61.0389901580766,11.5063260376076,-45.644560991936));
#50853=CARTESIAN_POINT('Ctrl Pts',(61.0393440524272,11.5081845335494,-46.0174562444788));
#50854=CARTESIAN_POINT('Ctrl Pts',(61.0399174477217,11.5107693709555,-46.3895780162853));
#50855=CARTESIAN_POINT('Ctrl Pts',(61.0410285266999,11.5153152039897,-46.8845402270902));
#50856=CARTESIAN_POINT('Ctrl Pts',(61.042309730768,11.5201214408717,-47.2545020559948));
#50857=CARTESIAN_POINT('Ctrl Pts',(61.0439765688629,11.5260573269785,-47.6238702479814));
#50858=CARTESIAN_POINT('Ctrl Pts',(61.0451979805278,11.5311868441681,-47.8583439704282));
#50859=CARTESIAN_POINT('Ctrl Pts',(61.0478905014547,11.54627495127,-48.3401165469988));
#50860=CARTESIAN_POINT('Ctrl Pts',(61.0532534115344,11.5828352334387,-49.1916789368563));
#50861=CARTESIAN_POINT('Ctrl Pts',(61.062428503681,11.6519949668785,-50.4463578455976));
#50862=CARTESIAN_POINT('Ctrl Pts',(61.0755188185728,11.7179578989,-52.0063055054175));
#50863=CARTESIAN_POINT('Ctrl Pts',(61.0858830118634,11.7178472866256,-53.0838602731508));
#50864=CARTESIAN_POINT('Ctrl Pts',(61.0931433051171,11.692434627005,-53.7713622472881));
#50865=CARTESIAN_POINT('Ctrl Pts',(61.0965370029646,11.6755684209064,-54.0770339158701));
#50866=CARTESIAN_POINT('Ctrl Pts',(61.1041095778333,11.6247984603233,-54.6556827303067));
#50867=CARTESIAN_POINT('Ctrl Pts',(61.1188092586801,11.5008147164422,-55.6380313969055));
#50868=CARTESIAN_POINT('Ctrl Pts',(61.1497715914765,11.1836218272256,-57.4462290259746));
#50869=CARTESIAN_POINT('Ctrl Pts',(61.1670585779046,11.0216045517656,-58.733328081795));
#50870=CARTESIAN_POINT('Ctrl Pts',(61.1785128178043,11.0690131276586,-59.4972030211869));
#50871=CARTESIAN_POINT('Ctrl Pts',(61.1797256393047,11.0766416381124,-59.610448755841));
#50872=CARTESIAN_POINT('Ctrl Pts',(61.1821403331636,11.0943651818359,-59.8263975881668));
#50873=CARTESIAN_POINT('Ctrl Pts',(61.1860684267584,11.1336759262185,-60.2121735570825));
#50874=CARTESIAN_POINT('Ctrl Pts',(61.1929862876842,11.2430089381107,-60.9875889820288));
#50875=CARTESIAN_POINT('Ctrl Pts',(61.1988812462932,11.4341741250438,-61.8925738653455));
#50876=CARTESIAN_POINT('Ctrl Pts',(61.2034447566965,11.6805866699791,-62.8071682611196));
#50877=CARTESIAN_POINT('Ctrl Pts',(61.2056763108923,11.8375892467775,-63.3247484688506));
#50878=CARTESIAN_POINT('Ctrl Pts',(61.2070945659281,11.9489406644992,-63.6704733688684));
#50879=CARTESIAN_POINT('Ctrl Pts',(61.2080264110695,12.0248889722813,-63.9011526967969));
#50880=CARTESIAN_POINT('Ctrl Pts',(61.2089503354553,12.1032751394498,-64.1319376965954));
#50881=CARTESIAN_POINT('Ctrl Pts',(61.2097599890901,12.1738487662449,-64.3340311888907));
#50882=CARTESIAN_POINT('Ctrl Pts',(61.210225349747,12.2147156178177,-64.4495369264779));
#50883=CARTESIAN_POINT('Ctrl Pts',(61.2109285935608,12.2765309047319,-64.622787105303));
#50884=CARTESIAN_POINT('Ctrl Pts',(61.2115229163368,12.3291239896802,-64.7672168561216));
#50885=CARTESIAN_POINT('Ctrl Pts',(61.2125656045197,12.4172282475888,-65.0056835116515));
#50886=CARTESIAN_POINT('Ctrl Pts',(61.2153513922814,12.5001116560548,-65.2186040921951));
#50887=CARTESIAN_POINT('Ctrl Pts',(61.21959239646,12.6894555668514,-65.6686299937227));
#50888=CARTESIAN_POINT('Ctrl Pts',(61.2264764890157,13.0580265678792,-66.4581526677089));
#50889=CARTESIAN_POINT('Ctrl Pts',(61.2346640709762,13.9381721898705,-68.0971499643503));
#50890=CARTESIAN_POINT('Ctrl Pts',(61.2318777407206,14.8361818361123,-69.5916598166225));
#50891=CARTESIAN_POINT('Ctrl Pts',(61.2264107813354,15.46766355341,-70.7931005604253));
#50892=CARTESIAN_POINT('Ctrl Pts',(61.2268891177495,15.5965515817802,-71.0376558745414));
#50893=CARTESIAN_POINT('Ctrl Pts',(61.2268525774728,15.8619018084997,-71.5401728351865));
#50894=CARTESIAN_POINT('Ctrl Pts',(61.227175206126,16.1919015707836,-72.1629050847276));
#50895=CARTESIAN_POINT('Ctrl Pts',(61.2272904510929,16.5909525148039,-72.9135914650207));
#50896=CARTESIAN_POINT('Ctrl Pts',(61.227545933965,17.3904573528723,-74.4140808562323));
#50897=CARTESIAN_POINT('Ctrl Pts',(61.2275121731408,18.0603429850346,-75.6669195975717));
#50898=CARTESIAN_POINT('Ctrl Pts',(61.227246123972,19.032055779478,-77.4943066306203));
#50899=CARTESIAN_POINT('Ctrl Pts',(61.2273623803738,19.4677567453798,-78.3136026414037));
#50900=CARTESIAN_POINT('Ctrl Pts',(61.2273623803738,19.9042783327692,-79.134580343502));
#50901=CARTESIAN_POINT('Ctrl Pts',(62.8338034543076,6.85465958390862,24.8297410593479));
#50902=CARTESIAN_POINT('Ctrl Pts',(62.8339996969438,6.85466517832061,24.780833104738));
#50903=CARTESIAN_POINT('Ctrl Pts',(62.8342054937221,6.85467103851654,24.7319257482639));
#50904=CARTESIAN_POINT('Ctrl Pts',(62.8366359551373,6.85474201651055,24.1809791522283));
#50905=CARTESIAN_POINT('Ctrl Pts',(62.8386904201629,6.85437239286699,23.1764427006591));
#50906=CARTESIAN_POINT('Ctrl Pts',(62.8435952494902,6.8532127051144,21.1672198892287));
#50907=CARTESIAN_POINT('Ctrl Pts',(62.8597597964598,6.85370795725647,19.6628112443166));
#50908=CARTESIAN_POINT('Ctrl Pts',(62.8930919457468,6.85688911109818,18.4116365613619));
#50909=CARTESIAN_POINT('Ctrl Pts',(62.9090906942054,6.85822469673433,17.9070296332427));
#50910=CARTESIAN_POINT('Ctrl Pts',(62.9492589590369,6.86126039912779,16.9017582496074));
#50911=CARTESIAN_POINT('Ctrl Pts',(63.0353244769336,6.86788486987616,15.1481225567426));
#50912=CARTESIAN_POINT('Ctrl Pts',(63.1165131117359,6.87689795515155,13.6519556095856));
#50913=CARTESIAN_POINT('Ctrl Pts',(63.166621001802,6.88753276948555,12.4049165190744));
#50914=CARTESIAN_POINT('Ctrl Pts',(63.1870252331573,6.8924666149016,11.907114685837));
#50915=CARTESIAN_POINT('Ctrl Pts',(63.2283614260835,6.90441102490564,10.9098087803523));
#50916=CARTESIAN_POINT('Ctrl Pts',(63.2789666126022,6.92188378938289,9.66026453628725));
#50917=CARTESIAN_POINT('Ctrl Pts',(63.3318608211209,6.94290977387995,8.1549576700279));
#50918=CARTESIAN_POINT('Ctrl Pts',(63.3576559632414,6.95412499495758,7.14673713804403));
#50919=CARTESIAN_POINT('Ctrl Pts',(63.3695506483973,6.95942395216364,6.51574970029781));
#50920=CARTESIAN_POINT('Ctrl Pts',(63.37404243367,6.96148280299519,6.26569418550467));
#50921=CARTESIAN_POINT('Ctrl Pts',(63.3820460089262,6.9654124654468,5.76408603878877));
#50922=CARTESIAN_POINT('Ctrl Pts',(63.3934765388819,6.9717498345268,4.8851799884167));
#50923=CARTESIAN_POINT('Ctrl Pts',(63.4060594893532,6.98214664403403,3.12244904729691));
#50924=CARTESIAN_POINT('Ctrl Pts',(63.3991675704029,6.98667516443248,1.61406737086219));
#50925=CARTESIAN_POINT('Ctrl Pts',(63.3852972835858,6.98713243255313,0.549525775104275));
#50926=CARTESIAN_POINT('Ctrl Pts',(63.3837639990198,6.98625219299159,0.400255301022558));
#50927=CARTESIAN_POINT('Ctrl Pts',(63.3811412856108,6.98092701478105,0.118531957809457));
#50928=CARTESIAN_POINT('Ctrl Pts',(63.3774764614481,6.96352864269567,-0.371543466982117));
#50929=CARTESIAN_POINT('Ctrl Pts',(63.3737734202508,6.92182301979145,-1.04015416616342));
#50930=CARTESIAN_POINT('Ctrl Pts',(63.3679524464333,6.86362502470972,-1.80122588976293));
#50931=CARTESIAN_POINT('Ctrl Pts',(63.3543676733274,6.79529729582811,-2.75769703195224));
#50932=CARTESIAN_POINT('Ctrl Pts',(63.3183836510661,6.76331689501261,-3.84604778170242));
#50933=CARTESIAN_POINT('Ctrl Pts',(63.2579635548131,6.84096872539738,-4.60500935093061));
#50934=CARTESIAN_POINT('Ctrl Pts',(63.2096948711453,6.93185648904187,-5.05892091186654));
#50935=CARTESIAN_POINT('Ctrl Pts',(63.1875270883532,6.97241744695262,-5.23793787000871));
#50936=CARTESIAN_POINT('Ctrl Pts',(63.1325072151405,7.07773702786777,-5.62136260647696));
#50937=CARTESIAN_POINT('Ctrl Pts',(63.0132528713079,7.3211497909772,-6.34163824906952));
#50938=CARTESIAN_POINT('Ctrl Pts',(62.8029591903338,7.82115058001278,-7.49543786075017));
#50939=CARTESIAN_POINT('Ctrl Pts',(62.5936741996999,8.43186353143849,-8.76560234032894));
#50940=CARTESIAN_POINT('Ctrl Pts',(62.4749644958831,8.86097524178464,-9.71157013411916));
#50941=CARTESIAN_POINT('Ctrl Pts',(62.4201981206369,9.09857704453463,-10.2697527203838));
#50942=CARTESIAN_POINT('Ctrl Pts',(62.398078422383,9.21353125528222,-10.5555417660092));
#50943=CARTESIAN_POINT('Ctrl Pts',(62.3840104205132,9.29775257792002,-10.772463221046));
#50944=CARTESIAN_POINT('Ctrl Pts',(62.3807629530719,9.34383659535855,-10.8850870497912));
#50945=CARTESIAN_POINT('Ctrl Pts',(62.3738072198155,9.44544236662011,-11.1302215713694));
#50946=CARTESIAN_POINT('Ctrl Pts',(62.3697513233476,9.62729441691419,-11.5525904946933));
#50947=CARTESIAN_POINT('Ctrl Pts',(62.3837759970867,10.0163201736675,-12.4162142254667));
#50948=CARTESIAN_POINT('Ctrl Pts',(62.4573913421418,10.6023053239374,-13.6872790388798));
#50949=CARTESIAN_POINT('Ctrl Pts',(62.5511457032355,11.0856172382757,-14.9067331093471));
#50950=CARTESIAN_POINT('Ctrl Pts',(62.6046192000456,11.3545866340079,-15.7588167884263));
#50951=CARTESIAN_POINT('Ctrl Pts',(62.6359406541165,11.517469480017,-16.3378185226344));
#50952=CARTESIAN_POINT('Ctrl Pts',(62.6528314507055,11.6183761444237,-16.7844671295404));
#50953=CARTESIAN_POINT('Ctrl Pts',(62.6609105379355,11.6874797908918,-17.1630699070993));
#50954=CARTESIAN_POINT('Ctrl Pts',(62.6638768603096,11.7137656612047,-17.3163953547192));
#50955=CARTESIAN_POINT('Ctrl Pts',(62.6693846908667,11.7590723540921,-17.6187124890694));
#50956=CARTESIAN_POINT('Ctrl Pts',(62.6741202236337,11.7948578504016,-17.918557602196));
#50957=CARTESIAN_POINT('Ctrl Pts',(62.6780970886857,11.8220961938048,-18.2143292670326));
#50958=CARTESIAN_POINT('Ctrl Pts',(62.6802676343343,11.8358525159284,-18.3977339849119));
#50959=CARTESIAN_POINT('Ctrl Pts',(62.6818193623433,11.8450278385985,-18.5434605906301));
#50960=CARTESIAN_POINT('Ctrl Pts',(62.6828920339916,11.8510352847634,-18.6522820837644));
#50961=CARTESIAN_POINT('Ctrl Pts',(62.6837117248072,11.855339726448,-18.742558930143));
#50962=CARTESIAN_POINT('Ctrl Pts',(62.6843229408963,11.8583828851285,-18.8145327501737));
#50963=CARTESIAN_POINT('Ctrl Pts',(62.6892804465,11.8819918798033,-19.4249596018789));
#50964=CARTESIAN_POINT('Ctrl Pts',(62.6909212274186,11.8589387563064,-20.5480089229867));
#50965=CARTESIAN_POINT('Ctrl Pts',(62.6815549707715,11.7610077131498,-22.0779988678205));
#50966=CARTESIAN_POINT('Ctrl Pts',(62.6769765822225,11.7219942672605,-23.0149704733893));
#50967=CARTESIAN_POINT('Ctrl Pts',(62.678220056782,11.7226271915843,-23.5743284523991));
#50968=CARTESIAN_POINT('Ctrl Pts',(62.678644904202,11.7228532665709,-23.832451669843));
#50969=CARTESIAN_POINT('Ctrl Pts',(62.6792855094788,11.723026759193,-24.3286037118354));
#50970=CARTESIAN_POINT('Ctrl Pts',(62.6798847761189,11.7227673230976,-25.2088475010981));
#50971=CARTESIAN_POINT('Ctrl Pts',(62.6795926748682,11.7212741826651,-26.4629661695656));
#50972=CARTESIAN_POINT('Ctrl Pts',(62.6783812027991,11.7193132858567,-27.9721096910006));
#50973=CARTESIAN_POINT('Ctrl Pts',(62.6776646395247,11.7188580444735,-28.9752003144069));
#50974=CARTESIAN_POINT('Ctrl Pts',(62.6774328269539,11.7191365464673,-29.5382568196351));
#50975=CARTESIAN_POINT('Ctrl Pts',(62.6773678117679,11.7192072595742,-29.6634641511824));
#50976=CARTESIAN_POINT('Ctrl Pts',(62.6771988612175,11.7193791972438,-29.9139050923193));
#50977=CARTESIAN_POINT('Ctrl Pts',(62.6768085203825,11.7197566517483,-30.3524295416403));
#50978=CARTESIAN_POINT('Ctrl Pts',(62.6757232234573,11.720782501297,-31.2301444231918));
#50979=CARTESIAN_POINT('Ctrl Pts',(62.6737354365148,11.7228454679361,-32.485293390133));
#50980=CARTESIAN_POINT('Ctrl Pts',(62.6723159850072,11.7252030895258,-33.7400843530539));
#50981=CARTESIAN_POINT('Ctrl Pts',(62.6722120112137,11.7269777063412,-34.7424026860366));
#50982=CARTESIAN_POINT('Ctrl Pts',(62.6726265131155,11.7277869860697,-35.2429657135305));
#50983=CARTESIAN_POINT('Ctrl Pts',(62.6731547159542,11.7283441744651,-35.6190412398323));
#50984=CARTESIAN_POINT('Ctrl Pts',(62.6735967149658,11.7287044977291,-35.8708943236863));
#50985=CARTESIAN_POINT('Ctrl Pts',(62.6747899970285,11.729373041004,-36.3738452418783));
#50986=CARTESIAN_POINT('Ctrl Pts',(62.6775925742435,11.730465877738,-37.2524165673159));
#50987=CARTESIAN_POINT('Ctrl Pts',(62.6851862006745,11.7324561459671,-39.0045608875198));
#50988=CARTESIAN_POINT('Ctrl Pts',(62.6922451067709,11.7347616180926,-40.5049707060355));
#50989=CARTESIAN_POINT('Ctrl Pts',(62.6952068493182,11.737792854927,-41.7597519346065));
#50990=CARTESIAN_POINT('Ctrl Pts',(62.6958432636562,11.7381880744333,-42.1383085302216));
#50991=CARTESIAN_POINT('Ctrl Pts',(62.6963424790514,11.7380992974207,-42.6406967467138));
#50992=CARTESIAN_POINT('Ctrl Pts',(62.6966562218629,11.7377491377675,-43.143320636721));
#50993=CARTESIAN_POINT('Ctrl Pts',(62.6967883997396,11.7370747742033,-43.7706967073052));
#50994=CARTESIAN_POINT('Ctrl Pts',(62.6968136404172,11.7367166265468,-44.5220789304071));
#50995=CARTESIAN_POINT('Ctrl Pts',(62.696959820954,11.7374781356162,-45.1464126012592));
#50996=CARTESIAN_POINT('Ctrl Pts',(62.6972931105947,11.7391196339414,-45.644579362675));
#50997=CARTESIAN_POINT('Ctrl Pts',(62.6976873260218,11.7409726571807,-46.0174643891432));
#50998=CARTESIAN_POINT('Ctrl Pts',(62.6982612772622,11.7435478375997,-46.3895748088443));
#50999=CARTESIAN_POINT('Ctrl Pts',(62.699314289724,11.7480739682818,-46.8845197763614));
#51000=CARTESIAN_POINT('Ctrl Pts',(62.7004802564573,11.7528587259553,-47.2544685737077));
#51001=CARTESIAN_POINT('Ctrl Pts',(62.7019745326836,11.7587656435187,-47.6238213681755));
#51002=CARTESIAN_POINT('Ctrl Pts',(62.7030616556681,11.7638730493905,-47.8582806542546));
#51003=CARTESIAN_POINT('Ctrl Pts',(62.7054176541727,11.778908025164,-48.3400318385945));
#51004=CARTESIAN_POINT('Ctrl Pts',(62.7100281194328,11.8153601828062,-49.1915678567995));
#51005=CARTESIAN_POINT('Ctrl Pts',(62.7177314548789,11.8843055589473,-50.4462446983413));
#51006=CARTESIAN_POINT('Ctrl Pts',(62.7286617221578,11.9499950058551,-52.0062206589874));
#51007=CARTESIAN_POINT('Ctrl Pts',(62.7374616794921,11.9496729009723,-53.083802632839));
#51008=CARTESIAN_POINT('Ctrl Pts',(62.7437552022857,11.9241453339071,-53.7713206746562));
#51009=CARTESIAN_POINT('Ctrl Pts',(62.7467278641718,11.9072308339431,-54.0769989676418));
#51010=CARTESIAN_POINT('Ctrl Pts',(62.7533807248429,11.8563573736431,-54.6556561230826));
#51011=CARTESIAN_POINT('Ctrl Pts',(62.7662999686102,11.7321679192571,-55.6380097865569));
#51012=CARTESIAN_POINT('Ctrl Pts',(62.7933936148545,11.414547770685,-57.4461878152757));
#51013=CARTESIAN_POINT('Ctrl Pts',(62.8076998606852,11.2521153761541,-58.733261786034));
#51014=CARTESIAN_POINT('Ctrl Pts',(62.8180464901747,11.2993569627382,-59.4971585371426));
#51015=CARTESIAN_POINT('Ctrl Pts',(62.8191331598324,11.3069696756115,-59.6104073149356));
#51016=CARTESIAN_POINT('Ctrl Pts',(62.8213202536788,11.3246626827443,-59.8263616687962));
#51017=CARTESIAN_POINT('Ctrl Pts',(62.8249140045037,11.3639265488461,-60.212145946727));
#51018=CARTESIAN_POINT('Ctrl Pts',(62.8313936816921,11.4731898642321,-60.9875725235415));
#51019=CARTESIAN_POINT('Ctrl Pts',(62.8371959216708,11.6643173799114,-61.8925545557377));
#51020=CARTESIAN_POINT('Ctrl Pts',(62.8418437083872,11.9107138368155,-62.8071348176643));
#51021=CARTESIAN_POINT('Ctrl Pts',(62.8441472669097,12.0677119439638,-63.3247042909219));
#51022=CARTESIAN_POINT('Ctrl Pts',(62.8456061691458,12.1790595583554,-63.6704210493343));
#51023=CARTESIAN_POINT('Ctrl Pts',(62.8465622073511,12.2550054220157,-63.9010948539475));
#51024=CARTESIAN_POINT('Ctrl Pts',(62.8475036289829,12.3333877584247,-64.1318738609332));
#51025=CARTESIAN_POINT('Ctrl Pts',(62.8483203676067,12.4039577282718,-64.3339621228141));
#51026=CARTESIAN_POINT('Ctrl Pts',(62.8487869286133,12.4448221972824,-64.4494648452406));
#51027=CARTESIAN_POINT('Ctrl Pts',(62.8494889349193,12.5066336621532,-64.622710503327));
#51028=CARTESIAN_POINT('Ctrl Pts',(62.85007524664,12.5592225331623,-64.7671363855174));
#51029=CARTESIAN_POINT('Ctrl Pts',(62.8510932906693,12.6473190338681,-65.0055968429213));
#51030=CARTESIAN_POINT('Ctrl Pts',(62.8538434577762,12.7301919550291,-65.2185134295923));
#51031=CARTESIAN_POINT('Ctrl Pts',(62.8580322198517,12.9195194071033,-65.6685318447977));
#51032=CARTESIAN_POINT('Ctrl Pts',(62.8648496511971,13.2880665087214,-66.4580453122164));
#51033=CARTESIAN_POINT('Ctrl Pts',(62.8730120924218,14.1681922648577,-68.0970346604163));
#51034=CARTESIAN_POINT('Ctrl Pts',(62.8703191702332,15.0662143539911,-69.5915443941704));
#51035=CARTESIAN_POINT('Ctrl Pts',(62.8648969504777,15.6977083703332,-70.7929890769424));
#51036=CARTESIAN_POINT('Ctrl Pts',(62.8653727258091,15.8265950679221,-71.0375437867453));
#51037=CARTESIAN_POINT('Ctrl Pts',(62.8653378608801,16.091945143954,-71.540060490455));
#51038=CARTESIAN_POINT('Ctrl Pts',(62.8656588470002,16.4219435551466,-72.1627921140557));
#51039=CARTESIAN_POINT('Ctrl Pts',(62.8657732483579,16.8209939328041,-72.9134781847798));
#51040=CARTESIAN_POINT('Ctrl Pts',(62.8660253985644,17.6204977093811,-74.4139671461493));
#51041=CARTESIAN_POINT('Ctrl Pts',(62.8659882824124,18.2903821499167,-75.6668058494398));
#51042=CARTESIAN_POINT('Ctrl Pts',(62.8657236935421,19.2620949450523,-77.4941932451861));
#51043=CARTESIAN_POINT('Ctrl Pts',(62.865838847551,19.6977951217313,-78.3134889537359));
#51044=CARTESIAN_POINT('Ctrl Pts',(62.865838847551,20.1343167091208,-79.1344666558342));
#51045=CARTESIAN_POINT('Ctrl Pts',(63.7696816038415,6.98566143559185,24.8297767096392));
#51046=CARTESIAN_POINT('Ctrl Pts',(63.7698678921138,6.98566675201186,24.7808702678244));
#51047=CARTESIAN_POINT('Ctrl Pts',(63.770063285565,6.98567237256011,24.7319644955167));
#51048=CARTESIAN_POINT('Ctrl Pts',(63.7723701752329,6.98573834934271,24.1810344654839));
#51049=CARTESIAN_POINT('Ctrl Pts',(63.7740711730229,6.9853197046968,23.1764585729357));
#51050=CARTESIAN_POINT('Ctrl Pts',(63.7779926509635,6.98404916981452,21.1672937642235));
#51051=CARTESIAN_POINT('Ctrl Pts',(63.7933492509724,6.98450658438664,19.6629800249552));
#51052=CARTESIAN_POINT('Ctrl Pts',(63.8262474576607,6.98780920603375,18.4119113393576));
#51053=CARTESIAN_POINT('Ctrl Pts',(63.8419144473533,6.98923463277581,17.907607162241));
#51054=CARTESIAN_POINT('Ctrl Pts',(63.8810500167875,6.99255841021727,16.902518936812));
#51055=CARTESIAN_POINT('Ctrl Pts',(63.9649304744712,6.99982554504736,15.1486732817769));
#51056=CARTESIAN_POINT('Ctrl Pts',(64.045922706762,7.00927886130776,13.6515024814671));
#51057=CARTESIAN_POINT('Ctrl Pts',(64.0990790942045,7.01972854564653,12.4033154118975));
#51058=CARTESIAN_POINT('Ctrl Pts',(64.1210943657946,7.02454584913399,11.9050847032849));
#51059=CARTESIAN_POINT('Ctrl Pts',(64.1668633343807,7.0361092645071,10.9072098485462));
#51060=CARTESIAN_POINT('Ctrl Pts',(64.2248180717729,7.05293517703396,9.65737999202147));
#51061=CARTESIAN_POINT('Ctrl Pts',(64.2870324562887,7.07297879196909,8.15222145300158));
#51062=CARTESIAN_POINT('Ctrl Pts',(64.318132387073,7.08355383094343,7.14433253005041));
#51063=CARTESIAN_POINT('Ctrl Pts',(64.3325098039232,7.08845799507042,6.51352704158455));
#51064=CARTESIAN_POINT('Ctrl Pts',(64.3381594740021,7.09024700447211,6.26157340593109));
#51065=CARTESIAN_POINT('Ctrl Pts',(64.349002880189,7.09322958834607,5.7579425291834));
#51066=CARTESIAN_POINT('Ctrl Pts',(64.3664328329182,7.09708822036689,4.87642538977047));
#51067=CARTESIAN_POINT('Ctrl Pts',(64.3919649797897,7.10102666734999,3.11502263829812));
#51068=CARTESIAN_POINT('Ctrl Pts',(64.3878539994614,7.1036005456068,1.61837907716535));
#51069=CARTESIAN_POINT('Ctrl Pts',(64.3636805619995,7.11115149785545,0.566888086807873));
#51070=CARTESIAN_POINT('Ctrl Pts',(64.3607244710463,7.11131284275915,0.418190770104461));
#51071=CARTESIAN_POINT('Ctrl Pts',(64.354643323769,7.10805053627403,0.138129618760668));
#51072=CARTESIAN_POINT('Ctrl Pts',(64.3433926111677,7.09451685315122,-0.349389769171667));
#51073=CARTESIAN_POINT('Ctrl Pts',(64.3251138253951,7.05882182021602,-1.01427458036217));
#51074=CARTESIAN_POINT('Ctrl Pts',(64.2980337169301,7.00853937644289,-1.77080918208802));
#51075=CARTESIAN_POINT('Ctrl Pts',(64.2536264651652,6.95114469802438,-2.72065910584223));
#51076=CARTESIAN_POINT('Ctrl Pts',(64.1798526413958,6.93254514534883,-3.79979071287078));
#51077=CARTESIAN_POINT('Ctrl Pts',(64.1045827204883,7.02209746192965,-4.55524739849757));
#51078=CARTESIAN_POINT('Ctrl Pts',(64.0561043596687,7.12374897730917,-5.0093374304298));
#51079=CARTESIAN_POINT('Ctrl Pts',(64.0353415718871,7.16704405464195,-5.17985062820318));
#51080=CARTESIAN_POINT('Ctrl Pts',(63.98473363006,7.28357400055431,-5.55607874846997));
#51081=CARTESIAN_POINT('Ctrl Pts',(63.8771459519287,7.55714666286979,-6.27006582117503));
#51082=CARTESIAN_POINT('Ctrl Pts',(63.6862239458142,8.12629593123083,-7.43081918066162));
#51083=CARTESIAN_POINT('Ctrl Pts',(63.4899286215678,8.81070481486742,-8.71655424625204));
#51084=CARTESIAN_POINT('Ctrl Pts',(63.3753462052385,9.27819727404204,-9.68536073164948));
#51085=CARTESIAN_POINT('Ctrl Pts',(63.3216748507195,9.53128700469291,-10.2617919553927));
#51086=CARTESIAN_POINT('Ctrl Pts',(63.2997626278364,9.65129343395131,-10.5588427326214));
#51087=CARTESIAN_POINT('Ctrl Pts',(63.2857604236112,9.73807711029578,-10.7852247866449));
#51088=CARTESIAN_POINT('Ctrl Pts',(63.2823617213375,9.78586054723457,-10.9049831939649));
#51089=CARTESIAN_POINT('Ctrl Pts',(63.2754976620879,9.88870298656934,-11.1630548483794));
#51090=CARTESIAN_POINT('Ctrl Pts',(63.2722409143818,10.0681221358058,-11.6063711256514));
#51091=CARTESIAN_POINT('Ctrl Pts',(63.2907849195653,10.4351709496067,-12.5041502226328));
#51092=CARTESIAN_POINT('Ctrl Pts',(63.3791152909834,10.9518091655088,-13.8041091500526));
#51093=CARTESIAN_POINT('Ctrl Pts',(63.4895054865479,11.3517098296877,-15.0210931865357));
#51094=CARTESIAN_POINT('Ctrl Pts',(63.5517804011852,11.5697933201517,-15.8557317029522));
#51095=CARTESIAN_POINT('Ctrl Pts',(63.5882492340872,11.7013443654089,-16.4186590645639));
#51096=CARTESIAN_POINT('Ctrl Pts',(63.607999460131,11.7828835971173,-16.847875169099));
#51097=CARTESIAN_POINT('Ctrl Pts',(63.6178114872258,11.8399722925678,-17.2090989649054));
#51098=CARTESIAN_POINT('Ctrl Pts',(63.6213085239353,11.8623207145412,-17.3601083476327));
#51099=CARTESIAN_POINT('Ctrl Pts',(63.6276475672903,11.900407547536,-17.6552939990412));
#51100=CARTESIAN_POINT('Ctrl Pts',(63.6328094590008,11.9304891212912,-17.9492712973279));
#51101=CARTESIAN_POINT('Ctrl Pts',(63.6368975837894,11.9531961683379,-18.2390478308779));
#51102=CARTESIAN_POINT('Ctrl Pts',(63.6390109632988,11.9646113444201,-18.4189964736862));
#51103=CARTESIAN_POINT('Ctrl Pts',(63.6404502007218,11.9721732543855,-18.5620282108745));
#51104=CARTESIAN_POINT('Ctrl Pts',(63.6414060292637,11.9770986096451,-18.6688979579715));
#51105=CARTESIAN_POINT('Ctrl Pts',(63.6421027861453,11.980601906427,-18.7575928191368));
#51106=CARTESIAN_POINT('Ctrl Pts',(63.6426012395683,11.983062011924,-18.8283338164298));
#51107=CARTESIAN_POINT('Ctrl Pts',(63.6465169594665,12.0020384064807,-19.4284380820498));
#51108=CARTESIAN_POINT('Ctrl Pts',(63.6437665657216,11.9799130102247,-20.5374370938092));
#51109=CARTESIAN_POINT('Ctrl Pts',(63.6262331561345,11.8913092865018,-22.0636011055071));
#51110=CARTESIAN_POINT('Ctrl Pts',(63.6178550717916,11.8553688654383,-23.0089316838751));
#51111=CARTESIAN_POINT('Ctrl Pts',(63.6180369322824,11.8554514432705,-23.5768919709824));
#51112=CARTESIAN_POINT('Ctrl Pts',(63.6180901726606,11.8554515811078,-23.8335704323226));
#51113=CARTESIAN_POINT('Ctrl Pts',(63.6181298419009,11.8553460194198,-24.3296650889028));
#51114=CARTESIAN_POINT('Ctrl Pts',(63.6180477607667,11.8549170294627,-25.2086330940246));
#51115=CARTESIAN_POINT('Ctrl Pts',(63.617617569276,11.8538473380592,-26.4623745102019));
#51116=CARTESIAN_POINT('Ctrl Pts',(63.6169168962429,11.8526439793394,-27.9714303035608));
#51117=CARTESIAN_POINT('Ctrl Pts',(63.6165915435084,11.8524503148402,-28.9751490983386));
#51118=CARTESIAN_POINT('Ctrl Pts',(63.6165192995794,11.8526705637204,-29.5386893428186));
#51119=CARTESIAN_POINT('Ctrl Pts',(63.6164967601456,11.8527266046447,-29.6639149713298));
#51120=CARTESIAN_POINT('Ctrl Pts',(63.6164280037698,11.8528638342163,-29.9144380091037));
#51121=CARTESIAN_POINT('Ctrl Pts',(63.616253499369,11.8531672651109,-30.3530667865238));
#51122=CARTESIAN_POINT('Ctrl Pts',(63.6157408857792,11.8540022964339,-31.2309600714044));
#51123=CARTESIAN_POINT('Ctrl Pts',(63.6148560405522,11.8557046509276,-32.4862181294635));
#51124=CARTESIAN_POINT('Ctrl Pts',(63.6146079535709,11.8576964546748,-33.7409637565676));
#51125=CARTESIAN_POINT('Ctrl Pts',(63.6152919776485,11.8592251366319,-34.7431600757416));
#51126=CARTESIAN_POINT('Ctrl Pts',(63.6160131572755,11.8599271411013,-35.2436261487335));
#51127=CARTESIAN_POINT('Ctrl Pts',(63.6167289651422,11.8604163713172,-35.619620607901));
#51128=CARTESIAN_POINT('Ctrl Pts',(63.6172899438139,11.8607294551642,-35.8714754330862));
#51129=CARTESIAN_POINT('Ctrl Pts',(63.6186993626869,11.8613087578331,-36.37439912327));
#51130=CARTESIAN_POINT('Ctrl Pts',(63.6218187659422,11.8622303558402,-37.2529306311206));
#51131=CARTESIAN_POINT('Ctrl Pts',(63.6298724249999,11.8639299681856,-39.0049923904734));
#51132=CARTESIAN_POINT('Ctrl Pts',(63.6371218535708,11.8659593552387,-40.5053086477893));
#51133=CARTESIAN_POINT('Ctrl Pts',(63.6402975958026,11.8688422992738,-41.7600225880003));
#51134=CARTESIAN_POINT('Ctrl Pts',(63.6410071078334,11.869200696979,-42.1385723752223));
#51135=CARTESIAN_POINT('Ctrl Pts',(63.6416120930757,11.8690739021615,-42.6409445598202));
#51136=CARTESIAN_POINT('Ctrl Pts',(63.642032528753,11.8686874249504,-43.1435512139115));
#51137=CARTESIAN_POINT('Ctrl Pts',(63.6422952454253,11.867973795946,-43.7709012458352));
#51138=CARTESIAN_POINT('Ctrl Pts',(63.6424540668545,11.8675753333189,-44.5222449913211));
#51139=CARTESIAN_POINT('Ctrl Pts',(63.6426771430182,11.868307260696,-45.1465391900779));
#51140=CARTESIAN_POINT('Ctrl Pts',(63.6430445603417,11.8699329547278,-45.6446739195639));
#51141=CARTESIAN_POINT('Ctrl Pts',(63.6434473531315,11.8717750306657,-46.0175326399235));
#51142=CARTESIAN_POINT('Ctrl Pts',(63.6440108357314,11.8743406804985,-46.3896147721523));
#51143=CARTESIAN_POINT('Ctrl Pts',(63.6450217165968,11.878855847725,-46.8845205001939));
#51144=CARTESIAN_POINT('Ctrl Pts',(63.6461202649225,11.8836338117009,-47.2544343843313));
#51145=CARTESIAN_POINT('Ctrl Pts',(63.6475192687113,11.8895347153681,-47.6237524624304));
#51146=CARTESIAN_POINT('Ctrl Pts',(63.6485331967311,11.8946380812674,-47.8581793904239));
#51147=CARTESIAN_POINT('Ctrl Pts',(63.6507112577407,11.9096697449189,-48.3398776255269));
#51148=CARTESIAN_POINT('Ctrl Pts',(63.6549321968964,11.9461224149325,-49.1913321247398));
#51149=CARTESIAN_POINT('Ctrl Pts',(63.661899745935,12.0151105243108,-50.4459332494086));
#51150=CARTESIAN_POINT('Ctrl Pts',(63.6717662960858,12.0808653012226,-52.0058840819985));
#51151=CARTESIAN_POINT('Ctrl Pts',(63.6798092951177,12.0806078845269,-53.0834891683857));
#51152=CARTESIAN_POINT('Ctrl Pts',(63.685631755365,12.0551039347417,-53.7710339616749));
#51153=CARTESIAN_POINT('Ctrl Pts',(63.6884005575708,12.0382035085977,-54.0766930057463));
#51154=CARTESIAN_POINT('Ctrl Pts',(63.6946078413911,11.98735499784,-54.6553335456784));
#51155=CARTESIAN_POINT('Ctrl Pts',(63.7066671306212,11.8632143320451,-55.6376601087274));
#51156=CARTESIAN_POINT('Ctrl Pts',(63.7318747171782,11.5456729000009,-57.445823902878));
#51157=CARTESIAN_POINT('Ctrl Pts',(63.7447371065881,11.3832748414712,-58.7329708717663));
#51158=CARTESIAN_POINT('Ctrl Pts',(63.754538293205,11.430516675957,-59.4970034620545));
#51159=CARTESIAN_POINT('Ctrl Pts',(63.7555614946527,11.4381288101711,-59.6102669072837));
#51160=CARTESIAN_POINT('Ctrl Pts',(63.757633595964,11.4558204399389,-59.8262498407748));
#51161=CARTESIAN_POINT('Ctrl Pts',(63.7610559846096,11.4950820129313,-60.21207989842));
#51162=CARTESIAN_POINT('Ctrl Pts',(63.7673006995254,11.6043374957319,-60.9875811955258));
#51163=CARTESIAN_POINT('Ctrl Pts',(63.7730285030241,11.7954459457701,-61.892608993598));
#51164=CARTESIAN_POINT('Ctrl Pts',(63.7776894929842,12.0418091415548,-62.8071976481216));
#51165=CARTESIAN_POINT('Ctrl Pts',(63.7800137401256,12.1987840166583,-63.3247589036427));
#51166=CARTESIAN_POINT('Ctrl Pts',(63.7814841169113,12.3101155783141,-63.670465471561));
#51167=CARTESIAN_POINT('Ctrl Pts',(63.7824465908856,12.3860503841301,-63.9011311488922));
#51168=CARTESIAN_POINT('Ctrl Pts',(63.7833920679633,12.4644220752372,-64.1319003996215));
#51169=CARTESIAN_POINT('Ctrl Pts',(63.7842086917249,12.5349825047279,-64.3339784746905));
#51170=CARTESIAN_POINT('Ctrl Pts',(63.7846739751752,12.5758415864843,-64.4494749475913));
#51171=CARTESIAN_POINT('Ctrl Pts',(63.7853727382513,12.6376450105055,-64.6227108076007));
#51172=CARTESIAN_POINT('Ctrl Pts',(63.7859534955754,12.6902275539118,-64.7671276588133));
#51173=CARTESIAN_POINT('Ctrl Pts',(63.7869571977421,12.7783138276445,-65.0055722940027));
#51174=CARTESIAN_POINT('Ctrl Pts',(63.7896889391107,12.8611817533433,-65.2184894552572));
#51175=CARTESIAN_POINT('Ctrl Pts',(63.7938509211842,13.0504980009258,-65.6685005511499));
#51176=CARTESIAN_POINT('Ctrl Pts',(63.8006373935899,13.4190322005449,-66.4580084393605));
#51177=CARTESIAN_POINT('Ctrl Pts',(63.8087973635566,14.2991477292712,-68.0969899064714));
#51178=CARTESIAN_POINT('Ctrl Pts',(63.8061589029106,15.1971835373538,-69.5915021464135));
#51179=CARTESIAN_POINT('Ctrl Pts',(63.8007532551723,15.8286835484324,-70.79295089124));
#51180=CARTESIAN_POINT('Ctrl Pts',(63.8012281362553,15.9575693622819,-71.0375049654813));
#51181=CARTESIAN_POINT('Ctrl Pts',(63.80119393312,16.2229190548772,-71.5400213331366));
#51182=CARTESIAN_POINT('Ctrl Pts',(63.8015145278415,16.5529169158553,-72.1627523725029));
#51183=CARTESIAN_POINT('Ctrl Pts',(63.8016287284012,16.9519670659933,-72.9134380477093));
#51184=CARTESIAN_POINT('Ctrl Pts',(63.8018798688152,17.7514707684386,-74.4139264495771));
#51185=CARTESIAN_POINT('Ctrl Pts',(63.8018421662859,18.4213568004002,-75.6667657179307));
#51186=CARTESIAN_POINT('Ctrl Pts',(63.8015784260252,19.3930708108336,-77.4941542216223));
#51187=CARTESIAN_POINT('Ctrl Pts',(63.8016933902503,19.8287710106649,-78.3134497248231));
#51188=CARTESIAN_POINT('Ctrl Pts',(63.8016933902503,20.2652925980544,-79.1344274269214));
#51189=CARTESIAN_POINT('Ctrl Pts',(64.7051644480017,7.116408924445,24.8300078402108));
#51190=CARTESIAN_POINT('Ctrl Pts',(64.7053377316389,7.11641758404992,24.7811081862549));
#51191=CARTESIAN_POINT('Ctrl Pts',(64.7055194879703,7.11642663879709,24.7322093827696));
#51192=CARTESIAN_POINT('Ctrl Pts',(64.7076663238738,7.11653619539653,24.1813574002294));
#51193=CARTESIAN_POINT('Ctrl Pts',(64.7089333530155,7.11620394562584,23.1767995651906));
#51194=CARTESIAN_POINT('Ctrl Pts',(64.7116337977528,7.1151212164358,21.1678109264179));
#51195=CARTESIAN_POINT('Ctrl Pts',(64.7259372767009,7.11587257535556,19.6636235887676));
#51196=CARTESIAN_POINT('Ctrl Pts',(64.7581661701847,7.11956838042874,18.4126884759235));
#51197=CARTESIAN_POINT('Ctrl Pts',(64.7733686324166,7.12124444398637,17.9090536171669));
#51198=CARTESIAN_POINT('Ctrl Pts',(64.8110765201189,7.12531406955845,16.9043953209941));
#51199=CARTESIAN_POINT('Ctrl Pts',(64.8919838728444,7.13421361679888,15.1502768679816));
#51200=CARTESIAN_POINT('Ctrl Pts',(64.9721346453416,7.14443725626699,13.6507990842287));
#51201=CARTESIAN_POINT('Ctrl Pts',(65.0286064914778,7.15405321817069,12.3998864389711));
#51202=CARTESIAN_POINT('Ctrl Pts',(65.0524238497418,7.15838930231741,11.9005515076783));
#51203=CARTESIAN_POINT('Ctrl Pts',(65.1033124598707,7.16848098141989,10.9011803927829));
#51204=CARTESIAN_POINT('Ctrl Pts',(65.1695026290478,7.1826159281451,9.6504907924942));
#51205=CARTESIAN_POINT('Ctrl Pts',(65.2424382899957,7.19881941234379,8.14580949006214));
#51206=CARTESIAN_POINT('Ctrl Pts',(65.279415387021,7.20694536660956,7.13907151701641));
#51207=CARTESIAN_POINT('Ctrl Pts',(65.2966875219862,7.21061662674163,6.50907888376672));
#51208=CARTESIAN_POINT('Ctrl Pts',(65.3036787475355,7.21175047116428,6.25454693463909));
#51209=CARTESIAN_POINT('Ctrl Pts',(65.3178846915829,7.21280660662359,5.74832922553668));
#51210=CARTESIAN_POINT('Ctrl Pts',(65.3424912086468,7.21212906964805,4.86351419160469));
#51211=CARTESIAN_POINT('Ctrl Pts',(65.3844723448837,7.20489497920306,3.10426541017931));
#51212=CARTESIAN_POINT('Ctrl Pts',(65.3858137145825,7.20635092613468,1.62312142967191));
#51213=CARTESIAN_POINT('Ctrl Pts',(65.3481542401232,7.2251071791514,0.591055189956906));
#51214=CARTESIAN_POINT('Ctrl Pts',(65.3433461152336,7.22703081940691,0.44438325056417));
#51215=CARTESIAN_POINT('Ctrl Pts',(65.3327329810604,7.22742217338679,0.168378150486671));
#51216=CARTESIAN_POINT('Ctrl Pts',(65.3115151626867,7.22106840646313,-0.31248537606016));
#51217=CARTESIAN_POINT('Ctrl Pts',(65.2743678438677,7.19689004199902,-0.968906342622114));
#51218=CARTESIAN_POINT('Ctrl Pts',(65.2201659061355,7.16070318601945,-1.71729646420262));
#51219=CARTESIAN_POINT('Ctrl Pts',(65.138127961995,7.12149506286709,-2.65933294316632));
#51220=CARTESIAN_POINT('Ctrl Pts',(65.0212677514518,7.12265966426902,-3.7353594689389));
#51221=CARTESIAN_POINT('Ctrl Pts',(64.9316222306538,7.22839559664225,-4.49980537871026));
#51222=CARTESIAN_POINT('Ctrl Pts',(64.8840064123095,7.34336633938095,-4.9622184634216));
#51223=CARTESIAN_POINT('Ctrl Pts',(64.8654860744028,7.39011619218726,-5.12730050726085));
#51224=CARTESIAN_POINT('Ctrl Pts',(64.8212346614502,7.51900353960278,-5.50122851333676));
#51225=CARTESIAN_POINT('Ctrl Pts',(64.7296348616273,7.82305607592105,-6.21448621908583));
#51226=CARTESIAN_POINT('Ctrl Pts',(64.5653983284746,8.45591926839147,-7.38356887466015));
#51227=CARTESIAN_POINT('Ctrl Pts',(64.3894189549537,9.2044426119807,-8.68093399280264));
#51228=CARTESIAN_POINT('Ctrl Pts',(64.2833592573959,9.70429145696223,-9.66825308483886));
#51229=CARTESIAN_POINT('Ctrl Pts',(64.2329302649014,9.96981790534443,-10.260255099096));
#51230=CARTESIAN_POINT('Ctrl Pts',(64.2121358258074,10.0934659819557,-10.5671612632986));
#51231=CARTESIAN_POINT('Ctrl Pts',(64.1987940709705,10.1817853643353,-10.8019331896955));
#51232=CARTESIAN_POINT('Ctrl Pts',(64.1954277904282,10.2307787537786,-10.9286766181756));
#51233=CARTESIAN_POINT('Ctrl Pts',(64.1890543368135,10.333726963384,-11.1992781972767));
#51234=CARTESIAN_POINT('Ctrl Pts',(64.1870161213236,10.5087215932017,-11.6633744855384));
#51235=CARTESIAN_POINT('Ctrl Pts',(64.2100564700399,10.849714601789,-12.5959843412346));
#51236=CARTESIAN_POINT('Ctrl Pts',(64.3099262271591,11.2916795511846,-13.926060762851));
#51237=CARTESIAN_POINT('Ctrl Pts',(64.4314133690616,11.6068604287468,-15.1387472185044));
#51238=CARTESIAN_POINT('Ctrl Pts',(64.4991553033842,11.7749762761074,-15.9542459159056));
#51239=CARTESIAN_POINT('Ctrl Pts',(64.5387721490654,11.8761248705765,-16.5000309301001));
#51240=CARTESIAN_POINT('Ctrl Pts',(64.5602746005103,11.9393429310418,-16.9112726833083));
#51241=CARTESIAN_POINT('Ctrl Pts',(64.5712560875011,11.9851279878435,-17.2549405326659));
#51242=CARTESIAN_POINT('Ctrl Pts',(64.5751173799452,12.0036216300577,-17.4032968766163));
#51243=CARTESIAN_POINT('Ctrl Pts',(64.5819960563146,12.0348061971104,-17.6908970949841));
#51244=CARTESIAN_POINT('Ctrl Pts',(64.5874005454603,12.0595013591101,-17.9785789158532));
#51245=CARTESIAN_POINT('Ctrl Pts',(64.5914977476405,12.0780348571595,-18.2620220641703));
#51246=CARTESIAN_POINT('Ctrl Pts',(64.5935263039422,12.0873359651854,-18.4383221303805));
#51247=CARTESIAN_POINT('Ctrl Pts',(64.5948496094316,12.093471000405,-18.5785196944922));
#51248=CARTESIAN_POINT('Ctrl Pts',(64.5956954738538,12.0974554188175,-18.6833389389178));
#51249=CARTESIAN_POINT('Ctrl Pts',(64.5962825131139,12.1002766722583,-18.7703750310557));
#51250=CARTESIAN_POINT('Ctrl Pts',(64.5966829631923,12.1022495682262,-18.8398241225591));
#51251=CARTESIAN_POINT('Ctrl Pts',(64.5997081438088,12.1174140974332,-19.429125594599));
#51252=CARTESIAN_POINT('Ctrl Pts',(64.5935514726399,12.0978119383031,-20.523616605654));
#51253=CARTESIAN_POINT('Ctrl Pts',(64.5700582332538,12.0211834039782,-22.0464062828513));
#51254=CARTESIAN_POINT('Ctrl Pts',(64.5591540788071,11.9893996189005,-23.0012058052287));
#51255=CARTESIAN_POINT('Ctrl Pts',(64.5586478717312,11.9891742673814,-23.5785306049086));
#51256=CARTESIAN_POINT('Ctrl Pts',(64.5584554623995,11.9890788471195,-23.8338647853036));
#51257=CARTESIAN_POINT('Ctrl Pts',(64.5581062924057,11.9888665684243,-24.330175180966));
#51258=CARTESIAN_POINT('Ctrl Pts',(64.5575807630889,11.9884492160853,-25.2081942502245));
#51259=CARTESIAN_POINT('Ctrl Pts',(64.5570784245764,11.9878231887438,-26.4618175147749));
#51260=CARTESIAN_POINT('Ctrl Pts',(64.5568079816915,11.9873249387177,-27.9709194770668));
#51261=CARTESIAN_POINT('Ctrl Pts',(64.5568342751215,11.9873189576655,-28.9752550644233));
#51262=CARTESIAN_POINT('Ctrl Pts',(64.556881406146,11.9874619766805,-29.5392444787746));
#51263=CARTESIAN_POINT('Ctrl Pts',(64.5568870580478,11.9874981317671,-29.6645309762994));
#51264=CARTESIAN_POINT('Ctrl Pts',(64.5568864496663,11.9875848055615,-29.9151901610847));
#51265=CARTESIAN_POINT('Ctrl Pts',(64.5568586814735,11.9877733062284,-30.3540233528818));
#51266=CARTESIAN_POINT('Ctrl Pts',(64.5567348204472,11.9882812665427,-31.2322527065777));
#51267=CARTESIAN_POINT('Ctrl Pts',(64.5565930177403,11.9893111427986,-32.4877533171019));
#51268=CARTESIAN_POINT('Ctrl Pts',(64.5571102567688,11.9905299977796,-33.7424380807836));
#51269=CARTESIAN_POINT('Ctrl Pts',(64.5582850642549,11.9914937807235,-34.7444188305187));
#51270=CARTESIAN_POINT('Ctrl Pts',(64.5591916232676,11.9919571000629,-35.2447088874826));
#51271=CARTESIAN_POINT('Ctrl Pts',(64.560014903911,11.9922875235368,-35.6205538474929));
#51272=CARTESIAN_POINT('Ctrl Pts',(64.5606423843809,11.9924959468476,-35.8724151994287));
#51273=CARTESIAN_POINT('Ctrl Pts',(64.5621629227882,11.9928662115165,-36.375292038802));
#51274=CARTESIAN_POINT('Ctrl Pts',(64.5654294808747,11.9934431707212,-37.2537654623141));
#51275=CARTESIAN_POINT('Ctrl Pts',(64.5736110546591,11.9944766845492,-39.0056869199685));
#51276=CARTESIAN_POINT('Ctrl Pts',(64.5808488152006,11.9960885048588,-40.5058778756516));
#51277=CARTESIAN_POINT('Ctrl Pts',(64.5840919930745,11.998692499389,-41.7604850705067));
#51278=CARTESIAN_POINT('Ctrl Pts',(64.5848300484984,11.9989679793655,-42.1390216083991));
#51279=CARTESIAN_POINT('Ctrl Pts',(64.5854822617532,11.998737275502,-42.6413621623367));
#51280=CARTESIAN_POINT('Ctrl Pts',(64.5859544069295,11.9982544377607,-43.1439364206192));
#51281=CARTESIAN_POINT('Ctrl Pts',(64.5862845444706,11.9974332527632,-43.7712388965695));
#51282=CARTESIAN_POINT('Ctrl Pts',(64.5865132311935,11.996928669566,-44.5225165702291));
#51283=CARTESIAN_POINT('Ctrl Pts',(64.5867722507586,11.9975928091762,-45.1467473655363));
#51284=CARTESIAN_POINT('Ctrl Pts',(64.5871458137777,11.9991734720114,-45.6448259117841));
#51285=CARTESIAN_POINT('Ctrl Pts',(64.5875405637534,12.0009882992427,-46.017639988042));
#51286=CARTESIAN_POINT('Ctrl Pts',(64.5880812445665,12.0035329507914,-46.389674977256));
#51287=CARTESIAN_POINT('Ctrl Pts',(64.58903925609,12.0080285644188,-46.884514076738));
#51288=CARTESIAN_POINT('Ctrl Pts',(64.5900704047181,12.0128018055357,-47.2543749322652));
#51289=CARTESIAN_POINT('Ctrl Pts',(64.5913788092078,12.018704641493,-47.6236360390374));
#51290=CARTESIAN_POINT('Ctrl Pts',(64.5923259078638,12.0238118420256,-47.8580083019323));
#51291=CARTESIAN_POINT('Ctrl Pts',(64.5943469155263,12.0388642729446,-48.3396172101738));
#51292=CARTESIAN_POINT('Ctrl Pts',(64.598236438171,12.0753873612504,-49.1909349420587));
#51293=CARTESIAN_POINT('Ctrl Pts',(64.604589974817,12.1445490533975,-50.445413008557));
#51294=CARTESIAN_POINT('Ctrl Pts',(64.6135711070628,12.2106012572339,-52.005316948034));
#51295=CARTESIAN_POINT('Ctrl Pts',(64.6209720428472,12.2105364455327,-53.0829618288254));
#51296=CARTESIAN_POINT('Ctrl Pts',(64.6263938213671,12.1851433349393,-53.7705517051657));
#51297=CARTESIAN_POINT('Ctrl Pts',(64.6289890533431,12.168300433645,-54.0761677617449));
#51298=CARTESIAN_POINT('Ctrl Pts',(64.6348195106565,12.1175678410791,-54.6547705509414));
#51299=CARTESIAN_POINT('Ctrl Pts',(64.6461529446247,11.9936343662937,-55.6370418971346));
#51300=CARTESIAN_POINT('Ctrl Pts',(64.6697751752082,11.6764941201765,-57.4452006237545));
#51301=CARTESIAN_POINT('Ctrl Pts',(64.6814108650537,11.5142323582384,-58.7324797036675));
#51302=CARTESIAN_POINT('Ctrl Pts',(64.6907380805086,11.5615131816963,-59.4967522491422));
#51303=CARTESIAN_POINT('Ctrl Pts',(64.6917061998664,11.5691335623824,-59.6100417519035));
#51304=CARTESIAN_POINT('Ctrl Pts',(64.6936774844079,11.5868372471862,-59.8260754687692));
#51305=CARTESIAN_POINT('Ctrl Pts',(64.6969467821477,11.6261143248605,-60.2119861150514));
#51306=CARTESIAN_POINT('Ctrl Pts',(64.7029706707221,11.7353764924318,-60.9876187997222));
#51307=CARTESIAN_POINT('Ctrl Pts',(64.708601255582,11.9264435194088,-61.8927265572519));
#51308=CARTESIAN_POINT('Ctrl Pts',(64.7132409633046,12.1727368523407,-62.8073341711799));
#51309=CARTESIAN_POINT('Ctrl Pts',(64.7155668810181,12.3296674972552,-63.3248851479995));
#51310=CARTESIAN_POINT('Ctrl Pts',(64.7170377866538,12.4409692098032,-63.6705764933628));
#51311=CARTESIAN_POINT('Ctrl Pts',(64.7180000959491,12.516884389208,-63.9012298813615));
#51312=CARTESIAN_POINT('Ctrl Pts',(64.7189438441818,12.5952365311638,-64.1319835338068));
#51313=CARTESIAN_POINT('Ctrl Pts',(64.7197566706395,12.6657808414747,-64.3340452126826));
#51314=CARTESIAN_POINT('Ctrl Pts',(64.7202189568698,12.7066309878131,-64.4495315147314));
#51315=CARTESIAN_POINT('Ctrl Pts',(64.7209123254143,12.7684213551073,-64.6227513556222));
#51316=CARTESIAN_POINT('Ctrl Pts',(64.7214864980503,12.8209935770223,-64.76715311935));
#51317=CARTESIAN_POINT('Ctrl Pts',(64.7224757287238,12.9090644458765,-65.0055712328325));
#51318=CARTESIAN_POINT('Ctrl Pts',(64.7251908376815,12.9919278859981,-65.2184917956168));
#51319=CARTESIAN_POINT('Ctrl Pts',(64.7293290180449,13.1812312427184,-65.668493382022));
#51320=CARTESIAN_POINT('Ctrl Pts',(64.736090236661,13.5497510630374,-66.4579956692628));
#51321=CARTESIAN_POINT('Ctrl Pts',(64.7442571039241,14.4298545252654,-68.0969663258554));
#51322=CARTESIAN_POINT('Ctrl Pts',(64.7416692429259,15.3278999041524,-69.5914813224));
#51323=CARTESIAN_POINT('Ctrl Pts',(64.7362702143423,15.9594013041192,-70.792934567142));
#51324=CARTESIAN_POINT('Ctrl Pts',(64.7367447246466,16.0882861195186,-71.037487791828));
#51325=CARTESIAN_POINT('Ctrl Pts',(64.7367107895737,16.3536348916276,-71.5400036063225));
#51326=CARTESIAN_POINT('Ctrl Pts',(64.7370311378445,16.6836316372613,-72.1627337480955));
#51327=CARTESIAN_POINT('Ctrl Pts',(64.7371452341623,17.0826813009422,-72.9134187811415));
#51328=CARTESIAN_POINT('Ctrl Pts',(64.7373959106816,17.8821848341678,-74.4139062621009));
#51329=CARTESIAN_POINT('Ctrl Pts',(64.7373575913811,18.5520718028474,-75.6667460982806));
#51330=CARTESIAN_POINT('Ctrl Pts',(64.7370939145941,19.5237863885987,-77.4941361560859));
#51331=CARTESIAN_POINT('Ctrl Pts',(64.7372086991403,19.9594861833032,-78.3134312752707));
#51332=CARTESIAN_POINT('Ctrl Pts',(64.7372086991403,20.3960077706927,-79.134408977369));
#51333=CARTESIAN_POINT('Ctrl Pts',(65.8737924036832,7.27972362482747,24.830719708439));
#51334=CARTESIAN_POINT('Ctrl Pts',(65.8739508172382,7.27974807209772,24.7818433134185));
#51335=CARTESIAN_POINT('Ctrl Pts',(65.874117012026,7.27977377214088,24.7329682485245));
#51336=CARTESIAN_POINT('Ctrl Pts',(65.8760799171986,7.28007502125495,24.182387718394));
#51337=CARTESIAN_POINT('Ctrl Pts',(65.8768102200667,7.28016042533186,23.1780799047975));
#51338=CARTESIAN_POINT('Ctrl Pts',(65.8780004617329,7.28030066667095,21.169620222429));
#51339=CARTESIAN_POINT('Ctrl Pts',(65.8911077508792,7.28229576947915,19.665670039577));
#51340=CARTESIAN_POINT('Ctrl Pts',(65.9227618899891,7.28723028562115,18.4149091012139));
#51341=CARTESIAN_POINT('Ctrl Pts',(65.937553649303,7.28968195281574,17.9129514766427));
#51342=CARTESIAN_POINT('Ctrl Pts',(65.9740318210956,7.29600607013808,16.9094461468704));
#51343=CARTESIAN_POINT('Ctrl Pts',(66.052400367403,7.30966848395803,15.1549455903662));
#51344=CARTESIAN_POINT('Ctrl Pts',(66.1324413024313,7.32212732942626,13.6500845762898));
#51345=CARTESIAN_POINT('Ctrl Pts',(66.1926144093613,7.32878968779399,12.3922404302263));
#51346=CARTESIAN_POINT('Ctrl Pts',(66.2184460262715,7.33140049277579,11.889861993171));
#51347=CARTESIAN_POINT('Ctrl Pts',(66.2749869489222,7.33634110993353,10.8863037890924));
#51348=CARTESIAN_POINT('Ctrl Pts',(66.3506619970192,7.34181448430412,9.63295368880396));
#51349=CARTESIAN_POINT('Ctrl Pts',(66.4352056598121,7.34676377096916,8.12930385968051));
#51350=CARTESIAN_POINT('Ctrl Pts',(66.478136134215,7.34879358540089,7.12596809701373));
#51351=CARTESIAN_POINT('Ctrl Pts',(66.4976942337235,7.34962526288238,6.49871069230604));
#51352=CARTESIAN_POINT('Ctrl Pts',(66.5058488789386,7.3492667756571,6.23927695465185));
#51353=CARTESIAN_POINT('Ctrl Pts',(66.5229619736932,7.34631065962563,5.72839423002403));
#51354=CARTESIAN_POINT('Ctrl Pts',(66.5537894968395,7.33657879141901,4.83765269592994));
#51355=CARTESIAN_POINT('Ctrl Pts',(66.6076953182298,7.30860900780446,3.08462563305782));
#51356=CARTESIAN_POINT('Ctrl Pts',(66.6059773542651,7.30441857674907,1.63634923035219));
#51357=CARTESIAN_POINT('Ctrl Pts',(66.5525035252899,7.34205993182231,0.639509927514526));
#51358=CARTESIAN_POINT('Ctrl Pts',(66.5454972435413,7.34687556071208,0.498621633521989));
#51359=CARTESIAN_POINT('Ctrl Pts',(66.5295692371147,7.35384522301292,0.232470692643993));
#51360=CARTESIAN_POINT('Ctrl Pts',(66.4967140612984,7.36146043161841,-0.232522042960739));
#51361=CARTESIAN_POINT('Ctrl Pts',(66.4370554102342,7.36240274310148,-0.871660388794319));
#51362=CARTESIAN_POINT('Ctrl Pts',(66.3499379299258,7.35979327114988,-1.60636393970138));
#51363=CARTESIAN_POINT('Ctrl Pts',(66.2205880386724,7.36471254279015,-2.53912840525394));
#51364=CARTESIAN_POINT('Ctrl Pts',(66.0504853909669,7.41083991360725,-3.62275211870216));
#51365=CARTESIAN_POINT('Ctrl Pts',(65.9458978498926,7.54818163125836,-4.42265037276126));
#51366=CARTESIAN_POINT('Ctrl Pts',(65.9003376268575,7.68627547992059,-4.91125268444285));
#51367=CARTESIAN_POINT('Ctrl Pts',(65.8857974344671,7.7395375765202,-5.07593826553621));
#51368=CARTESIAN_POINT('Ctrl Pts',(65.851550679021,7.88692863191168,-5.45610951698722));
#51369=CARTESIAN_POINT('Ctrl Pts',(65.7838109216027,8.2291281944258,-6.1772119318308));
#51370=CARTESIAN_POINT('Ctrl Pts',(65.6592480872348,8.92455344306608,-7.35621915105546));
#51371=CARTESIAN_POINT('Ctrl Pts',(65.5197104055659,9.72490024945947,-8.66369594631866));
#51372=CARTESIAN_POINT('Ctrl Pts',(65.4332486345925,10.2469747370881,-9.66784137781621));
#51373=CARTESIAN_POINT('Ctrl Pts',(65.3915395824349,10.5189069855576,-10.2740459695132));
#51374=CARTESIAN_POINT('Ctrl Pts',(65.3741909497076,10.6431397110077,-10.5899292385663));
#51375=CARTESIAN_POINT('Ctrl Pts',(65.3630348686882,10.7306814906878,-10.8323698730741));
#51376=CARTESIAN_POINT('Ctrl Pts',(65.3602648479762,10.7799034008029,-10.9672831411013));
#51377=CARTESIAN_POINT('Ctrl Pts',(65.3555790293633,10.8802607991245,-11.2519472653632));
#51378=CARTESIAN_POINT('Ctrl Pts',(65.3562655432189,11.0454233414466,-11.740082914407));
#51379=CARTESIAN_POINT('Ctrl Pts',(65.3850343039264,11.3464970901329,-12.7135974761297));
#51380=CARTESIAN_POINT('Ctrl Pts',(65.4920620350658,11.6891954949238,-14.0786275442094));
#51381=CARTESIAN_POINT('Ctrl Pts',(65.6153815271947,11.9022605191301,-15.2820323810785));
#51382=CARTESIAN_POINT('Ctrl Pts',(65.6832508100979,12.0135101653315,-16.0726545200068));
#51383=CARTESIAN_POINT('Ctrl Pts',(65.7229408331874,12.0806916995302,-16.5970732688898));
#51384=CARTESIAN_POINT('Ctrl Pts',(65.7446229165371,12.1239928860792,-16.9868636471961));
#51385=CARTESIAN_POINT('Ctrl Pts',(65.7561104052002,12.1574777034339,-17.3100775064337));
#51386=CARTESIAN_POINT('Ctrl Pts',(65.7601334531901,12.1714935706227,-17.4547857382721));
#51387=CARTESIAN_POINT('Ctrl Pts',(65.7672145337002,12.1948950758284,-17.7328729709252));
#51388=CARTESIAN_POINT('Ctrl Pts',(65.7726548632663,12.2135323017902,-18.0125373060938));
#51389=CARTESIAN_POINT('Ctrl Pts',(65.7766652600269,12.2274898916777,-18.2880871043883));
#51390=CARTESIAN_POINT('Ctrl Pts',(65.7785927735464,12.234507621214,-18.4598334864742));
#51391=CARTESIAN_POINT('Ctrl Pts',(65.7798115376444,12.2391332042683,-18.5965121130943));
#51392=CARTESIAN_POINT('Ctrl Pts',(65.7805676453171,12.2421378889634,-18.698786873932));
#51393=CARTESIAN_POINT('Ctrl Pts',(65.7810710484178,12.2442641987468,-18.7837683048892));
#51394=CARTESIAN_POINT('Ctrl Pts',(65.7813998146423,12.2457504059072,-18.8516184625018));
#51395=CARTESIAN_POINT('Ctrl Pts',(65.7837868785876,12.2571684848512,-19.4275595821506));
#51396=CARTESIAN_POINT('Ctrl Pts',(65.775621119517,12.2421443708687,-20.5042456873665));
#51397=CARTESIAN_POINT('Ctrl Pts',(65.7489945935547,12.182244252697,-22.0232569275389));
#51398=CARTESIAN_POINT('Ctrl Pts',(65.7368006727203,12.1568935455233,-22.9902043797373));
#51399=CARTESIAN_POINT('Ctrl Pts',(65.735881815348,12.1567382779436,-23.5794953406884));
#51400=CARTESIAN_POINT('Ctrl Pts',(65.7355519854163,12.1566846906698,-23.8333229661963));
#51401=CARTESIAN_POINT('Ctrl Pts',(65.7350187722687,12.1566038370863,-24.3301850550868));
#51402=CARTESIAN_POINT('Ctrl Pts',(65.7343892144717,12.1565210061183,-25.2074750919231));
#51403=CARTESIAN_POINT('Ctrl Pts',(65.734204367445,12.1565279610149,-26.4614142145459));
#51404=CARTESIAN_POINT('Ctrl Pts',(65.7345785465822,12.1566258136834,-27.9707176947722));
#51405=CARTESIAN_POINT('Ctrl Pts',(65.7348957843501,12.1566692990628,-28.9756419058403));
#51406=CARTESIAN_POINT('Ctrl Pts',(65.73499335781,12.1566700253318,-29.5400152762751));
#51407=CARTESIAN_POINT('Ctrl Pts',(65.7350113611297,12.1566698453262,-29.6653982285895));
#51408=CARTESIAN_POINT('Ctrl Pts',(65.7350357450659,12.1566666612928,-29.9162329999839));
#51409=CARTESIAN_POINT('Ctrl Pts',(65.7350528642071,12.1566545758727,-30.3553462864775));
#51410=CARTESIAN_POINT('Ctrl Pts',(65.7350212283644,12.1566115529058,-31.2340211692203));
#51411=CARTESIAN_POINT('Ctrl Pts',(65.7350004144236,12.1565345212241,-32.4898442622548));
#51412=CARTESIAN_POINT('Ctrl Pts',(65.7355825509547,12.1565358623201,-33.7444453855406));
#51413=CARTESIAN_POINT('Ctrl Pts',(65.7367503236109,12.1566441564589,-34.7461353310499));
#51414=CARTESIAN_POINT('Ctrl Pts',(65.737626123592,12.1567431118176,-35.2461922563658));
#51415=CARTESIAN_POINT('Ctrl Pts',(65.7384156043536,12.1568380753438,-35.621838751668));
#51416=CARTESIAN_POINT('Ctrl Pts',(65.7390146685704,12.1568893906108,-35.8737074001352));
#51417=CARTESIAN_POINT('Ctrl Pts',(65.7404592386519,12.1569543472302,-36.376520769494));
#51418=CARTESIAN_POINT('Ctrl Pts',(65.7435442296114,12.1570041167726,-37.2549134713066));
#51419=CARTESIAN_POINT('Ctrl Pts',(65.7512391420775,12.157082948218,-39.0066502662914));
#51420=CARTESIAN_POINT('Ctrl Pts',(65.7580076945452,12.1580020051857,-40.5066591357687));
#51421=CARTESIAN_POINT('Ctrl Pts',(65.7610437102886,12.1601730856183,-41.7611157742616));
#51422=CARTESIAN_POINT('Ctrl Pts',(65.7617352350437,12.160327216616,-42.1396320632631));
#51423=CARTESIAN_POINT('Ctrl Pts',(65.7623464778483,12.1599518390054,-42.6419294274402));
#51424=CARTESIAN_POINT('Ctrl Pts',(65.7627881425271,12.1593327211339,-43.1444589945198));
#51425=CARTESIAN_POINT('Ctrl Pts',(65.7630951305003,12.1583595684145,-43.7716969484013));
#51426=CARTESIAN_POINT('Ctrl Pts',(65.7633030202572,12.1577030883427,-44.5228852355069));
#51427=CARTESIAN_POINT('Ctrl Pts',(65.7635365165661,12.158267411624,-45.1470299426665));
#51428=CARTESIAN_POINT('Ctrl Pts',(65.763877580132,12.1597882142212,-45.6450361333077));
#51429=CARTESIAN_POINT('Ctrl Pts',(65.7642392853216,12.1615669803864,-46.0177924223416));
#51430=CARTESIAN_POINT('Ctrl Pts',(65.7647362832457,12.1640849783657,-46.3897663728969));
#51431=CARTESIAN_POINT('Ctrl Pts',(65.7656192323513,12.1685577943658,-46.884520536456));
#51432=CARTESIAN_POINT('Ctrl Pts',(65.7665716015208,12.173328871499,-47.2543106941164));
#51433=CARTESIAN_POINT('Ctrl Pts',(65.7677823268629,12.1792395220295,-47.6234988671514));
#51434=CARTESIAN_POINT('Ctrl Pts',(65.768660862589,12.1843559187658,-47.8578016457596));
#51435=CARTESIAN_POINT('Ctrl Pts',(65.7705320125628,12.1994478294434,-48.3392960083222));
#51436=CARTESIAN_POINT('Ctrl Pts',(65.7741265585029,12.2360873515124,-49.1904350310024));
#51437=CARTESIAN_POINT('Ctrl Pts',(65.7799734947423,12.305546019183,-50.4447401645545));
#51438=CARTESIAN_POINT('Ctrl Pts',(65.7882309135466,12.3720591124559,-52.004565952058));
#51439=CARTESIAN_POINT('Ctrl Pts',(65.7950932312151,12.3723191345176,-53.0822510115124));
#51440=CARTESIAN_POINT('Ctrl Pts',(65.8001647624651,12.3470993371356,-53.7698948839355));
#51441=CARTESIAN_POINT('Ctrl Pts',(65.8026093112487,12.3303424812056,-54.0754504737583));
#51442=CARTESIAN_POINT('Ctrl Pts',(65.80811148906,12.2797835304874,-54.6539989744145));
#51443=CARTESIAN_POINT('Ctrl Pts',(65.8188108636188,12.1561703997236,-55.6361936231354));
#51444=CARTESIAN_POINT('Ctrl Pts',(65.8410155509584,11.8396438854787,-57.4443509994081));
#51445=CARTESIAN_POINT('Ctrl Pts',(65.8515345739574,11.6776885026692,-58.7318267365958));
#51446=CARTESIAN_POINT('Ctrl Pts',(65.8604129888326,11.7250675012197,-59.4964199594489));
#51447=CARTESIAN_POINT('Ctrl Pts',(65.861327518522,11.7327010985785,-59.6097436907726));
#51448=CARTESIAN_POINT('Ctrl Pts',(65.8631991793557,11.750426218956,-59.8258444305473));
#51449=CARTESIAN_POINT('Ctrl Pts',(65.8663119320418,11.7897326716554,-60.2118619231453));
#51450=CARTESIAN_POINT('Ctrl Pts',(65.8720888383968,11.8990178725946,-60.9876702353197));
#51451=CARTESIAN_POINT('Ctrl Pts',(65.8775618097942,12.0900399279052,-61.8928903527658));
#51452=CARTESIAN_POINT('Ctrl Pts',(65.8821141524937,12.3362439701848,-62.8075302866294));
#51453=CARTESIAN_POINT('Ctrl Pts',(65.8844065364392,12.4931153111574,-63.3250712383876));
#51454=CARTESIAN_POINT('Ctrl Pts',(65.8858572476094,12.6043773164143,-63.6707448858102));
#51455=CARTESIAN_POINT('Ctrl Pts',(65.8868063248849,12.6802661008852,-63.9013834884364));
#51456=CARTESIAN_POINT('Ctrl Pts',(65.8877368577102,12.7585927555402,-64.1321181809914));
#51457=CARTESIAN_POINT('Ctrl Pts',(65.88853723751,12.8291158174461,-64.3341594200084));
#51458=CARTESIAN_POINT('Ctrl Pts',(65.8889920597898,12.8699542671041,-64.4496329679656));
#51459=CARTESIAN_POINT('Ctrl Pts',(65.8896738172377,12.931727576733,-64.6228326327851));
#51460=CARTESIAN_POINT('Ctrl Pts',(65.8902373768405,12.9842867686261,-64.7672152994411));
#51461=CARTESIAN_POINT('Ctrl Pts',(65.8912070711975,13.072338288075,-65.0055995948209));
#51462=CARTESIAN_POINT('Ctrl Pts',(65.893904219689,13.1551982552599,-65.2185261014648));
#51463=CARTESIAN_POINT('Ctrl Pts',(65.8980167064991,13.3444882335856,-65.6685173087278));
#51464=CARTESIAN_POINT('Ctrl Pts',(65.9047560011375,13.712995741147,-66.4580151443174));
#51465=CARTESIAN_POINT('Ctrl Pts',(65.9129480637986,14.5930912526722,-68.0969738663711));
#51466=CARTESIAN_POINT('Ctrl Pts',(65.9104230697323,15.4911509741754,-69.5914929057301));
#51467=CARTESIAN_POINT('Ctrl Pts',(65.9050180119411,16.1226507856015,-70.7929510454671));
#51468=CARTESIAN_POINT('Ctrl Pts',(65.905492870021,16.2515347021751,-71.0375033190314));
#51469=CARTESIAN_POINT('Ctrl Pts',(65.9054587234462,16.5168823300383,-71.5400184758909));
#51470=CARTESIAN_POINT('Ctrl Pts',(65.9057793254249,16.8468781801207,-72.16274762481));
#51471=CARTESIAN_POINT('Ctrl Pts',(65.9058935864885,17.2459274490871,-72.9134318972112));
#51472=CARTESIAN_POINT('Ctrl Pts',(65.9061448213465,18.0454312362688,-74.4139182816276));
#51473=CARTESIAN_POINT('Ctrl Pts',(65.9061070245676,18.7153204568336,-75.6667589613612));
#51474=CARTESIAN_POINT('Ctrl Pts',(65.9058430512839,19.6870361875413,-77.4941510467294));
#51475=CARTESIAN_POINT('Ctrl Pts',(65.9059580210467,20.1227358835157,-78.3134457653799));
#51476=CARTESIAN_POINT('Ctrl Pts',(65.9059580210468,20.5592574709051,-79.1344234674783));
#51477=CARTESIAN_POINT('Ctrl Pts',(67.742805807408,7.54160808040336,24.8323707857055));
#51478=CARTESIAN_POINT('Ctrl Pts',(67.7429599438519,7.54167108069228,24.7835456054049));
#51479=CARTESIAN_POINT('Ctrl Pts',(67.7431216903204,7.54173699953244,24.7347227544535));
#51480=CARTESIAN_POINT('Ctrl Pts',(67.7450311299336,7.54251984739689,24.1847408960325));
#51481=CARTESIAN_POINT('Ctrl Pts',(67.7454542159906,7.5438074607775,23.1811252872465));
#51482=CARTESIAN_POINT('Ctrl Pts',(67.7457811718776,7.54716938456641,21.1737567515317));
#51483=CARTESIAN_POINT('Ctrl Pts',(67.7585271372276,7.5523488600553,19.670023507983));
#51484=CARTESIAN_POINT('Ctrl Pts',(67.7907393057243,7.55998007425724,18.4193411943366));
#51485=CARTESIAN_POINT('Ctrl Pts',(67.8058150390089,7.5640412743569,17.9206087648972));
#51486=CARTESIAN_POINT('Ctrl Pts',(67.8430415813513,7.57501016242088,16.9193609442862));
#51487=CARTESIAN_POINT('Ctrl Pts',(67.923184578734,7.59854283053069,15.164547126133));
#51488=CARTESIAN_POINT('Ctrl Pts',(68.0052074536955,7.61535646055261,13.6489946955723));
#51489=CARTESIAN_POINT('Ctrl Pts',(68.0672619893672,7.61551626660768,12.3772722079416));
#51490=CARTESIAN_POINT('Ctrl Pts',(68.0942310002145,7.61423207400124,11.8679018653112));
#51491=CARTESIAN_POINT('Ctrl Pts',(68.1540374999369,7.60738627849624,10.855276744513));
#51492=CARTESIAN_POINT('Ctrl Pts',(68.2343088168184,7.5927071823393,9.59654129740986));
#51493=CARTESIAN_POINT('Ctrl Pts',(68.3226710656602,7.57204229887091,8.09728674270897));
#51494=CARTESIAN_POINT('Ctrl Pts',(68.36488440954,7.56107248393117,7.10370740136219));
#51495=CARTESIAN_POINT('Ctrl Pts',(68.3825936563245,7.55677141971308,6.48416185059279));
#51496=CARTESIAN_POINT('Ctrl Pts',(68.3900676092246,7.55355227014377,6.21620475198307));
#51497=CARTESIAN_POINT('Ctrl Pts',(68.4062982498568,7.54294496556681,5.6981199796925));
#51498=CARTESIAN_POINT('Ctrl Pts',(68.4362371178003,7.51642570758137,4.79874139178095));
#51499=CARTESIAN_POINT('Ctrl Pts',(68.4899239058001,7.45236885152295,3.05968374041152));
#51500=CARTESIAN_POINT('Ctrl Pts',(68.4782603854943,7.45751053612557,1.66993124882464));
#51501=CARTESIAN_POINT('Ctrl Pts',(68.3952039810378,7.53749913627296,0.744765281110461));
#51502=CARTESIAN_POINT('Ctrl Pts',(68.3842008427377,7.54887409653413,0.618453143136928));
#51503=CARTESIAN_POINT('Ctrl Pts',(68.3588698517668,7.57060264433434,0.37648458626731));
#51504=CARTESIAN_POINT('Ctrl Pts',(68.3061409379183,7.60917219534973,-0.0481057361875789));
#51505=CARTESIAN_POINT('Ctrl Pts',(68.2107690363639,7.66390644809047,-0.641870471575015));
#51506=CARTESIAN_POINT('Ctrl Pts',(68.0771380246689,7.73110573139229,-1.34336822452881));
#51507=CARTESIAN_POINT('Ctrl Pts',(67.890924435506,7.82906293108064,-2.26476025149921));
#51508=CARTESIAN_POINT('Ctrl Pts',(67.6756317739727,7.98687869646959,-3.40211825486226));
#51509=CARTESIAN_POINT('Ctrl Pts',(67.5657544580734,8.21094517780775,-4.30266306393722));
#51510=CARTESIAN_POINT('Ctrl Pts',(67.5245233815194,8.39728418406289,-4.85788153652574));
#51511=CARTESIAN_POINT('Ctrl Pts',(67.5168291122563,8.46556549575842,-5.03399865888036));
#51512=CARTESIAN_POINT('Ctrl Pts',(67.498094458793,8.64557686408299,-5.4390138280413));
#51513=CARTESIAN_POINT('Ctrl Pts',(67.4675356717595,9.03871021017994,-6.18601230987185));
#51514=CARTESIAN_POINT('Ctrl Pts',(67.4119456645733,9.78056419203286,-7.38113321014756));
#51515=CARTESIAN_POINT('Ctrl Pts',(67.3463105795069,10.5913338716633,-8.698408224898));
#51516=CARTESIAN_POINT('Ctrl Pts',(67.3047874436322,11.1043449629669,-9.71620119923863));
#51517=CARTESIAN_POINT('Ctrl Pts',(67.2848402889429,11.3648155613531,-10.333193746664));
#51518=CARTESIAN_POINT('Ctrl Pts',(67.276616690386,11.4807774373825,-10.6554301435584));
#51519=CARTESIAN_POINT('Ctrl Pts',(67.2713943662642,11.5609909900776,-10.903179458728));
#51520=CARTESIAN_POINT('Ctrl Pts',(67.2706582747739,11.6075462300508,-11.0489379719184));
#51521=CARTESIAN_POINT('Ctrl Pts',(67.2706437082626,11.6978855799641,-11.3507195952246));
#51522=CARTESIAN_POINT('Ctrl Pts',(67.2777911266133,11.8389824143185,-11.8693793215723));
#51523=CARTESIAN_POINT('Ctrl Pts',(67.3152599975797,12.0652822944397,-12.8944649700296));
#51524=CARTESIAN_POINT('Ctrl Pts',(67.4178518526037,12.2508045803798,-14.297925846491));
#51525=CARTESIAN_POINT('Ctrl Pts',(67.5218179503882,12.3237687493651,-15.4806007042437));
#51526=CARTESIAN_POINT('Ctrl Pts',(67.5782051432208,12.3618802613975,-16.2356740428478));
#51527=CARTESIAN_POINT('Ctrl Pts',(67.6112804917142,12.3861954203215,-16.7307739218762));
#51528=CARTESIAN_POINT('Ctrl Pts',(67.629802139802,12.4050714788559,-17.0924204541062));
#51529=CARTESIAN_POINT('Ctrl Pts',(67.6403480227297,12.4232144522942,-17.3892704623789));
#51530=CARTESIAN_POINT('Ctrl Pts',(67.6440742945143,12.4311287307314,-17.528045321064));
#51531=CARTESIAN_POINT('Ctrl Pts',(67.6505780086127,12.4442497558684,-17.7923100213903));
#51532=CARTESIAN_POINT('Ctrl Pts',(67.6555479589858,12.4548337104085,-18.0600251419076));
#51533=CARTESIAN_POINT('Ctrl Pts',(67.6591812474422,12.4628105347589,-18.3240974338833));
#51534=CARTESIAN_POINT('Ctrl Pts',(67.6609177587551,12.4668616236941,-18.4891951551348));
#51535=CARTESIAN_POINT('Ctrl Pts',(67.6620086072592,12.4695517469555,-18.6207627473085));
#51536=CARTESIAN_POINT('Ctrl Pts',(67.6626817085544,12.4713118687434,-18.719341087396));
#51537=CARTESIAN_POINT('Ctrl Pts',(67.6631263749856,12.472568013926,-18.801342808996));
#51538=CARTESIAN_POINT('Ctrl Pts',(67.6634144201367,12.4734530469214,-18.8668744929406));
#51539=CARTESIAN_POINT('Ctrl Pts',(67.665489578405,12.4802979967182,-19.4234602240196));
#51540=CARTESIAN_POINT('Ctrl Pts',(67.6578561832691,12.4726640092777,-20.4744941719435));
#51541=CARTESIAN_POINT('Ctrl Pts',(67.6337655920693,12.4387833875839,-21.988465865762));
#51542=CARTESIAN_POINT('Ctrl Pts',(67.6230151758788,12.4240519376188,-22.9735202222548));
#51543=CARTESIAN_POINT('Ctrl Pts',(67.6222887352555,12.4242543566942,-23.5804071061423));
#51544=CARTESIAN_POINT('Ctrl Pts',(67.6220452785285,12.4243530616591,-23.8322273689017));
#51545=CARTESIAN_POINT('Ctrl Pts',(67.6217257596303,12.4245729199584,-24.3301491602105));
#51546=CARTESIAN_POINT('Ctrl Pts',(67.6215528040221,12.4250111840498,-25.2067512724399));
#51547=CARTESIAN_POINT('Ctrl Pts',(67.6221423903727,12.4256848711193,-26.4613493695427));
#51548=CARTESIAN_POINT('Ctrl Pts',(67.6232783878271,12.4262595156381,-27.9708139359673));
#51549=CARTESIAN_POINT('Ctrl Pts',(67.6237412574751,12.4262578976759,-28.9762328565498));
#51550=CARTESIAN_POINT('Ctrl Pts',(67.6237439413753,12.4260895555892,-29.540893931356));
#51551=CARTESIAN_POINT('Ctrl Pts',(67.6237363434596,12.4260461708279,-29.6663925140077));
#51552=CARTESIAN_POINT('Ctrl Pts',(67.6236936517162,12.4259353214926,-29.9174178590788));
#51553=CARTESIAN_POINT('Ctrl Pts',(67.6235533346394,12.4256827987944,-30.3568433047905));
#51554=CARTESIAN_POINT('Ctrl Pts',(67.6230619887266,12.4249722866822,-31.2360054690753));
#51555=CARTESIAN_POINT('Ctrl Pts',(67.6220605631816,12.4235542229819,-32.4921751234464));
#51556=CARTESIAN_POINT('Ctrl Pts',(67.6214659505391,12.4220626275935,-33.7466652722228));
#51557=CARTESIAN_POINT('Ctrl Pts',(67.6217163791426,12.4211031591343,-34.7480293774022));
#51558=CARTESIAN_POINT('Ctrl Pts',(67.6221665004297,12.4207523160916,-35.2478226594728));
#51559=CARTESIAN_POINT('Ctrl Pts',(67.6226566408131,12.4205516900217,-35.6232470890529));
#51560=CARTESIAN_POINT('Ctrl Pts',(67.6230489596044,12.4204066068882,-35.8751235864376));
#51561=CARTESIAN_POINT('Ctrl Pts',(67.6240585281982,12.4200847295307,-36.3778662665607));
#51562=CARTESIAN_POINT('Ctrl Pts',(67.6263390287901,12.4194853605145,-37.2561695027686));
#51563=CARTESIAN_POINT('Ctrl Pts',(67.632325278412,12.4183496428496,-39.0077021554759));
#51564=CARTESIAN_POINT('Ctrl Pts',(67.6377577403294,12.4184603549216,-40.5075168278314));
#51565=CARTESIAN_POINT('Ctrl Pts',(67.6400657259184,12.4201103103411,-41.7618072942457));
#51566=CARTESIAN_POINT('Ctrl Pts',(67.640566899813,12.4201140133972,-42.1402991098985));
#51567=CARTESIAN_POINT('Ctrl Pts',(67.6409671962261,12.4195546774867,-42.6425468132931));
#51568=CARTESIAN_POINT('Ctrl Pts',(67.6412235640905,12.4187641583059,-43.1450256319257));
#51569=CARTESIAN_POINT('Ctrl Pts',(67.6413400338377,12.4176004139746,-43.7721916062135));
#51570=CARTESIAN_POINT('Ctrl Pts',(67.6413641591375,12.4167556818269,-44.5232827606698));
#51571=CARTESIAN_POINT('Ctrl Pts',(67.6414643897262,12.4171989357511,-45.1473364014215));
#51572=CARTESIAN_POINT('Ctrl Pts',(67.6416994860161,12.4186434241101,-45.6452650445642));
#51573=CARTESIAN_POINT('Ctrl Pts',(67.6419797628929,12.4203764116758,-46.0179601430549));
#51574=CARTESIAN_POINT('Ctrl Pts',(67.6423906812054,12.4228601301659,-46.3898699970262));
#51575=CARTESIAN_POINT('Ctrl Pts',(67.6431490489485,12.4273028228971,-46.8845347673267));
#51576=CARTESIAN_POINT('Ctrl Pts',(67.6439933574302,12.4320694683604,-47.2542530416625));
#51577=CARTESIAN_POINT('Ctrl Pts',(67.6450803751829,12.4379880016587,-47.623365509274));
#51578=CARTESIAN_POINT('Ctrl Pts',(67.6458792333846,12.443115489082,-47.857596045839));
#51579=CARTESIAN_POINT('Ctrl Pts',(67.6475973396259,12.4582553810702,-48.338970501715));
#51580=CARTESIAN_POINT('Ctrl Pts',(67.6509363558493,12.4950414285458,-49.1899211168199));
#51581=CARTESIAN_POINT('Ctrl Pts',(67.656417817741,12.564853518565,-50.4440395966513));
#51582=CARTESIAN_POINT('Ctrl Pts',(67.6641480331354,12.6319236783931,-52.0037696390739));
#51583=CARTESIAN_POINT('Ctrl Pts',(67.6705503166098,12.6325474504813,-53.0814906845916));
#51584=CARTESIAN_POINT('Ctrl Pts',(67.6752859075517,12.6075250848195,-53.7691884355505));
#51585=CARTESIAN_POINT('Ctrl Pts',(67.6775870605467,12.5908672031517,-54.0746701819692));
#51586=CARTESIAN_POINT('Ctrl Pts',(67.6827720266418,12.5405076679727,-54.6531513588603));
#51587=CARTESIAN_POINT('Ctrl Pts',(67.6928452005905,12.4172535357334,-55.6352548638888));
#51588=CARTESIAN_POINT('Ctrl Pts',(67.7135779644103,12.1014009951142,-57.4434256620884));
#51589=CARTESIAN_POINT('Ctrl Pts',(67.722851809162,11.9397251962228,-58.7311281481815));
#51590=CARTESIAN_POINT('Ctrl Pts',(67.7312041788753,11.9871955958615,-59.4960738850571));
#51591=CARTESIAN_POINT('Ctrl Pts',(67.7320550014244,11.994843426241,-59.6094351306532));
#51592=CARTESIAN_POINT('Ctrl Pts',(67.7338048432822,12.0125903784316,-59.8256094334167));
#51593=CARTESIAN_POINT('Ctrl Pts',(67.7367168107863,12.0519246469009,-60.2117438069852));
#51594=CARTESIAN_POINT('Ctrl Pts',(67.7421406544915,12.1612221789839,-60.9877445387918));
#51595=CARTESIAN_POINT('Ctrl Pts',(67.7473099928523,12.3521746086762,-61.893089307246));
#51596=CARTESIAN_POINT('Ctrl Pts',(67.7516355763801,12.5982643565659,-62.8077700981422));
#51597=CARTESIAN_POINT('Ctrl Pts',(67.7538236438324,12.7550642190386,-63.3253043393395));
#51598=CARTESIAN_POINT('Ctrl Pts',(67.7552120031394,12.8662790790965,-63.670961444785));
#51599=CARTESIAN_POINT('Ctrl Pts',(67.7561212496728,12.9421369640812,-63.901585841944));
#51600=CARTESIAN_POINT('Ctrl Pts',(67.7570142538266,13.0204336258431,-64.1323015373684));
#51601=CARTESIAN_POINT('Ctrl Pts',(67.7577833567588,13.090932190376,-64.3343219676662));
#51602=CARTESIAN_POINT('Ctrl Pts',(67.7582206747438,13.1317572074132,-64.4497824107023));
#51603=CARTESIAN_POINT('Ctrl Pts',(67.7588765153974,13.1935110196122,-64.6229612480362));
#51604=CARTESIAN_POINT('Ctrl Pts',(67.7594190688071,13.2460552613512,-64.7673239208043));
#51605=CARTESIAN_POINT('Ctrl Pts',(67.7603545218044,13.3340849364679,-65.0056726218981));
#51606=CARTESIAN_POINT('Ctrl Pts',(67.7630264114336,13.4169425237236,-65.2186078123409));
#51607=CARTESIAN_POINT('Ctrl Pts',(67.7671022826528,13.606220231183,-65.6685908050389));
#51608=CARTESIAN_POINT('Ctrl Pts',(67.7738174709853,13.9747193655418,-66.4580877883408));
#51609=CARTESIAN_POINT('Ctrl Pts',(67.7820693092672,14.8548163287521,-68.0970364510266));
#51610=CARTESIAN_POINT('Ctrl Pts',(67.7796422117366,15.7528921082611,-69.5915590716733));
#51611=CARTESIAN_POINT('Ctrl Pts',(67.7742085967677,16.3843827046983,-70.7930204305104));
#51612=CARTESIAN_POINT('Ctrl Pts',(67.774684987654,16.513266189984,-71.0375719095944));
#51613=CARTESIAN_POINT('Ctrl Pts',(67.7746497020258,16.778612436894,-71.5400864033351));
#51614=CARTESIAN_POINT('Ctrl Pts',(67.7749711303553,17.1086075096059,-72.162814636667));
#51615=CARTESIAN_POINT('Ctrl Pts',(67.7750858845402,17.507656420601,-72.9134981492027));
#51616=CARTESIAN_POINT('Ctrl Pts',(67.7753392151518,18.3071607215725,-74.4139834265988));
#51617=CARTESIAN_POINT('Ctrl Pts',(67.7753030677253,18.9770518098338,-75.6668248107347));
#51618=CARTESIAN_POINT('Ctrl Pts',(67.7750376848129,19.9487680324284,-77.4942188650752));
#51619=CARTESIAN_POINT('Ctrl Pts',(67.7751531793561,20.3844675706249,-78.3135131806212));
#51620=CARTESIAN_POINT('Ctrl Pts',(67.7751531793563,20.8209891580143,-79.1344908827197));
#51621=CARTESIAN_POINT('Ctrl Pts',(70.0797409538656,7.87081603166709,24.8335816570491));
#51622=CARTESIAN_POINT('Ctrl Pts',(70.0799756448786,7.87092046555902,24.7847958004515));
#51623=CARTESIAN_POINT('Ctrl Pts',(70.0802217288107,7.87102995712953,24.7360128868017));
#51624=CARTESIAN_POINT('Ctrl Pts',(70.0831285733729,7.87231907386717,24.1864933048158));
#51625=CARTESIAN_POINT('Ctrl Pts',(70.0857084291293,7.87498063209253,23.1838567634182));
#51626=CARTESIAN_POINT('Ctrl Pts',(70.0919148806055,7.88234851674442,21.1771127206445));
#51627=CARTESIAN_POINT('Ctrl Pts',(70.1112363140131,7.89089667541493,19.6727038446357));
#51628=CARTESIAN_POINT('Ctrl Pts',(70.1504814375106,7.90058700585656,18.421108582133));
#51629=CARTESIAN_POINT('Ctrl Pts',(70.1697464384192,7.90583508389004,17.9235973663367));
#51630=CARTESIAN_POINT('Ctrl Pts',(70.2189478657357,7.92004955211645,16.9233181300777));
#51631=CARTESIAN_POINT('Ctrl Pts',(70.3246403871964,7.95017189341619,15.1692536305156));
#51632=CARTESIAN_POINT('Ctrl Pts',(70.419845264702,7.9691245051039,13.6496635406286));
#51633=CARTESIAN_POINT('Ctrl Pts',(70.4697508893646,7.96305756993818,12.3711740566263));
#51634=CARTESIAN_POINT('Ctrl Pts',(70.4903986876751,7.95739611684289,11.8535050431065));
#51635=CARTESIAN_POINT('Ctrl Pts',(70.5322522714481,7.93720517842765,10.8327471216722));
#51636=CARTESIAN_POINT('Ctrl Pts',(70.5814197965239,7.90173999531898,9.57080124372721));
#51637=CARTESIAN_POINT('Ctrl Pts',(70.6215548553232,7.86287760978718,8.08311707062897));
#51638=CARTESIAN_POINT('Ctrl Pts',(70.6265529441638,7.851025563103,7.10767909393591));
#51639=CARTESIAN_POINT('Ctrl Pts',(70.6200554158803,7.85109623620988,6.50259304499254));
#51640=CARTESIAN_POINT('Ctrl Pts',(70.6172821755683,7.84916354644725,6.22780779202129));
#51641=CARTESIAN_POINT('Ctrl Pts',(70.6099684248821,7.83998838688957,5.70611026729234));
#51642=CARTESIAN_POINT('Ctrl Pts',(70.5919833713834,7.81404214662331,4.80405814351667));
#51643=CARTESIAN_POINT('Ctrl Pts',(70.530876070008,7.75724957337001,3.09228082865713));
#51644=CARTESIAN_POINT('Ctrl Pts',(70.4229142961228,7.78796452061628,1.78279487855182));
#51645=CARTESIAN_POINT('Ctrl Pts',(70.3374929882626,7.91062380588921,0.920546111644628));
#51646=CARTESIAN_POINT('Ctrl Pts',(70.3261887650127,7.92655009675492,0.815573102355774));
#51647=CARTESIAN_POINT('Ctrl Pts',(70.3016919401967,7.96074643074563,0.604598130449329));
#51648=CARTESIAN_POINT('Ctrl Pts',(70.2535232133574,8.02788989730723,0.229523060001451));
#51649=CARTESIAN_POINT('Ctrl Pts',(70.1733985653285,8.14395394628861,-0.321339018131735));
#51650=CARTESIAN_POINT('Ctrl Pts',(70.0679296073265,8.3158125006749,-1.00743831078729));
#51651=CARTESIAN_POINT('Ctrl Pts',(69.924485576269,8.58574606963455,-1.95189023868025));
#51652=CARTESIAN_POINT('Ctrl Pts',(69.7543354654112,8.99387404858029,-3.18250609368043));
#51653=CARTESIAN_POINT('Ctrl Pts',(69.6556906939328,9.37193157308521,-4.20526479014222));
#51654=CARTESIAN_POINT('Ctrl Pts',(69.6176271763688,9.6167934094289,-4.85189132462664));
#51655=CARTESIAN_POINT('Ctrl Pts',(69.6150404011341,9.70387094654282,-5.05485554963878));
#51656=CARTESIAN_POINT('Ctrl Pts',(69.608351339168,9.91053595098722,-5.50475572282167));
#51657=CARTESIAN_POINT('Ctrl Pts',(69.6107081740475,10.318116215295,-6.30236350776975));
#51658=CARTESIAN_POINT('Ctrl Pts',(69.6343815288851,11.000254972414,-7.52661118182464));
#51659=CARTESIAN_POINT('Ctrl Pts',(69.6766224457615,11.6866786141997,-8.85980820136688));
#51660=CARTESIAN_POINT('Ctrl Pts',(69.7071296898245,12.096953840095,-9.87707362096165));
#51661=CARTESIAN_POINT('Ctrl Pts',(69.7227081692398,12.2973745110336,-10.4848255250078));
#51662=CARTESIAN_POINT('Ctrl Pts',(69.7293972812761,12.383871734745,-10.7982467733909));
#51663=CARTESIAN_POINT('Ctrl Pts',(69.7338313852413,12.4427638036451,-11.037717319835));
#51664=CARTESIAN_POINT('Ctrl Pts',(69.7372583324694,12.4792643931483,-11.1910809255586));
#51665=CARTESIAN_POINT('Ctrl Pts',(69.7450988986082,12.5453767274486,-11.4999472238591));
#51666=CARTESIAN_POINT('Ctrl Pts',(69.7613520093288,12.6419821016412,-12.0328588232142));
#51667=CARTESIAN_POINT('Ctrl Pts',(69.8016786896662,12.7677585020227,-13.0749199230374));
#51668=CARTESIAN_POINT('Ctrl Pts',(69.8691448168152,12.8029397807458,-14.4766219386973));
#51669=CARTESIAN_POINT('Ctrl Pts',(69.9235912109219,12.7682710815651,-15.6327397218786));
#51670=CARTESIAN_POINT('Ctrl Pts',(69.9528675113096,12.7526652494517,-16.362145317967));
#51671=CARTESIAN_POINT('Ctrl Pts',(69.9702913827983,12.7458820279233,-16.8377412914816));
#51672=CARTESIAN_POINT('Ctrl Pts',(69.9807618700987,12.7469619944152,-17.1822398002294));
#51673=CARTESIAN_POINT('Ctrl Pts',(69.9877367721392,12.7532498652985,-17.4633817754817));
#51674=CARTESIAN_POINT('Ctrl Pts',(69.9902724907931,12.7559041355279,-17.5957929350974));
#51675=CARTESIAN_POINT('Ctrl Pts',(69.9946923357774,12.7603733220597,-17.8480941322808));
#51676=CARTESIAN_POINT('Ctrl Pts',(69.9981362569232,12.7639894309032,-18.1046860591192));
#51677=CARTESIAN_POINT('Ctrl Pts',(70.0007143766111,12.7667555359829,-18.3585719929953));
#51678=CARTESIAN_POINT('Ctrl Pts',(70.0019843123243,12.7681708635531,-18.5176750764189));
#51679=CARTESIAN_POINT('Ctrl Pts',(70.0028084377921,12.7691206629677,-18.6446774706336));
#51680=CARTESIAN_POINT('Ctrl Pts',(70.0033337386207,12.7697465689295,-18.7399452824287));
#51681=CARTESIAN_POINT('Ctrl Pts',(70.0036969413586,12.7701976032863,-18.8192833935171));
#51682=CARTESIAN_POINT('Ctrl Pts',(70.0039442061729,12.7705181741567,-18.8827414859159));
#51683=CARTESIAN_POINT('Ctrl Pts',(70.0058065097664,12.7730150550074,-19.4220227073925));
#51684=CARTESIAN_POINT('Ctrl Pts',(70.0019467478389,12.7707690700143,-20.4500579544624));
#51685=CARTESIAN_POINT('Ctrl Pts',(69.9880028636105,12.759451471308,-21.9592536776598));
#51686=CARTESIAN_POINT('Ctrl Pts',(69.9819325942476,12.7544739985022,-22.9601843403765));
#51687=CARTESIAN_POINT('Ctrl Pts',(69.9818504352436,12.7546855124083,-23.5825598396711));
#51688=CARTESIAN_POINT('Ctrl Pts',(69.9818498694438,12.7547732795172,-23.8326459407025));
#51689=CARTESIAN_POINT('Ctrl Pts',(69.9819618693895,12.7549581583201,-24.331515238654));
#51690=CARTESIAN_POINT('Ctrl Pts',(69.9824089703596,12.7552944272569,-25.2074733334245));
#51691=CARTESIAN_POINT('Ctrl Pts',(69.9835134424833,12.7557536480768,-26.4623751878375));
#51692=CARTESIAN_POINT('Ctrl Pts',(69.9847399796544,12.756098892895,-27.9712796662369));
#51693=CARTESIAN_POINT('Ctrl Pts',(69.9849507476041,12.7560682675524,-28.9764144739503));
#51694=CARTESIAN_POINT('Ctrl Pts',(69.9847403411927,12.7559468487486,-29.5408469533237));
#51695=CARTESIAN_POINT('Ctrl Pts',(69.9846807995037,12.7559155593729,-29.6662922695801));
#51696=CARTESIAN_POINT('Ctrl Pts',(69.9845152198024,12.755835586929,-29.917220044137));
#51697=CARTESIAN_POINT('Ctrl Pts',(69.9841125650528,12.7556530022131,-30.356482175709));
#51698=CARTESIAN_POINT('Ctrl Pts',(69.9829269517545,12.7551400505817,-31.2353717708401));
#51699=CARTESIAN_POINT('Ctrl Pts',(69.9805586324968,12.7541171006627,-32.4912989215736));
#51700=CARTESIAN_POINT('Ctrl Pts',(69.9783895266914,12.7530531299486,-33.7457658728073));
#51701=CARTESIAN_POINT('Ctrl Pts',(69.9774310607184,12.7523853076487,-34.7472738759857));
#51702=CARTESIAN_POINT('Ctrl Pts',(69.9773215948423,12.7521475451418,-35.2471770527657));
#51703=CARTESIAN_POINT('Ctrl Pts',(69.977419139063,12.75201737046,-35.6227053059714));
#51704=CARTESIAN_POINT('Ctrl Pts',(69.977541730052,12.7519174157327,-35.8745739800902));
#51705=CARTESIAN_POINT('Ctrl Pts',(69.9779905683333,12.7516793667049,-36.3773483318021));
#51706=CARTESIAN_POINT('Ctrl Pts',(69.9792445246214,12.7512023133202,-37.2556757877539));
#51707=CARTESIAN_POINT('Ctrl Pts',(69.9830984509896,12.750259756629,-39.0072979426011));
#51708=CARTESIAN_POINT('Ctrl Pts',(69.9868932895405,12.7504494223442,-40.507159154037));
#51709=CARTESIAN_POINT('Ctrl Pts',(69.9883161118172,12.7521845202418,-41.7615060469929));
#51710=CARTESIAN_POINT('Ctrl Pts',(69.9885876280256,12.7522183251696,-42.1400024337612));
#51711=CARTESIAN_POINT('Ctrl Pts',(69.9887376000478,12.751702152804,-42.6422704841182));
#51712=CARTESIAN_POINT('Ctrl Pts',(69.9887763116878,12.7509546805858,-43.1447697673002));
#51713=CARTESIAN_POINT('Ctrl Pts',(69.9886741002939,12.7498432673778,-43.7719674815809));
#51714=CARTESIAN_POINT('Ctrl Pts',(69.9884953414307,12.7490527076822,-44.5231042257711));
#51715=CARTESIAN_POINT('Ctrl Pts',(69.9884545849398,12.7495288403564,-45.1472023879138));
#51716=CARTESIAN_POINT('Ctrl Pts',(69.9885812323078,12.7509907750599,-45.6451736508804));
#51717=CARTESIAN_POINT('Ctrl Pts',(69.988778939342,12.752731048271,-46.0179027182678));
#51718=CARTESIAN_POINT('Ctrl Pts',(69.9891028664157,12.7552157067239,-46.3898487461034));
#51719=CARTESIAN_POINT('Ctrl Pts',(69.9897351377018,12.7596501127633,-46.8845654751457));
#51720=CARTESIAN_POINT('Ctrl Pts',(69.9904684256117,12.7643991235181,-47.2543243694849));
#51721=CARTESIAN_POINT('Ctrl Pts',(69.9914269985218,12.7702904757354,-47.6234817042101));
#51722=CARTESIAN_POINT('Ctrl Pts',(69.9921449188023,12.7753983944061,-47.8577567510985));
#51723=CARTESIAN_POINT('Ctrl Pts',(69.9937153663376,12.7904898297555,-48.3392024846442));
#51724=CARTESIAN_POINT('Ctrl Pts',(69.9968245713006,12.8271665626957,-49.1902597011841));
#51725=CARTESIAN_POINT('Ctrl Pts',(70.0020056610302,12.8967595109998,-50.4444639950959));
#51726=CARTESIAN_POINT('Ctrl Pts',(70.0092629589438,12.9634701930194,-52.0042114998902));
#51727=CARTESIAN_POINT('Ctrl Pts',(70.0151774431333,12.963824528338,-53.0818878650222));
#51728=CARTESIAN_POINT('Ctrl Pts',(70.0195221116976,12.9386285707829,-53.769543617284));
#51729=CARTESIAN_POINT('Ctrl Pts',(70.0216564325669,12.9218892369982,-54.075048710684));
#51730=CARTESIAN_POINT('Ctrl Pts',(70.0264592121177,12.8713560782644,-54.6535485980993));
#51731=CARTESIAN_POINT('Ctrl Pts',(70.0357543986074,12.7477707333624,-55.6356845180778));
#51732=CARTESIAN_POINT('Ctrl Pts',(70.0545927477608,12.4311929338987,-57.4438736407867));
#51733=CARTESIAN_POINT('Ctrl Pts',(70.0622016950512,12.2690410492287,-58.7314980847868));
#51734=CARTESIAN_POINT('Ctrl Pts',(70.0698758147919,12.3163383864376,-59.4962722687201));
#51735=CARTESIAN_POINT('Ctrl Pts',(70.0706456017594,12.3239632483135,-59.6096143697204));
#51736=CARTESIAN_POINT('Ctrl Pts',(70.0722406933252,12.3416695007431,-59.8257516674088));
#51737=CARTESIAN_POINT('Ctrl Pts',(70.0748997350423,12.3809415586232,-60.2118271282564));
#51738=CARTESIAN_POINT('Ctrl Pts',(70.0798848449523,12.4901511750555,-60.9877325346741));
#51739=CARTESIAN_POINT('Ctrl Pts',(70.0846859736845,12.6810750279437,-61.8930224122099));
#51740=CARTESIAN_POINT('Ctrl Pts',(70.0887363756449,12.9271799879292,-62.8076960822796));
#51741=CARTESIAN_POINT('Ctrl Pts',(70.0907962690645,13.0839977672833,-63.3252423160145));
#51742=CARTESIAN_POINT('Ctrl Pts',(70.0921067372744,13.195225846899,-63.6709135692915));
#51743=CARTESIAN_POINT('Ctrl Pts',(70.0929658003375,13.2710925766303,-63.9015489775992));
#51744=CARTESIAN_POINT('Ctrl Pts',(70.0938109233596,13.3493980555299,-64.1322780048317));
#51745=CARTESIAN_POINT('Ctrl Pts',(70.0945394273088,13.4199035667187,-64.3343120637915));
#51746=CARTESIAN_POINT('Ctrl Pts',(70.0949538252675,13.4607322800446,-64.4497808485651));
#51747=CARTESIAN_POINT('Ctrl Pts',(70.0955755227905,13.5224913056746,-64.6229727263848));
#51748=CARTESIAN_POINT('Ctrl Pts',(70.0960900007352,13.5750392045839,-64.7673474251791));
#51749=CARTESIAN_POINT('Ctrl Pts',(70.0969790953196,13.6630733166992,-65.0057170674026));
#51750=CARTESIAN_POINT('Ctrl Pts',(70.0996177025827,13.7459300625678,-65.2186519130424));
#51751=CARTESIAN_POINT('Ctrl Pts',(70.1036433012842,13.9352112916688,-65.6686450143725));
#51752=CARTESIAN_POINT('Ctrl Pts',(70.1103217310111,14.3037186771198,-66.4581500926349));
#51753=CARTESIAN_POINT('Ctrl Pts',(70.1186392504916,15.1838405759538,-68.0971096194841));
#51754=CARTESIAN_POINT('Ctrl Pts',(70.1163397261599,16.0819302159619,-69.5916293629507));
#51755=CARTESIAN_POINT('Ctrl Pts',(70.1108790104758,16.7134126638863,-70.7930853094538));
#51756=CARTESIAN_POINT('Ctrl Pts',(70.1113567541731,16.8422974277222,-71.0376376506106));
#51757=CARTESIAN_POINT('Ctrl Pts',(70.1113202628326,17.1076442349163,-71.5401526000775));
#51758=CARTESIAN_POINT('Ctrl Pts',(70.1116423816177,17.4376404292802,-72.1628816489));
#51759=CARTESIAN_POINT('Ctrl Pts',(70.1117575330375,17.8366898205343,-72.9135656961683));
#51760=CARTESIAN_POINT('Ctrl Pts',(70.1120128139938,18.6361945871019,-74.4140517265804));
#51761=CARTESIAN_POINT('Ctrl Pts',(70.1119785342542,19.3060848488128,-75.6668924674932));
#51762=CARTESIAN_POINT('Ctrl Pts',(70.1117120950068,20.2778001540279,-77.4942851400854));
#51763=CARTESIAN_POINT('Ctrl Pts',(70.1118280829169,20.7135000717299,-78.3135797649147));
#51764=CARTESIAN_POINT('Ctrl Pts',(70.1118280829168,21.1500216591192,-79.1345574670135));
#51765=CARTESIAN_POINT('Ctrl Pts',(72.8865625591464,8.26574019266068,24.8276674291661));
#51766=CARTESIAN_POINT('Ctrl Pts',(72.8869359246848,8.26572049517288,24.7786937745789));
#51767=CARTESIAN_POINT('Ctrl Pts',(72.8873273851381,8.26569974190122,24.7297204267048));
#51768=CARTESIAN_POINT('Ctrl Pts',(72.8919447951196,8.26546070767614,24.17797013955));
#51769=CARTESIAN_POINT('Ctrl Pts',(72.8988873922156,8.26451654009221,23.1728032601338));
#51770=CARTESIAN_POINT('Ctrl Pts',(72.9173560080737,8.26165580699735,21.1618516897943));
#51771=CARTESIAN_POINT('Ctrl Pts',(72.9479727662523,8.25994157807903,19.6553564107176));
#51772=CARTESIAN_POINT('Ctrl Pts',(72.9958158327139,8.26031865031543,18.4025752947981));
#51773=CARTESIAN_POINT('Ctrl Pts',(73.0208253794137,8.25951792114091,17.8901989626081));
#51774=CARTESIAN_POINT('Ctrl Pts',(73.0873380218554,8.25553385745433,16.8798709913457));
#51775=CARTESIAN_POINT('Ctrl Pts',(73.2296748200099,8.24591178499764,15.1295740970655));
#51776=CARTESIAN_POINT('Ctrl Pts',(73.3371582268296,8.24853883578068,13.6575163179087));
#51777=CARTESIAN_POINT('Ctrl Pts',(73.3530585220882,8.2749226805994,12.4397384118938));
#51778=CARTESIAN_POINT('Ctrl Pts',(73.356533238332,8.2849822560771,11.9323304672573));
#51779=CARTESIAN_POINT('Ctrl Pts',(73.351918135292,8.30439994752229,10.9377185673971));
#51780=CARTESIAN_POINT('Ctrl Pts',(73.324432495624,8.33151574081882,9.70196617136291));
#51781=CARTESIAN_POINT('Ctrl Pts',(73.2565738047078,8.38018797690781,8.24482455372541));
#51782=CARTESIAN_POINT('Ctrl Pts',(73.188921906069,8.43134132223997,7.28751763953783));
#51783=CARTESIAN_POINT('Ctrl Pts',(73.139908835424,8.47204451181113,6.69392156609347));
#51784=CARTESIAN_POINT('Ctrl Pts',(73.1173372266464,8.49011925131763,6.44016523067723));
#51785=CARTESIAN_POINT('Ctrl Pts',(73.0653378607807,8.52148234509983,5.94599916456272));
#51786=CARTESIAN_POINT('Ctrl Pts',(72.9587586513335,8.57066940381603,5.08370778538657));
#51787=CARTESIAN_POINT('Ctrl Pts',(72.7116581638965,8.65615239472504,3.39681284085337));
#51788=CARTESIAN_POINT('Ctrl Pts',(72.5399901263606,8.79326075224883,1.99040804109539));
#51789=CARTESIAN_POINT('Ctrl Pts',(72.488100820693,9.02163723228497,1.02355785184261));
#51790=CARTESIAN_POINT('Ctrl Pts',(72.4833544360269,9.04789388573715,0.919138805898511));
#51791=CARTESIAN_POINT('Ctrl Pts',(72.4734944993745,9.10670425273688,0.701380761297459));
#51792=CARTESIAN_POINT('Ctrl Pts',(72.4573641049337,9.22167130677439,0.317256690956153));
#51793=CARTESIAN_POINT('Ctrl Pts',(72.4350064423105,9.41948780353124,-0.250089179012498));
#51794=CARTESIAN_POINT('Ctrl Pts',(72.4069158908792,9.69866948764853,-0.953704395888368));
#51795=CARTESIAN_POINT('Ctrl Pts',(72.367097095033,10.1105519747146,-1.9213359299363));
#51796=CARTESIAN_POINT('Ctrl Pts',(72.3145247685813,10.6685132376829,-3.18402347160584));
#51797=CARTESIAN_POINT('Ctrl Pts',(72.2842979906458,11.0951808963158,-4.26275861171817));
#51798=CARTESIAN_POINT('Ctrl Pts',(72.2768707776213,11.3322038028194,-4.96442639381475));
#51799=CARTESIAN_POINT('Ctrl Pts',(72.2817991873453,11.4180358849558,-5.2019584464972));
#51800=CARTESIAN_POINT('Ctrl Pts',(72.2957055330416,11.5998824492514,-5.70484469018419));
#51801=CARTESIAN_POINT('Ctrl Pts',(72.3400044590547,11.9223023270952,-6.58102264467085));
#51802=CARTESIAN_POINT('Ctrl Pts',(72.4485046707705,12.3824968693468,-7.8717536828968));
#51803=CARTESIAN_POINT('Ctrl Pts',(72.5868482248549,12.7732400063546,-9.21294999905228));
#51804=CARTESIAN_POINT('Ctrl Pts',(72.6694839019536,12.9825682881853,-10.1808033039262));
#51805=CARTESIAN_POINT('Ctrl Pts',(72.7079819980637,13.0811308336793,-10.7403201973301));
#51806=CARTESIAN_POINT('Ctrl Pts',(72.7235630104351,13.1230129893701,-11.0222398269303));
#51807=CARTESIAN_POINT('Ctrl Pts',(72.7336302268316,13.1516841759947,-11.235476861186));
#51808=CARTESIAN_POINT('Ctrl Pts',(72.7399593853654,13.1707010880872,-11.3844405524316));
#51809=CARTESIAN_POINT('Ctrl Pts',(72.7517498643427,13.2030198757993,-11.6767974705028));
#51810=CARTESIAN_POINT('Ctrl Pts',(72.7697996681693,13.2473586325557,-12.1844527718077));
#51811=CARTESIAN_POINT('Ctrl Pts',(72.7962782320539,13.2919511946022,-13.1752477705232));
#51812=CARTESIAN_POINT('Ctrl Pts',(72.8109024014116,13.2660096011693,-14.5238591316298));
#51813=CARTESIAN_POINT('Ctrl Pts',(72.8099755885965,13.2058906010588,-15.6607465153076));
#51814=CARTESIAN_POINT('Ctrl Pts',(72.8094437551831,13.1754828967126,-16.3890783692441));
#51815=CARTESIAN_POINT('Ctrl Pts',(72.809549987816,13.159168467406,-16.8669534234));
#51816=CARTESIAN_POINT('Ctrl Pts',(72.8106563092265,13.1530496688261,-17.2167613707435));
#51817=CARTESIAN_POINT('Ctrl Pts',(72.8127028755648,13.1530106002742,-17.5037664142363));
#51818=CARTESIAN_POINT('Ctrl Pts',(72.8134629462877,13.1529462455956,-17.631446044319));
#51819=CARTESIAN_POINT('Ctrl Pts',(72.8147612394063,13.1528359207374,-17.8787319632469));
#51820=CARTESIAN_POINT('Ctrl Pts',(72.8157545524651,13.1527002033884,-18.1292115146335));
#51821=CARTESIAN_POINT('Ctrl Pts',(72.8164679719332,13.1525607492633,-18.3782333876691));
#51822=CARTESIAN_POINT('Ctrl Pts',(72.8168062584366,13.1524676775119,-18.5342986085837));
#51823=CARTESIAN_POINT('Ctrl Pts',(72.8170154966428,13.1523917172578,-18.6590504455465));
#51824=CARTESIAN_POINT('Ctrl Pts',(72.81714308237,13.1523334865433,-18.752668411454));
#51825=CARTESIAN_POINT('Ctrl Pts',(72.8172257706092,13.1522841134498,-18.8306852443342));
#51826=CARTESIAN_POINT('Ctrl Pts',(72.817278168026,13.152244180255,-18.893112099867));
#51827=CARTESIAN_POINT('Ctrl Pts',(72.8176480539968,13.151901641012,-19.423789566149));
#51828=CARTESIAN_POINT('Ctrl Pts',(72.8160192886251,13.1511430274956,-20.4402588086319));
#51829=CARTESIAN_POINT('Ctrl Pts',(72.8110708994919,13.1500609857134,-21.946711243545));
#51830=CARTESIAN_POINT('Ctrl Pts',(72.8089031262298,13.1495061882381,-22.9551201162143));
#51831=CARTESIAN_POINT('Ctrl Pts',(72.8087715182586,13.1492717851851,-23.5849046078959));
#51832=CARTESIAN_POINT('Ctrl Pts',(72.8087370586053,13.1491837194568,-23.8341005320297));
#51833=CARTESIAN_POINT('Ctrl Pts',(72.8087323220412,13.1490219551124,-24.3333279217166));
#51834=CARTESIAN_POINT('Ctrl Pts',(72.8088662673866,13.1487767703018,-25.2087732822766));
#51835=CARTESIAN_POINT('Ctrl Pts',(72.8093266109851,13.1485371767267,-26.4634727764513));
#51836=CARTESIAN_POINT('Ctrl Pts',(72.8098422061217,13.1484307095398,-27.9716158872549));
#51837=CARTESIAN_POINT('Ctrl Pts',(72.8098636816209,13.1484791110874,-28.9762238937061));
#51838=CARTESIAN_POINT('Ctrl Pts',(72.809695974041,13.1485404445919,-29.5403115148885));
#51839=CARTESIAN_POINT('Ctrl Pts',(72.8096504359251,13.1485557179075,-29.6656275973256));
#51840=CARTESIAN_POINT('Ctrl Pts',(72.8095299300256,13.1485922645576,-29.9163418893078));
#51841=CARTESIAN_POINT('Ctrl Pts',(72.8092477764273,13.1486715934479,-30.3552440960804));
#51842=CARTESIAN_POINT('Ctrl Pts',(72.8084470491389,13.1488858874495,-31.2335561262111));
#51843=CARTESIAN_POINT('Ctrl Pts',(72.8069060771625,13.1493246110313,-32.4890162027479));
#51844=CARTESIAN_POINT('Ctrl Pts',(72.8055811662997,13.1498610648749,-33.7435174707489));
#51845=CARTESIAN_POINT('Ctrl Pts',(72.8050973616134,13.1503012894563,-34.7453688189319));
#51846=CARTESIAN_POINT('Ctrl Pts',(72.8051223743103,13.1505189541041,-35.2455401860808));
#51847=CARTESIAN_POINT('Ctrl Pts',(72.8052695179574,13.1506776609489,-35.6213073903767));
#51848=CARTESIAN_POINT('Ctrl Pts',(72.8054127632015,13.1507670975923,-35.8731634916129));
#51849=CARTESIAN_POINT('Ctrl Pts',(72.8058580763078,13.1508899756323,-36.3760126603184));
#51850=CARTESIAN_POINT('Ctrl Pts',(72.8070010659971,13.151001693871,-37.2544170873883));
#51851=CARTESIAN_POINT('Ctrl Pts',(72.8103276560061,13.1510724644046,-39.0062487185812));
#51852=CARTESIAN_POINT('Ctrl Pts',(72.8135232736315,13.1519042845439,-40.5062738671393));
#51853=CARTESIAN_POINT('Ctrl Pts',(72.8147874625334,13.1540974660561,-41.7607797533392));
#51854=CARTESIAN_POINT('Ctrl Pts',(72.8150437115558,13.1542686847748,-42.1392980320379));
#51855=CARTESIAN_POINT('Ctrl Pts',(72.8152170000764,13.1539277490992,-42.6416181546101));
#51856=CARTESIAN_POINT('Ctrl Pts',(72.8153010284797,13.1533492477975,-43.1441703083421));
#51857=CARTESIAN_POINT('Ctrl Pts',(72.8152838011158,13.1524330871771,-43.7714444955365));
#51858=CARTESIAN_POINT('Ctrl Pts',(72.8152106934443,13.1518401424435,-44.5226858579805));
#51859=CARTESIAN_POINT('Ctrl Pts',(72.8152263278303,13.1524409218818,-45.1468828510351));
#51860=CARTESIAN_POINT('Ctrl Pts',(72.815358309241,13.153972508572,-45.6449411346028));
#51861=CARTESIAN_POINT('Ctrl Pts',(72.8155348943229,13.1557487952531,-46.0177390087985));
#51862=CARTESIAN_POINT('Ctrl Pts',(72.8158073722611,13.1582518130966,-46.38975745001));
#51863=CARTESIAN_POINT('Ctrl Pts',(72.8163236379806,13.16268521408,-46.8845758652391));
#51864=CARTESIAN_POINT('Ctrl Pts',(72.8169088176789,13.1674030382691,-47.2544162259643));
#51865=CARTESIAN_POINT('Ctrl Pts',(72.8176675448834,13.1732397249461,-47.6236601496442));
#51866=CARTESIAN_POINT('Ctrl Pts',(72.8182420222224,13.1783039805414,-47.8580173951434));
#51867=CARTESIAN_POINT('Ctrl Pts',(72.8194910411997,13.1932756057432,-48.3395992515894));
#51868=CARTESIAN_POINT('Ctrl Pts',(72.8219486073975,13.2296643335382,-49.1908687776819));
#51869=CARTESIAN_POINT('Ctrl Pts',(72.8259596787755,13.2986484891989,-50.4452782120899));
#51870=CARTESIAN_POINT('Ctrl Pts',(72.8314631100544,13.3644210345925,-52.0051236883727));
#51871=CARTESIAN_POINT('Ctrl Pts',(72.8359915178612,13.3641025210508,-53.0827529928531));
#51872=CARTESIAN_POINT('Ctrl Pts',(72.8394034112851,13.3385039554964,-53.7703454551854));
#51873=CARTESIAN_POINT('Ctrl Pts',(72.8411346048377,13.3215759995062,-54.0759284754757));
#51874=CARTESIAN_POINT('Ctrl Pts',(72.8450369657781,13.2706456813332,-54.6544988397768));
#51875=CARTESIAN_POINT('Ctrl Pts',(72.8525511039821,13.1463106982952,-55.6367316934619));
#51876=CARTESIAN_POINT('Ctrl Pts',(72.8673326133932,12.8281734952145,-57.4449133974758));
#51877=CARTESIAN_POINT('Ctrl Pts',(72.8716417191591,12.6650265360812,-58.7322902670711));
#51878=CARTESIAN_POINT('Ctrl Pts',(72.8780571431512,12.7119587273811,-59.4966710357007));
#51879=CARTESIAN_POINT('Ctrl Pts',(72.878680938848,12.719537487613,-59.6099712697978));
#51880=CARTESIAN_POINT('Ctrl Pts',(72.8800066542427,12.7371627024027,-59.8260265119129));
#51881=CARTESIAN_POINT('Ctrl Pts',(72.882252534028,12.7763144747118,-60.2119714384574));
#51882=CARTESIAN_POINT('Ctrl Pts',(72.8866217314193,12.8853688503928,-60.9876622988252));
#51883=CARTESIAN_POINT('Ctrl Pts',(72.8911013820776,13.0762781429483,-61.8928145456306));
#51884=CARTESIAN_POINT('Ctrl Pts',(72.8950177095436,13.322458888845,-62.8074465123463));
#51885=CARTESIAN_POINT('Ctrl Pts',(72.8970367991066,13.4793367386658,-63.3250031405502));
#51886=CARTESIAN_POINT('Ctrl Pts',(72.8983197062041,13.5906053760081,-63.6706948039897));
#51887=CARTESIAN_POINT('Ctrl Pts',(72.8991593399374,13.6664987843523,-63.9013474223356));
#51888=CARTESIAN_POINT('Ctrl Pts',(72.8999819509068,13.7448296381239,-64.1320988669824));
#51889=CARTESIAN_POINT('Ctrl Pts',(72.9006855457522,13.815355017023,-64.3341572392981));
#51890=CARTESIAN_POINT('Ctrl Pts',(72.9010838538832,13.8561942287203,-64.4496412499583));
#51891=CARTESIAN_POINT('Ctrl Pts',(72.9016793794264,13.9179680385629,-64.6228572582028));
#51892=CARTESIAN_POINT('Ctrl Pts',(72.9021674144054,13.9705261148409,-64.767254909506));
#51893=CARTESIAN_POINT('Ctrl Pts',(72.9030045822634,14.0585728029474,-65.0056652986328));
#51894=CARTESIAN_POINT('Ctrl Pts',(72.9055939633252,14.1414228933973,-65.2185919113378));
#51895=CARTESIAN_POINT('Ctrl Pts',(72.9095453337735,14.3307041702797,-65.6685963244501));
#51896=CARTESIAN_POINT('Ctrl Pts',(72.916148601967,14.699210204333,-66.4581050158198));
#51897=CARTESIAN_POINT('Ctrl Pts',(72.9244920846649,15.5793474471033,-68.0970777158963));
#51898=CARTESIAN_POINT('Ctrl Pts',(72.9223525060322,16.4774546468999,-69.5915925940898));
#51899=CARTESIAN_POINT('Ctrl Pts',(72.916907887135,17.1089423094142,-70.793043389865));
#51900=CARTESIAN_POINT('Ctrl Pts',(72.917384567627,17.2378279180548,-71.0375967877744));
#51901=CARTESIAN_POINT('Ctrl Pts',(72.9173485145221,17.5031761663896,-71.5401125120657));
#51902=CARTESIAN_POINT('Ctrl Pts',(72.9176699512543,17.8331733766952,-72.1628426787913));
#51903=CARTESIAN_POINT('Ctrl Pts',(72.917784753143,18.2322232294136,-72.9135276172968));
#51904=CARTESIAN_POINT('Ctrl Pts',(72.9180388995489,19.0317276241097,-74.4140149343857));
#51905=CARTESIAN_POINT('Ctrl Pts',(72.9180039490813,19.7016155224588,-75.6668546533854));
#51906=CARTESIAN_POINT('Ctrl Pts',(72.9177383558073,20.6733298082105,-77.4942448926987));
#51907=CARTESIAN_POINT('Ctrl Pts',(72.9178539859473,21.1090298969448,-78.3135399675102));
#51908=CARTESIAN_POINT('Ctrl Pts',(72.9178539859467,21.5455514843342,-79.1345176696082));
#51909=CARTESIAN_POINT('Ctrl Pts',(75.6920843231871,8.65897692250244,24.8219643854307));
#51910=CARTESIAN_POINT('Ctrl Pts',(75.6923132292224,8.65879783026269,24.7728102144334));
#51911=CARTESIAN_POINT('Ctrl Pts',(75.6925532150177,8.6586101781166,24.7236580540939));
#51912=CARTESIAN_POINT('Ctrl Pts',(75.6953902922843,8.65640201617935,24.1696573197671));
#51913=CARTESIAN_POINT('Ctrl Pts',(75.6995064690153,8.64928079164444,23.1576519092927));
#51914=CARTESIAN_POINT('Ctrl Pts',(75.7103280108074,8.62912680918379,21.1444176786476));
#51915=CARTESIAN_POINT('Ctrl Pts',(75.7291509450652,8.61495252403147,19.6425276742755));
#51916=CARTESIAN_POINT('Ctrl Pts',(75.7594327416392,8.61193509309899,18.397120827803));
#51917=CARTESIAN_POINT('Ctrl Pts',(75.7767158149842,8.60615829648623,17.864843351189));
#51918=CARTESIAN_POINT('Ctrl Pts',(75.8250678816251,8.58547956144294,16.8429107530138));
#51919=CARTESIAN_POINT('Ctrl Pts',(75.9298815198313,8.54285802791338,15.0989495736632));
#51920=CARTESIAN_POINT('Ctrl Pts',(75.9978315522776,8.55572607586397,13.6999726172356));
#51921=CARTESIAN_POINT('Ctrl Pts',(75.983190075358,8.6425795941063,12.5772390575261));
#51922=CARTESIAN_POINT('Ctrl Pts',(75.9735243054875,8.68395341370793,12.0967435015462));
#51923=CARTESIAN_POINT('Ctrl Pts',(75.9417752207441,8.78149154793085,11.1511657014746));
#51924=CARTESIAN_POINT('Ctrl Pts',(75.8808350755608,8.93152341758648,9.95652328614932));
#51925=CARTESIAN_POINT('Ctrl Pts',(75.7827348239014,9.150895172005,8.52051663293493));
#51926=CARTESIAN_POINT('Ctrl Pts',(75.7040125639903,9.32420736540206,7.55808056960739));
#51927=CARTESIAN_POINT('Ctrl Pts',(75.6507853624626,9.44159633993459,6.95787391536139));
#51928=CARTESIAN_POINT('Ctrl Pts',(75.6279709087828,9.48720988729069,6.73800874146035));
#51929=CARTESIAN_POINT('Ctrl Pts',(75.5737377326004,9.58669194486765,6.27848372446474));
#51930=CARTESIAN_POINT('Ctrl Pts',(75.4618114014312,9.77627927411454,5.46037967472472));
#51931=CARTESIAN_POINT('Ctrl Pts',(75.2042613425529,10.2136783601429,3.74248125930447));
#51932=CARTESIAN_POINT('Ctrl Pts',(75.0088960863467,10.6627469527714,2.17071336334972));
#51933=CARTESIAN_POINT('Ctrl Pts',(74.944959962901,10.981253033238,1.03842468921417));
#51934=CARTESIAN_POINT('Ctrl Pts',(74.9402607665987,11.0169954680218,0.91882325276358));
#51935=CARTESIAN_POINT('Ctrl Pts',(74.9308100590913,11.0923951315099,0.670911402430064));
#51936=CARTESIAN_POINT('Ctrl Pts',(74.9185898285984,11.2290321678571,0.241146043059909));
#51937=CARTESIAN_POINT('Ctrl Pts',(74.9106916827709,11.4373076654428,-0.376998997526034));
#51938=CARTESIAN_POINT('Ctrl Pts',(74.916714958484,11.6983244017743,-1.12353421260398));
#51939=CARTESIAN_POINT('Ctrl Pts',(74.9434983842269,12.0509531026759,-2.13199781589735));
#51940=CARTESIAN_POINT('Ctrl Pts',(75.0080227454324,12.4805622284169,-3.4239925620957));
#51941=CARTESIAN_POINT('Ctrl Pts',(75.0746002971343,12.7666822976329,-4.50465271514652));
#51942=CARTESIAN_POINT('Ctrl Pts',(75.111308775638,12.9118512205026,-5.19568686901404));
#51943=CARTESIAN_POINT('Ctrl Pts',(75.1268413713536,12.9684034239111,-5.46586079559349));
#51944=CARTESIAN_POINT('Ctrl Pts',(75.1645636494145,13.0725467650836,-6.00799829553516));
#51945=CARTESIAN_POINT('Ctrl Pts',(75.244641386475,13.2327333351681,-6.95036646159278));
#51946=CARTESIAN_POINT('Ctrl Pts',(75.388561523126,13.398832966976,-8.28171045726725));
#51947=CARTESIAN_POINT('Ctrl Pts',(75.5307112116867,13.495115191397,-9.57979399837247));
#51948=CARTESIAN_POINT('Ctrl Pts',(75.6076903576886,13.5418896972981,-10.4684029145841));
#51949=CARTESIAN_POINT('Ctrl Pts',(75.6427125496599,13.5653831954232,-10.9705768831649));
#51950=CARTESIAN_POINT('Ctrl Pts',(75.6567949286975,13.5764163657282,-11.219687102322));
#51951=CARTESIAN_POINT('Ctrl Pts',(75.6659591397543,13.584614346601,-11.4068884650896));
#51952=CARTESIAN_POINT('Ctrl Pts',(75.6716655675417,13.5900814285709,-11.5428871613284));
#51953=CARTESIAN_POINT('Ctrl Pts',(75.6815054359044,13.5992084051951,-11.8080288277756));
#51954=CARTESIAN_POINT('Ctrl Pts',(75.694750288452,13.6113493218069,-12.2723888815295));
#51955=CARTESIAN_POINT('Ctrl Pts',(75.7071041132252,13.621656524442,-13.1891666318357));
#51956=CARTESIAN_POINT('Ctrl Pts',(75.6937196831686,13.606320519813,-14.4733937850652));
#51957=CARTESIAN_POINT('Ctrl Pts',(75.6670647741677,13.5781474141517,-15.6010295207835));
#51958=CARTESIAN_POINT('Ctrl Pts',(75.6527978341287,13.5628795901601,-16.343621465258));
#51959=CARTESIAN_POINT('Ctrl Pts',(75.644851449895,13.5543270872537,-16.8363600570689));
#51960=CARTESIAN_POINT('Ctrl Pts',(75.6413638372204,13.5504924104114,-17.2035737118605));
#51961=CARTESIAN_POINT('Ctrl Pts',(75.6406188912779,13.5495739023617,-17.5079155494171));
#51962=CARTESIAN_POINT('Ctrl Pts',(75.6403306860592,13.5492306750639,-17.6332689205196));
#51963=CARTESIAN_POINT('Ctrl Pts',(75.6397839187813,13.5486117359053,-17.8812884146137));
#51964=CARTESIAN_POINT('Ctrl Pts',(75.6392789801523,13.5480923740326,-18.1305446269046));
#51965=CARTESIAN_POINT('Ctrl Pts',(75.6388134337367,13.5476613064233,-18.3794207281482));
#51966=CARTESIAN_POINT('Ctrl Pts',(75.638538067035,13.5474270114781,-18.5351722177618));
#51967=CARTESIAN_POINT('Ctrl Pts',(75.6383268201157,13.5472593072431,-18.659770610816));
#51968=CARTESIAN_POINT('Ctrl Pts',(75.6381727881497,13.5471431295646,-18.7532550160439));
#51969=CARTESIAN_POINT('Ctrl Pts',(75.6380480220344,13.5470540416721,-18.8311735243319));
#51970=CARTESIAN_POINT('Ctrl Pts',(75.6379503208938,13.5469872704047,-18.8935211128262));
#51971=CARTESIAN_POINT('Ctrl Pts',(75.6371316346039,13.5464447006677,-19.423542940964));
#51972=CARTESIAN_POINT('Ctrl Pts',(75.6359351108233,13.5461755172403,-20.4390817726704));
#51973=CARTESIAN_POINT('Ctrl Pts',(75.634828360188,13.5467565616507,-21.9453949711133));
#51974=CARTESIAN_POINT('Ctrl Pts',(75.6342670266766,13.5469587534658,-22.9544223560489));
#51975=CARTESIAN_POINT('Ctrl Pts',(75.6338911420669,13.5467744906389,-23.5848356961732));
#51976=CARTESIAN_POINT('Ctrl Pts',(75.6337578246949,13.5467046700915,-23.8339636838752));
#51977=CARTESIAN_POINT('Ctrl Pts',(75.6335472035545,13.5465764365443,-24.333237735561));
#51978=CARTESIAN_POINT('Ctrl Pts',(75.6333112229087,13.5463810387052,-25.2086785091867));
#51979=CARTESIAN_POINT('Ctrl Pts',(75.633273505873,13.5461888092674,-26.4634348811356));
#51980=CARTESIAN_POINT('Ctrl Pts',(75.6334421176052,13.5460988580601,-27.9716593715141));
#51981=CARTESIAN_POINT('Ctrl Pts',(75.6335262374093,13.5461411274059,-28.9763405113967));
#51982=CARTESIAN_POINT('Ctrl Pts',(75.6335162580107,13.5461929051318,-29.5404813865156));
#51983=CARTESIAN_POINT('Ctrl Pts',(75.6335116717496,13.546205695701,-29.6658206594576));
#51984=CARTESIAN_POINT('Ctrl Pts',(75.6334941440586,13.5462364561623,-29.9165726274603));
#51985=CARTESIAN_POINT('Ctrl Pts',(75.6334441674742,13.5463038818912,-30.3555370725306));
#51986=CARTESIAN_POINT('Ctrl Pts',(75.6332866957545,13.5464864765899,-31.233946560225));
#51987=CARTESIAN_POINT('Ctrl Pts',(75.633012427691,13.5468616560165,-32.4894782454011));
#51988=CARTESIAN_POINT('Ctrl Pts',(75.6329779848593,13.5473140281086,-33.7439606386439));
#51989=CARTESIAN_POINT('Ctrl Pts',(75.6332773217597,13.547675246526,-34.7457481434029));
#51990=CARTESIAN_POINT('Ctrl Pts',(75.6335670343689,13.5478517301423,-35.2458674650133));
#51991=CARTESIAN_POINT('Ctrl Pts',(75.633848830281,13.5479780496411,-35.6215904838746));
#51992=CARTESIAN_POINT('Ctrl Pts',(75.6340681767887,13.5480441756403,-35.8734483901231));
#51993=CARTESIAN_POINT('Ctrl Pts',(75.6346144032638,13.5481148955266,-36.3762834856865));
#51994=CARTESIAN_POINT('Ctrl Pts',(75.6358149761765,13.5481248859595,-37.2546699759255));
#51995=CARTESIAN_POINT('Ctrl Pts',(75.6388918280923,13.5479599794559,-39.0064589139521));
#51996=CARTESIAN_POINT('Ctrl Pts',(75.64164937319,13.5485990819942,-40.5064445315137));
#51997=CARTESIAN_POINT('Ctrl Pts',(75.6428605986345,13.5506975221396,-41.7609180823806));
#51998=CARTESIAN_POINT('Ctrl Pts',(75.6431314381623,13.5508451721668,-42.1394333505526));
#51999=CARTESIAN_POINT('Ctrl Pts',(75.6433632198811,13.5504806601518,-42.6417446845613));
#52000=CARTESIAN_POINT('Ctrl Pts',(75.6435247248323,13.549883063377,-43.144287692992));
#52001=CARTESIAN_POINT('Ctrl Pts',(75.6436261736509,13.5489497761417,-43.7715478943923));
#52002=CARTESIAN_POINT('Ctrl Pts',(75.6436868543797,13.5483419216635,-44.5227689553694));
#52003=CARTESIAN_POINT('Ctrl Pts',(75.643770464559,13.5489307026378,-45.1469456734117));
#52004=CARTESIAN_POINT('Ctrl Pts',(75.6439086844781,13.5504500405917,-45.6449859955142));
#52005=CARTESIAN_POINT('Ctrl Pts',(75.6440605249743,13.5522152988932,-46.0177693785017));
#52006=CARTESIAN_POINT('Ctrl Pts',(75.6442733557844,13.5547047661443,-46.3897723471156));
#52007=CARTESIAN_POINT('Ctrl Pts',(75.644656281772,13.5591157996639,-46.8845688284039));
#52008=CARTESIAN_POINT('Ctrl Pts',(75.6450727331189,13.5638112097244,-47.2543912144994));
#52009=CARTESIAN_POINT('Ctrl Pts',(75.6456054473631,13.569620112677,-47.6236160183188));
#52010=CARTESIAN_POINT('Ctrl Pts',(75.6460158611401,13.5746647580007,-47.8579532218034));
#52011=CARTESIAN_POINT('Ctrl Pts',(75.6468902362759,13.5895954379087,-48.3395036708315));
#52012=CARTESIAN_POINT('Ctrl Pts',(75.6485756605151,13.6259076839064,-49.1907264409587));
#52013=CARTESIAN_POINT('Ctrl Pts',(75.6511845953537,13.6947708828899,-50.4450997762995));
#52014=CARTESIAN_POINT('Ctrl Pts',(75.6546283694998,13.760376303753,-52.0049425857155));
#52015=CARTESIAN_POINT('Ctrl Pts',(75.6575932745508,13.7599238349314,-53.0825947549811));
#52016=CARTESIAN_POINT('Ctrl Pts',(75.6599861051391,13.7342309340774,-53.7702079294383));
#52017=CARTESIAN_POINT('Ctrl Pts',(75.6612766328049,13.7172644585284,-54.0757846386637));
#52018=CARTESIAN_POINT('Ctrl Pts',(75.6642063201746,13.6662457593704,-54.6543510537387));
#52019=CARTESIAN_POINT('Ctrl Pts',(75.6698177772266,13.5417335286409,-55.6365739687886));
#52020=CARTESIAN_POINT('Ctrl Pts',(75.6803344558201,13.2231856481331,-57.4447430780544));
#52021=CARTESIAN_POINT('Ctrl Pts',(75.6812461445865,13.0596673289293,-58.7321420750093));
#52022=CARTESIAN_POINT('Ctrl Pts',(75.6863576792012,13.1064489388915,-59.4965882134124));
#52023=CARTESIAN_POINT('Ctrl Pts',(75.6868298303791,13.1140110602154,-59.6098960670077));
#52024=CARTESIAN_POINT('Ctrl Pts',(75.6878765509766,13.1316047602574,-59.8259658717656));
#52025=CARTESIAN_POINT('Ctrl Pts',(75.6896957250427,13.1707074094786,-60.2119341104625));
#52026=CARTESIAN_POINT('Ctrl Pts',(75.6934350108314,13.2796839737662,-60.9876625420266));
#52027=CARTESIAN_POINT('Ctrl Pts',(75.6976019424888,13.4705397296793,-61.8928354957714));
#52028=CARTESIAN_POINT('Ctrl Pts',(75.7014059645446,13.7166821115159,-62.8074682445014));
#52029=CARTESIAN_POINT('Ctrl Pts',(75.7033987287794,13.8735410785524,-63.3250187717106));
#52030=CARTESIAN_POINT('Ctrl Pts',(75.7046635121384,13.984796963924,-63.670703925322));
#52031=CARTESIAN_POINT('Ctrl Pts',(75.7054898861349,14.0606817798573,-63.9013515810976));
#52032=CARTESIAN_POINT('Ctrl Pts',(75.7062958025135,14.1390037284096,-64.1320971550734));
#52033=CARTESIAN_POINT('Ctrl Pts',(75.7069791147956,14.2095209049496,-64.3341496424494));
#52034=CARTESIAN_POINT('Ctrl Pts',(75.707363808776,14.2503552783613,-64.4496300809221));
#52035=CARTESIAN_POINT('Ctrl Pts',(75.7079366922177,14.3121216714576,-64.6228405330907));
#52036=CARTESIAN_POINT('Ctrl Pts',(75.7084008077015,14.3646731779577,-64.7672331121068));
#52037=CARTESIAN_POINT('Ctrl Pts',(75.7091894624142,14.4527084142938,-65.0056347430462));
#52038=CARTESIAN_POINT('Ctrl Pts',(75.7117295644385,14.5355494140757,-65.2185608369));
#52039=CARTESIAN_POINT('Ctrl Pts',(75.7156081698465,14.7248152544026,-65.6685602924904));
#52040=CARTESIAN_POINT('Ctrl Pts',(75.7221368537155,15.0933038646535,-66.4580645030462));
#52041=CARTESIAN_POINT('Ctrl Pts',(75.7305054466675,15.973436498,-68.0970319185886));
#52042=CARTESIAN_POINT('Ctrl Pts',(75.7285229169979,16.8715677772082,-69.5915478892842));
#52043=CARTESIAN_POINT('Ctrl Pts',(75.7230950724573,17.5030606903351,-70.79300135306));
#52044=CARTESIAN_POINT('Ctrl Pts',(75.7235707246569,17.6319456085467,-71.0375543406922));
#52045=CARTESIAN_POINT('Ctrl Pts',(75.7235352277703,17.897293641091,-71.5400698659183));
#52046=CARTESIAN_POINT('Ctrl Pts',(75.7238560437055,18.2272902790581,-72.1627996419));
#52047=CARTESIAN_POINT('Ctrl Pts',(75.7239705541676,18.6263398955066,-72.9134843431913));
#52048=CARTESIAN_POINT('Ctrl Pts',(75.7242235888834,19.4258440108923,-74.4139713263615));
#52049=CARTESIAN_POINT('Ctrl Pts',(75.7241877630892,20.0957322587687,-75.6668112765516));
#52050=CARTESIAN_POINT('Ctrl Pts',(75.7239228263678,21.0674470105801,-77.4942020668528));
#52051=CARTESIAN_POINT('Ctrl Pts',(75.7240381076587,21.5031469039378,-78.3134969859117));
#52052=CARTESIAN_POINT('Ctrl Pts',(75.7240381076589,21.9396684913276,-79.1344746880088));
#52053=CARTESIAN_POINT('Ctrl Pts',(77.5604728961388,8.92232863282295,24.831637685054));
#52054=CARTESIAN_POINT('Ctrl Pts',(77.5603493570431,8.9223354387487,24.7827883082522));
#52055=CARTESIAN_POINT('Ctrl Pts',(77.5602200765458,8.92234251567576,24.7339548685087));
#52056=CARTESIAN_POINT('Ctrl Pts',(77.5587043201865,8.92243143920465,24.1833245240063));
#52057=CARTESIAN_POINT('Ctrl Pts',(77.5541707126617,8.91819490443657,23.1672111498827));
#52058=CARTESIAN_POINT('Ctrl Pts',(77.5413564917759,8.90545159573916,21.1638460926666));
#52059=CARTESIAN_POINT('Ctrl Pts',(77.5316712108527,8.90605028564952,19.6764700508711));
#52060=CARTESIAN_POINT('Ctrl Pts',(77.5282133989158,8.92709808728221,18.448523681775));
#52061=CARTESIAN_POINT('Ctrl Pts',(77.5286669548489,8.93215210326381,17.9183992030719));
#52062=CARTESIAN_POINT('Ctrl Pts',(77.5346523607888,8.93339918176008,16.9032327124148));
#52063=CARTESIAN_POINT('Ctrl Pts',(77.5517074438493,8.93291389719877,15.1689361934228));
#52064=CARTESIAN_POINT('Ctrl Pts',(77.5545025014536,8.98867950575542,13.7837990376749));
#52065=CARTESIAN_POINT('Ctrl Pts',(77.5334676759905,9.12212002089865,12.6722367779447));
#52066=CARTESIAN_POINT('Ctrl Pts',(77.5228404246978,9.18526329919579,12.2029990094417));
#52067=CARTESIAN_POINT('Ctrl Pts',(77.4980025165873,9.33590048471274,11.2680893222593));
#52068=CARTESIAN_POINT('Ctrl Pts',(77.4599776567047,9.56976218287444,10.0770564394827));
#52069=CARTESIAN_POINT('Ctrl Pts',(77.4034435343428,9.90993885287635,8.62874999365388));
#52070=CARTESIAN_POINT('Ctrl Pts',(77.3556580024562,10.167949986372,7.65090706207837));
#52071=CARTESIAN_POINT('Ctrl Pts',(77.321538390164,10.3354614075502,7.03946341289537));
#52072=CARTESIAN_POINT('Ctrl Pts',(77.3107460750445,10.3972646607645,6.82714530720268));
#52073=CARTESIAN_POINT('Ctrl Pts',(77.2797603948243,10.5378416373698,6.37251376862689));
#52074=CARTESIAN_POINT('Ctrl Pts',(77.2107265384483,10.8110338890849,5.56040597038144));
#52075=CARTESIAN_POINT('Ctrl Pts',(77.0244884890886,11.4497714059702,3.83689517844971));
#52076=CARTESIAN_POINT('Ctrl Pts',(76.8477086808871,12.0394308712412,2.23618777764992));
#52077=CARTESIAN_POINT('Ctrl Pts',(76.8045266887848,12.3642912864388,1.02478882366062));
#52078=CARTESIAN_POINT('Ctrl Pts',(76.8018332405895,12.3998220875874,0.895053963897795));
#52079=CARTESIAN_POINT('Ctrl Pts',(76.7975599881676,12.4719209199013,0.627727535400199));
#52080=CARTESIAN_POINT('Ctrl Pts',(76.7961484035108,12.5954373158584,0.164847484187591));
#52081=CARTESIAN_POINT('Ctrl Pts',(76.8081210516562,12.7669303911879,-0.496937328452192));
#52082=CARTESIAN_POINT('Ctrl Pts',(76.8421695164869,12.9613919414899,-1.28751891755477));
#52083=CARTESIAN_POINT('Ctrl Pts',(76.907368785551,13.2023184560712,-2.34000853818552));
#52084=CARTESIAN_POINT('Ctrl Pts',(77.0165417606542,13.4604237900536,-3.65296048391174));
#52085=CARTESIAN_POINT('Ctrl Pts',(77.1017261429008,13.6092121570947,-4.70299436939395));
#52086=CARTESIAN_POINT('Ctrl Pts',(77.1431648681345,13.6839081189796,-5.36010504112367));
#52087=CARTESIAN_POINT('Ctrl Pts',(77.1600267658594,13.7126643979356,-5.64135389354874));
#52088=CARTESIAN_POINT('Ctrl Pts',(77.1964793930761,13.7580485585429,-6.18849990687238));
#52089=CARTESIAN_POINT('Ctrl Pts',(77.2650550752343,13.8119150283283,-7.13940043609606));
#52090=CARTESIAN_POINT('Ctrl Pts',(77.3689169294206,13.8308884985355,-8.45695460822024));
#52091=CARTESIAN_POINT('Ctrl Pts',(77.462013437121,13.816844559987,-9.72341652820403));
#52092=CARTESIAN_POINT('Ctrl Pts',(77.5127825171445,13.8093833979168,-10.5800335004951));
#52093=CARTESIAN_POINT('Ctrl Pts',(77.5362618868962,13.8084300066986,-11.0609219709444));
#52094=CARTESIAN_POINT('Ctrl Pts',(77.5459376584656,13.809491089976,-11.2982666676243));
#52095=CARTESIAN_POINT('Ctrl Pts',(77.5523645061952,13.8110319626543,-11.4761344552283));
#52096=CARTESIAN_POINT('Ctrl Pts',(77.5563684421625,13.8120414729932,-11.6047533692288));
#52097=CARTESIAN_POINT('Ctrl Pts',(77.563207858177,13.8137762526411,-11.8565333451865));
#52098=CARTESIAN_POINT('Ctrl Pts',(77.5722345549043,13.8162026642452,-12.2989412671837));
#52099=CARTESIAN_POINT('Ctrl Pts',(77.5797025409249,13.8189354435846,-13.1791858349696));
#52100=CARTESIAN_POINT('Ctrl Pts',(77.567442235306,13.8185734893195,-14.4318920297639));
#52101=CARTESIAN_POINT('Ctrl Pts',(77.5460838146306,13.8157763860591,-15.5573993650377));
#52102=CARTESIAN_POINT('Ctrl Pts',(77.5346131764236,13.8141983409583,-16.3094404958222));
#52103=CARTESIAN_POINT('Ctrl Pts',(77.5281856114487,13.8133451222479,-16.8112991818371));
#52104=CARTESIAN_POINT('Ctrl Pts',(77.5252183902111,13.8130219840261,-17.1885933255562));
#52105=CARTESIAN_POINT('Ctrl Pts',(77.5243996636297,13.8130791069995,-17.5028139971062));
#52106=CARTESIAN_POINT('Ctrl Pts',(77.5240871618263,13.8130991471089,-17.6275881030977));
#52107=CARTESIAN_POINT('Ctrl Pts',(77.5235038017461,13.8131319862885,-17.8770200759137));
#52108=CARTESIAN_POINT('Ctrl Pts',(77.5229737621476,13.8131503186923,-18.1266527225266));
#52109=CARTESIAN_POINT('Ctrl Pts',(77.5225027146661,13.8131612174878,-18.3763532857022));
#52110=CARTESIAN_POINT('Ctrl Pts',(77.5222286852055,13.8131635716777,-18.5324781127209));
#52111=CARTESIAN_POINT('Ctrl Pts',(77.5220225660326,13.8131636975449,-18.6574033620728));
#52112=CARTESIAN_POINT('Ctrl Pts',(77.5218738432195,13.813162692245,-18.751114001786));
#52113=CARTESIAN_POINT('Ctrl Pts',(77.521754696824,13.8131609973018,-18.8292191327213));
#52114=CARTESIAN_POINT('Ctrl Pts',(77.5216623650211,13.8131592229898,-18.8917108710437));
#52115=CARTESIAN_POINT('Ctrl Pts',(77.5208923228423,13.8131409579113,-19.4229383341762));
#52116=CARTESIAN_POINT('Ctrl Pts',(77.5198724781134,13.8130142665158,-20.4400567461457));
#52117=CARTESIAN_POINT('Ctrl Pts',(77.5191849299256,13.8127636053189,-21.9468185573054));
#52118=CARTESIAN_POINT('Ctrl Pts',(77.5188102789848,13.8126523539833,-22.9548510961017));
#52119=CARTESIAN_POINT('Ctrl Pts',(77.5184901432129,13.8126348355234,-23.5842786925733));
#52120=CARTESIAN_POINT('Ctrl Pts',(77.518378556833,13.8126299471196,-23.833530244898));
#52121=CARTESIAN_POINT('Ctrl Pts',(77.5182042363923,13.8126263820134,-24.3327687054052));
#52122=CARTESIAN_POINT('Ctrl Pts',(77.5180151513301,13.8126344714252,-25.208307411824));
#52123=CARTESIAN_POINT('Ctrl Pts',(77.5180051341375,13.8126742818782,-26.4631549208369));
#52124=CARTESIAN_POINT('Ctrl Pts',(77.5181998543373,13.8127276901683,-27.9716117860686));
#52125=CARTESIAN_POINT('Ctrl Pts',(77.5183118867057,13.8127381523655,-28.9764795533715));
#52126=CARTESIAN_POINT('Ctrl Pts',(77.5183308400025,13.8127295345326,-29.5407447854088));
#52127=CARTESIAN_POINT('Ctrl Pts',(77.5183339048034,13.812727087905,-29.666131624305));
#52128=CARTESIAN_POINT('Ctrl Pts',(77.5183347783658,13.8127200803141,-29.9169621574733));
#52129=CARTESIAN_POINT('Ctrl Pts',(77.5183243363575,13.8127027278597,-30.3560580092875));
#52130=CARTESIAN_POINT('Ctrl Pts',(77.518269227131,13.8126510859042,-31.2346771096834));
#52131=CARTESIAN_POINT('Ctrl Pts',(77.5181715016671,13.8125492224116,-32.4903732179553));
#52132=CARTESIAN_POINT('Ctrl Pts',(77.5182537665264,13.8124629578631,-33.7448337842219));
#52133=CARTESIAN_POINT('Ctrl Pts',(77.5185517121816,13.8124355035215,-34.7464923619268));
#52134=CARTESIAN_POINT('Ctrl Pts',(77.5187986221067,13.8124413142602,-35.2465094381523));
#52135=CARTESIAN_POINT('Ctrl Pts',(77.5190288078211,13.8124547826457,-35.6221430941577));
#52136=CARTESIAN_POINT('Ctrl Pts',(77.5192053564713,13.8124450077209,-35.8740052140173));
#52137=CARTESIAN_POINT('Ctrl Pts',(77.5196367643728,13.8123646406697,-36.3768122071899));
#52138=CARTESIAN_POINT('Ctrl Pts',(77.5205700476009,13.8121075927323,-37.2551664983108));
#52139=CARTESIAN_POINT('Ctrl Pts',(77.5229237682906,13.8114319945058,-39.0068748203133));
#52140=CARTESIAN_POINT('Ctrl Pts',(77.5250122180607,13.8116906843296,-40.5067882721922));
#52141=CARTESIAN_POINT('Ctrl Pts',(77.5259381954873,13.813562957597,-41.7611981469901));
#52142=CARTESIAN_POINT('Ctrl Pts',(77.5261466829081,13.8136486587969,-42.1397048423366));
#52143=CARTESIAN_POINT('Ctrl Pts',(77.5263276066643,13.8132122244767,-42.6419967409788));
#52144=CARTESIAN_POINT('Ctrl Pts',(77.5264555505707,13.8125484706242,-43.1445197670677));
#52145=CARTESIAN_POINT('Ctrl Pts',(77.5265392299621,13.8115434069221,-43.771750998851));
#52146=CARTESIAN_POINT('Ctrl Pts',(77.5265911327969,13.8108650239228,-44.5229319723421));
#52147=CARTESIAN_POINT('Ctrl Pts',(77.5266560653333,13.8114066209184,-45.1470702553536));
#52148=CARTESIAN_POINT('Ctrl Pts',(77.526759449157,13.8128950100562,-45.6450776120453));
#52149=CARTESIAN_POINT('Ctrl Pts',(77.5268719395928,13.8146399341467,-46.0178347404532));
#52150=CARTESIAN_POINT('Ctrl Pts',(77.527028916975,13.8171118245038,-46.3898099848536));
#52151=CARTESIAN_POINT('Ctrl Pts',(77.5273111040197,13.8215026578271,-46.8845677443817));
#52152=CARTESIAN_POINT('Ctrl Pts',(77.5276172544658,13.8261866864606,-47.2543582726095));
#52153=CARTESIAN_POINT('Ctrl Pts',(77.5280099686407,13.8319856870836,-47.6235498894623));
#52154=CARTESIAN_POINT('Ctrl Pts',(77.5283224254491,13.8370251439549,-47.8578555760083));
#52155=CARTESIAN_POINT('Ctrl Pts',(77.5289836202813,13.8519535520393,-48.339354009538));
#52156=CARTESIAN_POINT('Ctrl Pts',(77.5302513326552,13.8882797198523,-49.1904957378282));
#52157=CARTESIAN_POINT('Ctrl Pts',(77.5321365443416,13.9572103613029,-50.4447910137057));
#52158=CARTESIAN_POINT('Ctrl Pts',(77.5345196910022,14.0229255419454,-52.0045983515733));
#52159=CARTESIAN_POINT('Ctrl Pts',(77.5366551468569,14.0225402161045,-53.0822690254463));
#52160=CARTESIAN_POINT('Ctrl Pts',(77.5384933987961,13.9968718774403,-53.7699066660649));
#52161=CARTESIAN_POINT('Ctrl Pts',(77.539544778281,13.9799211159562,-54.0754555282557));
#52162=CARTESIAN_POINT('Ctrl Pts',(77.5419458309468,13.9289293555925,-54.6539969527055));
#52163=CARTESIAN_POINT('Ctrl Pts',(77.5465201665502,13.8044596468729,-55.6361849190021));
#52164=CARTESIAN_POINT('Ctrl Pts',(77.5546852113387,13.485954960897,-57.4443545537156));
#52165=CARTESIAN_POINT('Ctrl Pts',(77.5536961524377,13.322378317418,-58.7318441547698));
#52166=CARTESIAN_POINT('Ctrl Pts',(77.5580618267775,13.3691275726486,-59.4964367021951));
#52167=CARTESIAN_POINT('Ctrl Pts',(77.5584463406522,13.3766868573184,-59.6097601494794));
#52168=CARTESIAN_POINT('Ctrl Pts',(77.5593301880504,13.3942737779871,-59.825860501517));
#52169=CARTESIAN_POINT('Ctrl Pts',(77.5608951149712,13.4333639449777,-60.2118774121813));
#52170=CARTESIAN_POINT('Ctrl Pts',(77.5642389625225,13.5423107223386,-60.9876858226565));
#52171=CARTESIAN_POINT('Ctrl Pts',(77.5681638311065,13.7331210512987,-61.8929098456432));
#52172=CARTESIAN_POINT('Ctrl Pts',(77.571838979276,13.979209515868,-62.8075572239394));
#52173=CARTESIAN_POINT('Ctrl Pts',(77.573783286313,14.136036565878,-63.3251031269268));
#52174=CARTESIAN_POINT('Ctrl Pts',(77.5750180640539,14.2472713001593,-63.6707801762678));
#52175=CARTESIAN_POINT('Ctrl Pts',(77.5758245506604,14.3231420864373,-63.9014210705629));
#52176=CARTESIAN_POINT('Ctrl Pts',(77.5766099015153,14.4014502698545,-64.1321579673947));
#52177=CARTESIAN_POINT('Ctrl Pts',(77.5772733489536,14.4719557255358,-64.3342011137818));
#52178=CARTESIAN_POINT('Ctrl Pts',(77.5776459531678,14.5127835239758,-64.4496757244623));
#52179=CARTESIAN_POINT('Ctrl Pts',(77.5781998706167,14.5745401929167,-64.6228769593256));
#52180=CARTESIAN_POINT('Ctrl Pts',(77.5786462129329,14.6270838893925,-64.767260806259));
#52181=CARTESIAN_POINT('Ctrl Pts',(77.5794018194922,14.7151068641564,-65.0056469865528));
#52182=CARTESIAN_POINT('Ctrl Pts',(77.5819117301522,14.7979431048304,-65.2185757513146));
#52183=CARTESIAN_POINT('Ctrl Pts',(77.5857459671956,14.9871981458478,-65.6685704184725));
#52184=CARTESIAN_POINT('Ctrl Pts',(77.592233829575,15.3556765477811,-66.4580724905346));
#52185=CARTESIAN_POINT('Ctrl Pts',(77.6006340957855,16.2358080969961,-68.0970343525443));
#52186=CARTESIAN_POINT('Ctrl Pts',(77.5987537175233,17.1339558157083,-69.5915520005254));
#52187=CARTESIAN_POINT('Ctrl Pts',(77.5933231368364,17.7654478982166,-70.7930076564631));
#52188=CARTESIAN_POINT('Ctrl Pts',(77.5937988748601,17.8943323860493,-71.0375602056355));
#52189=CARTESIAN_POINT('Ctrl Pts',(77.5937632152446,18.1596798707538,-71.5400754235968));
#52190=CARTESIAN_POINT('Ctrl Pts',(77.5940840363107,18.4896760382719,-72.1628047274669));
#52191=CARTESIAN_POINT('Ctrl Pts',(77.5941985862454,18.8887254494592,-72.9134890727134));
#52192=CARTESIAN_POINT('Ctrl Pts',(77.5944518616113,19.6882296468342,-74.4139755411582));
#52193=CARTESIAN_POINT('Ctrl Pts',(77.5944162020427,20.3581187868093,-75.6668158277755));
#52194=CARTESIAN_POINT('Ctrl Pts',(77.5941510398116,21.3298339704383,-77.4942075157172));
#52195=CARTESIAN_POINT('Ctrl Pts',(77.5942663414283,21.7655337658572,-78.3135022343861));
#52196=CARTESIAN_POINT('Ctrl Pts',(77.5942663414295,22.2020553532467,-79.1344799364846));
#52197=CARTESIAN_POINT('Ctrl Pts',(78.4944431928074,9.05472319120301,24.8422120491812));
#52198=CARTESIAN_POINT('Ctrl Pts',(78.4941090996625,9.05495389158687,24.79369851169));
#52199=CARTESIAN_POINT('Ctrl Pts',(78.493759402762,9.05519524519429,24.7452129330012));
#52200=CARTESIAN_POINT('Ctrl Pts',(78.4896386357447,9.05804650036688,24.1983783588369));
#52201=CARTESIAN_POINT('Ctrl Pts',(78.4798996030533,9.05886922538468,23.181079865532));
#52202=CARTESIAN_POINT('Ctrl Pts',(78.4531620503516,9.05915179220653,21.1871854887968));
#52203=CARTESIAN_POINT('Ctrl Pts',(78.4266520106487,9.07673406666645,19.710806800959));
#52204=CARTESIAN_POINT('Ctrl Pts',(78.4037275756009,9.11889086547707,18.495513535801));
#52205=CARTESIAN_POINT('Ctrl Pts',(78.3942568697667,9.13425597018717,17.9735746968858));
#52206=CARTESIAN_POINT('Ctrl Pts',(78.3756192466889,9.15833365518852,16.9680112857039));
#52207=CARTESIAN_POINT('Ctrl Pts',(78.3429789670015,9.20099516530317,15.2406404115276));
#52208=CARTESIAN_POINT('Ctrl Pts',(78.3159389388634,9.29108207535428,13.8416153133473));
#52209=CARTESIAN_POINT('Ctrl Pts',(78.2930576982901,9.4564531271892,12.7110753825502));
#52210=CARTESIAN_POINT('Ctrl Pts',(78.2829059329715,9.5323412143847,12.243553384385));
#52211=CARTESIAN_POINT('Ctrl Pts',(78.2620281608176,9.71268002071975,11.304618676111));
#52212=CARTESIAN_POINT('Ctrl Pts',(78.2337441668383,9.98800839152576,10.1083439598779));
#52213=CARTESIAN_POINT('Ctrl Pts',(78.1943694058521,10.3776671196108,8.64933905863135));
#52214=CARTESIAN_POINT('Ctrl Pts',(78.1617028150339,10.6634373708522,7.66204859777137));
#52215=CARTESIAN_POINT('Ctrl Pts',(78.138675834175,10.8451931975712,7.04333807577186));
#52216=CARTESIAN_POINT('Ctrl Pts',(78.133284707382,10.91279587007,6.83011630244702));
#52217=CARTESIAN_POINT('Ctrl Pts',(78.1148497326943,11.0649203335883,6.3732471355136));
#52218=CARTESIAN_POINT('Ctrl Pts',(78.0724604624009,11.3579055907103,5.55881360490552));
#52219=CARTESIAN_POINT('Ctrl Pts',(77.9531033376769,12.0288023749603,3.83067103963575));
#52220=CARTESIAN_POINT('Ctrl Pts',(77.8409734441138,12.6322082264952,2.21796256708511));
#52221=CARTESIAN_POINT('Ctrl Pts',(77.8219828150867,12.9419384726309,0.991072244389946));
#52222=CARTESIAN_POINT('Ctrl Pts',(77.8215972792297,12.975935451507,0.857316122256786));
#52223=CARTESIAN_POINT('Ctrl Pts',(77.8219267219958,13.0435170228269,0.58349967768362));
#52224=CARTESIAN_POINT('Ctrl Pts',(77.8276567418555,13.1564000121974,0.109434330121606));
#52225=CARTESIAN_POINT('Ctrl Pts',(77.8480946596581,13.3048998846505,-0.565528789552421));
#52226=CARTESIAN_POINT('Ctrl Pts',(77.8890671108874,13.4621622433645,-1.36765415444729));
#52227=CARTESIAN_POINT('Ctrl Pts',(77.9598017899087,13.6450089607257,-2.42939005995793));
#52228=CARTESIAN_POINT('Ctrl Pts',(78.0673887569699,13.8241004616619,-3.74124171730161));
#52229=CARTESIAN_POINT('Ctrl Pts',(78.1457996681103,13.9209575761983,-4.77638478515412));
#52230=CARTESIAN_POINT('Ctrl Pts',(78.1830513985844,13.970442181397,-5.42026114022125));
#52231=CARTESIAN_POINT('Ctrl Pts',(78.1978295335833,13.9887362190921,-5.70206761049167));
#52232=CARTESIAN_POINT('Ctrl Pts',(78.2283353769435,14.0140207271012,-6.24661171807938));
#52233=CARTESIAN_POINT('Ctrl Pts',(78.2827028003512,14.0343205019205,-7.19391202090573));
#52234=CARTESIAN_POINT('Ctrl Pts',(78.359136378551,14.0116016943059,-8.50391706664852));
#52235=CARTESIAN_POINT('Ctrl Pts',(78.423976017323,13.9655408145372,-9.76132343244577));
#52236=CARTESIAN_POINT('Ctrl Pts',(78.4589425569872,13.9419477084446,-10.6099258168552));
#52237=CARTESIAN_POINT('Ctrl Pts',(78.4753458853024,13.9336425316214,-11.0859840763551));
#52238=CARTESIAN_POINT('Ctrl Pts',(78.4822600622728,13.9316444870457,-11.3208245121042));
#52239=CARTESIAN_POINT('Ctrl Pts',(78.4869465685096,13.9311036750484,-11.4967517629155));
#52240=CARTESIAN_POINT('Ctrl Pts',(78.4898770373256,13.9307321440272,-11.623045554729));
#52241=CARTESIAN_POINT('Ctrl Pts',(78.4948702825629,13.9301885643896,-11.8709732103692));
#52242=CARTESIAN_POINT('Ctrl Pts',(78.5014546892992,13.9296568401639,-12.3068657247852));
#52243=CARTESIAN_POINT('Ctrl Pts',(78.5069032837125,13.9302020950339,-13.1764570240478));
#52244=CARTESIAN_POINT('Ctrl Pts',(78.4978378653358,13.9344964994918,-14.4200848218227));
#52245=CARTESIAN_POINT('Ctrl Pts',(78.4820063937416,13.9395702721035,-15.5449319278543));
#52246=CARTESIAN_POINT('Ctrl Pts',(78.4734805308755,13.9422589450028,-16.2996340877095));
#52247=CARTESIAN_POINT('Ctrl Pts',(78.4686845731225,13.9437987418975,-16.8040935922028));
#52248=CARTESIAN_POINT('Ctrl Pts',(78.466476154674,13.9445889988638,-17.1842831031095));
#52249=CARTESIAN_POINT('Ctrl Pts',(78.4658437641202,13.9449513613105,-17.5013555911005));
#52250=CARTESIAN_POINT('Ctrl Pts',(78.4656010874182,13.9450851860882,-17.6259547666494));
#52251=CARTESIAN_POINT('Ctrl Pts',(78.4651447089073,13.9453221683621,-17.8757847301294));
#52252=CARTESIAN_POINT('Ctrl Pts',(78.4647301387349,13.9455144798975,-18.1255167174223));
#52253=CARTESIAN_POINT('Ctrl Pts',(78.4643542822628,13.9456664704443,-18.3754473313692));
#52254=CARTESIAN_POINT('Ctrl Pts',(78.464134732944,13.945745754614,-18.5316753566071));
#52255=CARTESIAN_POINT('Ctrl Pts',(78.4639679306339,13.9458002634768,-18.6566914677372));
#52256=CARTESIAN_POINT('Ctrl Pts',(78.4638471299424,13.9458368577808,-18.7504649012776));
#52257=CARTESIAN_POINT('Ctrl Pts',(78.4637499605465,13.9458639021429,-18.8286219308702));
#52258=CARTESIAN_POINT('Ctrl Pts',(78.4636742768409,13.9458835255714,-18.8911537046507));
#52259=CARTESIAN_POINT('Ctrl Pts',(78.463042393415,13.9460392519842,-19.4227165195588));
#52260=CARTESIAN_POINT('Ctrl Pts',(78.4621900746086,13.9459949146705,-20.440284171059));
#52261=CARTESIAN_POINT('Ctrl Pts',(78.4615280251198,13.9455267728767,-21.9471797075837));
#52262=CARTESIAN_POINT('Ctrl Pts',(78.4611999873932,13.9453399496592,-22.9549425208703));
#52263=CARTESIAN_POINT('Ctrl Pts',(78.4609431021595,13.9453828946249,-23.5841025152867));
#52264=CARTESIAN_POINT('Ctrl Pts',(78.4608535890108,13.9454010566074,-23.8333894477468));
#52265=CARTESIAN_POINT('Ctrl Pts',(78.4607184682495,13.9454414150757,-24.3326208669306));
#52266=CARTESIAN_POINT('Ctrl Pts',(78.4605860170337,13.9455196094341,-25.2081915966555));
#52267=CARTESIAN_POINT('Ctrl Pts',(78.4606293995287,13.9456374044057,-26.4630707237769));
#52268=CARTESIAN_POINT('Ctrl Pts',(78.4608481281189,13.9457336479593,-27.9715986041808));
#52269=CARTESIAN_POINT('Ctrl Pts',(78.4609673331931,13.9457344249985,-28.9765203813875));
#52270=CARTESIAN_POINT('Ctrl Pts',(78.4609884526296,13.9457063344184,-29.540821666395));
#52271=CARTESIAN_POINT('Ctrl Pts',(78.4609918239648,13.9456988577156,-29.6662231086672));
#52272=CARTESIAN_POINT('Ctrl Pts',(78.4609937810264,13.9456794893836,-29.9170775082585));
#52273=CARTESIAN_POINT('Ctrl Pts',(78.4609860880103,13.9456348791229,-30.3562133193338));
#52274=CARTESIAN_POINT('Ctrl Pts',(78.4609380217542,13.9455082933016,-31.2348958299418));
#52275=CARTESIAN_POINT('Ctrl Pts',(78.4608427072243,13.9452560614607,-32.4906412365538));
#52276=CARTESIAN_POINT('Ctrl Pts',(78.4608903888004,13.9449994336256,-33.7450945241474));
#52277=CARTESIAN_POINT('Ctrl Pts',(78.4611216241635,13.9448455174262,-34.7467138347845));
#52278=CARTESIAN_POINT('Ctrl Pts',(78.4613193079934,13.9447958246403,-35.2466997987045));
#52279=CARTESIAN_POINT('Ctrl Pts',(78.461505640177,13.9447715070098,-35.6223062745813));
#52280=CARTESIAN_POINT('Ctrl Pts',(78.4616488668374,13.9447361246778,-35.8741696747715));
#52281=CARTESIAN_POINT('Ctrl Pts',(78.4620000281453,13.944603781278,-36.3769680926777));
#52282=CARTESIAN_POINT('Ctrl Pts',(78.4627607934637,13.9442552423288,-37.2553128588882));
#52283=CARTESIAN_POINT('Ctrl Pts',(78.4646856170524,13.9433973484837,-39.0069967046669));
#52284=CARTESIAN_POINT('Ctrl Pts',(78.4663917055818,13.9435233444552,-40.5068899646765));
#52285=CARTESIAN_POINT('Ctrl Pts',(78.46714472153,13.9453184823223,-41.7612812521414));
#52286=CARTESIAN_POINT('Ctrl Pts',(78.4673136122907,13.9453830940369,-42.1397854037017));
#52287=CARTESIAN_POINT('Ctrl Pts',(78.4674590403002,13.944922388335,-42.6420714137411));
#52288=CARTESIAN_POINT('Ctrl Pts',(78.4675606952721,13.944236753947,-43.1445884497504));
#52289=CARTESIAN_POINT('Ctrl Pts',(78.4676249130845,13.9432084599653,-43.7718110240772));
#52290=CARTESIAN_POINT('Ctrl Pts',(78.4676621414338,13.9425076337916,-44.5229801532958));
#52291=CARTESIAN_POINT('Ctrl Pts',(78.4677114744421,13.9430341003948,-45.1471072349507));
#52292=CARTESIAN_POINT('Ctrl Pts',(78.4677941646448,13.9445118311423,-45.6451047487846));
#52293=CARTESIAN_POINT('Ctrl Pts',(78.4678853687203,13.9462493848491,-46.0178540917725));
#52294=CARTESIAN_POINT('Ctrl Pts',(78.4680137314505,13.9487143687068,-46.3898211431151));
#52295=CARTESIAN_POINT('Ctrl Pts',(78.468245817902,13.9530964035972,-46.8845673874747));
#52296=CARTESIAN_POINT('Ctrl Pts',(78.4684987565137,13.9577740969672,-47.2543487119385));
#52297=CARTESIAN_POINT('Ctrl Pts',(78.4688242791751,13.9635665868806,-47.6235305269572));
#52298=CARTESIAN_POINT('Ctrl Pts',(78.4690901755611,13.9686021051196,-47.8578271204967));
#52299=CARTESIAN_POINT('Ctrl Pts',(78.4696516956716,13.9835247681664,-48.3393103767143));
#52300=CARTESIAN_POINT('Ctrl Pts',(78.4707272102901,14.0198457808104,-49.1904283932384));
#52301=CARTESIAN_POINT('Ctrl Pts',(78.4722864807893,14.0887798041541,-50.4447004336901));
#52302=CARTESIAN_POINT('Ctrl Pts',(78.4741878925538,14.1545044719243,-52.0044960602158));
#52303=CARTESIAN_POINT('Ctrl Pts',(78.4759415582901,14.1541186517246,-53.0821713407886));
#52304=CARTESIAN_POINT('Ctrl Pts',(78.4775197830763,14.128444258846,-53.7698156277294));
#52305=CARTESIAN_POINT('Ctrl Pts',(78.4784589984044,14.1114926364803,-54.0753552618592));
#52306=CARTESIAN_POINT('Ctrl Pts',(78.4806112561439,14.0604964950487,-54.6538882235983));
#52307=CARTESIAN_POINT('Ctrl Pts',(78.484696308313,13.9360143457923,-55.6360647242936));
#52308=CARTESIAN_POINT('Ctrl Pts',(78.4917435111746,13.6174640782452,-57.4442357062244));
#52309=CARTESIAN_POINT('Ctrl Pts',(78.489846084057,13.4538183235814,-58.7317543181104));
#52310=CARTESIAN_POINT('Ctrl Pts',(78.493853653258,13.5005381781814,-59.4963920782044));
#52311=CARTESIAN_POINT('Ctrl Pts',(78.4941958612439,13.5080944186318,-59.6097203083738));
#52312=CARTESIAN_POINT('Ctrl Pts',(78.4950009250074,13.5256751424072,-59.8258300484725));
#52313=CARTESIAN_POINT('Ctrl Pts',(78.4964423261334,13.5647549519809,-60.2118618619371));
#52314=CARTESIAN_POINT('Ctrl Pts',(78.4995917413089,13.6736820495239,-60.9876947443874));
#52315=CARTESIAN_POINT('Ctrl Pts',(78.5033926265082,13.864471271119,-61.8929344557591));
#52316=CARTESIAN_POINT('Ctrl Pts',(78.506997430927,14.1105389952847,-62.8075866886342));
#52317=CARTESIAN_POINT('Ctrl Pts',(78.5089138128884,14.2673546408238,-63.3251314947716));
#52318=CARTESIAN_POINT('Ctrl Pts',(78.5101313622486,14.3785819038062,-63.670806272742));
#52319=CARTESIAN_POINT('Ctrl Pts',(78.5109264734954,14.4544477553733,-63.9014452443889));
#52320=CARTESIAN_POINT('Ctrl Pts',(78.5117003346679,14.5327510772896,-64.1321796173828));
#52321=CARTESIAN_POINT('Ctrl Pts',(78.5123529433146,14.6032523571431,-64.3342200198336));
#52322=CARTESIAN_POINT('Ctrl Pts',(78.512719049699,14.6440777935191,-64.4496929092764));
#52323=CARTESIAN_POINT('Ctrl Pts',(78.5132628684145,14.7058309470756,-64.6228914140419));
#52324=CARTESIAN_POINT('Ctrl Pts',(78.5136999945135,14.7583717665777,-64.767272657901));
#52325=CARTESIAN_POINT('Ctrl Pts',(78.5144387501633,14.8463901122126,-65.0056542121464));
#52326=CARTESIAN_POINT('Ctrl Pts',(78.5169338299697,14.9292242776233,-65.2185839652863));
#52327=CARTESIAN_POINT('Ctrl Pts',(78.5207461591452,15.1184751040468,-65.6685774074326));
#52328=CARTESIAN_POINT('Ctrl Pts',(78.5272145085589,15.4869498109295,-66.4580791539563));
#52329=CARTESIAN_POINT('Ctrl Pts',(78.5356322362024,16.3670826107093,-68.0970395727417));
#52330=CARTESIAN_POINT('Ctrl Pts',(78.5338034505173,17.2652381054602,-69.5915577683127));
#52331=CARTESIAN_POINT('Ctrl Pts',(78.5283703489949,17.8967293937733,-70.7930139710155));
#52332=CARTESIAN_POINT('Ctrl Pts',(78.5288462002196,18.0256137916774,-71.0375664036789));
#52333=CARTESIAN_POINT('Ctrl Pts',(78.5288104159599,18.2909610994936,-71.540081533252));
#52334=CARTESIAN_POINT('Ctrl Pts',(78.5291313145272,18.620957153872,-72.1628107124065));
#52335=CARTESIAN_POINT('Ctrl Pts',(78.5292459193545,19.0200065150567,-72.9134949563425));
#52336=CARTESIAN_POINT('Ctrl Pts',(78.52949943309,19.8195107725196,-74.4139812784567));
#52337=CARTESIAN_POINT('Ctrl Pts',(78.5294640739157,20.489400205506,-75.6668216809661));
#52338=CARTESIAN_POINT('Ctrl Pts',(78.5291988379399,21.461115499897,-77.494213646795));
#52339=CARTESIAN_POINT('Ctrl Pts',(78.5293142151722,21.8968152797781,-78.3135083149078));
#52340=CARTESIAN_POINT('Ctrl Pts',(78.5293142151733,22.3333368671674,-79.1344860170071));
#52341=CARTESIAN_POINT('',(-4.76125591968157E-15,2.14773017928896,-8.66962570190719));
#52342=CARTESIAN_POINT('',(-10.8669314563932,2.70458533911839,-5.6515925146482));
#52343=CARTESIAN_POINT('Ctrl Pts',(-4.42970115563661E-15,2.14773017928896,
-8.66962570190719));
#52344=CARTESIAN_POINT('Ctrl Pts',(-0.732788448239405,2.14811194208377,
-8.63073774781089));
#52345=CARTESIAN_POINT('Ctrl Pts',(-2.74012589153777,2.08364837443475,-8.55044425906516));
#52346=CARTESIAN_POINT('Ctrl Pts',(-4.65602395402778,1.93383212333491,-8.52049681196753));
#52347=CARTESIAN_POINT('Ctrl Pts',(-6.35178884646186,1.89995064476493,-8.21329860288647));
#52348=CARTESIAN_POINT('Ctrl Pts',(-7.78927254448508,1.96366399905155,-7.6984650995689));
#52349=CARTESIAN_POINT('Ctrl Pts',(-9.41546628484877,2.25717994847875,-6.74202902301025));
#52350=CARTESIAN_POINT('Ctrl Pts',(-10.402035668676,2.55608056709905,-6.0139438933557));
#52351=CARTESIAN_POINT('Ctrl Pts',(-10.8669314563932,2.70458533911839,-5.6515925146482));
#52352=CARTESIAN_POINT('',(10.8669314593876,2.70458534007494,-5.65159251231429));
#52353=CARTESIAN_POINT('Ctrl Pts',(10.8669314593876,2.70458534007494,-5.65159251231429));
#52354=CARTESIAN_POINT('Ctrl Pts',(9.84130490508928,2.37696258947676,-6.45099144354073));
#52355=CARTESIAN_POINT('Ctrl Pts',(8.64584176151521,2.09714053636285,-7.22243788779773));
#52356=CARTESIAN_POINT('Ctrl Pts',(7.56815391157874,1.97195531073023,-7.75084487345448));
#52357=CARTESIAN_POINT('Ctrl Pts',(7.09293395924904,1.93789858980489,-7.93919586996905));
#52358=CARTESIAN_POINT('Ctrl Pts',(6.68079083609235,1.92043728607192,-8.08002239814288));
#52359=CARTESIAN_POINT('Ctrl Pts',(6.2887344545226,1.91141535836306,-8.19558998704663));
#52360=CARTESIAN_POINT('Ctrl Pts',(5.19190123252587,1.91538845500566,-8.4485082380012));
#52361=CARTESIAN_POINT('Ctrl Pts',(3.54842407610298,2.01867949236351,-8.54807461885338));
#52362=CARTESIAN_POINT('Ctrl Pts',(1.33100482704111,2.14842359650083,-8.598991326133));
#52363=CARTESIAN_POINT('Ctrl Pts',(-4.42970115563661E-15,2.14773017928896,
-8.66962570190719));
#52364=CARTESIAN_POINT('',(16.6867771002228,4.07882260827389,0.570992448038681));
#52365=CARTESIAN_POINT('Ctrl Pts',(16.6867770992602,4.0788226180366,0.570992448535458));
#52366=CARTESIAN_POINT('Ctrl Pts',(16.6866006155042,4.07881770793486,0.570746939936513));
#52367=CARTESIAN_POINT('Ctrl Pts',(16.6864241325273,4.07881279553261,0.570501437345728));
#52368=CARTESIAN_POINT('Ctrl Pts',(16.6862476503278,4.07880788082875,0.570255940758842));
#52369=CARTESIAN_POINT('Ctrl Pts',(16.6516203780579,4.07784357514131,0.522087472883436));
#52370=CARTESIAN_POINT('Ctrl Pts',(16.6169978550456,4.07676173618344,0.473723921485881));
#52371=CARTESIAN_POINT('Ctrl Pts',(16.5823724030183,4.07556338852267,0.425511095989113));
#52372=CARTESIAN_POINT('Ctrl Pts',(16.5692484174572,4.07510918225312,0.407237127314825));
#52373=CARTESIAN_POINT('Ctrl Pts',(16.5561240069721,4.07463825977875,0.388985341062362));
#52374=CARTESIAN_POINT('Ctrl Pts',(16.5429987376474,4.07415075972573,0.370776534107786));
#52375=CARTESIAN_POINT('Ctrl Pts',(16.4944642419689,4.07234808668097,0.303444181483954));
#52376=CARTESIAN_POINT('Ctrl Pts',(16.4459179975801,4.07031893631195,0.236703222909966));
#52377=CARTESIAN_POINT('Ctrl Pts',(16.3973395991362,4.0680420516515,0.170323522116401));
#52378=CARTESIAN_POINT('Ctrl Pts',(16.304432925526,4.06368748693193,0.0433716794553504));
#52379=CARTESIAN_POINT('Ctrl Pts',(16.2114090994963,4.05842679877864,-0.0822720722562958));
#52380=CARTESIAN_POINT('Ctrl Pts',(16.1181189016894,4.05213093153233,-0.206993715717981));
#52381=CARTESIAN_POINT('Ctrl Pts',(16.111845521893,4.05170756051037,-0.215380730181117));
#52382=CARTESIAN_POINT('Ctrl Pts',(16.1055709354821,4.05127950565539,-0.223763555358829));
#52383=CARTESIAN_POINT('Ctrl Pts',(16.0992950962031,4.05084672649476,-0.232142299942472));
#52384=CARTESIAN_POINT('Ctrl Pts',(16.0121664484622,4.04483837265388,-0.348465974416771));
#52385=CARTESIAN_POINT('Ctrl Pts',(15.9247963048648,4.03792023437012,-0.464003684927603));
#52386=CARTESIAN_POINT('Ctrl Pts',(15.8370636993764,4.0299759162962,-0.579152551411837));
#52387=CARTESIAN_POINT('Ctrl Pts',(15.7187187913346,4.01925960863978,-0.73448000281174));
#52388=CARTESIAN_POINT('Ctrl Pts',(15.5997216093824,4.00671090090665,-0.888472620810391));
#52389=CARTESIAN_POINT('Ctrl Pts',(15.4793949306149,3.992065579383,-1.04164356221155));
#52390=CARTESIAN_POINT('Ctrl Pts',(15.3596494685553,3.97749099949079,-1.19407463851209));
#52391=CARTESIAN_POINT('Ctrl Pts',(15.2385873144689,3.96084067042942,-1.34569398391442));
#52392=CARTESIAN_POINT('Ctrl Pts',(15.115550686801,3.94182264816488,-1.4969645929773));
#52393=CARTESIAN_POINT('Ctrl Pts',(15.0637667141605,3.93381829398767,-1.56063175640255));
#52394=CARTESIAN_POINT('Ctrl Pts',(15.0116332052113,3.9253940638159,-1.62423685097789));
#52395=CARTESIAN_POINT('Ctrl Pts',(14.9591024156658,3.9165262015244,-1.68781278599852));
#52396=CARTESIAN_POINT('Ctrl Pts',(14.9133737464421,3.908806623255,-1.7431563840731));
#52397=CARTESIAN_POINT('Ctrl Pts',(14.8673492403764,3.90075028178363,-1.79848155516262));
#52398=CARTESIAN_POINT('Ctrl Pts',(14.821108096381,3.89236131247767,-1.85368816089058));
#52399=CARTESIAN_POINT('Ctrl Pts',(14.7421989228348,3.87804577921783,-1.9478966353333));
#52400=CARTESIAN_POINT('Ctrl Pts',(14.6626580969073,3.8627588588919,-2.04175953296958));
#52401=CARTESIAN_POINT('Ctrl Pts',(14.5828955564093,3.84655993363014,-2.13478415056217));
#52402=CARTESIAN_POINT('Ctrl Pts',(14.5025695248271,3.83024656931088,-2.22846595061526));
#52403=CARTESIAN_POINT('Ctrl Pts',(14.422019141762,3.81300816310403,-2.32129716270607));
#52404=CARTESIAN_POINT('Ctrl Pts',(14.3416751210386,3.79495689677215,-2.41278157909349));
#52405=CARTESIAN_POINT('Ctrl Pts',(14.2674756527927,3.77828615573967,-2.49726944748248));
#52406=CARTESIAN_POINT('Ctrl Pts',(14.1934526773196,3.76092283109034,-2.58060847594324));
#52407=CARTESIAN_POINT('Ctrl Pts',(14.11994836497,3.74299347675259,-2.66241771614859));
#52408=CARTESIAN_POINT('Ctrl Pts',(14.091758713591,3.73611738700936,-2.69379239182739));
#52409=CARTESIAN_POINT('Ctrl Pts',(14.0636453423154,3.72915841731571,-2.7249421892367));
#52410=CARTESIAN_POINT('Ctrl Pts',(14.0356273648762,3.72212505706484,-2.75584609692576));
#52411=CARTESIAN_POINT('Ctrl Pts',(14.0158271275187,3.71715459826958,-2.77768581425887));
#52412=CARTESIAN_POINT('Ctrl Pts',(13.9960728675733,3.71214686676995,-2.79940253671174));
#52413=CARTESIAN_POINT('Ctrl Pts',(13.9763646379192,3.70710306984621,-2.82099787017943));
#52414=CARTESIAN_POINT('Ctrl Pts',(13.8574048089802,3.67665846727242,-2.95134834915652));
#52415=CARTESIAN_POINT('Ctrl Pts',(13.7401260229588,3.64490042631668,-3.07727439623639));
#52416=CARTESIAN_POINT('Ctrl Pts',(13.6244886164948,3.61215382052082,-3.19910641675052));
#52417=CARTESIAN_POINT('Ctrl Pts',(13.5036610600527,3.57793744987508,-3.32640661990492));
#52418=CARTESIAN_POINT('Ctrl Pts',(13.3846249977527,3.54264299708048,-3.44923749763812));
#52419=CARTESIAN_POINT('Ctrl Pts',(13.2672861145932,3.50662094584695,-3.56799588009648));
#52420=CARTESIAN_POINT('Ctrl Pts',(13.2291660948582,3.4949184200776,-3.60657705422325));
#52421=CARTESIAN_POINT('Ctrl Pts',(13.1912248612021,3.48313887990425,-3.64472853208236));
#52422=CARTESIAN_POINT('Ctrl Pts',(13.1534582886814,3.47129366217228,-3.68246420730061));
#52423=CARTESIAN_POINT('Ctrl Pts',(13.0350852174139,3.43416678755334,-3.8007404360869));
#52424=CARTESIAN_POINT('Ctrl Pts',(12.9183376887957,3.39636362404428,-3.91503983158288));
#52425=CARTESIAN_POINT('Ctrl Pts',(12.8032900468155,3.35831030135525,-4.02541934004456));
#52426=CARTESIAN_POINT('Ctrl Pts',(12.728600000419,3.33360571473129,-4.09707878882871));
#52427=CARTESIAN_POINT('Ctrl Pts',(12.6546256074055,3.30879546598555,-4.1670867890684));
#52428=CARTESIAN_POINT('Ctrl Pts',(12.5813792188602,3.28399106130667,-4.23546594227292));
#52429=CARTESIAN_POINT('Ctrl Pts',(12.4713187082152,3.24671979784344,-4.33821291271917));
#52430=CARTESIAN_POINT('Ctrl Pts',(12.3629026011617,3.20946416281579,-4.43728130970139));
#52431=CARTESIAN_POINT('Ctrl Pts',(12.2561598418245,3.17256125137376,-4.5327698916291));
#52432=CARTESIAN_POINT('Ctrl Pts',(12.149762552496,3.13577777519101,-4.62794942738419));
#52433=CARTESIAN_POINT('Ctrl Pts',(12.0450276505195,3.09934499196931,-4.71957257257733));
#52434=CARTESIAN_POINT('Ctrl Pts',(11.9419638342286,3.06355324889592,-4.80775726087006));
#52435=CARTESIAN_POINT('Ctrl Pts',(11.8377523564963,3.02736294884177,-4.89692392489513));
#52436=CARTESIAN_POINT('Ctrl Pts',(11.7352492971318,2.99182818284969,-4.98257537944035));
#52437=CARTESIAN_POINT('Ctrl Pts',(11.6344449097747,2.95720154072858,-5.06485012041152));
#52438=CARTESIAN_POINT('Ctrl Pts',(11.5323329411863,2.92212574010822,-5.1481920858352));
#52439=CARTESIAN_POINT('Ctrl Pts',(11.431963904345,2.88798175631234,-5.22806941702913));
#52440=CARTESIAN_POINT('Ctrl Pts',(11.3333099431412,2.85498269623455,-5.30463916990859));
#52441=CARTESIAN_POINT('Ctrl Pts',(11.2317900216267,2.82102499247617,-5.38343332280276));
#52442=CARTESIAN_POINT('Ctrl Pts',(11.1320861988524,2.78827966370978,-5.45872516267022));
#52443=CARTESIAN_POINT('Ctrl Pts',(11.0341506839636,2.75692715602264,-5.53069595057747));
#52444=CARTESIAN_POINT('Ctrl Pts',(10.9928851789487,2.74371665659696,-5.56102111824196));
#52445=CARTESIAN_POINT('Ctrl Pts',(10.9519334162765,2.73075282403085,-5.59075676961424));
#52446=CARTESIAN_POINT('Ctrl Pts',(10.9112909871464,2.71804658071908,-5.61991682939025));
#52447=CARTESIAN_POINT('Ctrl Pts',(10.8964872733027,2.71341842255918,-5.63053817240124));
#52448=CARTESIAN_POINT('Ctrl Pts',(10.8817245953344,2.70882442578679,-5.64108315195563));
#52449=CARTESIAN_POINT('Ctrl Pts',(10.867002428818,2.70426484961688,-5.65155246189065));
#52450=CARTESIAN_POINT('',(21.1401475865982,4.08070793355491,6.62997524452016));
#52451=CARTESIAN_POINT('Ctrl Pts',(21.1401277912671,4.08070389027384,6.62994920882078));
#52452=CARTESIAN_POINT('Ctrl Pts',(21.0563644921349,4.08064024620979,6.51979585635074));
#52453=CARTESIAN_POINT('Ctrl Pts',(20.9712950286701,4.08056610843344,6.40796762284914));
#52454=CARTESIAN_POINT('Ctrl Pts',(20.8846961507685,4.08048805817888,6.29405879478709));
#52455=CARTESIAN_POINT('Ctrl Pts',(20.8746571610368,4.08047901018978,6.28085389441233));
#52456=CARTESIAN_POINT('Ctrl Pts',(20.8645975893816,4.08046991265708,6.26762099621871));
#52457=CARTESIAN_POINT('Ctrl Pts',(20.8545170605049,4.08046077832543,6.25435943227145));
#52458=CARTESIAN_POINT('Ctrl Pts',(20.761284055216,4.08037629652872,6.1317056036129));
#52459=CARTESIAN_POINT('Ctrl Pts',(20.6662576987441,4.08028827813828,6.00659886428616));
#52460=CARTESIAN_POINT('Ctrl Pts',(20.5690642470972,4.08020917541913,5.87840956843418));
#52461=CARTESIAN_POINT('Ctrl Pts',(20.4326379910561,4.08009814234401,5.69847578275955));
#52462=CARTESIAN_POINT('Ctrl Pts',(20.2919440715206,4.08000319764964,5.51247161641301));
#52463=CARTESIAN_POINT('Ctrl Pts',(20.1459857511765,4.07997954828105,5.31870077800298));
#52464=CARTESIAN_POINT('Ctrl Pts',(20.1362693355262,4.0799779739474,5.30580149276543));
#52465=CARTESIAN_POINT('Ctrl Pts',(20.1265295797202,4.07997671576694,5.2928677727711));
#52466=CARTESIAN_POINT('Ctrl Pts',(20.1167661849073,4.07997579012312,5.2798991102106));
#52467=CARTESIAN_POINT('Ctrl Pts',(20.0785787432934,4.07997216966425,5.22917494573398));
#52468=CARTESIAN_POINT('Ctrl Pts',(20.0400297848654,4.07997378208828,5.17791638188733));
#52469=CARTESIAN_POINT('Ctrl Pts',(20.0011014776089,4.07998188596764,5.12609307809296));
#52470=CARTESIAN_POINT('Ctrl Pts',(19.9977449105617,4.07998258471918,5.12162464866327));
#52471=CARTESIAN_POINT('Ctrl Pts',(19.9943855153735,4.07998333231857,5.11715201016286));
#52472=CARTESIAN_POINT('Ctrl Pts',(19.9910232903037,4.0799841289361,5.11267515602838));
#52473=CARTESIAN_POINT('Ctrl Pts',(19.9642901914985,4.07999046285325,5.07707962585797));
#52474=CARTESIAN_POINT('Ctrl Pts',(19.9373781731281,4.07999989586757,5.04121756185854));
#52475=CARTESIAN_POINT('Ctrl Pts',(19.9102821059269,4.08001286913029,5.00507829021745));
#52476=CARTESIAN_POINT('Ctrl Pts',(19.8234646575681,4.08005443625358,4.88928586447036));
#52477=CARTESIAN_POINT('Ctrl Pts',(19.7347628514344,4.08013214834245,4.7706540119105));
#52478=CARTESIAN_POINT('Ctrl Pts',(19.6439993917317,4.08026028155559,4.64882337427558));
#52479=CARTESIAN_POINT('Ctrl Pts',(19.5975888619335,4.08032580054666,4.58652711037373));
#52480=CARTESIAN_POINT('Ctrl Pts',(19.5506396858042,4.08040449335367,4.52339509780919));
#52481=CARTESIAN_POINT('Ctrl Pts',(19.5031310854659,4.08049818336552,4.45938387691135));
#52482=CARTESIAN_POINT('Ctrl Pts',(19.4447501728308,4.08061331427568,4.38072372973177));
#52483=CARTESIAN_POINT('Ctrl Pts',(19.3856534202294,4.08074934835936,4.30091019527115));
#52484=CARTESIAN_POINT('Ctrl Pts',(19.3255293965389,4.080913099628,4.21949508424769));
#52485=CARTESIAN_POINT('Ctrl Pts',(19.2688772893524,4.0810673949305,4.14278136295625));
#52486=CARTESIAN_POINT('Ctrl Pts',(19.2113117835773,4.08124630895807,4.06464383760304));
#52487=CARTESIAN_POINT('Ctrl Pts',(19.153024043681,4.08144838923387,3.98535013860247));
#52488=CARTESIAN_POINT('Ctrl Pts',(19.1013031567088,4.08162770260444,3.91498988015165));
#52489=CARTESIAN_POINT('Ctrl Pts',(19.0489158781451,4.08182661596193,3.84358652788689));
#52490=CARTESIAN_POINT('Ctrl Pts',(18.9958265893946,4.08204565924289,3.77109062298675));
#52491=CARTESIAN_POINT('Ctrl Pts',(18.9587689592859,4.0821985568438,3.72048669719649));
#52492=CARTESIAN_POINT('Ctrl Pts',(18.9219798015889,4.08235871849574,3.67018402584651));
#52493=CARTESIAN_POINT('Ctrl Pts',(18.885449910933,4.0825252126899,3.62017431206734));
#52494=CARTESIAN_POINT('Ctrl Pts',(18.7893760662606,4.08296309347907,3.4886484468794));
#52495=CARTESIAN_POINT('Ctrl Pts',(18.6948839522869,4.08344449533075,3.35886253084306));
#52496=CARTESIAN_POINT('Ctrl Pts',(18.602321754467,4.08394799909736,3.23132511241665));
#52497=CARTESIAN_POINT('Ctrl Pts',(18.5589985833635,4.08418366095874,3.17163200301858));
#52498=CARTESIAN_POINT('Ctrl Pts',(18.5160990740038,4.08442424751788,3.11243192432935));
#52499=CARTESIAN_POINT('Ctrl Pts',(18.4734425356514,4.08466551982131,3.05348729325027));
#52500=CARTESIAN_POINT('Ctrl Pts',(18.3914292931626,4.08512940003032,2.9401578832974));
#52501=CARTESIAN_POINT('Ctrl Pts',(18.3106734624825,4.0855993150209,2.82826791101076));
#52502=CARTESIAN_POINT('Ctrl Pts',(18.2310417730918,4.08604651058148,2.71772553516501));
#52503=CARTESIAN_POINT('Ctrl Pts',(18.1756290479738,4.08635769730703,2.64080321525077));
#52504=CARTESIAN_POINT('Ctrl Pts',(18.1207596302947,4.08665785079446,2.56453223458843));
#52505=CARTESIAN_POINT('Ctrl Pts',(18.066379339977,4.08693723904721,2.4888705876708));
#52506=CARTESIAN_POINT('Ctrl Pts',(18.0192713524714,4.08717926457232,2.42332720978834));
#52507=CARTESIAN_POINT('Ctrl Pts',(17.9725602422526,4.08740424180746,2.35828267344141));
#52508=CARTESIAN_POINT('Ctrl Pts',(17.9261657622048,4.08760622745652,2.2936473939049));
#52509=CARTESIAN_POINT('Ctrl Pts',(17.8410139049816,4.08797694942886,2.17501659797828));
#52510=CARTESIAN_POINT('Ctrl Pts',(17.7569288166908,4.08827013511229,2.05776474700644));
#52511=CARTESIAN_POINT('Ctrl Pts',(17.6738446859609,4.08842721492592,1.94189413170338));
#52512=CARTESIAN_POINT('Ctrl Pts',(17.564867849343,4.08863324778726,1.78991308548242));
#52513=CARTESIAN_POINT('Ctrl Pts',(17.4575265240186,4.08860949102722,1.64018729925338));
#52514=CARTESIAN_POINT('Ctrl Pts',(17.3514015519163,4.08820812095149,1.49234200613465));
#52515=CARTESIAN_POINT('Ctrl Pts',(17.3352343295005,4.08814697568891,1.46981905334015));
#52516=CARTESIAN_POINT('Ctrl Pts',(17.3190953908043,4.08807705423024,1.44733982362486));
#52517=CARTESIAN_POINT('Ctrl Pts',(17.3029833106586,4.08799781807257,1.4249030794789));
#52518=CARTESIAN_POINT('Ctrl Pts',(17.2996967352419,4.08798165531732,1.42032638602437));
#52519=CARTESIAN_POINT('Ctrl Pts',(17.2964112608272,4.08796510254446,1.4157514373454));
#52520=CARTESIAN_POINT('Ctrl Pts',(17.2931268880962,4.08794815631246,1.41117824074195));
#52521=CARTESIAN_POINT('Ctrl Pts',(17.2201023048574,4.08757137461583,1.30949801033402));
#52522=CARTESIAN_POINT('Ctrl Pts',(17.1476227548266,4.08700004957664,1.20868450230697));
#52523=CARTESIAN_POINT('Ctrl Pts',(17.0755476342745,4.08617659776486,1.10861146158045));
#52524=CARTESIAN_POINT('Ctrl Pts',(16.9597498463747,4.08485361838562,0.947831477366912));
#52525=CARTESIAN_POINT('Ctrl Pts',(16.8449967071095,4.08288234496673,0.788964410925807));
#52526=CARTESIAN_POINT('Ctrl Pts',(16.7307073558031,4.07998384329684,0.63148608409984));
#52527=CARTESIAN_POINT('Ctrl Pts',(16.7159333272004,4.07960915793826,0.611129075522529));
#52528=CARTESIAN_POINT('Ctrl Pts',(16.7011671087498,4.07921864284779,0.590795559364228));
#52529=CARTESIAN_POINT('Ctrl Pts',(16.6867771007016,4.0788225980919,0.570992447894296));
#52530=CARTESIAN_POINT('',(25.4568055127483,4.08055401005754,12.6479974296003));
#52531=CARTESIAN_POINT('Ctrl Pts',(25.4568055127483,4.08055401005754,12.6479974296003));
#52532=CARTESIAN_POINT('Ctrl Pts',(25.2812500090543,4.0807927703833,12.3850689542157));
#52533=CARTESIAN_POINT('Ctrl Pts',(25.0429611356646,4.08107710014979,12.0284743263647));
#52534=CARTESIAN_POINT('Ctrl Pts',(24.5376155259781,4.08153855678031,11.2800885455859));
#52535=CARTESIAN_POINT('Ctrl Pts',(23.7755577618618,4.08195087821486,10.1719836389024));
#52536=CARTESIAN_POINT('Ctrl Pts',(22.5853601008239,4.08176221127767,8.52809651334861));
#52537=CARTESIAN_POINT('Ctrl Pts',(21.7185595769906,4.08113204177903,7.3898603299135));
#52538=CARTESIAN_POINT('Ctrl Pts',(21.1401574799756,4.0807159798154,6.62998826233519));
#52539=CARTESIAN_POINT('',(30.3134449388696,4.07585023121522,18.6659931355559));
#52540=CARTESIAN_POINT('Ctrl Pts',(30.3134449229822,4.07585757700923,18.6659931355313));
#52541=CARTESIAN_POINT('Ctrl Pts',(28.1961718099026,4.07126384474955,16.7705691222953));
#52542=CARTESIAN_POINT('Ctrl Pts',(26.9909999267723,4.07846746334965,14.9457506743408));
#52543=CARTESIAN_POINT('Ctrl Pts',(25.4568055127483,4.08055401005754,12.6479974296003));
#52544=CARTESIAN_POINT('',(43.9982567711944,4.57019451624003,24.6840336607938));
#52545=CARTESIAN_POINT('Ctrl Pts',(43.9982567712356,4.57019451569775,24.6840336607913));
#52546=CARTESIAN_POINT('Ctrl Pts',(43.6563954192405,4.54439404820984,24.6501193006367));
#52547=CARTESIAN_POINT('Ctrl Pts',(43.307245667739,4.51904928549701,24.6083964604157));
#52548=CARTESIAN_POINT('Ctrl Pts',(42.9531363255538,4.49443707659921,24.5592450950212));
#52549=CARTESIAN_POINT('Ctrl Pts',(42.6880707668603,4.4760138154056,24.5224532553921));
#52550=CARTESIAN_POINT('Ctrl Pts',(42.4202264763677,4.45800003649193,24.4814991107356));
#52551=CARTESIAN_POINT('Ctrl Pts',(42.1505826287051,4.44049282217423,24.4365424344902));
#52552=CARTESIAN_POINT('Ctrl Pts',(41.9700544718839,4.42877163825239,24.4064436728469));
#52553=CARTESIAN_POINT('Ctrl Pts',(41.7887197355172,4.41727717030993,24.3745508395979));
#52554=CARTESIAN_POINT('Ctrl Pts',(41.6068694434254,4.40603746857656,24.3409115700462));
#52555=CARTESIAN_POINT('Ctrl Pts',(41.1987030733588,4.38080974854174,24.2654076025424));
#52556=CARTESIAN_POINT('Ctrl Pts',(40.7879492108107,4.3568639312022,24.1811059500155));
#52557=CARTESIAN_POINT('Ctrl Pts',(40.3744467654769,4.33428844255932,24.0823265719964));
#52558=CARTESIAN_POINT('Ctrl Pts',(40.0624031037516,4.31725217537188,24.0077841378032));
#52559=CARTESIAN_POINT('Ctrl Pts',(39.7487808519831,4.3010002904592,23.9249989010293));
#52560=CARTESIAN_POINT('Ctrl Pts',(39.4359132798453,4.2856784881585,23.8348004629979));
#52561=CARTESIAN_POINT('Ctrl Pts',(39.413276747975,4.28456992818944,23.8282744436882));
#52562=CARTESIAN_POINT('Ctrl Pts',(39.3906441679139,4.28346621432707,23.8217096183546));
#52563=CARTESIAN_POINT('Ctrl Pts',(39.3680164239544,4.28236739107164,23.815106301441));
#52564=CARTESIAN_POINT('Ctrl Pts',(39.0567379154496,4.26725143144832,23.7242677872822));
#52565=CARTESIAN_POINT('Ctrl Pts',(38.7463740872753,4.25306528550943,23.6261449516955));
#52566=CARTESIAN_POINT('Ctrl Pts',(38.4392040695246,4.23988360976955,23.5215568239253));
#52567=CARTESIAN_POINT('Ctrl Pts',(38.2841859690802,4.23323127322697,23.4687748075857));
#52568=CARTESIAN_POINT('Ctrl Pts',(38.1299813891894,4.22683393748975,23.4143461882941));
#52569=CARTESIAN_POINT('Ctrl Pts',(37.9768840192784,4.22069622128782,23.358376409543));
#52570=CARTESIAN_POINT('Ctrl Pts',(37.8169834657751,4.21428576356078,23.2999195032816));
#52571=CARTESIAN_POINT('Ctrl Pts',(37.6582906920349,4.20815851721116,23.2397814235049));
#52572=CARTESIAN_POINT('Ctrl Pts',(37.501140466546,4.20231456368994,23.1780824960211));
#52573=CARTESIAN_POINT('Ctrl Pts',(37.2372789042477,4.19250233019609,23.0744875100938));
#52574=CARTESIAN_POINT('Ctrl Pts',(36.9777656061434,4.18349013246665,22.9664921446601));
#52575=CARTESIAN_POINT('Ctrl Pts',(36.7241912711045,4.17525629897779,22.8546669878381));
#52576=CARTESIAN_POINT('Ctrl Pts',(36.6777761731309,4.17374915044075,22.8341981355427));
#52577=CARTESIAN_POINT('Ctrl Pts',(36.631560268027,4.1722680138333,22.8136008994392));
#52578=CARTESIAN_POINT('Ctrl Pts',(36.5855442937473,4.17081238439013,22.7928811810314));
#52579=CARTESIAN_POINT('Ctrl Pts',(36.1877852789154,4.15823002049714,22.6137813160287));
#52580=CARTESIAN_POINT('Ctrl Pts',(35.8049617339917,4.14754953335667,22.4255293822829));
#52581=CARTESIAN_POINT('Ctrl Pts',(35.4375616951524,4.13840101146235,22.2319430741017));
#52582=CARTESIAN_POINT('Ctrl Pts',(35.0903110062494,4.1297542226915,22.0489736354198));
#52583=CARTESIAN_POINT('Ctrl Pts',(34.7568397309836,4.12247648315498,21.8612392508755));
#52584=CARTESIAN_POINT('Ctrl Pts',(34.4375796112242,4.11629332984187,21.6719653816336));
#52585=CARTESIAN_POINT('Ctrl Pts',(34.2188688560817,4.11205752948168,21.5423023629583));
#52586=CARTESIAN_POINT('Ctrl Pts',(34.006827791327,4.1083361809388,21.4119169089772));
#52587=CARTESIAN_POINT('Ctrl Pts',(33.8015966607754,4.10505052539575,21.2818452639727));
#52588=CARTESIAN_POINT('Ctrl Pts',(33.5101520730079,4.10038463225022,21.0971331452181));
#52589=CARTESIAN_POINT('Ctrl Pts',(33.2324412026286,4.09659432928849,20.9130543381718));
#52590=CARTESIAN_POINT('Ctrl Pts',(32.9688572095313,4.0934483100564,20.732570880017));
#52591=CARTESIAN_POINT('Ctrl Pts',(32.9185685258695,4.09284808709105,20.6981367877694));
#52592=CARTESIAN_POINT('Ctrl Pts',(32.868794031995,4.09227146343527,20.6638335403719));
#52593=CARTESIAN_POINT('Ctrl Pts',(32.8195364096049,4.09171703638411,20.6296816684234));
#52594=CARTESIAN_POINT('Ctrl Pts',(32.5448903765516,4.08862571400945,20.4392608625282));
#52595=CARTESIAN_POINT('Ctrl Pts',(32.2863121035037,4.08622000587309,20.253550189542));
#52596=CARTESIAN_POINT('Ctrl Pts',(32.0443288798291,4.08429089599327,20.0741560370317));
#52597=CARTESIAN_POINT('Ctrl Pts',(31.8158602799689,4.0824695257903,19.9047809447226));
#52598=CARTESIAN_POINT('Ctrl Pts',(31.6021849429662,4.08107388003582,19.7410364759486));
#52599=CARTESIAN_POINT('Ctrl Pts',(31.4037380340014,4.07996894633293,19.5842664599639));
#52600=CARTESIAN_POINT('Ctrl Pts',(31.2690106400237,4.07921879688951,19.4778338840288));
#52601=CARTESIAN_POINT('Ctrl Pts',(31.1413043559806,4.0786025832564,19.3746189789883));
#52602=CARTESIAN_POINT('Ctrl Pts',(31.0185339853794,4.0780801427807,19.2732361504699));
#52603=CARTESIAN_POINT('Ctrl Pts',(30.8391071505753,4.07731660479943,19.1250668492333));
#52604=CARTESIAN_POINT('Ctrl Pts',(30.6702229751989,4.07675152626773,18.9808100222224));
#52605=CARTESIAN_POINT('Ctrl Pts',(30.5053789318961,4.07630814667192,18.8361514122018));
#52606=CARTESIAN_POINT('Ctrl Pts',(30.4409125747783,4.07613475206942,18.7795790700843));
#52607=CARTESIAN_POINT('Ctrl Pts',(30.3770641474424,4.07598054873336,18.7229454371387));
#52608=CARTESIAN_POINT('Ctrl Pts',(30.3134449547349,4.07584288616601,18.6659931355875));
#52609=CARTESIAN_POINT('',(48.9436857109461,5.01442544687573,24.6839747938942));
#52610=CARTESIAN_POINT('Ctrl Pts',(48.9436857109461,5.01442544687573,24.6839747938942));
#52611=CARTESIAN_POINT('Ctrl Pts',(48.562059296251,4.9745603086499,24.7263748666625));
#52612=CARTESIAN_POINT('Ctrl Pts',(48.1741509009344,4.93536251604839,24.7583003138797));
#52613=CARTESIAN_POINT('Ctrl Pts',(47.4017479491975,4.85999473704396,24.8018982028682));
#52614=CARTESIAN_POINT('Ctrl Pts',(47.0216137408318,4.82422047595138,24.8130651984859));
#52615=CARTESIAN_POINT('Ctrl Pts',(45.7588804631496,4.70971082580307,24.8171749588499));
#52616=CARTESIAN_POINT('Ctrl Pts',(44.8709429698041,4.63605663134738,24.7706071307739));
#52617=CARTESIAN_POINT('Ctrl Pts',(43.9982567712502,4.57019451569886,24.6840336607964));
#52618=CARTESIAN_POINT('',(60.9536795918051,6.58767285120455,18.6650422826153));
#52619=CARTESIAN_POINT('Ctrl Pts',(60.9536837037562,6.58764335981454,18.6650422970777));
#52620=CARTESIAN_POINT('Ctrl Pts',(60.8748932120277,6.57672320333976,18.8030200801626));
#52621=CARTESIAN_POINT('Ctrl Pts',(60.7989278472826,6.56617190512782,18.9327111752887));
#52622=CARTESIAN_POINT('Ctrl Pts',(60.7243765115728,6.5557970610253,19.0561356442329));
#52623=CARTESIAN_POINT('Ctrl Pts',(60.6409508535265,6.54418723286943,19.194252117166));
#52624=CARTESIAN_POINT('Ctrl Pts',(60.5592962133145,6.53279847920326,19.3245213816899));
#52625=CARTESIAN_POINT('Ctrl Pts',(60.4775049273693,6.52136765023818,19.449789902365));
#52626=CARTESIAN_POINT('Ctrl Pts',(60.395713641424,6.5099368212731,19.57505842304));
#52627=CARTESIAN_POINT('Ctrl Pts',(60.313786862902,6.49846407086503,19.6953265126474));
#52628=CARTESIAN_POINT('Ctrl Pts',(60.2298692144609,6.48669009469553,19.8134515963786));
#52629=CARTESIAN_POINT('Ctrl Pts',(60.0741012759495,6.46483524020335,20.0327153760616));
#52630=CARTESIAN_POINT('Ctrl Pts',(59.9113909123673,6.44192971076875,20.2445747818266));
#52631=CARTESIAN_POINT('Ctrl Pts',(59.7396908055897,6.41768204830029,20.4483176667295));
#52632=CARTESIAN_POINT('Ctrl Pts',(59.5728651506258,6.3941227608394,20.646276426663));
#52633=CARTESIAN_POINT('Ctrl Pts',(59.3975528519521,6.36929636809518,20.836573053325));
#52634=CARTESIAN_POINT('Ctrl Pts',(59.2119236140565,6.34294486051316,21.0185603920136));
#52635=CARTESIAN_POINT('Ctrl Pts',(59.100465832935,6.32712256550406,21.1278314593971));
#52636=CARTESIAN_POINT('Ctrl Pts',(58.9852895190672,6.31075062049767,21.2341069843407));
#52637=CARTESIAN_POINT('Ctrl Pts',(58.8660073159028,6.29377513369926,21.3372477590069));
#52638=CARTESIAN_POINT('Ctrl Pts',(58.7509346282163,6.27739871845157,21.4367486555033));
#52639=CARTESIAN_POINT('Ctrl Pts',(58.6320408505898,6.26046044518029,21.5333321072928));
#52640=CARTESIAN_POINT('Ctrl Pts',(58.508979876986,6.24292110566031,21.626876022722));
#52641=CARTESIAN_POINT('Ctrl Pts',(58.4887780107034,6.24004182247823,21.6422323263145));
#52642=CARTESIAN_POINT('Ctrl Pts',(58.4684635545249,6.23714630659417,21.6575066607819));
#52643=CARTESIAN_POINT('Ctrl Pts',(58.4480394154578,6.23423502388466,21.672698581597));
#52644=CARTESIAN_POINT('Ctrl Pts',(58.2005563901708,6.19895847929953,21.8567818622138));
#52645=CARTESIAN_POINT('Ctrl Pts',(57.9369665378702,6.16136281992631,22.0287628026985));
#52646=CARTESIAN_POINT('Ctrl Pts',(57.6624596166534,6.12230615533265,22.1878640684998));
#52647=CARTESIAN_POINT('Ctrl Pts',(57.5773728776958,6.11020006995563,22.2371794293332));
#52648=CARTESIAN_POINT('Ctrl Pts',(57.4912374652112,6.0979539425225,22.2852575101044));
#52649=CARTESIAN_POINT('Ctrl Pts',(57.4042083778879,6.0855940225361,22.3320755299395));
#52650=CARTESIAN_POINT('Ctrl Pts',(57.2087214193683,6.05783085461144,22.4372393617452));
#52651=CARTESIAN_POINT('Ctrl Pts',(57.008734261632,6.02949259342333,22.536044413206));
#52652=CARTESIAN_POINT('Ctrl Pts',(56.7999697583721,6.00003337925011,22.6310713355561));
#52653=CARTESIAN_POINT('Ctrl Pts',(56.6080942544555,5.97295740859317,22.7184106021788));
#52654=CARTESIAN_POINT('Ctrl Pts',(56.4088045308582,5.94493368525431,22.8025582988609));
#52655=CARTESIAN_POINT('Ctrl Pts',(56.1988074787868,5.91557352121889,22.8855191124983));
#52656=CARTESIAN_POINT('Ctrl Pts',(56.1803234096789,5.91298922160278,22.892821374113));
#52657=CARTESIAN_POINT('Ctrl Pts',(56.161756401499,5.91039459699341,22.9001144410366));
#52658=CARTESIAN_POINT('Ctrl Pts',(56.1431042186586,5.9077894003739,22.9073996808841));
#52659=CARTESIAN_POINT('Ctrl Pts',(56.1156742180694,5.9039581841876,22.918113393859));
#52660=CARTESIAN_POINT('Ctrl Pts',(56.0880595906354,5.90010405620253,22.9288101736885));
#52661=CARTESIAN_POINT('Ctrl Pts',(56.0604141437415,5.89624864805948,22.9394423898106));
#52662=CARTESIAN_POINT('Ctrl Pts',(55.9718745527707,5.88390099959056,22.9734940030897));
#52663=CARTESIAN_POINT('Ctrl Pts',(55.883019639351,5.87154145844787,23.0068833672292));
#52664=CARTESIAN_POINT('Ctrl Pts',(55.7988925218622,5.85986943633177,23.0380458796224));
#52665=CARTESIAN_POINT('Ctrl Pts',(55.7294946088525,5.85024098358503,23.0637523746121));
#52666=CARTESIAN_POINT('Ctrl Pts',(55.6633188405804,5.84107739387149,23.087943519035));
#52667=CARTESIAN_POINT('Ctrl Pts',(55.586943735967,5.8305287518237,23.1150152712605));
#52668=CARTESIAN_POINT('Ctrl Pts',(55.5418250424742,5.82429712766124,23.1310079444903));
#52669=CARTESIAN_POINT('Ctrl Pts',(55.4931472946897,5.81758269461732,23.1480059080949));
#52670=CARTESIAN_POINT('Ctrl Pts',(55.4381475647196,5.81001182026829,23.166915463685));
#52671=CARTESIAN_POINT('Ctrl Pts',(55.42725455157,5.80851236501854,23.1706606100304));
#52672=CARTESIAN_POINT('Ctrl Pts',(55.4161134782451,5.80697932863549,23.1744807518226));
#52673=CARTESIAN_POINT('Ctrl Pts',(55.4047258589144,5.80541300399653,23.1783744667056));
#52674=CARTESIAN_POINT('Ctrl Pts',(55.2889072779726,5.78948258941978,23.2179757669642));
#52675=CARTESIAN_POINT('Ctrl Pts',(55.1475857888739,5.77010467587343,23.2651873818611));
#52676=CARTESIAN_POINT('Ctrl Pts',(54.9823558303551,5.74761445563296,23.318513632426));
#52677=CARTESIAN_POINT('Ctrl Pts',(54.8248950225142,5.7261817307244,23.3693324704161));
#52678=CARTESIAN_POINT('Ctrl Pts',(54.6457219044543,5.70192243219709,23.4257044042999));
#52679=CARTESIAN_POINT('Ctrl Pts',(54.4462107368371,5.67517291439529,23.4863366809526));
#52680=CARTESIAN_POINT('Ctrl Pts',(54.3159317007704,5.65770571475885,23.5259290238333));
#52681=CARTESIAN_POINT('Ctrl Pts',(54.1769804185357,5.63917762942309,23.5673380043009));
#52682=CARTESIAN_POINT('Ctrl Pts',(54.0297364015009,5.61969401951032,23.610204179057));
#52683=CARTESIAN_POINT('Ctrl Pts',(53.7970966485848,5.58891068252112,23.6779310484032));
#52684=CARTESIAN_POINT('Ctrl Pts',(53.543745884538,5.55574006612116,23.7492900999149));
#52685=CARTESIAN_POINT('Ctrl Pts',(53.2732679872795,5.52091196649709,23.8221539563539));
#52686=CARTESIAN_POINT('Ctrl Pts',(52.9749987252396,5.48250531043235,23.9025045096144));
#52687=CARTESIAN_POINT('Ctrl Pts',(52.6559018189042,5.44208830841857,23.9846854993892));
#52688=CARTESIAN_POINT('Ctrl Pts',(52.3207576286579,5.40057964484992,24.0658311066893));
#52689=CARTESIAN_POINT('Ctrl Pts',(52.1333765429832,5.37737190719322,24.1112000924457));
#52690=CARTESIAN_POINT('Ctrl Pts',(51.9409784566618,5.35382241515805,24.1562453376084));
#52691=CARTESIAN_POINT('Ctrl Pts',(51.7443946064197,5.33008577804881,24.2004655968722));
#52692=CARTESIAN_POINT('Ctrl Pts',(51.3432051841192,5.28164391612837,24.2907105495789));
#52693=CARTESIAN_POINT('Ctrl Pts',(50.9246090760015,5.23242789976439,24.3775258737374));
#52694=CARTESIAN_POINT('Ctrl Pts',(50.4929870595525,5.1833823052378,24.4556071075138));
#52695=CARTESIAN_POINT('Ctrl Pts',(50.1455722059097,5.14390524569282,24.5184551073167));
#52696=CARTESIAN_POINT('Ctrl Pts',(49.7897170355193,5.10453958577619,24.5756445440186));
#52697=CARTESIAN_POINT('Ctrl Pts',(49.427729627481,5.06568535151103,24.624411660777));
#52698=CARTESIAN_POINT('Ctrl Pts',(49.2675194938438,5.04848905703845,24.645995246613));
#52699=CARTESIAN_POINT('Ctrl Pts',(49.1061080943944,5.03139228669694,24.6659290919299));
#52700=CARTESIAN_POINT('Ctrl Pts',(48.9436951551741,5.01442643343101,24.6839737446064));
#52701=CARTESIAN_POINT('Ctrl Pts',(48.9436920070984,5.01442610457919,24.6839740943688));
#52702=CARTESIAN_POINT('Ctrl Pts',(48.9436888590223,5.01442577572742,24.6839744441305));
#52703=CARTESIAN_POINT('Ctrl Pts',(48.9436857109458,5.01442544687569,24.6839747938914));
#52704=CARTESIAN_POINT('',(63.880064779209,6.9882076388047,12.6528714883835));
#52705=CARTESIAN_POINT('Ctrl Pts',(63.880064779209,6.9882076388047,12.6528714883835));
#52706=CARTESIAN_POINT('Ctrl Pts',(63.7740445264651,6.97254843494423,12.8870707048835));
#52707=CARTESIAN_POINT('Ctrl Pts',(63.6123361644209,6.94905832898685,13.2403034399106));
#52708=CARTESIAN_POINT('Ctrl Pts',(63.2900524331968,6.90311702623842,13.9391278664585));
#52709=CARTESIAN_POINT('Ctrl Pts',(62.4853443970193,6.79282876561949,15.6488004126113));
#52710=CARTESIAN_POINT('Ctrl Pts',(61.5478879227764,6.66996297123436,17.6228958620238));
#52711=CARTESIAN_POINT('Ctrl Pts',(60.9536795918051,6.58767285120455,18.6650422826153));
#52712=CARTESIAN_POINT('',(66.3006594538148,7.32609989629238,6.62697998093854));
#52713=CARTESIAN_POINT('Ctrl Pts',(66.300659446523,7.32609992703372,6.62697998211673));
#52714=CARTESIAN_POINT('Ctrl Pts',(66.2961516437242,7.32560197128319,6.63876773876303));
#52715=CARTESIAN_POINT('Ctrl Pts',(66.2911264841868,7.32504638436974,6.65192702458933));
#52716=CARTESIAN_POINT('Ctrl Pts',(66.2861021175671,7.32449011260781,6.66510631411833));
#52717=CARTESIAN_POINT('Ctrl Pts',(66.2265869187196,7.31790089907496,6.8212191331768));
#52718=CARTESIAN_POINT('Ctrl Pts',(66.1665664874988,7.31115403387545,6.98156417267042));
#52719=CARTESIAN_POINT('Ctrl Pts',(66.1052920653522,7.30410522937434,7.14672695293512));
#52720=CARTESIAN_POINT('Ctrl Pts',(66.0780532869344,7.30097177144541,7.22014800232068));
#52721=CARTESIAN_POINT('Ctrl Pts',(66.0505665836933,7.29777863650945,7.29452052682466));
#52722=CARTESIAN_POINT('Ctrl Pts',(66.0227663772338,7.29451325221887,7.36989242818266));
#52723=CARTESIAN_POINT('Ctrl Pts',(65.9666413110708,7.28792085839536,7.52205867042603));
#52724=CARTESIAN_POINT('Ctrl Pts',(65.909236835321,7.28103353146028,7.6783020694003));
#52725=CARTESIAN_POINT('Ctrl Pts',(65.8500061686631,7.27374086686791,7.83903564120958));
#52726=CARTESIAN_POINT('Ctrl Pts',(65.8311638865591,7.27142094627116,7.89016772319501));
#52727=CARTESIAN_POINT('Ctrl Pts',(65.8121369439297,7.26906003851291,7.94175385688256));
#52728=CARTESIAN_POINT('Ctrl Pts',(65.7929082290069,7.2666546952333,7.99380629067399));
#52729=CARTESIAN_POINT('Ctrl Pts',(65.7752908491144,7.26445091580764,8.04149681518978));
#52730=CARTESIAN_POINT('Ctrl Pts',(65.7575039285222,7.2622097550886,8.08957923853654));
#52731=CARTESIAN_POINT('Ctrl Pts',(65.7395342230684,7.25992847772148,8.13806342420129));
#52732=CARTESIAN_POINT('Ctrl Pts',(65.6805357302456,7.25243854269072,8.29724766276983));
#52733=CARTESIAN_POINT('Ctrl Pts',(65.6195662658539,7.24451574763741,8.46076214982886));
#52734=CARTESIAN_POINT('Ctrl Pts',(65.5561656976303,7.2360675884905,8.62895040123494));
#52735=CARTESIAN_POINT('Ctrl Pts',(65.5431387561496,7.2343317416691,8.66350811215447));
#52736=CARTESIAN_POINT('Ctrl Pts',(65.5300092729086,7.23257373433867,8.69826299491312));
#52737=CARTESIAN_POINT('Ctrl Pts',(65.5167734110897,7.23079279556236,8.73321779621613));
#52738=CARTESIAN_POINT('Ctrl Pts',(65.4837676855844,7.22635174161383,8.82038314991143));
#52739=CARTESIAN_POINT('Ctrl Pts',(65.4501686905856,7.2217789113791,8.90861216197532));
#52740=CARTESIAN_POINT('Ctrl Pts',(65.4157860386741,7.21704230591978,8.99829403032095));
#52741=CARTESIAN_POINT('Ctrl Pts',(65.3746164943489,7.21137072802897,9.10567846545784));
#52742=CARTESIAN_POINT('Ctrl Pts',(65.3323234237302,7.20546441961582,9.21514745632922));
#52743=CARTESIAN_POINT('Ctrl Pts',(65.2890065927822,7.19933679696803,9.32633307246552));
#52744=CARTESIAN_POINT('Ctrl Pts',(65.2609113571545,7.19536242953717,9.39844790670901));
#52745=CARTESIAN_POINT('Ctrl Pts',(65.2323499986339,7.19128946807759,9.47137580262029));
#52746=CARTESIAN_POINT('Ctrl Pts',(65.2032963048797,7.18711403038382,9.54513708528809));
#52747=CARTESIAN_POINT('Ctrl Pts',(65.1896601075941,7.18515431081674,9.57975655264426));
#52748=CARTESIAN_POINT('Ctrl Pts',(65.1760188101892,7.18318688194893,9.614296963272));
#52749=CARTESIAN_POINT('Ctrl Pts',(65.1623711062258,7.18121190329217,9.64875990838282));
#52750=CARTESIAN_POINT('Ctrl Pts',(65.1239051352521,7.17564543790808,9.74589351047838));
#52751=CARTESIAN_POINT('Ctrl Pts',(65.0853174690523,7.1700104476921,9.84259099567689));
#52752=CARTESIAN_POINT('Ctrl Pts',(65.0467091952298,7.16432647860304,9.93853650237319));
#52753=CARTESIAN_POINT('Ctrl Pts',(65.0032832899394,7.157933250445,10.0464543156895));
#52754=CARTESIAN_POINT('Ctrl Pts',(64.9598301710589,7.15147790800914,10.1534246055419));
#52755=CARTESIAN_POINT('Ctrl Pts',(64.9161906946988,7.14495370650557,10.259929264202));
#52756=CARTESIAN_POINT('Ctrl Pts',(64.9110320486335,7.14418247712284,10.2725192374135));
#52757=CARTESIAN_POINT('Ctrl Pts',(64.9058719259585,7.14341042276849,10.2850999251361));
#52758=CARTESIAN_POINT('Ctrl Pts',(64.9007103369394,7.14263756622216,10.2976714500119));
#52759=CARTESIAN_POINT('Ctrl Pts',(64.8220237704832,7.13085564639699,10.4893198210735));
#52760=CARTESIAN_POINT('Ctrl Pts',(64.7429951170709,7.11888689900363,10.6788439805008));
#52761=CARTESIAN_POINT('Ctrl Pts',(64.6636556105198,7.10681277214228,10.8666766704469));
#52762=CARTESIAN_POINT('Ctrl Pts',(64.6542323662028,7.10537871422744,10.8889857747636));
#52763=CARTESIAN_POINT('Ctrl Pts',(64.6448047349602,7.10394316921425,10.9112709982386));
#52764=CARTESIAN_POINT('Ctrl Pts',(64.635372092164,7.10250614545892,10.9335340503097));
#52765=CARTESIAN_POINT('Ctrl Pts',(64.6040882617547,7.09774018448415,11.0073705731617));
#52766=CARTESIAN_POINT('Ctrl Pts',(64.5727530941267,7.0929587717943,11.0809541181071));
#52767=CARTESIAN_POINT('Ctrl Pts',(64.5413598033906,7.08816550566459,11.154309716269));
#52768=CARTESIAN_POINT('Ctrl Pts',(64.5177330860973,7.08455807423252,11.2095174354665));
#52769=CARTESIAN_POINT('Ctrl Pts',(64.4940763830003,7.08094447718144,11.2645891973131));
#52770=CARTESIAN_POINT('Ctrl Pts',(64.470382570531,7.07732545714221,11.3195459712094));
#52771=CARTESIAN_POINT('Ctrl Pts',(64.4035641046536,7.06711952817599,11.4745285146928));
#52772=CARTESIAN_POINT('Ctrl Pts',(64.3364505075205,7.05687048265302,11.6285966092296));
#52773=CARTESIAN_POINT('Ctrl Pts',(64.2690337523511,7.04661896634741,11.7819573743463));
#52774=CARTESIAN_POINT('Ctrl Pts',(64.2510791342558,7.04388875395878,11.822800840656));
#52775=CARTESIAN_POINT('Ctrl Pts',(64.2331023996129,7.04115822385004,11.8635955499663));
#52776=CARTESIAN_POINT('Ctrl Pts',(64.2151029610433,7.03842800906183,11.9043463944726));
#52777=CARTESIAN_POINT('Ctrl Pts',(64.1803315818,7.03315377045434,11.9830690203668));
#52778=CARTESIAN_POINT('Ctrl Pts',(64.1454755177022,7.02788073298689,12.0616278828523));
#52779=CARTESIAN_POINT('Ctrl Pts',(64.1105266707577,7.02261257245995,12.1400667643143));
#52780=CARTESIAN_POINT('Ctrl Pts',(64.0341919105036,7.01110593330125,12.3113918217761));
#52781=CARTESIAN_POINT('Ctrl Pts',(63.9574150642832,6.99962279118902,12.482143738577));
#52782=CARTESIAN_POINT('Ctrl Pts',(63.8801064158733,6.98820114899864,12.6527834466791));
#52783=CARTESIAN_POINT('',(71.7123823850219,8.64377894688336,1.033152900074));
#52784=CARTESIAN_POINT('Ctrl Pts',(71.7123823116865,8.64377889138672,1.0331528409219));
#52785=CARTESIAN_POINT('Ctrl Pts',(71.7085363523106,8.64137100788826,1.03413021557008));
#52786=CARTESIAN_POINT('Ctrl Pts',(71.7046868561564,8.63896427541392,1.03511038928643));
#52787=CARTESIAN_POINT('Ctrl Pts',(71.7008338384512,8.63655872418921,1.03609341408942));
#52788=CARTESIAN_POINT('Ctrl Pts',(71.6209904060947,8.58671014284756,1.05646396007881));
#52789=CARTESIAN_POINT('Ctrl Pts',(71.5396217322624,8.53745717547068,1.07756846979329));
#52790=CARTESIAN_POINT('Ctrl Pts',(71.456859049088,8.48908067659746,1.09980595760576));
#52791=CARTESIAN_POINT('Ctrl Pts',(71.3807680272526,8.44460390166829,1.12025083814614));
#52792=CARTESIAN_POINT('Ctrl Pts',(71.3034986191992,8.40086816269192,1.14165286565924));
#52793=CARTESIAN_POINT('Ctrl Pts',(71.2251186384731,8.35808201230144,1.16434513180719));
#52794=CARTESIAN_POINT('Ctrl Pts',(71.1467386577471,8.31529586191095,1.18703739795513));
#52795=CARTESIAN_POINT('Ctrl Pts',(71.0672485802617,8.27345962988279,1.21101900311761));
#52796=CARTESIAN_POINT('Ctrl Pts',(70.9866768879313,8.2327678316685,1.23665789244156));
#52797=CARTESIAN_POINT('Ctrl Pts',(70.9225854914917,8.20039921564761,1.25705255181145));
#52798=CARTESIAN_POINT('Ctrl Pts',(70.8577935182715,8.1687475991007,1.27851198822847));
#52799=CARTESIAN_POINT('Ctrl Pts',(70.7925061661959,8.1379986244689,1.30115319693028));
#52800=CARTESIAN_POINT('Ctrl Pts',(70.7267525239182,8.10703003692366,1.32395611189601));
#52801=CARTESIAN_POINT('Ctrl Pts',(70.6604961163344,8.07697706982272,1.3479577397916));
#52802=CARTESIAN_POINT('Ctrl Pts',(70.5939313780561,8.04798541106798,1.37330331984324));
#52803=CARTESIAN_POINT('Ctrl Pts',(70.5257910186144,8.01830750502556,1.3992488426478));
#52804=CARTESIAN_POINT('Ctrl Pts',(70.4573271547263,7.98974176606292,1.4266027777622));
#52805=CARTESIAN_POINT('Ctrl Pts',(70.3887376769203,7.96239790239819,1.45554731412904));
#52806=CARTESIAN_POINT('Ctrl Pts',(70.3778897660787,7.9580732770389,1.4601250971929));
#52807=CARTESIAN_POINT('Ctrl Pts',(70.3670386998171,7.95377912294994,1.46474271725));
#52808=CARTESIAN_POINT('Ctrl Pts',(70.3561852489274,7.94951577156251,1.46940094995523));
#52809=CARTESIAN_POINT('Ctrl Pts',(70.3065003382005,7.9299990081631,1.49072540044166));
#52810=CARTESIAN_POINT('Ctrl Pts',(70.2567653163896,7.91112852120851,1.51290089381212));
#52811=CARTESIAN_POINT('Ctrl Pts',(70.2070623135176,7.89291853271043,1.53600529080569));
#52812=CARTESIAN_POINT('Ctrl Pts',(70.159209965595,7.87538657981169,1.55824941248034));
#52813=CARTESIAN_POINT('Ctrl Pts',(70.1113957992755,7.85847545200609,1.5813364086832));
#52814=CARTESIAN_POINT('Ctrl Pts',(70.0640678103716,7.84231378742065,1.60505474719515));
#52815=CARTESIAN_POINT('Ctrl Pts',(70.0464012568961,7.83628097431651,1.61390830943973));
#52816=CARTESIAN_POINT('Ctrl Pts',(70.0288026585101,7.83035211896612,1.62284973799107));
#52817=CARTESIAN_POINT('Ctrl Pts',(70.0112961471453,7.82453231586902,1.63186758920309));
#52818=CARTESIAN_POINT('Ctrl Pts',(69.9525478479664,7.80500223780914,1.66212966769005));
#52819=CARTESIAN_POINT('Ctrl Pts',(69.8948362221269,7.78669457785894,1.69325323137175));
#52820=CARTESIAN_POINT('Ctrl Pts',(69.8377704723018,7.7693827643488,1.72543337981226));
#52821=CARTESIAN_POINT('Ctrl Pts',(69.8322750469301,7.76771563863002,1.72853232453389));
#52822=CARTESIAN_POINT('Ctrl Pts',(69.8267856033749,7.76605778674206,1.73164106526536));
#52823=CARTESIAN_POINT('Ctrl Pts',(69.8213017872758,7.76440903040879,1.73475977511561));
#52824=CARTESIAN_POINT('Ctrl Pts',(69.7467647250881,7.7419988235152,1.77714986731706));
#52825=CARTESIAN_POINT('Ctrl Pts',(69.6732726250391,7.72127062399585,1.82137723267184));
#52826=CARTESIAN_POINT('Ctrl Pts',(69.6008174128332,7.70204255404898,1.86742873080328));
#52827=CARTESIAN_POINT('Ctrl Pts',(69.5519019344798,7.68906142804534,1.89851871027355));
#52828=CARTESIAN_POINT('Ctrl Pts',(69.5034597369955,7.67676431036926,1.93043932883238));
#52829=CARTESIAN_POINT('Ctrl Pts',(69.4554974352252,7.66509865519602,1.96317722051819));
#52830=CARTESIAN_POINT('Ctrl Pts',(69.3814453687939,7.64708730378109,2.01372334613052));
#52831=CARTESIAN_POINT('Ctrl Pts',(69.3085341262881,7.63057938939238,2.06622116555943));
#52832=CARTESIAN_POINT('Ctrl Pts',(69.2367320173285,7.61537862467897,2.12062321961406));
#52833=CARTESIAN_POINT('Ctrl Pts',(69.1931442909367,7.60615094623228,2.15364818060257));
#52834=CARTESIAN_POINT('Ctrl Pts',(69.1499659753585,7.59740542792075,2.18737417453181));
#52835=CARTESIAN_POINT('Ctrl Pts',(69.1071959837192,7.58910201458796,2.22178463376911));
#52836=CARTESIAN_POINT('Ctrl Pts',(69.050583461092,7.57811119702716,2.26733205679904));
#52837=CARTESIAN_POINT('Ctrl Pts',(68.9946823019327,7.56789262939594,2.31408266864305));
#52838=CARTESIAN_POINT('Ctrl Pts',(68.9392638713717,7.5583260135376,2.36208160192688));
#52839=CARTESIAN_POINT('Ctrl Pts',(68.9115546560912,7.55354270560842,2.38608106856881));
#52840=CARTESIAN_POINT('Ctrl Pts',(68.883965998737,7.54892353081008,2.41039260184554));
#52841=CARTESIAN_POINT('Ctrl Pts',(68.8567731667949,7.54449996075162,2.43489503258616));
#52842=CARTESIAN_POINT('Ctrl Pts',(68.8295803348527,7.54007639069317,2.45939746332675));
#52843=CARTESIAN_POINT('Ctrl Pts',(68.8027835039613,7.53584644002574,2.48409084385879));
#52844=CARTESIAN_POINT('Ctrl Pts',(68.7758795221472,7.53172516776694,2.50914205840402));
#52845=CARTESIAN_POINT('Ctrl Pts',(68.7301518127084,7.52472039272396,2.55172068738643));
#52846=CARTESIAN_POINT('Ctrl Pts',(68.6840624656445,7.51802262568023,2.59538653605302));
#52847=CARTESIAN_POINT('Ctrl Pts',(68.6372644191002,7.51157227596553,2.64100742771448));
#52848=CARTESIAN_POINT('Ctrl Pts',(68.5897557349075,7.50502397640697,2.68732108169315));
#52849=CARTESIAN_POINT('Ctrl Pts',(68.5415167591615,7.49873099597664,2.73564949180677));
#52850=CARTESIAN_POINT('Ctrl Pts',(68.4921482382404,7.49265420489694,2.78693336440043));
#52851=CARTESIAN_POINT('Ctrl Pts',(68.4421098073691,7.48649495433225,2.83891313745651));
#52852=CARTESIAN_POINT('Ctrl Pts',(68.3909109596423,7.48055824363085,2.89392903813864));
#52853=CARTESIAN_POINT('Ctrl Pts',(68.3380983558102,7.47482122749588,2.95299557340639));
#52854=CARTESIAN_POINT('Ctrl Pts',(68.2828747081629,7.46882230044824,3.01475866203846));
#52855=CARTESIAN_POINT('Ctrl Pts',(68.2258865060699,7.46304247477419,3.08095050350886));
#52856=CARTESIAN_POINT('Ctrl Pts',(68.1665747574627,7.45746619752795,3.15277143207088));
#52857=CARTESIAN_POINT('Ctrl Pts',(68.1342306780551,7.45442532353104,3.19193705896753));
#52858=CARTESIAN_POINT('Ctrl Pts',(68.1011949235458,7.45144510807664,3.23277736689701));
#52859=CARTESIAN_POINT('Ctrl Pts',(68.067372593208,7.44852266268155,3.27549181431079));
#52860=CARTESIAN_POINT('Ctrl Pts',(68.0393618341962,7.44610237073628,3.31086678939027));
#52861=CARTESIAN_POINT('Ctrl Pts',(68.0108461331695,7.44372514058797,3.34750216611316));
#52862=CARTESIAN_POINT('Ctrl Pts',(67.9818717403097,7.44139632116286,3.38541042745233));
#52863=CARTESIAN_POINT('Ctrl Pts',(67.9352181391225,7.4376465337826,3.44644904575164));
#52864=CARTESIAN_POINT('Ctrl Pts',(67.8873742724675,7.43402312749421,3.51078829405039));
#52865=CARTESIAN_POINT('Ctrl Pts',(67.8385661574121,7.4305321130176,3.57847174093336));
#52866=CARTESIAN_POINT('Ctrl Pts',(67.7799537039465,7.42633984041443,3.65975111171679));
#52867=CARTESIAN_POINT('Ctrl Pts',(67.7199498519168,7.42233929637198,3.74585372531127));
#52868=CARTESIAN_POINT('Ctrl Pts',(67.658984107429,7.41850083566823,3.83683942029884));
#52869=CARTESIAN_POINT('Ctrl Pts',(67.5959003797892,7.41452902475006,3.93098600786092));
#52870=CARTESIAN_POINT('Ctrl Pts',(67.5317869521182,7.41073023073603,4.03036110899213));
#52871=CARTESIAN_POINT('Ctrl Pts',(67.4671609034974,7.40703976043349,4.13500568014468));
#52872=CARTESIAN_POINT('Ctrl Pts',(67.3976824709064,7.40307219475965,4.24750738708804));
#52873=CARTESIAN_POINT('Ctrl Pts',(67.327611744913,7.39922890666538,4.3660999664496));
#52874=CARTESIAN_POINT('Ctrl Pts',(67.2576354760908,7.39540446226772,4.49079996308749));
#52875=CARTESIAN_POINT('Ctrl Pts',(67.2253998664584,7.39364267503987,4.5482448723464));
#52876=CARTESIAN_POINT('Ctrl Pts',(67.1931848694007,7.3918846469134,4.60698535420133));
#52877=CARTESIAN_POINT('Ctrl Pts',(67.1610601855551,7.39011941651789,4.66702057018075));
#52878=CARTESIAN_POINT('Ctrl Pts',(67.1027034504911,7.38691275204104,4.77607873897899));
#52879=CARTESIAN_POINT('Ctrl Pts',(67.0445967951296,7.38367598971354,4.88940658137533));
#52880=CARTESIAN_POINT('Ctrl Pts',(66.987257923219,7.3803305620751,5.00568290057736));
#52881=CARTESIAN_POINT('Ctrl Pts',(66.9741040662662,7.37956310231986,5.03235733658942));
#52882=CARTESIAN_POINT('Ctrl Pts',(66.9609906888157,7.37879001909429,5.05918675937889));
#52883=CARTESIAN_POINT('Ctrl Pts',(66.9479241477424,7.37801056057405,5.08615491125607));
#52884=CARTESIAN_POINT('Ctrl Pts',(66.8875144375256,7.37440693945733,5.21083505658684));
#52885=CARTESIAN_POINT('Ctrl Pts',(66.8281056642597,7.37066314832943,5.33848162552259));
#52886=CARTESIAN_POINT('Ctrl Pts',(66.7703316269961,7.36673766393218,5.46737610691827));
#52887=CARTESIAN_POINT('Ctrl Pts',(66.7485076159051,7.36525482113496,5.51606570392032));
#52888=CARTESIAN_POINT('Ctrl Pts',(66.7269168694435,7.36374656641509,5.56493325569604));
#52889=CARTESIAN_POINT('Ctrl Pts',(66.7055933079143,7.36221263535037,5.61388618348348));
#52890=CARTESIAN_POINT('Ctrl Pts',(66.6705404894961,7.35969107688538,5.69435764161353));
#52891=CARTESIAN_POINT('Ctrl Pts',(66.6362070137045,7.35709334765865,5.77457740473056));
#52892=CARTESIAN_POINT('Ctrl Pts',(66.6024276407753,7.35440345015614,5.85511097730033));
#52893=CARTESIAN_POINT('Ctrl Pts',(66.5697369835203,7.35180024856651,5.93304893736597));
#52894=CARTESIAN_POINT('Ctrl Pts',(66.5375651271738,7.34911077725039,6.01128296840618));
#52895=CARTESIAN_POINT('Ctrl Pts',(66.5057598873521,7.346313564451,6.09054288218826));
#52896=CARTESIAN_POINT('Ctrl Pts',(66.4858044278963,7.34455851820955,6.14027267529217));
#52897=CARTESIAN_POINT('Ctrl Pts',(66.465993265484,7.34276095254317,6.19040585962652));
#52898=CARTESIAN_POINT('Ctrl Pts',(66.4462888775018,7.34091441397408,6.24112139183781));
#52899=CARTESIAN_POINT('Ctrl Pts',(66.4177191712417,7.33823708826549,6.31465465049112));
#52900=CARTESIAN_POINT('Ctrl Pts',(66.3893738107666,7.33545693498657,6.38941296128914));
#52901=CARTESIAN_POINT('Ctrl Pts',(66.3611415770503,7.33254927110616,6.46471849632842));
#52902=CARTESIAN_POINT('Ctrl Pts',(66.3411307769353,7.3304883402816,6.51809450703888));
#52903=CARTESIAN_POINT('Ctrl Pts',(66.3211768417519,7.32836327159669,6.57174617528332));
#52904=CARTESIAN_POINT('Ctrl Pts',(66.3012408988535,7.32616401149819,6.62541455568106));
#52905=CARTESIAN_POINT('Ctrl Pts',(66.3010470943458,7.32614263169574,6.62593628540793));
#52906=CARTESIAN_POINT('Ctrl Pts',(66.3008532829922,7.32612125012428,6.62645809298242));
#52907=CARTESIAN_POINT('Ctrl Pts',(66.300659464751,7.32609986677702,6.62697997853453));
#52908=CARTESIAN_POINT('',(77.889681615155,13.4545721695848,-1.3438880610302));
#52909=CARTESIAN_POINT('Ctrl Pts',(77.8897369876382,13.454578052485,-1.34376136630412));
#52910=CARTESIAN_POINT('Ctrl Pts',(77.7696649432831,13.3860274200672,-1.26444509700194));
#52911=CARTESIAN_POINT('Ctrl Pts',(77.6507591912599,13.3147757364772,-1.18781988562592));
#52912=CARTESIAN_POINT('Ctrl Pts',(77.5329174622466,13.2411051793034,-1.11382860288741));
#52913=CARTESIAN_POINT('Ctrl Pts',(77.4085913534954,13.1633808130739,-1.03576586279179));
#52914=CARTESIAN_POINT('Ctrl Pts',(77.2854492624687,13.0829643495867,-0.960634817073859));
#52915=CARTESIAN_POINT('Ctrl Pts',(77.1633377242301,13.0001610172308,-0.888327978216956));
#52916=CARTESIAN_POINT('Ctrl Pts',(77.0305214521826,12.9100988488619,-0.809682463476546));
#52917=CARTESIAN_POINT('Ctrl Pts',(76.8989239464047,12.8172131254906,-0.734377989221384));
#52918=CARTESIAN_POINT('Ctrl Pts',(76.7683148872926,12.7218623074812,-0.662230278878765));
#52919=CARTESIAN_POINT('Ctrl Pts',(76.6491405067779,12.6348593480762,-0.59639902074026));
#52920=CARTESIAN_POINT('Ctrl Pts',(76.5307882492475,12.545803177586,-0.533195049924176));
#52921=CARTESIAN_POINT('Ctrl Pts',(76.4130672370339,12.4549458820906,-0.472450897944697));
#52922=CARTESIAN_POINT('Ctrl Pts',(76.2762974708588,12.3493867229691,-0.401877571173899));
#52923=CARTESIAN_POINT('Ctrl Pts',(76.1403792450269,12.2413957409076,-0.334625199413047));
#52924=CARTESIAN_POINT('Ctrl Pts',(76.004996467159,12.1313534640472,-0.270409688323707));
#52925=CARTESIAN_POINT('Ctrl Pts',(75.8959215084883,12.0426947957172,-0.218672648144735));
#52926=CARTESIAN_POINT('Ctrl Pts',(75.7872165562079,11.9527241237791,-0.168939362331957));
#52927=CARTESIAN_POINT('Ctrl Pts',(75.6791301262885,11.8620082672792,-0.121234670160239));
#52928=CARTESIAN_POINT('Ctrl Pts',(75.5617280619492,11.7634738922486,-0.0694184584137104));
#52929=CARTESIAN_POINT('Ctrl Pts',(75.4450556136026,11.6640617599789,-0.019995805029085));
#52930=CARTESIAN_POINT('Ctrl Pts',(75.3293856079521,11.5645181097544,0.0270406542219756));
#52931=CARTESIAN_POINT('Ctrl Pts',(75.2545888435804,11.5001492795753,0.0574562744140373));
#52932=CARTESIAN_POINT('Ctrl Pts',(75.1802103035331,11.4357258127535,0.0868749546023082));
#52933=CARTESIAN_POINT('Ctrl Pts',(75.1063155860452,11.3714486085643,0.115306615285322));
#52934=CARTESIAN_POINT('Ctrl Pts',(75.0634481505555,11.334160436991,0.131800248682));
#52935=CARTESIAN_POINT('Ctrl Pts',(75.0207456102727,11.2969243424609,0.147958040871395));
#52936=CARTESIAN_POINT('Ctrl Pts',(74.9781991372383,11.2597586237108,0.163796713837524));
#52937=CARTESIAN_POINT('Ctrl Pts',(74.8570163150392,11.1539015134508,0.208909150968764));
#52938=CARTESIAN_POINT('Ctrl Pts',(74.7370964572705,11.0486184760316,0.251433430739692));
#52939=CARTESIAN_POINT('Ctrl Pts',(74.6182988652355,10.9443033407062,0.29167327561244));
#52940=CARTESIAN_POINT('Ctrl Pts',(74.53257013101,10.8690256826425,0.320711835294296));
#52941=CARTESIAN_POINT('Ctrl Pts',(74.447426725528,10.7942510487121,0.348560587500119));
#52942=CARTESIAN_POINT('Ctrl Pts',(74.362827427958,10.7201158474377,0.375331231937685));
#52943=CARTESIAN_POINT('Ctrl Pts',(74.3241300435651,10.6862049467191,0.387576651793423));
#52944=CARTESIAN_POINT('Ctrl Pts',(74.2855466310907,10.652427718942,0.399596480972964));
#52945=CARTESIAN_POINT('Ctrl Pts',(74.2470739624078,10.6187965603701,0.411402002610675));
#52946=CARTESIAN_POINT('Ctrl Pts',(74.1152717740108,10.503580734438,0.451846131918322));
#52947=CARTESIAN_POINT('Ctrl Pts',(73.9847620349683,10.390081163806,0.489768074617004));
#52948=CARTESIAN_POINT('Ctrl Pts',(73.855569922101,10.2788762885707,0.525598948152581));
#52949=CARTESIAN_POINT('Ctrl Pts',(73.7181119302229,10.160556381127,0.563722327468323));
#52950=CARTESIAN_POINT('Ctrl Pts',(73.5821457405882,10.0448340625995,0.599478074205453));
#52951=CARTESIAN_POINT('Ctrl Pts',(73.4477337028793,9.93236292982832,0.633364489974651));
#52952=CARTESIAN_POINT('Ctrl Pts',(73.4400508513117,9.925934197451,0.635301402076798));
#52953=CARTESIAN_POINT('Ctrl Pts',(73.4323730851476,9.91951607647723,0.637232202501358));
#52954=CARTESIAN_POINT('Ctrl Pts',(73.4247004187787,9.91310868515717,0.639156982847771));
#52955=CARTESIAN_POINT('Ctrl Pts',(73.3484071455047,9.84939669333381,0.658296065130513));
#52956=CARTESIAN_POINT('Ctrl Pts',(73.2726503620905,9.78677844675524,0.676809304159524));
#52957=CARTESIAN_POINT('Ctrl Pts',(73.1970992174034,9.72507933887715,0.694899701214236));
#52958=CARTESIAN_POINT('Ctrl Pts',(73.1320183483839,9.67193081842693,0.710483035736911));
#52959=CARTESIAN_POINT('Ctrl Pts',(73.0670904212155,9.61946453509583,0.725752353116069));
#52960=CARTESIAN_POINT('Ctrl Pts',(73.0021168694563,9.56759598842738,0.740829004151231));
#52961=CARTESIAN_POINT('Ctrl Pts',(72.932838096084,9.51229057272347,0.756904651272255));
#52962=CARTESIAN_POINT('Ctrl Pts',(72.8635071947699,9.45766382673869,0.772761034710399));
#52963=CARTESIAN_POINT('Ctrl Pts',(72.7938955857395,9.40365790551125,0.788511490263578));
#52964=CARTESIAN_POINT('Ctrl Pts',(72.7382855472508,9.36051465110428,0.801093923735916));
#52965=CARTESIAN_POINT('Ctrl Pts',(72.6824966686878,9.31776823977093,0.813608634719925));
#52966=CARTESIAN_POINT('Ctrl Pts',(72.6264202454239,9.27541176713065,0.826110541299093));
#52967=CARTESIAN_POINT('Ctrl Pts',(72.5945374139565,9.25132955574594,0.833218629819788));
#52968=CARTESIAN_POINT('Ctrl Pts',(72.5625640095599,9.22737353904165,0.840326021588078));
#52969=CARTESIAN_POINT('Ctrl Pts',(72.5303081355092,9.20341764626573,0.847487344676562));
#52970=CARTESIAN_POINT('Ctrl Pts',(72.487572237045,9.1716784163914,0.856975401825411));
#52971=CARTESIAN_POINT('Ctrl Pts',(72.4443402247944,9.13993774890631,0.866558533369955));
#52972=CARTESIAN_POINT('Ctrl Pts',(72.4001654819828,9.10791760692907,0.876355253944482));
#52973=CARTESIAN_POINT('Ctrl Pts',(72.3718124277847,9.08736584447092,0.882643167166719));
#52974=CARTESIAN_POINT('Ctrl Pts',(72.3430712691142,9.06669988959138,0.889018841982827));
#52975=CARTESIAN_POINT('Ctrl Pts',(72.313826406605,9.04585705470419,0.895511213136602));
#52976=CARTESIAN_POINT('Ctrl Pts',(72.2782005556,9.02046648465175,0.903420166284219));
#52977=CARTESIAN_POINT('Ctrl Pts',(72.2418271176384,8.99481287323038,0.911501910042503));
#52978=CARTESIAN_POINT('Ctrl Pts',(72.2045037278336,8.9687958769127,0.919834021587207));
#52979=CARTESIAN_POINT('Ctrl Pts',(72.1538128961915,8.93346084472328,0.931150294459102));
#52980=CARTESIAN_POINT('Ctrl Pts',(72.1013168125388,8.89743020840457,0.942915182554698));
#52981=CARTESIAN_POINT('Ctrl Pts',(72.0474557803843,8.86112788084346,0.955113998180602));
#52982=CARTESIAN_POINT('Ctrl Pts',(71.9937786728343,8.82494951843807,0.967271157301807));
#52983=CARTESIAN_POINT('Ctrl Pts',(71.9387461380037,8.78850141025257,0.979861167387469));
#52984=CARTESIAN_POINT('Ctrl Pts',(71.8827684068436,8.75215890578048,0.992874181303956));
#52985=CARTESIAN_POINT('Ctrl Pts',(71.8301767728057,8.71801476210752,1.00510003704056));
#52986=CARTESIAN_POINT('Ctrl Pts',(71.7767506298625,8.68396339190662,1.01770080297037));
#52987=CARTESIAN_POINT('Ctrl Pts',(71.7228079848105,8.65028033847831,1.03064780199761));
#52988=CARTESIAN_POINT('Ctrl Pts',(71.7193349032355,8.648111664841,1.03148139077935));
#52989=CARTESIAN_POINT('Ctrl Pts',(71.7158596731749,8.64594450634418,1.03231640289029));
#52990=CARTESIAN_POINT('Ctrl Pts',(71.7123823764776,8.64377893173703,1.03315282533716));
#52991=CARTESIAN_POINT('',(76.015201080752,13.203464720596,-5.13235367185313));
#52992=CARTESIAN_POINT('Ctrl Pts',(76.0153669751839,13.2030576234056,-5.13241323346553));
#52993=CARTESIAN_POINT('Ctrl Pts',(76.421418629627,13.284909104379,-4.56170310137939));
#52994=CARTESIAN_POINT('Ctrl Pts',(76.7911800730128,13.3487897444448,-3.96280879484323));
#52995=CARTESIAN_POINT('Ctrl Pts',(77.4282530545409,13.4417516204142,-2.69007218753358));
#52996=CARTESIAN_POINT('Ctrl Pts',(77.6871091804814,13.4682801109617,-2.03089402659865));
#52997=CARTESIAN_POINT('Ctrl Pts',(77.8897919794669,13.4547521623004,-1.34470326831834));
#52998=CARTESIAN_POINT('',(69.6237422477963,12.3291004120382,-10.9554808154403));
#52999=CARTESIAN_POINT('Ctrl Pts',(69.6237422477963,12.3291004120382,-10.9554808154403));
#53000=CARTESIAN_POINT('Ctrl Pts',(70.0827581319187,12.3750434414314,-10.6014370912123));
#53001=CARTESIAN_POINT('Ctrl Pts',(70.9196713183267,12.4282942768532,-9.96905190676241));
#53002=CARTESIAN_POINT('Ctrl Pts',(71.9983599818921,12.4985273335172,-9.148643524566));
#53003=CARTESIAN_POINT('Ctrl Pts',(72.8711908196415,12.5908103550809,-8.44939111030075));
#53004=CARTESIAN_POINT('Ctrl Pts',(73.8194076466462,12.7307073058631,-7.63287520525915));
#53005=CARTESIAN_POINT('Ctrl Pts',(74.8903772207131,12.9478927784384,-6.5947327339628));
#53006=CARTESIAN_POINT('Ctrl Pts',(75.636641075592,13.1281023785155,-5.67240251279549));
#53007=CARTESIAN_POINT('Ctrl Pts',(76.015201080752,13.203464720596,-5.13235367185313));
#53008=CARTESIAN_POINT('',(56.9472987453407,10.4971210955841,-16.8490842893539));
#53009=CARTESIAN_POINT('Ctrl Pts',(56.9472987452418,10.4971210960185,-16.8490842892186));
#53010=CARTESIAN_POINT('Ctrl Pts',(57.5279764227459,10.5627663098217,-16.6356348664524));
#53011=CARTESIAN_POINT('Ctrl Pts',(59.2489796005507,10.727653207555,-16.0034819097119));
#53012=CARTESIAN_POINT('Ctrl Pts',(61.3469127090617,10.8548490654473,-15.2216988808759));
#53013=CARTESIAN_POINT('Ctrl Pts',(63.6263802921922,11.1482588003824,-14.3361986078586));
#53014=CARTESIAN_POINT('Ctrl Pts',(65.6200127215301,11.5559853879963,-13.4649812857152));
#53015=CARTESIAN_POINT('Ctrl Pts',(67.2665644790765,11.9454658004384,-12.5548298006343));
#53016=CARTESIAN_POINT('Ctrl Pts',(68.6272491818126,12.2018297485735,-11.6733467842871));
#53017=CARTESIAN_POINT('Ctrl Pts',(69.3091557765954,12.295115398284,-11.1879566051838));
#53018=CARTESIAN_POINT('Ctrl Pts',(69.6237422477963,12.3291004120382,-10.9554808154403));
#53019=CARTESIAN_POINT('',(43.6350103091031,8.95468725191293,-22.9398456748034));
#53020=CARTESIAN_POINT('Ctrl Pts',(43.6350103091031,8.95468725191292,-22.9398456748034));
#53021=CARTESIAN_POINT('Ctrl Pts',(43.9816241860284,8.96228593705789,-22.557621122663));
#53022=CARTESIAN_POINT('Ctrl Pts',(45.0665104587698,8.90088112468958,-21.464400433797));
#53023=CARTESIAN_POINT('Ctrl Pts',(46.5058625028201,8.76988624042247,-20.3242063737796));
#53024=CARTESIAN_POINT('Ctrl Pts',(48.0929903702374,8.97675586023584,-19.5751405126828));
#53025=CARTESIAN_POINT('Ctrl Pts',(48.9363712410941,9.12178060695302,-19.2461729821237));
#53026=CARTESIAN_POINT('Ctrl Pts',(49.8971073949701,9.31033141838707,-18.924603413807));
#53027=CARTESIAN_POINT('Ctrl Pts',(51.3205749059214,9.59771447476012,-18.4933476791936));
#53028=CARTESIAN_POINT('Ctrl Pts',(53.704075386902,10.0351563165077,-17.8376971923096));
#53029=CARTESIAN_POINT('Ctrl Pts',(55.8717928719535,10.3637905543193,-17.2067231078532));
#53030=CARTESIAN_POINT('Ctrl Pts',(56.9472987452418,10.4971210960185,-16.8490842892186));
#53031=CARTESIAN_POINT('',(39.8379457614118,8.40789306792086,-29.2047706348498));
#53032=CARTESIAN_POINT('Ctrl Pts',(39.8379458507108,8.40789307202619,-29.2047705582436));
#53033=CARTESIAN_POINT('Ctrl Pts',(39.8654457076855,8.40364510819277,-29.0955685679339));
#53034=CARTESIAN_POINT('Ctrl Pts',(39.8944208207261,8.39988236979115,-28.9853680288274));
#53035=CARTESIAN_POINT('Ctrl Pts',(39.9245087456163,8.39664864008142,-28.8750526458601));
#53036=CARTESIAN_POINT('Ctrl Pts',(39.9491018028661,8.39400547674688,-28.7848838310032));
#53037=CARTESIAN_POINT('Ctrl Pts',(39.974439446193,8.39171630686269,-28.6946375080915));
#53038=CARTESIAN_POINT('Ctrl Pts',(40.0003463528771,8.38980515356937,-28.6047839467515));
#53039=CARTESIAN_POINT('Ctrl Pts',(40.036943271421,8.38710539777634,-28.4778539544787));
#53040=CARTESIAN_POINT('Ctrl Pts',(40.0746628015218,8.38514479988263,-28.351668786224));
#53041=CARTESIAN_POINT('Ctrl Pts',(40.1151217116781,8.38440583150625,-28.2241319360277));
#53042=CARTESIAN_POINT('Ctrl Pts',(40.1509951639247,8.38375061497522,-28.111049623936));
#53043=CARTESIAN_POINT('Ctrl Pts',(40.1890192933759,8.38405564745187,-27.9969067272385));
#53044=CARTESIAN_POINT('Ctrl Pts',(40.230302310591,8.3856577702999,-27.8802179261844));
#53045=CARTESIAN_POINT('Ctrl Pts',(40.2509085167103,8.38645746169511,-27.8219733101525));
#53046=CARTESIAN_POINT('Ctrl Pts',(40.2723265910565,8.38758035193068,-27.7630938340167));
#53047=CARTESIAN_POINT('Ctrl Pts',(40.294695712765,8.38906805768105,-27.703389664616));
#53048=CARTESIAN_POINT('Ctrl Pts',(40.3301636319506,8.39142692666185,-27.6087242288008));
#53049=CARTESIAN_POINT('Ctrl Pts',(40.3680208790409,8.39470347103164,-27.5119877200577));
#53050=CARTESIAN_POINT('Ctrl Pts',(40.4088318964747,8.39906594238233,-27.4123919238348));
#53051=CARTESIAN_POINT('Ctrl Pts',(40.4156338083733,8.39979302902838,-27.3957924398233));
#53052=CARTESIAN_POINT('Ctrl Pts',(40.4225178367521,8.40055025887844,-27.3791134347866));
#53053=CARTESIAN_POINT('Ctrl Pts',(40.4294866832965,8.40133837812109,-27.3623511375053));
#53054=CARTESIAN_POINT('Ctrl Pts',(40.4660898787361,8.40547789855459,-27.2743087850876));
#53055=CARTESIAN_POINT('Ctrl Pts',(40.5050731911368,8.41048451571273,-27.1839285580151));
#53056=CARTESIAN_POINT('Ctrl Pts',(40.5468152791266,8.41653147821018,-27.0912433138878));
#53057=CARTESIAN_POINT('Ctrl Pts',(40.5863426940439,8.42225761236248,-27.0034755888465));
#53058=CARTESIAN_POINT('Ctrl Pts',(40.6283436920716,8.42891728279138,-26.9136409650853));
#53059=CARTESIAN_POINT('Ctrl Pts',(40.6731712777039,8.43663873332445,-26.8217452228992));
#53060=CARTESIAN_POINT('Ctrl Pts',(40.7158607183075,8.44399189319812,-26.7342326394656));
#53061=CARTESIAN_POINT('Ctrl Pts',(40.7611133986222,8.4523085787623,-26.6448508348228));
#53062=CARTESIAN_POINT('Ctrl Pts',(40.8092660707817,8.4616729323727,-26.5535842941883));
#53063=CARTESIAN_POINT('Ctrl Pts',(40.8546173937697,8.47049250159107,-26.4676273124322));
#53064=CARTESIAN_POINT('Ctrl Pts',(40.9025411427559,8.48024183005811,-26.3799983939024));
#53065=CARTESIAN_POINT('Ctrl Pts',(40.9533481888092,8.49095967199949,-26.2906670701268));
#53066=CARTESIAN_POINT('Ctrl Pts',(40.9708435866532,8.49465035908641,-26.2599058436672));
#53067=CARTESIAN_POINT('Ctrl Pts',(40.9886811427199,8.49845557165255,-26.2289425997796));
#53068=CARTESIAN_POINT('Ctrl Pts',(41.006874407862,8.50237580188874,-26.1977756141706));
#53069=CARTESIAN_POINT('Ctrl Pts',(41.0543714794208,8.51261032848971,-26.1164081117363));
#53070=CARTESIAN_POINT('Ctrl Pts',(41.1042913860663,8.5236312272845,-26.0336524923972));
#53071=CARTESIAN_POINT('Ctrl Pts',(41.156883062279,8.53543041516824,-25.9494837002749));
#53072=CARTESIAN_POINT('Ctrl Pts',(41.182392510285,8.54115357882281,-25.9086578589823));
#53073=CARTESIAN_POINT('Ctrl Pts',(41.2085309627192,8.5470592965295,-25.8674994260819));
#53074=CARTESIAN_POINT('Ctrl Pts',(41.2353251982349,8.5531467156204,-25.8260048651385));
#53075=CARTESIAN_POINT('Ctrl Pts',(41.29696834527,8.56715150668316,-25.7305419690284));
#53076=CARTESIAN_POINT('Ctrl Pts',(41.3620507458278,8.58211304497296,-25.6333500282192));
#53077=CARTESIAN_POINT('Ctrl Pts',(41.4303930158195,8.59780001240496,-25.5346447309645));
#53078=CARTESIAN_POINT('Ctrl Pts',(41.4648092332714,8.60569975121032,-25.4849381149217));
#53079=CARTESIAN_POINT('Ctrl Pts',(41.5000518250078,8.61378278089177,-25.4348478483315));
#53080=CARTESIAN_POINT('Ctrl Pts',(41.5360953172835,8.62201528938143,-25.384402666044));
#53081=CARTESIAN_POINT('Ctrl Pts',(41.559761387381,8.62742073460035,-25.3512804810191));
#53082=CARTESIAN_POINT('Ctrl Pts',(41.5837751341606,8.63289296667882,-25.3179985849375));
#53083=CARTESIAN_POINT('Ctrl Pts',(41.6093083635431,8.63869517343395,-25.2830281569375));
#53084=CARTESIAN_POINT('Ctrl Pts',(41.6273155224164,8.64278714540074,-25.2583654696045));
#53085=CARTESIAN_POINT('Ctrl Pts',(41.646078875468,8.64704290198039,-25.2328624102245));
#53086=CARTESIAN_POINT('Ctrl Pts',(41.6660177860212,8.65154646109351,-25.2059722122501));
#53087=CARTESIAN_POINT('Ctrl Pts',(41.7061938401206,8.66062094056852,-25.1517896105636));
#53088=CARTESIAN_POINT('Ctrl Pts',(41.7511315850727,8.67069915813332,-25.0919867008814));
#53089=CARTESIAN_POINT('Ctrl Pts',(41.8008463390065,8.68169374062394,-25.0271020172724));
#53090=CARTESIAN_POINT('Ctrl Pts',(41.8505610929402,8.69268832311456,-24.9622173336634));
#53091=CARTESIAN_POINT('Ctrl Pts',(41.9050537586142,8.704600084385,-24.8922502534608));
#53092=CARTESIAN_POINT('Ctrl Pts',(41.9643405116155,8.7172845050543,-24.8177290368986));
#53093=CARTESIAN_POINT('Ctrl Pts',(42.0110422922183,8.72727636666222,-24.7590266568565));
#53094=CARTESIAN_POINT('Ctrl Pts',(42.0606925307826,8.73773282487033,-24.6974848315058));
#53095=CARTESIAN_POINT('Ctrl Pts',(42.1132268093581,8.74852068902431,-24.6333316508617));
#53096=CARTESIAN_POINT('Ctrl Pts',(42.1717469346412,8.76053774110816,-24.5618687456805));
#53097=CARTESIAN_POINT('Ctrl Pts',(42.2338464229499,8.7729672300637,-24.4871659557205));
#53098=CARTESIAN_POINT('Ctrl Pts',(42.2994250245914,8.78556845114903,-24.4094937624744));
#53099=CARTESIAN_POINT('Ctrl Pts',(42.3634124541936,8.79786392142312,-24.3337061751673));
#53100=CARTESIAN_POINT('Ctrl Pts',(42.4307126950835,8.81032240727235,-24.2550903585965));
#53101=CARTESIAN_POINT('Ctrl Pts',(42.501209777579,8.8226782550421,-24.1739053400292));
#53102=CARTESIAN_POINT('Ctrl Pts',(42.5570843250992,8.83247124758767,-24.1095597527043));
#53103=CARTESIAN_POINT('Ctrl Pts',(42.6149667148955,8.84219877627966,-24.0436001241147));
#53104=CARTESIAN_POINT('Ctrl Pts',(42.6747857552258,8.85171312383745,-23.9761668200724));
#53105=CARTESIAN_POINT('Ctrl Pts',(42.7238451349108,8.85951612413157,-23.9208627555447));
#53106=CARTESIAN_POINT('Ctrl Pts',(42.7742443970811,8.8670794989284,-23.8640393593037));
#53107=CARTESIAN_POINT('Ctrl Pts',(42.8258983427455,8.8743404967404,-23.806024202641));
#53108=CARTESIAN_POINT('Ctrl Pts',(42.8935600993232,8.8838517133599,-23.7300298646009));
#53109=CARTESIAN_POINT('Ctrl Pts',(42.9633750842634,8.89284222249282,-23.6519886341592));
#53110=CARTESIAN_POINT('Ctrl Pts',(43.0350811932542,8.90130616648017,-23.5731341011721));
#53111=CARTESIAN_POINT('Ctrl Pts',(43.0937059954034,8.90822603772467,-23.5086649581661));
#53112=CARTESIAN_POINT('Ctrl Pts',(43.1535941612811,8.91479461164248,-23.4436558523941));
#53113=CARTESIAN_POINT('Ctrl Pts',(43.2145942946101,8.92102322071077,-23.3787767103528));
#53114=CARTESIAN_POINT('Ctrl Pts',(43.2511690823933,8.92475780361125,-23.3398761256784));
#53115=CARTESIAN_POINT('Ctrl Pts',(43.288144220567,8.92836938755794,-23.3010181242117));
#53116=CARTESIAN_POINT('Ctrl Pts',(43.3255173890699,8.93177350374001,-23.2619819456453));
#53117=CARTESIAN_POINT('Ctrl Pts',(43.3607688402983,8.93498436437547,-23.2251618953257));
#53118=CARTESIAN_POINT('Ctrl Pts',(43.3963743880188,8.93801049201531,-23.1881827163246));
#53119=CARTESIAN_POINT('Ctrl Pts',(43.4323243751605,8.94079491063417,-23.1508996625381));
#53120=CARTESIAN_POINT('Ctrl Pts',(43.4663601170789,8.94343106605561,-23.1156018363774));
#53121=CARTESIAN_POINT('Ctrl Pts',(43.5007045420071,8.94585052166189,-23.0800314125403));
#53122=CARTESIAN_POINT('Ctrl Pts',(43.5353428904246,8.94801909874426,-23.0441085446635));
#53123=CARTESIAN_POINT('Ctrl Pts',(43.56843184955,8.95009067437406,-23.0097925232266));
#53124=CARTESIAN_POINT('Ctrl Pts',(43.6017889679761,8.95193331677229,-22.9751548483822));
#53125=CARTESIAN_POINT('Ctrl Pts',(43.6353959980847,8.95353081601041,-22.9401679958081));
#53126=CARTESIAN_POINT('',(38.9090196509257,8.64412049687874,-35.3258758917141));
#53127=CARTESIAN_POINT('Ctrl Pts',(38.9087434864013,8.64500019882641,-35.3257985374456));
#53128=CARTESIAN_POINT('Ctrl Pts',(38.9479517964268,8.6357301980531,-35.0802394942275));
#53129=CARTESIAN_POINT('Ctrl Pts',(38.9841706465803,8.62691819966679,-34.8358387398463));
#53130=CARTESIAN_POINT('Ctrl Pts',(39.0183707678307,8.61831927471614,-34.592222979301));
#53131=CARTESIAN_POINT('Ctrl Pts',(39.0533216837988,8.60953157770287,-34.3432591258404));
#53132=CARTESIAN_POINT('Ctrl Pts',(39.0861634603905,8.60096397289051,-34.0951162517341));
#53133=CARTESIAN_POINT('Ctrl Pts',(39.1178679600129,8.59241082953619,-33.847691734173));
#53134=CARTESIAN_POINT('Ctrl Pts',(39.1483258371988,8.58419399618631,-33.6099959604378));
#53135=CARTESIAN_POINT('Ctrl Pts',(39.177733914408,8.57599040915156,-33.3729645385711));
#53136=CARTESIAN_POINT('Ctrl Pts',(39.2069267841172,8.56763119233727,-33.1364750675382));
#53137=CARTESIAN_POINT('Ctrl Pts',(39.2209380749374,8.5636191366887,-33.0229705444275));
#53138=CARTESIAN_POINT('Ctrl Pts',(39.2348992662765,8.55957176304503,-32.9095908069147));
#53139=CARTESIAN_POINT('Ctrl Pts',(39.2488997523204,8.55547356312888,-32.7963217176363));
#53140=CARTESIAN_POINT('Ctrl Pts',(39.26811319789,8.54984943402538,-32.6408778655624));
#53141=CARTESIAN_POINT('Ctrl Pts',(39.287411692567,8.54413100777768,-32.4856347486376));
#53142=CARTESIAN_POINT('Ctrl Pts',(39.3068613012534,8.53834397345013,-32.3318970469014));
#53143=CARTESIAN_POINT('Ctrl Pts',(39.3222504300968,8.53376509382722,-32.2102550468871));
#53144=CARTESIAN_POINT('Ctrl Pts',(39.3377340677726,8.52914351924649,-32.0895562304329));
#53145=CARTESIAN_POINT('Ctrl Pts',(39.3533417882143,8.52450910313885,-31.9704683767878));
#53146=CARTESIAN_POINT('Ctrl Pts',(39.3684284241685,8.52002941317148,-31.8553564293885));
#53147=CARTESIAN_POINT('Ctrl Pts',(39.3836241066648,8.51553644644276,-31.7417266115632));
#53148=CARTESIAN_POINT('Ctrl Pts',(39.3993540901875,8.51096525102908,-31.6274715263285));
#53149=CARTESIAN_POINT('Ctrl Pts',(39.4141691946333,8.50665992309289,-31.5198616856205));
#53150=CARTESIAN_POINT('Ctrl Pts',(39.4294581565008,8.50228588894945,-31.4116967681536));
#53151=CARTESIAN_POINT('Ctrl Pts',(39.4455740757653,8.49775799379722,-31.3011828176225));
#53152=CARTESIAN_POINT('Ctrl Pts',(39.4524220787895,8.49583399311276,-31.254223047284));
#53153=CARTESIAN_POINT('Ctrl Pts',(39.4594193759509,8.49388175815388,-31.2068387470179));
#53154=CARTESIAN_POINT('Ctrl Pts',(39.4665929841818,8.49189240305858,-31.1588905269845));
#53155=CARTESIAN_POINT('Ctrl Pts',(39.4847506007671,8.48685700860855,-31.0375254667118));
#53156=CARTESIAN_POINT('Ctrl Pts',(39.5040385640118,8.48158512359671,-30.912541647874));
#53157=CARTESIAN_POINT('Ctrl Pts',(39.524965953692,8.47609349451604,-30.7832819655347));
#53158=CARTESIAN_POINT('Ctrl Pts',(39.5439349368359,8.47111577770303,-30.6661185365096));
#53159=CARTESIAN_POINT('Ctrl Pts',(39.5642507061145,8.46595797996059,-30.5454436942775));
#53160=CARTESIAN_POINT('Ctrl Pts',(39.5862904148607,8.46059797969943,-30.4207161971419));
#53161=CARTESIAN_POINT('Ctrl Pts',(39.5961523203423,8.45819958974947,-30.3649055327691));
#53162=CARTESIAN_POINT('Ctrl Pts',(39.6063593530292,8.45576024361895,-30.3082830308203));
#53163=CARTESIAN_POINT('Ctrl Pts',(39.6169450976819,8.45327533083215,-30.2507978882589));
#53164=CARTESIAN_POINT('Ctrl Pts',(39.632271772875,8.44967752525343,-30.1675674555055));
#53165=CARTESIAN_POINT('Ctrl Pts',(39.6483434234174,8.44608466718477,-30.0835384063042));
#53166=CARTESIAN_POINT('Ctrl Pts',(39.6652506185106,8.44244734684986,-29.9982286935872));
#53167=CARTESIAN_POINT('Ctrl Pts',(39.682240834708,8.43879216581432,-29.9125000759897));
#53168=CARTESIAN_POINT('Ctrl Pts',(39.7000749896951,8.43509186361522,-29.8254738199901));
#53169=CARTESIAN_POINT('Ctrl Pts',(39.7188369052445,8.43129884492167,-29.7368106658926));
#53170=CARTESIAN_POINT('Ctrl Pts',(39.7281696213245,8.42941208839834,-29.6927070645427));
#53171=CARTESIAN_POINT('Ctrl Pts',(39.7377318669302,8.42750219560164,-29.6481990543948));
#53172=CARTESIAN_POINT('Ctrl Pts',(39.7475337255395,8.42556209647708,-29.6032497837854));
#53173=CARTESIAN_POINT('Ctrl Pts',(39.757461449336,8.42359708463452,-29.5577233217899));
#53174=CARTESIAN_POINT('Ctrl Pts',(39.7676348147295,8.42160156843537,-29.5117485114425));
#53175=CARTESIAN_POINT('Ctrl Pts',(39.7780765752702,8.41953687256901,-29.4650397996942));
#53176=CARTESIAN_POINT('Ctrl Pts',(39.7825055440345,8.41866111282865,-29.4452278700344));
#53177=CARTESIAN_POINT('Ctrl Pts',(39.7869828223184,8.41777282382613,-29.425283308357));
#53178=CARTESIAN_POINT('Ctrl Pts',(39.7915102532766,8.41686865746927,-29.4051814390361));
#53179=CARTESIAN_POINT('Ctrl Pts',(39.7979316406918,8.41558625194641,-29.3766703713094));
#53180=CARTESIAN_POINT('Ctrl Pts',(39.8044540915392,8.4142714260871,-29.3478383316315));
#53181=CARTESIAN_POINT('Ctrl Pts',(39.8110618301717,8.41296548896544,-29.3190355764946));
#53182=CARTESIAN_POINT('Ctrl Pts',(39.8174072319651,8.41171139944787,-29.2913763326495));
#53183=CARTESIAN_POINT('Ctrl Pts',(39.8238312870333,8.41046549363018,-29.263743939833));
#53184=CARTESIAN_POINT('Ctrl Pts',(39.8303182042911,8.40926931741567,-29.2364965182498));
#53185=CARTESIAN_POINT('Ctrl Pts',(39.8325491549127,8.40885793401687,-29.2271257108693));
#53186=CARTESIAN_POINT('Ctrl Pts',(39.8347875241813,8.40845247797901,-29.2178008778995));
#53187=CARTESIAN_POINT('Ctrl Pts',(39.8370326159301,8.4080547876622,-29.208538029524));
#53188=CARTESIAN_POINT('Ctrl Pts',(39.837336887212,8.40800088975689,-29.2072826604502));
#53189=CARTESIAN_POINT('Ctrl Pts',(39.837641291277,8.40794698587253,-29.2060268678952));
#53190=CARTESIAN_POINT('Ctrl Pts',(39.8379458282931,8.40789307599463,-29.2047706507169));
#53191=CARTESIAN_POINT('',(37.4911183000542,8.66292929398162,-41.3743318420141));
#53192=CARTESIAN_POINT('Ctrl Pts',(37.4911898651196,8.66293555381076,-41.3740674147214));
#53193=CARTESIAN_POINT('Ctrl Pts',(37.6801716473364,8.68001236440291,-40.6833502317314));
#53194=CARTESIAN_POINT('Ctrl Pts',(38.0233165576779,8.70919148388572,-39.5173351893382));
#53195=CARTESIAN_POINT('Ctrl Pts',(38.4518695777218,8.70933987554425,-37.8053909622071));
#53196=CARTESIAN_POINT('Ctrl Pts',(38.6892091015529,8.68608245062232,-36.6248757859991));
#53197=CARTESIAN_POINT('Ctrl Pts',(38.818728329062,8.66459053329314,-35.8932912681495));
#53198=CARTESIAN_POINT('Ctrl Pts',(38.8824625141317,8.65036952003038,-35.4979095277334));
#53199=CARTESIAN_POINT('Ctrl Pts',(38.9091460645523,8.64371781549238,-35.3259113004388));
#53200=CARTESIAN_POINT('',(36.4975121937785,8.64395853169441,-47.4046427887098));
#53201=CARTESIAN_POINT('Ctrl Pts',(36.4974760183619,8.64411817641805,-47.4042708861961));
#53202=CARTESIAN_POINT('Ctrl Pts',(36.5017609841129,8.64268775187304,-47.3573097347399));
#53203=CARTESIAN_POINT('Ctrl Pts',(36.5059335353835,8.64129768267962,-47.3111892821043));
#53204=CARTESIAN_POINT('Ctrl Pts',(36.5099914476731,8.6399524796883,-47.2660110824115));
#53205=CARTESIAN_POINT('Ctrl Pts',(36.5144484058799,8.63847499247709,-47.2163901607351));
#53206=CARTESIAN_POINT('Ctrl Pts',(36.518767198879,8.63705162890043,-47.1679050560211));
#53207=CARTESIAN_POINT('Ctrl Pts',(36.5229530172055,8.63568534639452,-47.1206225324743));
#53208=CARTESIAN_POINT('Ctrl Pts',(36.5274144350992,8.63422910612218,-47.0702268678377));
#53209=CARTESIAN_POINT('Ctrl Pts',(36.5317261160483,8.63283736585082,-47.0211834002847));
#53210=CARTESIAN_POINT('Ctrl Pts',(36.5358915607992,8.631513263941,-46.9736167749596));
#53211=CARTESIAN_POINT('Ctrl Pts',(36.537647500156,8.63095509001365,-46.9535651083383));
#53212=CARTESIAN_POINT('Ctrl Pts',(36.5393775323541,8.63040888592338,-46.9337750226926));
#53213=CARTESIAN_POINT('Ctrl Pts',(36.5410820584912,8.62987472195882,-46.9142539481906));
#53214=CARTESIAN_POINT('Ctrl Pts',(36.5414176071999,8.62976956779039,-46.9104110787865));
#53215=CARTESIAN_POINT('Ctrl Pts',(36.5417522008652,8.62966486911207,-46.9065782521653));
#53216=CARTESIAN_POINT('Ctrl Pts',(36.5420870513848,8.62956024964645,-46.9027416653917));
#53217=CARTESIAN_POINT('Ctrl Pts',(36.5460702365561,8.62831575791135,-46.8571038818039));
#53218=CARTESIAN_POINT('Ctrl Pts',(36.5500453677753,8.62709642970009,-46.8114405783938));
#53219=CARTESIAN_POINT('Ctrl Pts',(36.5540243986474,8.62590470392077,-46.7657539407575));
#53220=CARTESIAN_POINT('Ctrl Pts',(36.556385723778,8.62519748346384,-46.7386415586093));
#53221=CARTESIAN_POINT('Ctrl Pts',(36.5587485687228,8.62449993284698,-46.7115197533868));
#53222=CARTESIAN_POINT('Ctrl Pts',(36.5611163443151,8.62381217719835,-46.6843811764931));
#53223=CARTESIAN_POINT('Ctrl Pts',(36.562423756438,8.62343241989551,-46.66939609744));
#53224=CARTESIAN_POINT('Ctrl Pts',(36.5637327734946,8.62305562005744,-46.6544047768329));
#53225=CARTESIAN_POINT('Ctrl Pts',(36.5650426602007,8.62268214977037,-46.6394210330265));
#53226=CARTESIAN_POINT('Ctrl Pts',(36.5684349148007,8.62171496207895,-46.6006171627238));
#53227=CARTESIAN_POINT('Ctrl Pts',(36.5718357059482,8.62076932915961,-46.5618331423751));
#53228=CARTESIAN_POINT('Ctrl Pts',(36.5752641319001,8.61984224913339,-46.5229435211988));
#53229=CARTESIAN_POINT('Ctrl Pts',(36.5814415558131,8.61817181307802,-46.4528712258681));
#53230=CARTESIAN_POINT('Ctrl Pts',(36.5877090791056,8.61656174374666,-46.3824547510109));
#53231=CARTESIAN_POINT('Ctrl Pts',(36.594089463791,8.61503000670491,-46.3119630026283));
#53232=CARTESIAN_POINT('Ctrl Pts',(36.595834692974,8.61461103005729,-46.2926813664097));
#53233=CARTESIAN_POINT('Ctrl Pts',(36.5975882890355,8.61419790459739,-46.2733946228975));
#53234=CARTESIAN_POINT('Ctrl Pts',(36.5993525794991,8.61379052995912,-46.2540873946039));
#53235=CARTESIAN_POINT('Ctrl Pts',(36.6123492664835,8.61078959515377,-46.1118602455913));
#53236=CARTESIAN_POINT('Ctrl Pts',(36.6259089518447,8.60810497287949,-45.9687191069632));
#53237=CARTESIAN_POINT('Ctrl Pts',(36.6404465288085,8.60582064395813,-45.8241744715311));
#53238=CARTESIAN_POINT('Ctrl Pts',(36.6574427818986,8.60314997658452,-45.6551836408901));
#53239=CARTESIAN_POINT('Ctrl Pts',(36.6757747741864,8.60102579619041,-45.4842673506916));
#53240=CARTESIAN_POINT('Ctrl Pts',(36.6961137047484,8.59958744575822,-45.3106010637092));
#53241=CARTESIAN_POINT('Ctrl Pts',(36.7014364382353,8.59921102694957,-45.2651522944906));
#53242=CARTESIAN_POINT('Ctrl Pts',(36.7068966967673,8.59888163230131,-45.2195153674192));
#53243=CARTESIAN_POINT('Ctrl Pts',(36.7125067718823,8.59860188028545,-45.1736754567841));
#53244=CARTESIAN_POINT('Ctrl Pts',(36.716359917578,8.5984097393152,-45.142191412322));
#53245=CARTESIAN_POINT('Ctrl Pts',(36.7202825680454,8.59824107383479,-45.1106211484891));
#53246=CARTESIAN_POINT('Ctrl Pts',(36.7242791266398,8.59809669301701,-45.0789560892659));
#53247=CARTESIAN_POINT('Ctrl Pts',(36.7366984669174,8.59764802838137,-44.9805566448154));
#53248=CARTESIAN_POINT('Ctrl Pts',(36.7498311650086,8.59743340908391,-44.8812354332942));
#53249=CARTESIAN_POINT('Ctrl Pts',(36.7638292859017,8.59748007452552,-44.7806458610636));
#53250=CARTESIAN_POINT('Ctrl Pts',(36.7691763788146,8.59749790009325,-44.7422220045413));
#53251=CARTESIAN_POINT('Ctrl Pts',(36.7746499508775,8.59755391226604,-44.7036127882181));
#53252=CARTESIAN_POINT('Ctrl Pts',(36.7802459639653,8.59764698565104,-44.664850828662));
#53253=CARTESIAN_POINT('Ctrl Pts',(36.7831524683006,8.59769532688841,-44.6447183161522));
#53254=CARTESIAN_POINT('Ctrl Pts',(36.7860916992519,8.59775366030292,-44.6245466950945));
#53255=CARTESIAN_POINT('Ctrl Pts',(36.7890641096592,8.59782186120053,-44.6043338411012));
#53256=CARTESIAN_POINT('Ctrl Pts',(36.7982395704418,8.5980323888786,-44.5419392778655));
#53257=CARTESIAN_POINT('Ctrl Pts',(36.8077393750307,8.59833696666467,-44.4790921606058));
#53258=CARTESIAN_POINT('Ctrl Pts',(36.8175796728728,8.59873406400653,-44.415757223244));
#53259=CARTESIAN_POINT('Ctrl Pts',(36.8188383897378,8.59878485851797,-44.407655765841));
#53260=CARTESIAN_POINT('Ctrl Pts',(36.8201026882879,8.59883717004869,-44.399546329321));
#53261=CARTESIAN_POINT('Ctrl Pts',(36.821372612154,8.59889099821599,-44.391428839473));
#53262=CARTESIAN_POINT('Ctrl Pts',(36.8223610381664,8.59893289455495,-44.3851107141618));
#53263=CARTESIAN_POINT('Ctrl Pts',(36.8233528898425,8.59897571162432,-44.3787876223995));
#53264=CARTESIAN_POINT('Ctrl Pts',(36.8243458969836,8.59901934535582,-44.3724740243719));
#53265=CARTESIAN_POINT('Ctrl Pts',(36.838789710824,8.59965402104843,-44.2806394032497));
#53266=CARTESIAN_POINT('Ctrl Pts',(36.8535934776877,8.60046538228348,-44.1900559875258));
#53267=CARTESIAN_POINT('Ctrl Pts',(36.8687566014926,8.60143265418725,-44.1006242196692));
#53268=CARTESIAN_POINT('Ctrl Pts',(36.8826235674842,8.60231724279622,-44.0188371618449));
#53269=CARTESIAN_POINT('Ctrl Pts',(36.8967918685694,8.6033324784733,-43.9380103420868));
#53270=CARTESIAN_POINT('Ctrl Pts',(36.9112857225907,8.60447070040713,-43.8580679367849));
#53271=CARTESIAN_POINT('Ctrl Pts',(36.9384153257078,8.60660122478518,-43.7084317030483));
#53272=CARTESIAN_POINT('Ctrl Pts',(36.9666925269518,8.60916555894038,-43.5619136599842));
#53273=CARTESIAN_POINT('Ctrl Pts',(36.9959471215658,8.61202820481559,-43.4179272462726));
#53274=CARTESIAN_POINT('Ctrl Pts',(37.0180880069539,8.61419475386768,-43.3089533662543));
#53275=CARTESIAN_POINT('Ctrl Pts',(37.0407868905128,8.61653172315501,-43.2014336937385));
#53276=CARTESIAN_POINT('Ctrl Pts',(37.0639612478015,8.61897702647482,-43.0950922117049));
#53277=CARTESIAN_POINT('Ctrl Pts',(37.071407004209,8.61976268506439,-43.0609254487882));
#53278=CARTESIAN_POINT('Ctrl Pts',(37.0789018371853,8.62055951697033,-43.0268800101056));
#53279=CARTESIAN_POINT('Ctrl Pts',(37.0864429363177,8.62136543706961,-42.9929462645575));
#53280=CARTESIAN_POINT('Ctrl Pts',(37.1086169465024,8.62373518187414,-42.8931667488425));
#53281=CARTESIAN_POINT('Ctrl Pts',(37.1311886149013,8.62618323438476,-42.7943634428842));
#53282=CARTESIAN_POINT('Ctrl Pts',(37.1541236014169,8.62867697054841,-42.696357845321));
#53283=CARTESIAN_POINT('Ctrl Pts',(37.1694195627341,8.63034011047957,-42.6309952680123));
#53284=CARTESIAN_POINT('Ctrl Pts',(37.1848765769503,8.63202351303894,-42.5659898511523));
#53285=CARTESIAN_POINT('Ctrl Pts',(37.2004833982249,8.63371744373424,-42.5012925931775));
#53286=CARTESIAN_POINT('Ctrl Pts',(37.2234845648212,8.63621394071077,-42.405942464998));
#53287=CARTESIAN_POINT('Ctrl Pts',(37.2468132737793,8.63873357086562,-42.3112505507811));
#53288=CARTESIAN_POINT('Ctrl Pts',(37.2704802586746,8.6412502632337,-42.2168802808142));
#53289=CARTESIAN_POINT('Ctrl Pts',(37.2806197694381,8.6423284753282,-42.1764497666481));
#53290=CARTESIAN_POINT('Ctrl Pts',(37.2908220477617,8.64340621535967,-42.1360759299403));
#53291=CARTESIAN_POINT('Ctrl Pts',(37.3010859637758,8.644481192736,-42.0957411959757));
#53292=CARTESIAN_POINT('Ctrl Pts',(37.3309930243853,8.647613468322,-41.9782136040035));
#53293=CARTESIAN_POINT('Ctrl Pts',(37.3614146919285,8.65072108931857,-41.8610575206228));
#53294=CARTESIAN_POINT('Ctrl Pts',(37.3921802979378,8.65373381794591,-41.7443617179619));
#53295=CARTESIAN_POINT('Ctrl Pts',(37.4247914593669,8.65692727298719,-41.6206656120724));
#53296=CARTESIAN_POINT('Ctrl Pts',(37.4577901536412,8.66001389139707,-41.4974790863762));
#53297=CARTESIAN_POINT('Ctrl Pts',(37.4909751693545,8.66291677591587,-41.3748606964831));
#53298=CARTESIAN_POINT('',(34.9058155546954,8.66668722396345,-53.4453943172971));
#53299=CARTESIAN_POINT('Ctrl Pts',(34.9063163914155,8.66722257324602,-53.4437571318374));
#53300=CARTESIAN_POINT('Ctrl Pts',(35.1934727320302,8.72417720600899,-52.7556732998408));
#53301=CARTESIAN_POINT('Ctrl Pts',(35.6781869696737,8.77551394752499,-51.5893141420722));
#53302=CARTESIAN_POINT('Ctrl Pts',(36.1004243200409,8.76372397778573,-50.1832810022625));
#53303=CARTESIAN_POINT('Ctrl Pts',(36.3808701953256,8.69787452481665,-48.6485604468675));
#53304=CARTESIAN_POINT('Ctrl Pts',(36.4554561965542,8.65716158483284,-47.8501354265767));
#53305=CARTESIAN_POINT('Ctrl Pts',(36.4974177553681,8.64413762617975,-47.4049093964135));
#53306=CARTESIAN_POINT('',(32.8153450360175,8.33795397633509,-59.2035503428015));
#53307=CARTESIAN_POINT('Ctrl Pts',(32.8153447698313,8.33795299861922,-59.2035496355344));
#53308=CARTESIAN_POINT('Ctrl Pts',(32.8259142758667,8.33379969528807,-59.1737918941683));
#53309=CARTESIAN_POINT('Ctrl Pts',(32.836888046712,8.32960496057437,-59.1426558331879));
#53310=CARTESIAN_POINT('Ctrl Pts',(32.84820294588,8.32543107112663,-59.1103062534762));
#53311=CARTESIAN_POINT('Ctrl Pts',(32.8590619641319,8.32142534902326,-59.0792600487053));
#53312=CARTESIAN_POINT('Ctrl Pts',(32.8702352647792,8.31743909897791,-59.047095978524));
#53313=CARTESIAN_POINT('Ctrl Pts',(32.8816554232607,8.31352701533988,-59.0140069035606));
#53314=CARTESIAN_POINT('Ctrl Pts',(32.8847282162794,8.31247440093782,-59.0051037102549));
#53315=CARTESIAN_POINT('Ctrl Pts',(32.887818809973,8.31142714143201,-58.9961338291535));
#53316=CARTESIAN_POINT('Ctrl Pts',(32.8909257279932,8.31038625917849,-58.9871016512053));
#53317=CARTESIAN_POINT('Ctrl Pts',(32.9166461377401,8.30176938616025,-58.9123293797061));
#53318=CARTESIAN_POINT('Ctrl Pts',(32.9434850606827,8.29359020115758,-58.8332884311441));
#53319=CARTESIAN_POINT('Ctrl Pts',(32.9715704512017,8.286120681936,-58.7496650526602));
#53320=CARTESIAN_POINT('Ctrl Pts',(32.9994388641737,8.27870886951243,-58.6666877180873));
#53321=CARTESIAN_POINT('Ctrl Pts',(33.028543782772,8.27192349048084,-58.5792095859131));
#53322=CARTESIAN_POINT('Ctrl Pts',(33.0590264471052,8.26603260100496,-58.4868732050853));
#53323=CARTESIAN_POINT('Ctrl Pts',(33.0827962253682,8.2614390019979,-58.414871123053));
#53324=CARTESIAN_POINT('Ctrl Pts',(33.1073972028525,8.25743539344415,-58.3399095066768));
#53325=CARTESIAN_POINT('Ctrl Pts',(33.1329039327878,8.25415052960207,-58.2617933242852));
#53326=CARTESIAN_POINT('Ctrl Pts',(33.1444908198075,8.25265832161187,-58.2263076551273));
#53327=CARTESIAN_POINT('Ctrl Pts',(33.1562652731685,8.25131438810635,-58.1901689837327));
#53328=CARTESIAN_POINT('Ctrl Pts',(33.1682348793725,8.25013104739556,-58.153357072047));
#53329=CARTESIAN_POINT('Ctrl Pts',(33.172888612169,8.24967096947977,-58.13904475485));
#53330=CARTESIAN_POINT('Ctrl Pts',(33.1775716886937,8.24923518581891,-58.1246311479278));
#53331=CARTESIAN_POINT('Ctrl Pts',(33.1822843164442,8.24882444181012,-58.1101157969434));
#53332=CARTESIAN_POINT('Ctrl Pts',(33.1977570970947,8.24747586256983,-58.0624581304058));
#53333=CARTESIAN_POINT('Ctrl Pts',(33.2135484995211,8.24639726237193,-58.0137034575228));
#53334=CARTESIAN_POINT('Ctrl Pts',(33.2297106092063,8.24563674393401,-57.9637961640372));
#53335=CARTESIAN_POINT('Ctrl Pts',(33.2471482039732,8.24481620672745,-57.9099502753097));
#53336=CARTESIAN_POINT('Ctrl Pts',(33.2650142543286,8.24436619688766,-57.8547722516667));
#53337=CARTESIAN_POINT('Ctrl Pts',(33.2833684711262,8.24434526101578,-57.7982094792638));
#53338=CARTESIAN_POINT('Ctrl Pts',(33.3063215665668,8.24431907939927,-57.7274741965948));
#53339=CARTESIAN_POINT('Ctrl Pts',(33.3300375594471,8.24496406860893,-57.6545752851795));
#53340=CARTESIAN_POINT('Ctrl Pts',(33.3546344753326,8.24638956625908,-57.5794018081793));
#53341=CARTESIAN_POINT('Ctrl Pts',(33.3614229390721,8.24678298709094,-57.558654799686));
#53342=CARTESIAN_POINT('Ctrl Pts',(33.3682785492559,8.24723583050548,-57.5377343596278));
#53343=CARTESIAN_POINT('Ctrl Pts',(33.3752037881199,8.24775032850502,-57.516638067781));
#53344=CARTESIAN_POINT('Ctrl Pts',(33.3821513819785,8.24826648732813,-57.4954736761183));
#53345=CARTESIAN_POINT('Ctrl Pts',(33.389166411806,8.24884449413713,-57.474140342021));
#53346=CARTESIAN_POINT('Ctrl Pts',(33.3962529902172,8.2494866177797,-57.4526306323922));
#53347=CARTESIAN_POINT('Ctrl Pts',(33.4076971023218,8.25052358294455,-57.417894612547));
#53348=CARTESIAN_POINT('Ctrl Pts',(33.4193286235789,8.25172775605007,-57.3826960849223));
#53349=CARTESIAN_POINT('Ctrl Pts',(33.4311705155945,8.25310999857074,-57.3469870633452));
#53350=CARTESIAN_POINT('Ctrl Pts',(33.4429082771928,8.25448008648889,-57.3115920452495));
#53351=CARTESIAN_POINT('Ctrl Pts',(33.4548527326506,8.25602512572448,-57.2756954318753));
#53352=CARTESIAN_POINT('Ctrl Pts',(33.4669948717588,8.25773922660508,-57.2393361990404));
#53353=CARTESIAN_POINT('Ctrl Pts',(33.4748222932729,8.25884422054318,-57.2158972449326));
#53354=CARTESIAN_POINT('Ctrl Pts',(33.4827312053234,8.26001935464201,-57.1922679924709));
#53355=CARTESIAN_POINT('Ctrl Pts',(33.4907291824969,8.26126493817209,-57.1684294560724));
#53356=CARTESIAN_POINT('Ctrl Pts',(33.5104238457025,8.26433213223717,-57.1097281200348));
#53357=CARTESIAN_POINT('Ctrl Pts',(33.530650114247,8.26782441812749,-57.0497816457331));
#53358=CARTESIAN_POINT('Ctrl Pts',(33.5514510113948,8.27174678432962,-56.9885302069414));
#53359=CARTESIAN_POINT('Ctrl Pts',(33.5536522114834,8.27216185838965,-56.9820484349517));
#53360=CARTESIAN_POINT('Ctrl Pts',(33.5558598550761,8.27258176223285,-56.9755520437706));
#53361=CARTESIAN_POINT('Ctrl Pts',(33.5580739984412,8.27300651115138,-56.9690409614721));
#53362=CARTESIAN_POINT('Ctrl Pts',(33.5598274302077,8.27334287972545,-56.9638846835561));
#53363=CARTESIAN_POINT('Ctrl Pts',(33.5615847458961,8.27368225369376,-56.958719762588));
#53364=CARTESIAN_POINT('Ctrl Pts',(33.5633416033356,8.27402377918612,-56.9535589856994));
#53365=CARTESIAN_POINT('Ctrl Pts',(33.5837469887939,8.2779904979185,-56.8936180711393));
#53366=CARTESIAN_POINT('Ctrl Pts',(33.6042412054578,8.28227489925269,-56.8337918778109));
#53367=CARTESIAN_POINT('Ctrl Pts',(33.6248563320432,8.28685556871978,-56.7740171494789));
#53368=CARTESIAN_POINT('Ctrl Pts',(33.6443100297644,8.29117816935014,-56.7176100499874));
#53369=CARTESIAN_POINT('Ctrl Pts',(33.663873298769,8.29576527135127,-56.6612431340435));
#53370=CARTESIAN_POINT('Ctrl Pts',(33.6835833024292,8.30061282476209,-56.6048470285847));
#53371=CARTESIAN_POINT('Ctrl Pts',(33.6893816449354,8.30203889121431,-56.5882562688313));
#53372=CARTESIAN_POINT('Ctrl Pts',(33.6951926237817,8.30348754214602,-56.5716632461933));
#53373=CARTESIAN_POINT('Ctrl Pts',(33.7010204123138,8.30495966895789,-56.5550572898264));
#53374=CARTESIAN_POINT('Ctrl Pts',(33.715002721784,8.30849166613824,-56.5152154836775));
#53375=CARTESIAN_POINT('Ctrl Pts',(33.7290746865241,8.31215704388324,-56.4753195088408));
#53376=CARTESIAN_POINT('Ctrl Pts',(33.74322157891,8.31595074092791,-56.4354301621671));
#53377=CARTESIAN_POINT('Ctrl Pts',(33.7581621889465,8.31995728502219,-56.3933028060662));
#53378=CARTESIAN_POINT('Ctrl Pts',(33.773186237498,8.32410693444565,-56.3511832323761));
#53379=CARTESIAN_POINT('Ctrl Pts',(33.7883319940688,8.32840148291067,-56.3089714939313));
#53380=CARTESIAN_POINT('Ctrl Pts',(33.7954479669976,8.33041920255878,-56.2891390354705));
#53381=CARTESIAN_POINT('Ctrl Pts',(33.802591452665,8.33246909818501,-56.2692844582634));
#53382=CARTESIAN_POINT('Ctrl Pts',(33.8097645416245,8.33455082052943,-56.2494026966234));
#53383=CARTESIAN_POINT('Ctrl Pts',(33.8462246713151,8.34513201742883,-56.1483455911049));
#53384=CARTESIAN_POINT('Ctrl Pts',(33.8833759461346,8.35651669070866,-56.0467964423657));
#53385=CARTESIAN_POINT('Ctrl Pts',(33.9213794241352,8.36859834249817,-55.944346058535));
#53386=CARTESIAN_POINT('Ctrl Pts',(33.9236399780667,8.36931699318198,-55.9382520210905));
#53387=CARTESIAN_POINT('Ctrl Pts',(33.9259035368344,8.370038098574,-55.9321548016935));
#53388=CARTESIAN_POINT('Ctrl Pts',(33.9281701296812,8.37076163202236,-55.9260543186707));
#53389=CARTESIAN_POINT('Ctrl Pts',(33.9573143269606,8.38006493569585,-55.8476133754845));
#53390=CARTESIAN_POINT('Ctrl Pts',(33.9869603922587,8.38976832201774,-55.7686344037265));
#53391=CARTESIAN_POINT('Ctrl Pts',(34.0171999918353,8.39974841800064,-55.6889038557678));
#53392=CARTESIAN_POINT('Ctrl Pts',(34.0281218179651,8.40335299195699,-55.6601070729322));
#53393=CARTESIAN_POINT('Ctrl Pts',(34.0391208754096,8.40699358016688,-55.6312126412986));
#53394=CARTESIAN_POINT('Ctrl Pts',(34.0502007239699,8.41066410234706,-55.6022121085287));
#53395=CARTESIAN_POINT('Ctrl Pts',(34.0643034591948,8.41533604367935,-55.565299434785));
#53396=CARTESIAN_POINT('Ctrl Pts',(34.0785184752553,8.42007191091369,-55.5282494150646));
#53397=CARTESIAN_POINT('Ctrl Pts',(34.092875808014,8.42487556703544,-55.4909786487536));
#53398=CARTESIAN_POINT('Ctrl Pts',(34.1181955193908,8.43334700031626,-55.4252502114704));
#53399=CARTESIAN_POINT('Ctrl Pts',(34.1439565202898,8.44202869183888,-55.3588378159729));
#53400=CARTESIAN_POINT('Ctrl Pts',(34.1701229500259,8.45086466932254,-55.2917559898774));
#53401=CARTESIAN_POINT('Ctrl Pts',(34.1951835073361,8.45932721168519,-55.2275092445516));
#53402=CARTESIAN_POINT('Ctrl Pts',(34.2206382490956,8.46793947463191,-55.1625911095839));
#53403=CARTESIAN_POINT('Ctrl Pts',(34.2465119704947,8.47666674763625,-55.096886514898));
#53404=CARTESIAN_POINT('Ctrl Pts',(34.2810334275061,8.48831092418124,-55.0092215707671));
#53405=CARTESIAN_POINT('Ctrl Pts',(34.316300310326,8.50016098260613,-54.9201579067433));
#53406=CARTESIAN_POINT('Ctrl Pts',(34.3523754032991,8.51211590055436,-54.8294370320581));
#53407=CARTESIAN_POINT('Ctrl Pts',(34.3580566585003,8.51399861059544,-54.8151499326029));
#53408=CARTESIAN_POINT('Ctrl Pts',(34.3637579344201,8.51588386178967,-54.8008218174869));
#53409=CARTESIAN_POINT('Ctrl Pts',(34.3694794325271,8.5177711795535,-54.7864518076394));
#53410=CARTESIAN_POINT('Ctrl Pts',(34.4062918113315,8.52991426780531,-54.6939945113097));
#53411=CARTESIAN_POINT('Ctrl Pts',(34.4429234458461,8.54180511233091,-54.6023582808303));
#53412=CARTESIAN_POINT('Ctrl Pts',(34.4793139250894,8.55331711614767,-54.5115448246281));
#53413=CARTESIAN_POINT('Ctrl Pts',(34.4859936988634,8.55543023976629,-54.4948752628174));
#53414=CARTESIAN_POINT('Ctrl Pts',(34.492665423656,8.55753061500944,-54.4782333035134));
#53415=CARTESIAN_POINT('Ctrl Pts',(34.4993288064946,8.55961746400979,-54.4616188411806));
#53416=CARTESIAN_POINT('Ctrl Pts',(34.508307513822,8.56242943007335,-54.4392313544787));
#53417=CARTESIAN_POINT('Ctrl Pts',(34.5172710772812,8.56521684015726,-54.4168937849649));
#53418=CARTESIAN_POINT('Ctrl Pts',(34.5262216330844,8.56797891631761,-54.3945976038152));
#53419=CARTESIAN_POINT('Ctrl Pts',(34.5399062564537,8.5722018911588,-54.360508677014));
#53420=CARTESIAN_POINT('Ctrl Pts',(34.5535550570989,8.57636392293325,-54.3265300154006));
#53421=CARTESIAN_POINT('Ctrl Pts',(34.5671649038471,8.5804587094149,-54.2926582644767));
#53422=CARTESIAN_POINT('Ctrl Pts',(34.6093466406989,8.59314990344738,-54.1876777080735));
#53423=CARTESIAN_POINT('Ctrl Pts',(34.6511540459079,8.60519202444507,-54.083728340169));
#53424=CARTESIAN_POINT('Ctrl Pts',(34.6927510226543,8.6164196351585,-53.9801080854673));
#53425=CARTESIAN_POINT('Ctrl Pts',(34.7070257878526,8.6202725956188,-53.9445488953207));
#53426=CARTESIAN_POINT('Ctrl Pts',(34.7212757582281,8.62402996101889,-53.9090280240373));
#53427=CARTESIAN_POINT('Ctrl Pts',(34.7355072873544,8.62768595039805,-53.8735157136822));
#53428=CARTESIAN_POINT('Ctrl Pts',(34.7609434211676,8.63422033150661,-53.810044257439));
#53429=CARTESIAN_POINT('Ctrl Pts',(34.7863201703147,8.64043513357872,-53.7465942195638));
#53430=CARTESIAN_POINT('Ctrl Pts',(34.8112855448272,8.64622252443879,-53.6839604325147));
#53431=CARTESIAN_POINT('Ctrl Pts',(34.8178852864895,8.6477524548052,-53.6674028273544));
#53432=CARTESIAN_POINT('Ctrl Pts',(34.8244563799806,8.64925272860502,-53.6509021159995));
#53433=CARTESIAN_POINT('Ctrl Pts',(34.8309925582067,8.650721840173,-53.6344726598005));
#53434=CARTESIAN_POINT('Ctrl Pts',(34.8541971497883,8.65593744671606,-53.5761451773154));
#53435=CARTESIAN_POINT('Ctrl Pts',(34.8769595552522,8.66075536322111,-53.5187196936103));
#53436=CARTESIAN_POINT('Ctrl Pts',(34.8990072868524,8.6650774614646,-53.4628834086385));
#53437=CARTESIAN_POINT('Ctrl Pts',(34.9011747086567,8.66550234916474,-53.4573943731354));
#53438=CARTESIAN_POINT('Ctrl Pts',(34.9033352418631,8.6659224793078,-53.4519206795066));
#53439=CARTESIAN_POINT('Ctrl Pts',(34.9054886396442,8.66633778125862,-53.4464629701074));
#53440=CARTESIAN_POINT('',(30.3373688833396,9.77553124130065,-64.7925772570577));
#53441=CARTESIAN_POINT('Ctrl Pts',(30.3373684825906,9.77557092417984,-64.7925605023553));
#53442=CARTESIAN_POINT('Ctrl Pts',(30.3375463229291,9.77544705826916,-64.7922628769377));
#53443=CARTESIAN_POINT('Ctrl Pts',(30.3377241674401,9.77532319428866,-64.7919652277452));
#53444=CARTESIAN_POINT('Ctrl Pts',(30.3379020161204,9.77519933220178,-64.7916675546795));
#53445=CARTESIAN_POINT('Ctrl Pts',(30.4036061558056,9.72943991559357,-64.6816956805759));
#53446=CARTESIAN_POINT('Ctrl Pts',(30.4698883800189,9.68484787112186,-64.5713024429491));
#53447=CARTESIAN_POINT('Ctrl Pts',(30.5367348270984,9.64110666805661,-64.4594875830257));
#53448=CARTESIAN_POINT('Ctrl Pts',(30.5532694353223,9.6302871901708,-64.4318299440156));
#53449=CARTESIAN_POINT('Ctrl Pts',(30.5698384647393,9.61951997556837,-64.4040851911615));
#53450=CARTESIAN_POINT('Ctrl Pts',(30.5864416055175,9.60880010688694,-64.376236554061));
#53451=CARTESIAN_POINT('Ctrl Pts',(30.6029407158524,9.59814740577976,-64.3485624084078));
#53452=CARTESIAN_POINT('Ctrl Pts',(30.6194735127258,9.58754145673769,-64.3207856723907));
#53453=CARTESIAN_POINT('Ctrl Pts',(30.6360396182955,9.57697783103276,-64.2928904738032));
#53454=CARTESIAN_POINT('Ctrl Pts',(30.6688000900593,9.55608762481185,-64.2377260380931));
#53455=CARTESIAN_POINT('Ctrl Pts',(30.7016908435539,9.53536279863202,-64.1820984392842));
#53456=CARTESIAN_POINT('Ctrl Pts',(30.7347086744899,9.51477022684478,-64.1258818683911));
#53457=CARTESIAN_POINT('Ctrl Pts',(30.7989006919381,9.47473492803825,-64.0165877386031));
#53458=CARTESIAN_POINT('Ctrl Pts',(30.8635734637805,9.43519782370463,-63.9050699203138));
#53459=CARTESIAN_POINT('Ctrl Pts',(30.9286992633925,9.39592330007792,-63.7903478022949));
#53460=CARTESIAN_POINT('Ctrl Pts',(30.9322875485719,9.39375936210095,-63.7840268714457));
#53461=CARTESIAN_POINT('Ctrl Pts',(30.9358772074505,9.39159622837222,-63.7776962036545));
#53462=CARTESIAN_POINT('Ctrl Pts',(30.9394682353198,9.38943386640271,-63.7713556428843));
#53463=CARTESIAN_POINT('Ctrl Pts',(30.9673747151068,9.37262978890998,-63.7220820818283));
#53464=CARTESIAN_POINT('Ctrl Pts',(30.9953638849514,9.35587219743963,-63.6722110687769));
#53465=CARTESIAN_POINT('Ctrl Pts',(31.0234333085263,9.33914738700648,-63.6216701776393));
#53466=CARTESIAN_POINT('Ctrl Pts',(31.0543134478064,9.32074784722863,-63.5660684032211));
#53467=CARTESIAN_POINT('Ctrl Pts',(31.0852907474618,9.30238796850476,-63.5096560444589));
#53468=CARTESIAN_POINT('Ctrl Pts',(31.1163613946637,9.28404855304618,-63.4523275077404));
#53469=CARTESIAN_POINT('Ctrl Pts',(31.1829819817661,9.24472582452293,-63.3294056790099));
#53470=CARTESIAN_POINT('Ctrl Pts',(31.2500330279944,9.20549427976786,-63.2022717921672));
#53471=CARTESIAN_POINT('Ctrl Pts',(31.3174662640762,9.16620743702038,-63.0699186138175));
#53472=CARTESIAN_POINT('Ctrl Pts',(31.356885099242,9.14324188370522,-62.9925501168538));
#53473=CARTESIAN_POINT('Ctrl Pts',(31.3964342454244,9.12025823995894,-62.9133979272066));
#53474=CARTESIAN_POINT('Ctrl Pts',(31.436099984031,9.09723452561081,-62.8322600716));
#53475=CARTESIAN_POINT('Ctrl Pts',(31.4465581059631,9.09116417824198,-62.8108675646896));
#53476=CARTESIAN_POINT('Ctrl Pts',(31.4570222813784,9.08509167798631,-62.7893392930934));
#53477=CARTESIAN_POINT('Ctrl Pts',(31.4674908820943,9.07901874264532,-62.7676786570229));
#53478=CARTESIAN_POINT('Ctrl Pts',(31.5209901089275,9.047983329779,-62.6569831291357));
#53479=CARTESIAN_POINT('Ctrl Pts',(31.574607074813,9.01693952807107,-62.5428290251401));
#53480=CARTESIAN_POINT('Ctrl Pts',(31.6281106237607,8.98608871872255,-62.4256639577479));
#53481=CARTESIAN_POINT('Ctrl Pts',(31.6807944160655,8.95571059121297,-62.3102940393545));
#53482=CARTESIAN_POINT('Ctrl Pts',(31.7333686664999,8.92551918584558,-62.1920045938983));
#53483=CARTESIAN_POINT('Ctrl Pts',(31.7855822717626,8.89567426032026,-62.071244707503));
#53484=CARTESIAN_POINT('Ctrl Pts',(31.8368240386367,8.86638483070797,-61.9527324937746));
#53485=CARTESIAN_POINT('Ctrl Pts',(31.8877185600007,8.83742885512422,-61.8318400901663));
#53486=CARTESIAN_POINT('Ctrl Pts',(31.9379950259541,8.80893211037967,-61.7090524023681));
#53487=CARTESIAN_POINT('Ctrl Pts',(31.9905182826746,8.779161882669,-61.5807774903181));
#53488=CARTESIAN_POINT('Ctrl Pts',(32.0423671155747,8.74989268183046,-61.4504342096747));
#53489=CARTESIAN_POINT('Ctrl Pts',(32.0931938750543,8.72124186168149,-61.3186103997138));
#53490=CARTESIAN_POINT('Ctrl Pts',(32.1224075483681,8.70477424288037,-61.2428420887175));
#53491=CARTESIAN_POINT('Ctrl Pts',(32.1512828341325,8.68851045659444,-61.166585309833));
#53492=CARTESIAN_POINT('Ctrl Pts',(32.1797484643676,8.67246943556838,-61.0899561252136));
#53493=CARTESIAN_POINT('Ctrl Pts',(32.2341117036637,8.64183453104005,-60.9436108426356));
#53494=CARTESIAN_POINT('Ctrl Pts',(32.2870749287235,8.61198816189768,-60.7957628561251));
#53495=CARTESIAN_POINT('Ctrl Pts',(32.3387992780698,8.58324303503906,-60.6478476683524));
#53496=CARTESIAN_POINT('Ctrl Pts',(32.3944398342923,8.55232152771585,-60.4887333744958));
#53497=CARTESIAN_POINT('Ctrl Pts',(32.4486449703774,8.52267390784803,-60.3295428623252));
#53498=CARTESIAN_POINT('Ctrl Pts',(32.501630510655,8.49457301465818,-60.1718098794048));
#53499=CARTESIAN_POINT('Ctrl Pts',(32.5046546997238,8.49296913530613,-60.1628071522412));
#53500=CARTESIAN_POINT('Ctrl Pts',(32.5076749214702,8.49137028732541,-60.1538091845707));
#53501=CARTESIAN_POINT('Ctrl Pts',(32.5106912185181,8.48977651907442,-60.1448162661682));
#53502=CARTESIAN_POINT('Ctrl Pts',(32.5352852545509,8.47678138193424,-60.0714905440266));
#53503=CARTESIAN_POINT('Ctrl Pts',(32.5596149213573,8.46414266611182,-59.998591329611));
#53504=CARTESIAN_POINT('Ctrl Pts',(32.5835883165298,8.45183872019133,-59.9261096446501));
#53505=CARTESIAN_POINT('Ctrl Pts',(32.6107857864825,8.43788007157003,-59.8438802217977));
#53506=CARTESIAN_POINT('Ctrl Pts',(32.6375244536277,8.42435304402482,-59.762189720735));
#53507=CARTESIAN_POINT('Ctrl Pts',(32.6636616266459,8.41129914680092,-59.6814250560713));
#53508=CARTESIAN_POINT('Ctrl Pts',(32.6766561521125,8.40480918708737,-59.6412715746278));
#53509=CARTESIAN_POINT('Ctrl Pts',(32.6894507451753,8.39870830073878,-59.6027697852629));
#53510=CARTESIAN_POINT('Ctrl Pts',(32.7022892380683,8.39268048839557,-59.5642015698746));
#53511=CARTESIAN_POINT('Ctrl Pts',(32.7118904854834,8.38817259808776,-59.5353583885611));
#53512=CARTESIAN_POINT('Ctrl Pts',(32.7215159782231,8.38370675703068,-59.5064820798043));
#53513=CARTESIAN_POINT('Ctrl Pts',(32.731266476481,8.37912370098253,-59.4766551710175));
#53514=CARTESIAN_POINT('Ctrl Pts',(32.738674467287,8.37564170076368,-59.4539940248668));
#53515=CARTESIAN_POINT('Ctrl Pts',(32.7461545082956,8.37209237863037,-59.430785169056));
#53516=CARTESIAN_POINT('Ctrl Pts',(32.753749108309,8.3684033190236,-59.4065921797029));
#53517=CARTESIAN_POINT('Ctrl Pts',(32.7561506241305,8.36723678819956,-59.3989420274109));
#53518=CARTESIAN_POINT('Ctrl Pts',(32.7585635847051,8.36605624554138,-59.3911931144473));
#53519=CARTESIAN_POINT('Ctrl Pts',(32.7609893066747,8.36485926220333,-59.3833304692864));
#53520=CARTESIAN_POINT('Ctrl Pts',(32.7654154513653,8.36267516134063,-59.3689837281638));
#53521=CARTESIAN_POINT('Ctrl Pts',(32.7698841725407,8.36043567928045,-59.3542547618505));
#53522=CARTESIAN_POINT('Ctrl Pts',(32.7743993505077,8.35815864159974,-59.3392303200884));
#53523=CARTESIAN_POINT('Ctrl Pts',(32.7786170436054,8.35603162774136,-59.3251957715548));
#53524=CARTESIAN_POINT('Ctrl Pts',(32.7828752838157,8.3538717471765,-59.3109028270378));
#53525=CARTESIAN_POINT('Ctrl Pts',(32.7871761742764,8.35170090050936,-59.2964627260597));
#53526=CARTESIAN_POINT('Ctrl Pts',(32.7912324851766,8.34965350379485,-59.282843793066));
#53527=CARTESIAN_POINT('Ctrl Pts',(32.7953267422896,8.34759626861694,-59.2690934580539));
#53528=CARTESIAN_POINT('Ctrl Pts',(32.7994596002972,8.34555561824614,-59.2553498996653));
#53529=CARTESIAN_POINT('Ctrl Pts',(32.8033041258697,8.34365733562412,-59.2425651725866));
#53530=CARTESIAN_POINT('Ctrl Pts',(32.8071820576321,8.34177336230744,-59.229786038189));
#53531=CARTESIAN_POINT('Ctrl Pts',(32.8110928545661,8.33993297119414,-59.217168835316));
#53532=CARTESIAN_POINT('Ctrl Pts',(32.8121810991747,8.33942085160815,-59.2136578877435));
#53533=CARTESIAN_POINT('Ctrl Pts',(32.8132718816812,8.33891215942377,-59.2101597778347));
#53534=CARTESIAN_POINT('Ctrl Pts',(32.8143651736023,8.33840765419576,-59.206678606258));
#53535=CARTESIAN_POINT('Ctrl Pts',(32.8146919155016,8.33825687745151,-59.2056382211691));
#53536=CARTESIAN_POINT('Ctrl Pts',(32.8150189113244,8.33810590712252,-59.2045955534805));
#53537=CARTESIAN_POINT('Ctrl Pts',(32.8153461624519,8.33795474232361,-59.2035505847575));
#53538=CARTESIAN_POINT('',(27.8093579489698,12.8426393692443,-70.6502216958336));
#53539=CARTESIAN_POINT('Ctrl Pts',(27.8093579489706,12.8426393697467,-70.6502216955679));
#53540=CARTESIAN_POINT('Ctrl Pts',(28.1531837700217,12.2318062816667,-69.496432085362));
#53541=CARTESIAN_POINT('Ctrl Pts',(28.9080975096274,11.0141698218073,-67.3154640104755));
#53542=CARTESIAN_POINT('Ctrl Pts',(29.7727535124309,10.1579126475408,-65.7117945504243));
#53543=CARTESIAN_POINT('Ctrl Pts',(30.3373688833396,9.77553124130065,-64.7925772570577));
#53544=CARTESIAN_POINT('',(25.9580275654173,16.0437450369841,-76.6642789908813));
#53545=CARTESIAN_POINT('Ctrl Pts',(25.9580275654173,16.0437450369841,-76.6642789908813));
#53546=CARTESIAN_POINT('Ctrl Pts',(26.6559762479054,14.9591966918103,-74.6266658726109));
#53547=CARTESIAN_POINT('Ctrl Pts',(27.2836007288677,13.7527661001403,-72.3692972947473));
#53548=CARTESIAN_POINT('Ctrl Pts',(27.8093579489706,12.8426393697467,-70.6502216955679));
#53549=CARTESIAN_POINT('',(25.7066762097982,16.4237782457055,-77.3782777057259));
#53550=CARTESIAN_POINT('Ctrl Pts',(25.7066762161377,16.4237824971517,-77.3782754451113));
#53551=CARTESIAN_POINT('Ctrl Pts',(25.7493317432104,16.361108340562,-77.2605263204144));
#53552=CARTESIAN_POINT('Ctrl Pts',(25.7914521798399,16.2982559066625,-77.1424435089061));
#53553=CARTESIAN_POINT('Ctrl Pts',(25.8751675367156,16.1716233431714,-76.9045368904255));
#53554=CARTESIAN_POINT('Ctrl Pts',(25.9168664608344,16.1076591547755,-76.7843673153015));
#53555=CARTESIAN_POINT('Ctrl Pts',(25.9580275563336,16.0437394275245,-76.6642819734839));
#53556=CARTESIAN_POINT('',(20.8066780834701,16.2071460528291,-76.9702782129913));
#53557=CARTESIAN_POINT('Ctrl Pts',(20.8066780834701,16.2071460528291,-76.9702782129913));
#53558=CARTESIAN_POINT('Ctrl Pts',(20.7814199439412,16.2902997214971,-77.1267023814477));
#53559=CARTESIAN_POINT('Ctrl Pts',(20.7510970195006,16.462201386336,-77.4500437795191));
#53560=CARTESIAN_POINT('Ctrl Pts',(20.8055482815057,16.7173317962075,-77.9297992830641));
#53561=CARTESIAN_POINT('Ctrl Pts',(21.0009366844085,16.9521786769222,-78.3712110483715));
#53562=CARTESIAN_POINT('Ctrl Pts',(21.2717280412466,17.0949090521466,-78.6392688130115));
#53563=CARTESIAN_POINT('Ctrl Pts',(21.4878400853508,17.1684263103318,-78.777240406493));
#53564=CARTESIAN_POINT('Ctrl Pts',(21.6407851560214,17.2127260997074,-78.8603513323804));
#53565=CARTESIAN_POINT('Ctrl Pts',(21.9258991389736,17.2758277200359,-78.9786607564294));
#53566=CARTESIAN_POINT('Ctrl Pts',(22.3594194342618,17.3310653318226,-79.0820453922927));
#53567=CARTESIAN_POINT('Ctrl Pts',(22.9124146240747,17.3542009086611,-79.1251165545024));
#53568=CARTESIAN_POINT('Ctrl Pts',(23.5418771977656,17.3391957004687,-79.0966974225329));
#53569=CARTESIAN_POINT('Ctrl Pts',(24.2749365963644,17.2629716950359,-78.9536848243009));
#53570=CARTESIAN_POINT('Ctrl Pts',(24.9206297891638,17.1086649231884,-78.6644707327587));
#53571=CARTESIAN_POINT('Ctrl Pts',(25.3704424188049,16.8998240213439,-78.2726976801559));
#53572=CARTESIAN_POINT('Ctrl Pts',(25.6207437197086,16.674198124308,-77.8490131748246));
#53573=CARTESIAN_POINT('Ctrl Pts',(25.6912026729945,16.5078943516558,-77.5364389821151));
#53574=CARTESIAN_POINT('Ctrl Pts',(25.7066762066284,16.4237761199824,-77.3782788360332));
#53575=CARTESIAN_POINT('',(21.0403876071431,16.0446209665478,-76.6642753537542));
#53576=CARTESIAN_POINT('Ctrl Pts',(21.0403876071431,16.0446209665478,-76.6642753537542));
#53577=CARTESIAN_POINT('Ctrl Pts',(21.00240573693,16.0723625448958,-76.7165035747521));
#53578=CARTESIAN_POINT('Ctrl Pts',(20.9637701717481,16.0999221085431,-76.7683905060148));
#53579=CARTESIAN_POINT('Ctrl Pts',(20.8858789219625,16.1540987363042,-76.8703926297541));
#53580=CARTESIAN_POINT('Ctrl Pts',(20.8466178752764,16.1807440064858,-76.9205608786289));
#53581=CARTESIAN_POINT('Ctrl Pts',(20.8066780817163,16.2071484214984,-76.9702769535722));
#53582=CARTESIAN_POINT('',(23.6739538950181,12.8462304042226,-70.6468064576015));
#53583=CARTESIAN_POINT('Ctrl Pts',(23.6739538950114,12.8462304034107,-70.6468064580614));
#53584=CARTESIAN_POINT('Ctrl Pts',(23.6310070416931,12.9226146262459,-70.7905530926008));
#53585=CARTESIAN_POINT('Ctrl Pts',(23.5868595342126,12.9994632040654,-70.9351540957691));
#53586=CARTESIAN_POINT('Ctrl Pts',(23.4968949910939,13.1529431996464,-71.2239148776459));
#53587=CARTESIAN_POINT('Ctrl Pts',(23.4510453066928,13.2296432218887,-71.368204417614));
#53588=CARTESIAN_POINT('Ctrl Pts',(23.3130966014547,13.4560967906469,-71.7941829319882));
#53589=CARTESIAN_POINT('Ctrl Pts',(23.2147099938374,13.6120649244949,-72.0875323254961));
#53590=CARTESIAN_POINT('Ctrl Pts',(22.9103990595176,14.0734231098319,-72.9552509912363));
#53591=CARTESIAN_POINT('Ctrl Pts',(22.6919329352605,14.3771016959961,-73.5263966705118));
#53592=CARTESIAN_POINT('Ctrl Pts',(22.0400659372768,15.1823811459668,-75.0412727227511));
#53593=CARTESIAN_POINT('Ctrl Pts',(21.5785607485871,15.6515432869189,-75.9242400324668));
#53594=CARTESIAN_POINT('Ctrl Pts',(21.0403876071432,16.0446209665478,-76.6642753537542));
#53595=CARTESIAN_POINT('',(24.8344045918158,9.66888145222939,-64.6543282396439));
#53596=CARTESIAN_POINT('Ctrl Pts',(24.8344045929607,9.66888120903035,-64.6543283644958));
#53597=CARTESIAN_POINT('Ctrl Pts',(24.8303501358965,9.70941951662452,-64.73332914588));
#53598=CARTESIAN_POINT('Ctrl Pts',(24.8258802785889,9.74917832575716,-64.8106105339471));
#53599=CARTESIAN_POINT('Ctrl Pts',(24.8209763204938,9.78866534954903,-64.8871863689394));
#53600=CARTESIAN_POINT('Ctrl Pts',(24.8199646022781,9.79681177749121,-64.9029844580829));
#53601=CARTESIAN_POINT('Ctrl Pts',(24.8189342458198,9.80494663665857,-64.918752444668));
#53602=CARTESIAN_POINT('Ctrl Pts',(24.8178848358697,9.81307438905661,-64.9344991318275));
#53603=CARTESIAN_POINT('Ctrl Pts',(24.8155682503962,9.83101650322885,-64.9692601389317));
#53604=CARTESIAN_POINT('Ctrl Pts',(24.8131590265581,9.84892467935145,-65.0039180758427));
#53605=CARTESIAN_POINT('Ctrl Pts',(24.810645719863,9.8668831345148,-65.0386377886802));
#53606=CARTESIAN_POINT('Ctrl Pts',(24.8028781675356,9.92238501197181,-65.1459415199712));
#53607=CARTESIAN_POINT('Ctrl Pts',(24.7941090477931,9.97836864578574,-65.2538384783798));
#53608=CARTESIAN_POINT('Ctrl Pts',(24.7843654791308,10.0345257433411,-65.3617487507159));
#53609=CARTESIAN_POINT('Ctrl Pts',(24.7826546343078,10.0443862044268,-65.3806964009229));
#53610=CARTESIAN_POINT('Ctrl Pts',(24.7809138740523,10.0542519990379,-65.3996444807811));
#53611=CARTESIAN_POINT('Ctrl Pts',(24.7791435094063,10.0641214352372,-65.4185898648104));
#53612=CARTESIAN_POINT('Ctrl Pts',(24.7584167318918,10.1796691608203,-65.6403954462719));
#53613=CARTESIAN_POINT('Ctrl Pts',(24.7336388591999,10.2957131317301,-65.8618169276568));
#53614=CARTESIAN_POINT('Ctrl Pts',(24.7046949084052,10.4130044997939,-66.0845375417376));
#53615=CARTESIAN_POINT('Ctrl Pts',(24.7008996526852,10.4283842500809,-66.1137416296845));
#53616=CARTESIAN_POINT('Ctrl Pts',(24.6970326774042,10.4437854596428,-66.1429681011285));
#53617=CARTESIAN_POINT('Ctrl Pts',(24.6930936396352,10.4592098397787,-66.1722208064147));
#53618=CARTESIAN_POINT('Ctrl Pts',(24.6625714917577,10.5787276608925,-66.3988892084302));
#53619=CARTESIAN_POINT('Ctrl Pts',(24.6277268042723,10.6996122801159,-66.627083756415));
#53620=CARTESIAN_POINT('Ctrl Pts',(24.5885038182621,10.822311194009,-66.8579348550256));
#53621=CARTESIAN_POINT('Ctrl Pts',(24.5727743595823,10.8715167158845,-66.9505122741914));
#53622=CARTESIAN_POINT('Ctrl Pts',(24.5563411231441,10.9210138128591,-67.0435165697199));
#53623=CARTESIAN_POINT('Ctrl Pts',(24.539201945762,10.9708303881966,-67.137018880739));
#53624=CARTESIAN_POINT('Ctrl Pts',(24.5319183453243,10.9920008342364,-67.1767543626868));
#53625=CARTESIAN_POINT('Ctrl Pts',(24.5245072651196,11.0132289672869,-67.2165797658144));
#53626=CARTESIAN_POINT('Ctrl Pts',(24.5169724822948,11.0345099947928,-67.2564873906126));
#53627=CARTESIAN_POINT('Ctrl Pts',(24.4946558110608,11.0975405698481,-67.3746865959579));
#53628=CARTESIAN_POINT('Ctrl Pts',(24.4712375373057,11.1610700850315,-67.4937103111689));
#53629=CARTESIAN_POINT('Ctrl Pts',(24.4467384852227,11.2251548137537,-67.6136954338559));
#53630=CARTESIAN_POINT('Ctrl Pts',(24.400804523427,11.3453090740422,-67.8386589150087));
#53631=CARTESIAN_POINT('Ctrl Pts',(24.3512314195594,11.4670167961932,-68.0661686704969));
#53632=CARTESIAN_POINT('Ctrl Pts',(24.2986050952819,11.5895147520019,-68.2950168825741));
#53633=CARTESIAN_POINT('Ctrl Pts',(24.2194550792226,11.773751734208,-68.639204699408));
#53634=CARTESIAN_POINT('Ctrl Pts',(24.1333995603996,11.9597735798187,-68.986415264212));
#53635=CARTESIAN_POINT('Ctrl Pts',(24.0424408348367,12.1450384042839,-69.3326474110774));
#53636=CARTESIAN_POINT('Ctrl Pts',(23.9740416340358,12.2843539658368,-69.5930072829929));
#53637=CARTESIAN_POINT('Ctrl Pts',(23.9028690387089,12.423244236739,-69.8528192706222));
#53638=CARTESIAN_POINT('Ctrl Pts',(23.8297837772451,12.5606256545873,-70.1103770138851));
#53639=CARTESIAN_POINT('Ctrl Pts',(23.8169956343545,12.5846640607826,-70.1554433536292));
#53640=CARTESIAN_POINT('Ctrl Pts',(23.8041489695695,12.6086562304002,-70.200440596941));
#53641=CARTESIAN_POINT('Ctrl Pts',(23.7912484243222,12.6325963398636,-70.245359562372));
#53642=CARTESIAN_POINT('Ctrl Pts',(23.7525659360645,12.7043811354252,-70.3800497882137));
#53643=CARTESIAN_POINT('Ctrl Pts',(23.7133985611913,12.7756821419663,-70.5140424729259));
#53644=CARTESIAN_POINT('Ctrl Pts',(23.6739538950215,12.8462304046968,-70.6468064573353));
#53645=CARTESIAN_POINT('',(24.4986797976544,6.71047053280757,-58.7794556342451));
#53646=CARTESIAN_POINT('Ctrl Pts',(24.4986797976544,6.71047053280757,-58.7794556342451));
#53647=CARTESIAN_POINT('Ctrl Pts',(24.6381921878201,7.28402736458032,-60.1192331620747));
#53648=CARTESIAN_POINT('Ctrl Pts',(24.8491604058793,8.33135979595778,-62.1002014923607));
#53649=CARTESIAN_POINT('Ctrl Pts',(24.8726304141327,9.27135230412159,-63.8796298265301));
#53650=CARTESIAN_POINT('Ctrl Pts',(24.8344045906688,9.66888169588101,-64.6543281145597));
#53651=CARTESIAN_POINT('',(23.8104975525172,4.71983210132197,-53.1013215771875));
#53652=CARTESIAN_POINT('Ctrl Pts',(23.8104975547445,4.71983210069848,-53.1013215768221));
#53653=CARTESIAN_POINT('Ctrl Pts',(23.9337205829163,4.84404524606257,-53.6404826359787));
#53654=CARTESIAN_POINT('Ctrl Pts',(24.0199474940819,4.99885485594887,-54.1957970613934));
#53655=CARTESIAN_POINT('Ctrl Pts',(24.1600565300499,5.3462915437671,-55.3009470158922));
#53656=CARTESIAN_POINT('Ctrl Pts',(24.2146562929896,5.54550925178696,-55.8683918927849));
#53657=CARTESIAN_POINT('Ctrl Pts',(24.2888535333137,5.82844014520507,-56.6195254124793));
#53658=CARTESIAN_POINT('Ctrl Pts',(24.3080077308712,5.9038243509016,-56.8149835325362));
#53659=CARTESIAN_POINT('Ctrl Pts',(24.3413690767299,6.03831715020874,-57.1570027496823));
#53660=CARTESIAN_POINT('Ctrl Pts',(24.3556625645275,6.09700551911714,-57.304102153857));
#53661=CARTESIAN_POINT('Ctrl Pts',(24.3913918117882,6.24581854559107,-57.672515111601));
#53662=CARTESIAN_POINT('Ctrl Pts',(24.4128016567203,6.33691449783787,-57.8939185828946));
#53663=CARTESIAN_POINT('Ctrl Pts',(24.4449941284588,6.4753019929398,-58.2255323486235));
#53664=CARTESIAN_POINT('Ctrl Pts',(24.4557841965576,6.52189313240607,-58.3363874846924));
#53665=CARTESIAN_POINT('Ctrl Pts',(24.471911122741,6.59208959264157,-58.5024114063079));
#53666=CARTESIAN_POINT('Ctrl Pts',(24.4772911301109,6.61560292274562,-58.5578573126726));
#53667=CARTESIAN_POINT('Ctrl Pts',(24.4893061751536,6.66838686278425,-58.6819862965278));
#53668=CARTESIAN_POINT('Ctrl Pts',(24.4949961722313,6.69358513202795,-58.7410135943171));
#53669=CARTESIAN_POINT('Ctrl Pts',(24.4987083708446,6.71008931346543,-58.7796158705648));
#53670=CARTESIAN_POINT('',(18.0802312907388,4.08541520334038,-47.3815173795873));
#53671=CARTESIAN_POINT('Ctrl Pts',(18.0802313198441,4.08541519315892,-47.3815173754911));
#53672=CARTESIAN_POINT('Ctrl Pts',(18.0818954942396,4.08545546640632,-47.3820362045046));
#53673=CARTESIAN_POINT('Ctrl Pts',(18.0835590772247,4.08549575181441,-47.3825548949369));
#53674=CARTESIAN_POINT('Ctrl Pts',(18.0852220694125,4.08553604937883,-47.3830734479269));
#53675=CARTESIAN_POINT('Ctrl Pts',(18.1678282741835,4.0875377598395,-47.4088316534028));
#53676=CARTESIAN_POINT('Ctrl Pts',(18.248970713161,4.08957534677303,-47.4347714589022));
#53677=CARTESIAN_POINT('Ctrl Pts',(18.3287266556004,4.09163932528598,-47.4608648300448));
#53678=CARTESIAN_POINT('Ctrl Pts',(18.4252175502284,4.09413638227154,-47.4924332956463));
#53679=CARTESIAN_POINT('Ctrl Pts',(18.5196790922603,4.09667205963219,-47.5242270828985));
#53680=CARTESIAN_POINT('Ctrl Pts',(18.6122436622419,4.09923712348749,-47.5562764970958));
#53681=CARTESIAN_POINT('Ctrl Pts',(18.7731727968583,4.10369664300506,-47.6119963528975));
#53682=CARTESIAN_POINT('Ctrl Pts',(18.9283690860628,4.10824464966644,-47.6684960624441));
#53683=CARTESIAN_POINT('Ctrl Pts',(19.0785058320582,4.1128615144897,-47.7261539453444));
#53684=CARTESIAN_POINT('Ctrl Pts',(19.0996497598848,4.113511712787,-47.7342739702364));
#53685=CARTESIAN_POINT('Ctrl Pts',(19.1206933073599,4.11416329813255,-47.7424169078168));
#53686=CARTESIAN_POINT('Ctrl Pts',(19.1416383266119,4.11481622511397,-47.7505835985577));
#53687=CARTESIAN_POINT('Ctrl Pts',(19.2054083250036,4.11680415131512,-47.7754482142997));
#53688=CARTESIAN_POINT('Ctrl Pts',(19.2682650139487,4.11880450099507,-47.8005329842545));
#53689=CARTESIAN_POINT('Ctrl Pts',(19.3302603531123,4.12082313687603,-47.8259594010279));
#53690=CARTESIAN_POINT('Ctrl Pts',(19.476568492363,4.12558708951427,-47.8859653914153));
#53691=CARTESIAN_POINT('Ctrl Pts',(19.618073824103,4.13041529144838,-47.9473890021447));
#53692=CARTESIAN_POINT('Ctrl Pts',(19.7546645730943,4.1352530499461,-48.0100920493126));
#53693=CARTESIAN_POINT('Ctrl Pts',(19.7902338162518,4.13651283810608,-48.0264203874168));
#53694=CARTESIAN_POINT('Ctrl Pts',(19.8254696213882,4.13777331865906,-48.0428356976964));
#53695=CARTESIAN_POINT('Ctrl Pts',(19.8603696738727,4.13903362990627,-48.0593360018436));
#53696=CARTESIAN_POINT('Ctrl Pts',(19.907297533467,4.14072828951404,-48.0815229013225));
#53697=CARTESIAN_POINT('Ctrl Pts',(19.9536183372731,4.14242260338841,-48.1038634250931));
#53698=CARTESIAN_POINT('Ctrl Pts',(19.9993252666987,4.14411462066421,-48.1263504155863));
#53699=CARTESIAN_POINT('Ctrl Pts',(20.1283290996858,4.14889019226356,-48.1898179904686));
#53700=CARTESIAN_POINT('Ctrl Pts',(20.2524434881266,4.15364525445708,-48.2544528349789));
#53701=CARTESIAN_POINT('Ctrl Pts',(20.3715073556093,4.15834181382186,-48.319863761312));
#53702=CARTESIAN_POINT('Ctrl Pts',(20.5478383713987,4.1652973167886,-48.4167359302404));
#53703=CARTESIAN_POINT('Ctrl Pts',(20.7131238675307,4.17214241143718,-48.5155240818662));
#53704=CARTESIAN_POINT('Ctrl Pts',(20.8716066057245,4.17909356110718,-48.6185955718901));
#53705=CARTESIAN_POINT('Ctrl Pts',(20.9945301288674,4.18448506189186,-48.6985406235325));
#53706=CARTESIAN_POINT('Ctrl Pts',(21.1133631600208,4.18994138765124,-48.7810661753323));
#53707=CARTESIAN_POINT('Ctrl Pts',(21.2300788101569,4.19557937729348,-48.8672621022061));
#53708=CARTESIAN_POINT('Ctrl Pts',(21.2355169545766,4.19584206873096,-48.8712782379872));
#53709=CARTESIAN_POINT('Ctrl Pts',(21.2409504287901,4.19610515370641,-48.8753022806401));
#53710=CARTESIAN_POINT('Ctrl Pts',(21.2463793779124,4.19636866023458,-48.8793345271448));
#53711=CARTESIAN_POINT('Ctrl Pts',(21.3426159920706,4.20103972557494,-48.9508124029394));
#53712=CARTESIAN_POINT('Ctrl Pts',(21.4374324925893,4.20584148619805,-49.0248706969702));
#53713=CARTESIAN_POINT('Ctrl Pts',(21.5316270036835,4.21094199052955,-49.1031856542045));
#53714=CARTESIAN_POINT('Ctrl Pts',(21.6124142391004,4.21531650916537,-49.1703535689083));
#53715=CARTESIAN_POINT('Ctrl Pts',(21.6927443752873,4.21991037614473,-49.2406526714573));
#53716=CARTESIAN_POINT('Ctrl Pts',(21.7731004780744,4.22484894017138,-49.3151172586566));
#53717=CARTESIAN_POINT('Ctrl Pts',(21.8478383719207,4.22944221760988,-49.3843755504401));
#53718=CARTESIAN_POINT('Ctrl Pts',(21.9225992369863,4.23433303916604,-49.457237390789));
#53719=CARTESIAN_POINT('Ctrl Pts',(21.9977460885454,4.2396476973278,-49.5345114605038));
#53720=CARTESIAN_POINT('Ctrl Pts',(22.0033950397209,4.24004721166336,-49.5403203192636));
#53721=CARTESIAN_POINT('Ctrl Pts',(22.0090461570274,4.24044913664175,-49.5461540984415));
#53722=CARTESIAN_POINT('Ctrl Pts',(22.0146995869572,4.24085353401629,-49.5520131353011));
#53723=CARTESIAN_POINT('Ctrl Pts',(22.0940464373028,4.24652931992959,-49.6342457138667));
#53724=CARTESIAN_POINT('Ctrl Pts',(22.1738759302386,4.25269005891086,-49.721482999791));
#53725=CARTESIAN_POINT('Ctrl Pts',(22.2532325274327,4.25945526922204,-49.8134791920094));
#53726=CARTESIAN_POINT('Ctrl Pts',(22.3314807570317,4.26612599035213,-49.9041904803643));
#53727=CARTESIAN_POINT('Ctrl Pts',(22.4092680991043,4.27338434916336,-49.9995279779554));
#53728=CARTESIAN_POINT('Ctrl Pts',(22.4856729607389,4.28139444099833,-50.0992589162882));
#53729=CARTESIAN_POINT('Ctrl Pts',(22.5459313021454,4.28771177262047,-50.1779138709897));
#53730=CARTESIAN_POINT('Ctrl Pts',(22.6053293198368,4.29449772547797,-50.2593015052972));
#53731=CARTESIAN_POINT('Ctrl Pts',(22.663420454943,4.30185445637358,-50.3433131260172));
#53732=CARTESIAN_POINT('Ctrl Pts',(22.6811953577698,4.30410549134739,-50.3690192581471));
#53733=CARTESIAN_POINT('Ctrl Pts',(22.6988479689518,4.30641009737276,-50.3949711131632));
#53734=CARTESIAN_POINT('Ctrl Pts',(22.7163656995239,4.3087714756635,-50.4211654372162));
#53735=CARTESIAN_POINT('Ctrl Pts',(22.7378417722252,4.31166643580909,-50.4532786841583));
#53736=CARTESIAN_POINT('Ctrl Pts',(22.7591151053141,4.31464672184621,-50.4857563551764));
#53737=CARTESIAN_POINT('Ctrl Pts',(22.7801631127034,4.3177186863129,-50.5185925879126));
#53738=CARTESIAN_POINT('Ctrl Pts',(22.8488611872628,4.32774519571459,-50.6257659617633));
#53739=CARTESIAN_POINT('Ctrl Pts',(22.9151916406563,4.33874940122539,-50.7367729700415));
#53740=CARTESIAN_POINT('Ctrl Pts',(22.9788702095239,4.35089642274516,-50.8509037331451));
#53741=CARTESIAN_POINT('Ctrl Pts',(23.039777833928,4.36251487205255,-50.9600681471023));
#53742=CARTESIAN_POINT('Ctrl Pts',(23.098259047567,4.37517975057679,-51.0720902612061));
#53743=CARTESIAN_POINT('Ctrl Pts',(23.1541059170705,4.38902878270128,-51.1863693014867));
#53744=CARTESIAN_POINT('Ctrl Pts',(23.2079534667054,4.40238201899452,-51.2965571481546));
#53745=CARTESIAN_POINT('Ctrl Pts',(23.2593519356011,4.41683676555948,-51.4088432548648));
#53746=CARTESIAN_POINT('Ctrl Pts',(23.3081556564332,4.43249913743182,-51.5227089775153));
#53747=CARTESIAN_POINT('Ctrl Pts',(23.3388595793072,4.44235281763886,-51.5943454082353));
#53748=CARTESIAN_POINT('Ctrl Pts',(23.3685373195835,4.45268409619484,-51.6666074631411));
#53749=CARTESIAN_POINT('Ctrl Pts',(23.3971609632618,4.46351416843441,-51.7393700251083));
#53750=CARTESIAN_POINT('Ctrl Pts',(23.3979634190634,4.46381778646427,-51.7414099030724));
#53751=CARTESIAN_POINT('Ctrl Pts',(23.3987650360467,4.46412179584896,-51.7434501719335));
#53752=CARTESIAN_POINT('Ctrl Pts',(23.3995658157371,4.46442619750041,-51.7454908323607));
#53753=CARTESIAN_POINT('Ctrl Pts',(23.456663235734,4.4861307301565,-51.8909945793684));
#53754=CARTESIAN_POINT('Ctrl Pts',(23.5095017668692,4.5098262849802,-52.0384892149187));
#53755=CARTESIAN_POINT('Ctrl Pts',(23.5586490724152,4.53585951374875,-52.1882628922863));
#53756=CARTESIAN_POINT('Ctrl Pts',(23.6069335827223,4.5614357216169,-52.3354072491998));
#53757=CARTESIAN_POINT('Ctrl Pts',(23.6516553829564,4.58926716144762,-52.4847514954688));
#53758=CARTESIAN_POINT('Ctrl Pts',(23.6933757118896,4.61973038249599,-52.6365651937523));
#53759=CARTESIAN_POINT('Ctrl Pts',(23.7308930784603,4.64712469745508,-52.7730849747459));
#53760=CARTESIAN_POINT('Ctrl Pts',(23.7659833400795,4.67664726218901,-52.9116016648842));
#53761=CARTESIAN_POINT('Ctrl Pts',(23.7990721375966,4.70861665137786,-53.0523078155129));
#53762=CARTESIAN_POINT('Ctrl Pts',(23.8027789801418,4.71219808983686,-53.068070719718));
#53763=CARTESIAN_POINT('Ctrl Pts',(23.8064607237595,4.71581028662781,-53.0838610985039));
#53764=CARTESIAN_POINT('Ctrl Pts',(23.8101179823112,4.7194537290064,-53.0996792201637));
#53765=CARTESIAN_POINT('Ctrl Pts',(23.8102445371179,4.71957980572192,-53.100226586258));
#53766=CARTESIAN_POINT('Ctrl Pts',(23.8103710590392,4.71970592969668,-53.1007740390327));
#53767=CARTESIAN_POINT('Ctrl Pts',(23.810497548099,4.71983210089637,-53.1013215783063));
#53768=CARTESIAN_POINT('',(1.31624832366244E-14,4.0543744617278,-45.4831027428904));
#53769=CARTESIAN_POINT('Ctrl Pts',(3.43297346105942E-9,4.05427777602882,
-45.4831012288709));
#53770=CARTESIAN_POINT('Ctrl Pts',(6.05186862449095E-5,4.05427775975267,
-45.4831024054858));
#53771=CARTESIAN_POINT('Ctrl Pts',(0.000121034596136508,4.05427774347302,
-45.4831035821241));
#53772=CARTESIAN_POINT('Ctrl Pts',(0.000181551162595994,4.05427772718987,
-45.483104758786));
#53773=CARTESIAN_POINT('Ctrl Pts',(0.404036195742715,4.05416906235028,-45.4909571599143));
#53774=CARTESIAN_POINT('Ctrl Pts',(0.83713307952267,4.0539012467317,-45.4998582098889));
#53775=CARTESIAN_POINT('Ctrl Pts',(1.28696595037213,4.05344844944743,-45.5098531479376));
#53776=CARTESIAN_POINT('Ctrl Pts',(1.48640695053461,4.05324769412451,-45.5142845725181));
#53777=CARTESIAN_POINT('Ctrl Pts',(1.68913754270891,4.05301114478449,-45.5189306432058));
#53778=CARTESIAN_POINT('Ctrl Pts',(1.89406691812013,4.05273924500278,-45.5237937603419));
#53779=CARTESIAN_POINT('Ctrl Pts',(2.40207554685425,4.05206522042732,-45.5358491597334));
#53780=CARTESIAN_POINT('Ctrl Pts',(2.92359528397998,4.0511695350036,-45.5492383085822));
#53781=CARTESIAN_POINT('Ctrl Pts',(3.44183098945343,4.05031895343455,-45.5640819003926));
#53782=CARTESIAN_POINT('Ctrl Pts',(3.55707650285137,4.05012980068306,-45.5673828257067));
#53783=CARTESIAN_POINT('Ctrl Pts',(3.67215975304471,4.04994301706739,-45.5707556451171));
#53784=CARTESIAN_POINT('Ctrl Pts',(3.7868964873834,4.04976156559607,-45.5742015989867));
#53785=CARTESIAN_POINT('Ctrl Pts',(4.22095109987234,4.04907512590854,-45.5872378090565));
#53786=CARTESIAN_POINT('Ctrl Pts',(4.65004621640487,4.04846758781903,-45.6013200772451));
#53787=CARTESIAN_POINT('Ctrl Pts',(5.06447649274192,4.04800401280653,-45.616441724763));
#53788=CARTESIAN_POINT('Ctrl Pts',(5.44484785101927,4.04757853554959,-45.6303206374153));
#53789=CARTESIAN_POINT('Ctrl Pts',(5.81286752503525,4.04727488700343,-45.6450742828859));
#53790=CARTESIAN_POINT('Ctrl Pts',(6.16101928401631,4.04710852121872,-45.6607119137277));
#53791=CARTESIAN_POINT('Ctrl Pts',(6.19219321962801,4.04709362462226,-45.6621121263776));
#53792=CARTESIAN_POINT('Ctrl Pts',(6.2232078440126,4.04707980157761,-45.6635194407835));
#53793=CARTESIAN_POINT('Ctrl Pts',(6.25405774996299,4.04706704679936,-45.6649338724781));
#53794=CARTESIAN_POINT('Ctrl Pts',(6.39369015341136,4.04700931630432,-45.671335853001));
#53795=CARTESIAN_POINT('Ctrl Pts',(6.52992501973367,4.04697334440262,-45.6778867910422));
#53796=CARTESIAN_POINT('Ctrl Pts',(6.66370228859331,4.04695855294085,-45.6846379325746));
#53797=CARTESIAN_POINT('Ctrl Pts',(6.97370603308844,4.04692427650082,-45.7002824375976));
#53798=CARTESIAN_POINT('Ctrl Pts',(7.27051360118711,4.04700094253711,-45.7170033860239));
#53799=CARTESIAN_POINT('Ctrl Pts',(7.56580390759954,4.04720606586608,-45.7354275474617));
#53800=CARTESIAN_POINT('Ctrl Pts',(7.57251673859061,4.04721072893226,-45.7358463837025));
#53801=CARTESIAN_POINT('Ctrl Pts',(7.57922878490261,4.04721546021916,-45.736266099256));
#53802=CARTESIAN_POINT('Ctrl Pts',(7.58594018431063,4.04722025876168,-45.7366867010865));
#53803=CARTESIAN_POINT('Ctrl Pts',(7.95978215304528,4.04748754975046,-45.7601152897915));
#53804=CARTESIAN_POINT('Ctrl Pts',(8.33161933763295,4.04795972550633,-45.7862993479164));
#53805=CARTESIAN_POINT('Ctrl Pts',(8.70240386159958,4.04846734504311,-45.8158868079574));
#53806=CARTESIAN_POINT('Ctrl Pts',(8.75744748111489,4.04854270206272,-45.8202791188217));
#53807=CARTESIAN_POINT('Ctrl Pts',(8.81246786886126,4.04861892343029,-45.8247464065533));
#53808=CARTESIAN_POINT('Ctrl Pts',(8.86746810593587,4.04869554438674,-45.8292907621443));
#53809=CARTESIAN_POINT('Ctrl Pts',(9.21325287644122,4.04917725794381,-45.8578609836323));
#53810=CARTESIAN_POINT('Ctrl Pts',(9.55824383302655,4.04967203846346,-45.8894772374749));
#53811=CARTESIAN_POINT('Ctrl Pts',(9.90713893817511,4.05009215387646,-45.9248188740961));
#53812=CARTESIAN_POINT('Ctrl Pts',(9.98756366758387,4.05018899578657,-45.9329655678163));
#53813=CARTESIAN_POINT('Ctrl Pts',(10.0681959253425,4.0502820013443,-45.9413100595536));
#53814=CARTESIAN_POINT('Ctrl Pts',(10.1490934332731,4.05037031202927,-45.9498603773688));
#53815=CARTESIAN_POINT('Ctrl Pts',(10.4017415872042,4.05064611201496,-45.9765635733855));
#53816=CARTESIAN_POINT('Ctrl Pts',(10.6569707728277,4.05087496421816,-46.0052806388128));
#53817=CARTESIAN_POINT('Ctrl Pts',(10.9122399706433,4.05103425693971,-46.0356784115238));
#53818=CARTESIAN_POINT('Ctrl Pts',(11.0578538286592,4.05112512269216,-46.0530182903554));
#53819=CARTESIAN_POINT('Ctrl Pts',(11.2034804477291,4.05119360068566,-46.07090537708));
#53820=CARTESIAN_POINT('Ctrl Pts',(11.3486452763677,4.05123805153778,-46.0892809134502));
#53821=CARTESIAN_POINT('Ctrl Pts',(11.383976601352,4.05124887032575,-46.0937532918724));
#53822=CARTESIAN_POINT('Ctrl Pts',(11.4192805580855,4.05125827662745,-46.0982546159133));
#53823=CARTESIAN_POINT('Ctrl Pts',(11.4545498895211,4.05126637489147,-46.1027841806848));
#53824=CARTESIAN_POINT('Ctrl Pts',(11.7742497637354,4.05133978183977,-46.1438425514774));
#53825=CARTESIAN_POINT('Ctrl Pts',(12.0911755578599,4.05130574615934,-46.1872009234999));
#53826=CARTESIAN_POINT('Ctrl Pts',(12.4042033751243,4.05124265326174,-46.2324848587249));
#53827=CARTESIAN_POINT('Ctrl Pts',(12.694496373003,4.05118414272248,-46.2744798782957));
#53828=CARTESIAN_POINT('Ctrl Pts',(12.9814371435597,4.05110083046585,-46.3181318940072));
#53829=CARTESIAN_POINT('Ctrl Pts',(13.2641790028529,4.05105226727443,-46.3631417277007));
#53830=CARTESIAN_POINT('Ctrl Pts',(13.2863224412092,4.05104846396055,-46.3666667539572));
#53831=CARTESIAN_POINT('Ctrl Pts',(13.3084401516756,4.05104487157467,-46.3702001039138));
#53832=CARTESIAN_POINT('Ctrl Pts',(13.3305317410286,4.05104151756354,-46.3737416311182));
#53833=CARTESIAN_POINT('Ctrl Pts',(13.5484374371254,4.05100843446944,-46.4086743350719));
#53834=CARTESIAN_POINT('Ctrl Pts',(13.7638001579389,4.05099865212725,-46.4444031545213));
#53835=CARTESIAN_POINT('Ctrl Pts',(13.9762533895905,4.05103765329587,-46.4807836800727));
#53836=CARTESIAN_POINT('Ctrl Pts',(14.0502765809521,4.05105124212643,-46.4934594232647));
#53837=CARTESIAN_POINT('Ctrl Pts',(14.123945972003,4.05107078300246,-46.506215870132));
#53838=CARTESIAN_POINT('Ctrl Pts',(14.1972362791489,4.05109736515344,-46.5190461735337));
#53839=CARTESIAN_POINT('Ctrl Pts',(14.4152033436357,4.05117642108377,-46.5572037918853));
#53840=CARTESIAN_POINT('Ctrl Pts',(14.6298152039408,4.05132110559856,-46.5960153776103));
#53841=CARTESIAN_POINT('Ctrl Pts',(14.8403666086119,4.05164841295011,-46.63537629821));
#53842=CARTESIAN_POINT('Ctrl Pts',(14.9669073543126,4.05184512366027,-46.6590320902573));
#53843=CARTESIAN_POINT('Ctrl Pts',(15.0919820464878,4.05210702155462,-46.6828861270287));
#53844=CARTESIAN_POINT('Ctrl Pts',(15.2154428418291,4.05245235788283,-46.7069136265541));
#53845=CARTESIAN_POINT('Ctrl Pts',(15.4204518451068,4.05302579543639,-46.7468117473734));
#53846=CARTESIAN_POINT('Ctrl Pts',(15.6210091637685,4.05383142766662,-46.7871891841816));
#53847=CARTESIAN_POINT('Ctrl Pts',(15.8164619842098,4.05491944656549,-46.8279226001094));
#53848=CARTESIAN_POINT('Ctrl Pts',(15.9582682497402,4.05570883346984,-46.8574757863053));
#53849=CARTESIAN_POINT('Ctrl Pts',(16.0973882435089,4.05664596943625,-46.8872160234026));
#53850=CARTESIAN_POINT('Ctrl Pts',(16.2335823643503,4.0577373193662,-46.9170900353023));
#53851=CARTESIAN_POINT('Ctrl Pts',(16.4490700936387,4.05946406437406,-46.9643570021083));
#53852=CARTESIAN_POINT('Ctrl Pts',(16.6572464582291,4.06157688937563,-47.011941479225));
#53853=CARTESIAN_POINT('Ctrl Pts',(16.8582463821327,4.06407456508433,-47.0599168052684));
#53854=CARTESIAN_POINT('Ctrl Pts',(16.9176596804606,4.06481284970218,-47.0740977676451));
#53855=CARTESIAN_POINT('Ctrl Pts',(16.976446152718,4.06558452834257,-47.088312692545));
#53856=CARTESIAN_POINT('Ctrl Pts',(17.0346097395913,4.06638904300838,-47.1025630232352));
#53857=CARTESIAN_POINT('Ctrl Pts',(17.2060465166445,4.06876034451871,-47.1445657761052));
#53858=CARTESIAN_POINT('Ctrl Pts',(17.372076387095,4.07141599648714,-47.1868760786687));
#53859=CARTESIAN_POINT('Ctrl Pts',(17.5328887073449,4.07430357677168,-47.2294920695148));
#53860=CARTESIAN_POINT('Ctrl Pts',(17.70411692991,4.07737818721738,-47.2748683214965));
#53861=CARTESIAN_POINT('Ctrl Pts',(17.8694294628641,4.0807156401366,-47.3205910960604));
#53862=CARTESIAN_POINT('Ctrl Pts',(18.0289977932907,4.08426414519071,-47.3666573201107));
#53863=CARTESIAN_POINT('Ctrl Pts',(18.0461419230271,4.08464539898246,-47.3716067064925));
#53864=CARTESIAN_POINT('Ctrl Pts',(18.0632196968548,4.08502910018635,-47.3765600571397));
#53865=CARTESIAN_POINT('Ctrl Pts',(18.0802312943422,4.08541519258013,-47.3815173680596));
#53866=CARTESIAN_POINT('',(-18.0802309774523,4.08571015955263,-47.3814955774373));
#53867=CARTESIAN_POINT('Ctrl Pts',(-18.0802309774513,4.0857101605419,-47.3814955773641));
#53868=CARTESIAN_POINT('Ctrl Pts',(-17.5067139301086,4.0727934681898,-47.2143630626668));
#53869=CARTESIAN_POINT('Ctrl Pts',(-16.1440950398105,4.05188108130506,-46.8717506694211));
#53870=CARTESIAN_POINT('Ctrl Pts',(-14.1201831359268,4.05068380667564,-46.4964790979153));
#53871=CARTESIAN_POINT('Ctrl Pts',(-12.8049882654227,4.05125213987811,-46.2906560258708));
#53872=CARTESIAN_POINT('Ctrl Pts',(-11.4702101265463,4.0515968823569,-46.0956364270593));
#53873=CARTESIAN_POINT('Ctrl Pts',(-9.97768282702567,4.05009813281506,-45.9211073625856));
#53874=CARTESIAN_POINT('Ctrl Pts',(-8.13525028131847,4.04739085834718,-45.7662068083777));
#53875=CARTESIAN_POINT('Ctrl Pts',(-6.8682519065081,4.04686778354698,-45.692032173767));
#53876=CARTESIAN_POINT('Ctrl Pts',(-5.13414802380493,4.04767124663689,-45.6143613687216));
#53877=CARTESIAN_POINT('Ctrl Pts',(-2.82998160019649,4.05178951295812,-45.5424604326639));
#53878=CARTESIAN_POINT('Ctrl Pts',(-0.829721113891657,4.05412214869547,
-45.4992347614638));
#53879=CARTESIAN_POINT('Ctrl Pts',(1.31624832385343E-14,4.0543744617278,
-45.4831027428904));
#53880=CARTESIAN_POINT('',(-23.8104968601155,4.71986549956444,-53.1013140443576));
#53881=CARTESIAN_POINT('Ctrl Pts',(-23.8104968601155,4.71986549956443,-53.1013140443576));
#53882=CARTESIAN_POINT('Ctrl Pts',(-23.7477724747327,4.65732912739002,-52.8297917254588));
#53883=CARTESIAN_POINT('Ctrl Pts',(-23.5151124729736,4.47941158193885,-51.9618739110486));
#53884=CARTESIAN_POINT('Ctrl Pts',(-22.9893961882904,4.32328459465657,-50.7078659748253));
#53885=CARTESIAN_POINT('Ctrl Pts',(-21.9700525412669,4.23238141610583,-49.4407645829627));
#53886=CARTESIAN_POINT('Ctrl Pts',(-20.9139224437741,4.17982285241228,-48.6001017036111));
#53887=CARTESIAN_POINT('Ctrl Pts',(-19.7542941715404,4.1339665963394,-47.9759241951474));
#53888=CARTESIAN_POINT('Ctrl Pts',(-18.7286389805631,4.10128995312838,-47.5836512241988));
#53889=CARTESIAN_POINT('Ctrl Pts',(-18.0802309774513,4.0857101605419,-47.3814955773641));
#53890=CARTESIAN_POINT('',(-24.4986968589845,6.71024380605157,-58.7795509549468));
#53891=CARTESIAN_POINT('Ctrl Pts',(-24.4986797976549,6.71047053280741,-58.7794556342435));
#53892=CARTESIAN_POINT('Ctrl Pts',(-24.4252551199817,6.38406893036685,-58.0159461404066));
#53893=CARTESIAN_POINT('Ctrl Pts',(-24.2995445048026,5.84530779207223,-56.7153263194681));
#53894=CARTESIAN_POINT('Ctrl Pts',(-24.1427524316995,5.29535697555521,-55.1551273288394));
#53895=CARTESIAN_POINT('Ctrl Pts',(-24.0157643032102,4.99438929412664,-54.1765791490832));
#53896=CARTESIAN_POINT('Ctrl Pts',(-23.8948201762871,4.80482491391012,-53.4702756145878));
#53897=CARTESIAN_POINT('Ctrl Pts',(-23.8104968601155,4.71986549956443,-53.1013140443576));
#53898=CARTESIAN_POINT('',(-24.8344040968691,9.66898708497287,-64.6542740052741));
#53899=CARTESIAN_POINT('Ctrl Pts',(-24.8344040968691,9.66898708497287,-64.6542740052741));
#53900=CARTESIAN_POINT('Ctrl Pts',(-24.8344224440182,9.66879626623666,-64.653902178655));
#53901=CARTESIAN_POINT('Ctrl Pts',(-24.8344407806158,9.66860542911226,-64.6535303121725));
#53902=CARTESIAN_POINT('Ctrl Pts',(-24.8344591066652,9.668414573522,-64.6531584056758));
#53903=CARTESIAN_POINT('Ctrl Pts',(-24.8406922382788,9.60349998185404,-64.5266640318661));
#53904=CARTESIAN_POINT('Ctrl Pts',(-24.845543748124,9.53913720233528,-64.4020695812121));
#53905=CARTESIAN_POINT('Ctrl Pts',(-24.8491870326249,9.47559685187425,-64.2796392143731));
#53906=CARTESIAN_POINT('Ctrl Pts',(-24.8501169863959,9.45937808320314,-64.248388681701));
#53907=CARTESIAN_POINT('Ctrl Pts',(-24.8509682174295,9.44321271503155,-64.2172790189038));
#53908=CARTESIAN_POINT('Ctrl Pts',(-24.8517436631487,9.42710337089091,-64.1863110121561));
#53909=CARTESIAN_POINT('Ctrl Pts',(-24.8525260595257,9.41084963168299,-64.155065425677));
#53910=CARTESIAN_POINT('Ctrl Pts',(-24.8532313056664,9.39465292971663,-64.1239640567786));
#53911=CARTESIAN_POINT('Ctrl Pts',(-24.853862327618,9.37851683625275,-64.0930100676953));
#53912=CARTESIAN_POINT('Ctrl Pts',(-24.8551422263563,9.34578807679707,-64.0302262430248));
#53913=CARTESIAN_POINT('Ctrl Pts',(-24.8561167908272,9.31330875463947,-63.9680487208868));
#53914=CARTESIAN_POINT('Ctrl Pts',(-24.8568104559153,9.28110504994544,-63.9064976883872));
#53915=CARTESIAN_POINT('Ctrl Pts',(-24.8582409926514,9.21469175715154,-63.7795617727215));
#53916=CARTESIAN_POINT('Ctrl Pts',(-24.8584773379802,9.14945187681934,-63.6552897653036));
#53917=CARTESIAN_POINT('Ctrl Pts',(-24.8577256710445,9.08557210499735,-63.5338319601283));
#53918=CARTESIAN_POINT('Ctrl Pts',(-24.8573369025111,9.05253294360197,-63.4710129500809));
#53919=CARTESIAN_POINT('Ctrl Pts',(-24.8566837216044,9.01985732795747,-63.4089469492897));
#53920=CARTESIAN_POINT('Ctrl Pts',(-24.8557940882076,8.98757346065118,-63.3476620540359));
#53921=CARTESIAN_POINT('Ctrl Pts',(-24.8548818089494,8.95446779867432,-63.2848171350145));
#53922=CARTESIAN_POINT('Ctrl Pts',(-24.8537208873905,8.9217740456132,-63.2227935470531));
#53923=CARTESIAN_POINT('Ctrl Pts',(-24.8523401728298,8.88951735436266,-63.161617164268));
#53924=CARTESIAN_POINT('Ctrl Pts',(-24.8491493068904,8.81497133278947,-63.0202370110637));
#53925=CARTESIAN_POINT('Ctrl Pts',(-24.8447863435392,8.74276273534532,-62.8833818467826));
#53926=CARTESIAN_POINT('Ctrl Pts',(-24.8395922216543,8.67316848592726,-62.7513690700857));
#53927=CARTESIAN_POINT('Ctrl Pts',(-24.8350852872875,8.61278162528261,-62.6368217157227));
#53928=CARTESIAN_POINT('Ctrl Pts',(-24.8299522037595,8.55436225020739,-62.525920199597));
#53929=CARTESIAN_POINT('Ctrl Pts',(-24.8243995161682,8.49806401214277,-62.4188696888623));
#53930=CARTESIAN_POINT('Ctrl Pts',(-24.8179231259384,8.43240042978602,-62.2940110739286));
#53931=CARTESIAN_POINT('Ctrl Pts',(-24.8108764077816,8.36962333665799,-62.1743920867275));
#53932=CARTESIAN_POINT('Ctrl Pts',(-24.8035602182169,8.30994192047519,-62.0603472077105));
#53933=CARTESIAN_POINT('Ctrl Pts',(-24.795963710439,8.24797382380193,-61.9419327239393));
#53934=CARTESIAN_POINT('Ctrl Pts',(-24.7880766366637,8.18934299086503,-61.8295276615945));
#53935=CARTESIAN_POINT('Ctrl Pts',(-24.7802072266692,8.13423747464485,-61.723492436022));
#53936=CARTESIAN_POINT('Ctrl Pts',(-24.7790968967969,8.12646239356123,-61.7085314569205));
#53937=CARTESIAN_POINT('Ctrl Pts',(-24.7779868750224,8.11875742404929,-61.6936972647197));
#53938=CARTESIAN_POINT('Ctrl Pts',(-24.7768779853736,8.11112302824542,-61.6789908511765));
#53939=CARTESIAN_POINT('Ctrl Pts',(-24.7726019398298,8.08168364787585,-61.6222807049786));
#53940=CARTESIAN_POINT('Ctrl Pts',(-24.7683428924224,8.05329390958756,-61.567470659123));
#53941=CARTESIAN_POINT('Ctrl Pts',(-24.7641470319276,8.02597767604251,-61.514616177431));
#53942=CARTESIAN_POINT('Ctrl Pts',(-24.7535979342429,7.95730007906331,-61.3817311372514));
#53943=CARTESIAN_POINT('Ctrl Pts',(-24.7437087555778,7.89555086323448,-61.2614546023172));
#53944=CARTESIAN_POINT('Ctrl Pts',(-24.734591378146,7.84043481895105,-61.1535048428839));
#53945=CARTESIAN_POINT('Ctrl Pts',(-24.7236433235866,7.77425203070551,-61.023879864121));
#53946=CARTESIAN_POINT('Ctrl Pts',(-24.7138064905812,7.71762815366309,-60.9120270608297));
#53947=CARTESIAN_POINT('Ctrl Pts',(-24.7052248674143,7.67001622988454,-60.8174730315066));
#53948=CARTESIAN_POINT('Ctrl Pts',(-24.7014023754499,7.64880856409547,-60.7753560554688));
#53949=CARTESIAN_POINT('Ctrl Pts',(-24.6978285223653,7.62938908047058,-60.7366716068643));
#53950=CARTESIAN_POINT('Ctrl Pts',(-24.6945151438418,7.61171250297287,-60.7013800383922));
#53951=CARTESIAN_POINT('Ctrl Pts',(-24.6911719711583,7.59387697630155,-60.6657711253638));
#53952=CARTESIAN_POINT('Ctrl Pts',(-24.688096864724,7.57781359951931,-60.6336175901605));
#53953=CARTESIAN_POINT('Ctrl Pts',(-24.68499470864,7.56169084505966,-60.6012688132271));
#53954=CARTESIAN_POINT('Ctrl Pts',(-24.684165593198,7.5573817051171,-60.5926229328271));
#53955=CARTESIAN_POINT('Ctrl Pts',(-24.6833346094936,7.55306858444141,-60.5839632025695));
#53956=CARTESIAN_POINT('Ctrl Pts',(-24.6824962645542,7.54871708623057,-60.5752201349814));
#53957=CARTESIAN_POINT('Ctrl Pts',(-24.6785212311363,7.52808434904397,-60.5337646621742));
#53958=CARTESIAN_POINT('Ctrl Pts',(-24.6743778519337,7.50658795121024,-60.4904274495276));
#53959=CARTESIAN_POINT('Ctrl Pts',(-24.670260456794,7.48553430446318,-60.4478289601855));
#53960=CARTESIAN_POINT('Ctrl Pts',(-24.6632384283214,7.44962827604104,-60.3751791913624));
#53961=CARTESIAN_POINT('Ctrl Pts',(-24.6562928707284,7.41500093872425,-60.3046841856839));
#53962=CARTESIAN_POINT('Ctrl Pts',(-24.6493275032303,7.38086146759743,-60.2347361217812));
#53963=CARTESIAN_POINT('Ctrl Pts',(-24.648618581765,7.3773868190735,-60.2276169448002));
#53964=CARTESIAN_POINT('Ctrl Pts',(-24.6479094647092,7.37391726536273,-60.2205034482435));
#53965=CARTESIAN_POINT('Ctrl Pts',(-24.6472000572969,7.37045200118949,-60.2133939471382));
#53966=CARTESIAN_POINT('Ctrl Pts',(-24.6467056641082,7.36803702359793,-60.2084392640324));
#53967=CARTESIAN_POINT('Ctrl Pts',(-24.6462111299257,7.3656241294789,-60.2034865214929));
#53968=CARTESIAN_POINT('Ctrl Pts',(-24.6457164231681,7.36321304982242,-60.1985351552348));
#53969=CARTESIAN_POINT('Ctrl Pts',(-24.633104532769,7.30174578279113,-60.0723066620617));
#53970=CARTESIAN_POINT('Ctrl Pts',(-24.6203743116398,7.2414509890623,-59.9469538919258));
#53971=CARTESIAN_POINT('Ctrl Pts',(-24.6076554397387,7.18271338071539,-59.8231292097387));
#53972=CARTESIAN_POINT('Ctrl Pts',(-24.6038772972698,7.16526536690217,-59.7863470726034));
#53973=CARTESIAN_POINT('Ctrl Pts',(-24.6001000414851,7.14795446886728,-59.7496996349988));
#53974=CARTESIAN_POINT('Ctrl Pts',(-24.5963267699639,7.13078998746342,-59.713203608095));
#53975=CARTESIAN_POINT('Ctrl Pts',(-24.5886731810201,7.09597407655986,-59.6391761795279));
#53976=CARTESIAN_POINT('Ctrl Pts',(-24.58105329827,7.06139276976336,-59.5649721004123));
#53977=CARTESIAN_POINT('Ctrl Pts',(-24.5734606104834,7.02728461174253,-59.4910568103805));
#53978=CARTESIAN_POINT('Ctrl Pts',(-24.5636741126434,6.98332133757985,-59.3957846423995));
#53979=CARTESIAN_POINT('Ctrl Pts',(-24.5539335820194,6.94014571561547,-59.3009912537256));
#53980=CARTESIAN_POINT('Ctrl Pts',(-24.5442226032045,6.89808037257437,-59.2073294929134));
#53981=CARTESIAN_POINT('Ctrl Pts',(-24.5416644851313,6.88699929451397,-59.1826566100174));
#53982=CARTESIAN_POINT('Ctrl Pts',(-24.5391083193834,6.87599500118245,-59.1580622963691));
#53983=CARTESIAN_POINT('Ctrl Pts',(-24.5365535829411,6.86507286998188,-59.1335587093582));
#53984=CARTESIAN_POINT('Ctrl Pts',(-24.531532367751,6.84360593108926,-59.0853980532233));
#53985=CARTESIAN_POINT('Ctrl Pts',(-24.5265166119427,6.82245811143022,-59.0375914462527));
#53986=CARTESIAN_POINT('Ctrl Pts',(-24.5214880208954,6.8018476240916,-58.9906631794842));
#53987=CARTESIAN_POINT('Ctrl Pts',(-24.5202367873599,6.79671924266268,-58.9789863060638));
#53988=CARTESIAN_POINT('Ctrl Pts',(-24.5189847612876,6.79162401850022,-58.967363593278));
#53989=CARTESIAN_POINT('Ctrl Pts',(-24.5177316660908,6.78656507652644,-58.9558026410564));
#53990=CARTESIAN_POINT('Ctrl Pts',(-24.5145490120368,6.77371620261572,-58.9264397390598));
#53991=CARTESIAN_POINT('Ctrl Pts',(-24.5113596688225,6.7610994594533,-58.8974704883638));
#53992=CARTESIAN_POINT('Ctrl Pts',(-24.508181636039,6.74846010516535,-58.8682875733842));
#53993=CARTESIAN_POINT('Ctrl Pts',(-24.5052694035877,6.73687786538744,-58.8415454225581));
#53994=CARTESIAN_POINT('Ctrl Pts',(-24.5023666549417,6.72527668001029,-58.8146239786376));
#53995=CARTESIAN_POINT('Ctrl Pts',(-24.4994852743528,6.71347910466107,-58.7871019844863));
#53996=CARTESIAN_POINT('Ctrl Pts',(-24.4992222898793,6.71240233640863,-58.7845900437977));
#53997=CARTESIAN_POINT('Ctrl Pts',(-24.4989594820256,6.71132394573296,-58.7820731338583));
#53998=CARTESIAN_POINT('Ctrl Pts',(-24.4986968589845,6.71024380605157,-58.7795509549467));
#53999=CARTESIAN_POINT('',(-23.6739538968997,12.846244756358,-70.6467988317471));
#54000=CARTESIAN_POINT('Ctrl Pts',(-23.6739538968997,12.846244756358,-70.6467988317471));
#54001=CARTESIAN_POINT('Ctrl Pts',(-23.7652621574204,12.6829373366643,-70.3394704142904));
#54002=CARTESIAN_POINT('Ctrl Pts',(-24.0270822733915,12.1921901977266,-69.4189320572497));
#54003=CARTESIAN_POINT('Ctrl Pts',(-24.3752871742381,11.4464620234297,-68.0281725531546));
#54004=CARTESIAN_POINT('Ctrl Pts',(-24.6927334369296,10.5534106262424,-66.3568311811825));
#54005=CARTESIAN_POINT('Ctrl Pts',(-24.8064000890597,9.94888081636442,-65.1999953822759));
#54006=CARTESIAN_POINT('Ctrl Pts',(-24.834404590668,9.66888169588114,-64.6543281145607));
#54007=CARTESIAN_POINT('',(-21.0403876111779,16.0446155815448,-76.6642782169352));
#54008=CARTESIAN_POINT('Ctrl Pts',(-21.0403876111779,16.0446155815448,-76.6642782169352));
#54009=CARTESIAN_POINT('Ctrl Pts',(-21.1157744386118,15.9895528116427,-76.5606151308124));
#54010=CARTESIAN_POINT('Ctrl Pts',(-21.1894544949622,15.9330326908327,-76.4542145604713));
#54011=CARTESIAN_POINT('Ctrl Pts',(-21.2615519837989,15.8752394470457,-76.3454234075435));
#54012=CARTESIAN_POINT('Ctrl Pts',(-21.3425035537031,15.8103487845565,-76.2232719323215));
#54013=CARTESIAN_POINT('Ctrl Pts',(-21.4214605193681,15.7438528570669,-76.0981061976719));
#54014=CARTESIAN_POINT('Ctrl Pts',(-21.4985706912578,15.6759811894835,-75.9703585271215));
#54015=CARTESIAN_POINT('Ctrl Pts',(-21.5673831294008,15.615413111203,-75.8563576312315));
#54016=CARTESIAN_POINT('Ctrl Pts',(-21.6347244735916,15.5537485428601,-75.740298881361));
#54017=CARTESIAN_POINT('Ctrl Pts',(-21.7006795254284,15.491137347613,-75.6224646500583));
#54018=CARTESIAN_POINT('Ctrl Pts',(-21.7660650693083,15.4290667868266,-75.5056478924814));
#54019=CARTESIAN_POINT('Ctrl Pts',(-21.8302672176974,15.3658891486313,-75.3867550339643));
#54020=CARTESIAN_POINT('Ctrl Pts',(-21.8931017751448,15.301979237563,-75.2664911270759));
#54021=CARTESIAN_POINT('Ctrl Pts',(-21.9140608170538,15.2806615016086,-75.2263759998752));
#54022=CARTESIAN_POINT('Ctrl Pts',(-21.9348679110239,15.2592624788604,-75.1861086789179));
#54023=CARTESIAN_POINT('Ctrl Pts',(-21.9555168651605,15.2377965702097,-75.1457162520817));
#54024=CARTESIAN_POINT('Ctrl Pts',(-22.0271530207548,15.1633262042088,-75.0055852723458));
#54025=CARTESIAN_POINT('Ctrl Pts',(-22.096882122716,15.0880497994365,-74.863946650444));
#54026=CARTESIAN_POINT('Ctrl Pts',(-22.1648447318524,15.0120088428319,-74.720877921363));
#54027=CARTESIAN_POINT('Ctrl Pts',(-22.2328073409888,14.9359678862273,-74.5778091922819));
#54028=CARTESIAN_POINT('Ctrl Pts',(-22.2990048300633,14.8591617040834,-74.4333090900849));
#54029=CARTESIAN_POINT('Ctrl Pts',(-22.363614314154,14.7816525062363,-74.2874939422127));
#54030=CARTESIAN_POINT('Ctrl Pts',(-22.4167826773859,14.7178687252177,-74.1674999064158));
#54031=CARTESIAN_POINT('Ctrl Pts',(-22.4687952306308,14.6537059438917,-74.0467978231759));
#54032=CARTESIAN_POINT('Ctrl Pts',(-22.5197134187718,14.5892908679778,-73.9256254181383));
#54033=CARTESIAN_POINT('Ctrl Pts',(-22.5315313738241,14.5743403267345,-73.8975016751578));
#54034=CARTESIAN_POINT('Ctrl Pts',(-22.5432903955293,14.5593762976717,-73.8693527895989));
#54035=CARTESIAN_POINT('Ctrl Pts',(-22.5549912688892,14.5444005592069,-73.8411820979184));
#54036=CARTESIAN_POINT('Ctrl Pts',(-22.5802750736682,14.5120402698404,-73.7803095248174));
#54037=CARTESIAN_POINT('Ctrl Pts',(-22.6054781494533,14.4793808052658,-73.7188752021463));
#54038=CARTESIAN_POINT('Ctrl Pts',(-22.6305925092312,14.4464447355768,-73.656921526668));
#54039=CARTESIAN_POINT('Ctrl Pts',(-22.6570055251894,14.4118055513813,-73.5917642447962));
#54040=CARTESIAN_POINT('Ctrl Pts',(-22.6833051765735,14.3768807447599,-73.5260705381479));
#54041=CARTESIAN_POINT('Ctrl Pts',(-22.7095089054492,14.3416661164437,-73.4598327530951));
#54042=CARTESIAN_POINT('Ctrl Pts',(-22.7708723054029,14.2592011614813,-73.3047183525638));
#54043=CARTESIAN_POINT('Ctrl Pts',(-22.8317093809367,14.1751448480743,-73.1466165290608));
#54044=CARTESIAN_POINT('Ctrl Pts',(-22.8917965026637,14.0899135670005,-72.9863073813454));
#54045=CARTESIAN_POINT('Ctrl Pts',(-22.9019397255509,14.0755257937799,-72.959245818578));
#54046=CARTESIAN_POINT('Ctrl Pts',(-22.9120615982471,14.0611045940741,-72.9321214595726));
#54047=CARTESIAN_POINT('Ctrl Pts',(-22.9221610720533,14.0466520342293,-72.9049381755185));
#54048=CARTESIAN_POINT('Ctrl Pts',(-23.0008434107626,13.9340559494477,-72.6931603736021));
#54049=CARTESIAN_POINT('Ctrl Pts',(-23.0782166637999,13.8194803232158,-72.4776639036223));
#54050=CARTESIAN_POINT('Ctrl Pts',(-23.153934413458,13.7037037360802,-72.2599027125882));
#54051=CARTESIAN_POINT('Ctrl Pts',(-23.1663291103867,13.6847515654799,-72.2242560646371));
#54052=CARTESIAN_POINT('Ctrl Pts',(-23.1786794750302,13.6657672647917,-72.1885488265631));
#54053=CARTESIAN_POINT('Ctrl Pts',(-23.1909840247367,13.6467543026212,-72.1527874762431));
#54054=CARTESIAN_POINT('Ctrl Pts',(-23.2766051125639,13.5144527927993,-71.9039424725987));
#54055=CARTESIAN_POINT('Ctrl Pts',(-23.360006842537,13.3807628703025,-71.6524754466928));
#54056=CARTESIAN_POINT('Ctrl Pts',(-23.4407760922421,13.2467437015264,-71.4003541575491));
#54057=CARTESIAN_POINT('Ctrl Pts',(-23.4810080390131,13.1799874535214,-71.274770097753));
#54058=CARTESIAN_POINT('Ctrl Pts',(-23.5205870372981,13.1131486974205,-71.14902216018));
#54059=CARTESIAN_POINT('Ctrl Pts',(-23.5594144433799,13.0464455753219,-71.023518316434));
#54060=CARTESIAN_POINT('Ctrl Pts',(-23.5982418494616,12.9797424532234,-70.898014472688));
#54061=CARTESIAN_POINT('Ctrl Pts',(-23.6363197141491,12.9131779257759,-70.7727603664136));
#54062=CARTESIAN_POINT('Ctrl Pts',(-23.6738690325247,12.8463956913735,-70.6470828763833));
#54063=CARTESIAN_POINT('',(-20.8066780834711,16.2071460528287,-76.9702782129914));
#54064=CARTESIAN_POINT('Ctrl Pts',(-20.806678083471,16.2071460528287,-76.9702782129914));
#54065=CARTESIAN_POINT('Ctrl Pts',(-20.8862783237883,16.1545206907567,-76.8711944318144));
#54066=CARTESIAN_POINT('Ctrl Pts',(-20.964160252313,16.1002920803761,-76.7690967308679));
#54067=CARTESIAN_POINT('Ctrl Pts',(-21.040387611155,16.0446155815615,-76.6642782169667));
#54068=CARTESIAN_POINT('',(-25.7066762066276,16.4237761199824,-77.3782788360333));
#54069=CARTESIAN_POINT('Ctrl Pts',(-25.7066762066276,16.4237761199824,-77.3782788360333));
#54070=CARTESIAN_POINT('Ctrl Pts',(-25.6911863733062,16.507982961079,-77.5366055866555));
#54071=CARTESIAN_POINT('Ctrl Pts',(-25.6219414370306,16.672353368847,-77.845549521693));
#54072=CARTESIAN_POINT('Ctrl Pts',(-25.2871445035823,16.9752951011235,-78.4144172197497));
#54073=CARTESIAN_POINT('Ctrl Pts',(-24.6881842909862,17.1791668341045,-78.7966009790571));
#54074=CARTESIAN_POINT('Ctrl Pts',(-24.0052836532123,17.2918079376106,-79.007776150789));
#54075=CARTESIAN_POINT('Ctrl Pts',(-23.4548404136072,17.3408644644138,-79.0998653586004));
#54076=CARTESIAN_POINT('Ctrl Pts',(-22.915385779096,17.3537835256363,-79.1243293554279));
#54077=CARTESIAN_POINT('Ctrl Pts',(-22.453183479509,17.3348149207234,-79.0890214085024));
#54078=CARTESIAN_POINT('Ctrl Pts',(-22.1409244224793,17.3017278860839,-79.0271274374767));
#54079=CARTESIAN_POINT('Ctrl Pts',(-21.9683332638225,17.2768673638735,-78.980572195562));
#54080=CARTESIAN_POINT('Ctrl Pts',(-21.842286688042,17.2550204029918,-78.9396380523261));
#54081=CARTESIAN_POINT('Ctrl Pts',(-21.7192769440428,17.2296451041489,-78.8920701039884));
#54082=CARTESIAN_POINT('Ctrl Pts',(-21.6202901990439,17.2054366649431,-78.8466701327192));
#54083=CARTESIAN_POINT('Ctrl Pts',(-21.5578972221677,17.1881137776076,-78.8141735369845));
#54084=CARTESIAN_POINT('Ctrl Pts',(-21.5200612514553,17.1770416352821,-78.7934005178304));
#54085=CARTESIAN_POINT('Ctrl Pts',(-21.4920163013668,17.1684848139744,-78.7773452063036));
#54086=CARTESIAN_POINT('Ctrl Pts',(-21.4598148077115,17.1581297618176,-78.7579137361204));
#54087=CARTESIAN_POINT('Ctrl Pts',(-21.4325806776235,17.1489958995923,-78.7407724150982));
#54088=CARTESIAN_POINT('Ctrl Pts',(-21.410197465255,17.1411647504829,-78.726074667103));
#54089=CARTESIAN_POINT('Ctrl Pts',(-21.392491440011,17.1347699480245,-78.7140719746968));
#54090=CARTESIAN_POINT('Ctrl Pts',(-21.2430108509951,17.0796173710175,-78.6105496138558));
#54091=CARTESIAN_POINT('Ctrl Pts',(-21.0013130164285,16.9524612526866,-78.3717421247602));
#54092=CARTESIAN_POINT('Ctrl Pts',(-20.7388418587697,16.6352545775742,-77.7755268245789));
#54093=CARTESIAN_POINT('Ctrl Pts',(-20.7560657229672,16.3737697050196,-77.2837215842416));
#54094=CARTESIAN_POINT('Ctrl Pts',(-20.8066780834711,16.2071460528287,-76.9702782129914));
#54095=CARTESIAN_POINT('',(-25.9580275654167,16.0437450369841,-76.6642789908811));
#54096=CARTESIAN_POINT('Ctrl Pts',(-25.9580171294882,16.0437528221483,-76.6643138637023));
#54097=CARTESIAN_POINT('Ctrl Pts',(-25.8750885959483,16.1725292612534,-76.9062552995085));
#54098=CARTESIAN_POINT('Ctrl Pts',(-25.7912591348258,16.2994925070891,-77.1447932578045));
#54099=CARTESIAN_POINT('Ctrl Pts',(-25.7066761933522,16.4237671850429,-77.3782835868249));
#54100=CARTESIAN_POINT('',(-27.8093579489709,12.8426393697465,-70.6502216955646));
#54101=CARTESIAN_POINT('Ctrl Pts',(-27.8093579489709,12.8426393697465,-70.6502216955646));
#54102=CARTESIAN_POINT('Ctrl Pts',(-27.6629613805351,13.0960632412153,-71.1288965648361));
#54103=CARTESIAN_POINT('Ctrl Pts',(-27.3589056055191,13.6404286392169,-72.1540324778666));
#54104=CARTESIAN_POINT('Ctrl Pts',(-26.7510733868799,14.7393369280985,-74.2160146070454));
#54105=CARTESIAN_POINT('Ctrl Pts',(-26.2631471674262,15.5696171136249,-75.7735033231351));
#54106=CARTESIAN_POINT('Ctrl Pts',(-25.9580275654167,16.0437450369841,-76.6642789908811));
#54107=CARTESIAN_POINT('',(-30.33736888334,9.77553124130067,-64.7925772570574));
#54108=CARTESIAN_POINT('Ctrl Pts',(-30.3373681408964,9.77560492643774,-64.7925461433589));
#54109=CARTESIAN_POINT('Ctrl Pts',(-30.1852567493822,9.8786370639834,-65.0401821262795));
#54110=CARTESIAN_POINT('Ctrl Pts',(-30.0522518687011,9.97792805405255,-65.2605477273785));
#54111=CARTESIAN_POINT('Ctrl Pts',(-29.5847277881304,10.3617001491574,-66.0727023311734));
#54112=CARTESIAN_POINT('Ctrl Pts',(-29.2973751005394,10.6626910528547,-66.6432962914613));
#54113=CARTESIAN_POINT('Ctrl Pts',(-28.7957862062539,11.271428069297,-67.7691626336424));
#54114=CARTESIAN_POINT('Ctrl Pts',(-28.575739044809,11.5846998083453,-68.3335909516651));
#54115=CARTESIAN_POINT('Ctrl Pts',(-28.2728671785687,12.0549538215514,-69.1894896819946));
#54116=CARTESIAN_POINT('Ctrl Pts',(-28.1756180623507,12.2132686880608,-69.4789022400814));
#54117=CARTESIAN_POINT('Ctrl Pts',(-28.0350849141614,12.4495248094586,-69.9150228417591));
#54118=CARTESIAN_POINT('Ctrl Pts',(-27.9889555168352,12.5283881508439,-70.061304788306));
#54119=CARTESIAN_POINT('Ctrl Pts',(-27.9208881500455,12.646344253899,-70.281369857301));
#54120=CARTESIAN_POINT('Ctrl Pts',(-27.8983536215529,12.6856658373485,-70.3549429927763));
#54121=CARTESIAN_POINT('Ctrl Pts',(-27.8529729253694,12.7653429953578,-70.5044861836174));
#54122=CARTESIAN_POINT('Ctrl Pts',(-27.8307788796621,12.8045663382374,-70.5783475852013));
#54123=CARTESIAN_POINT('Ctrl Pts',(-27.8093579217479,12.8426234408141,-70.6502301207803));
#54124=CARTESIAN_POINT('',(-32.81521999432,8.33900374689714,-59.2033586636525));
#54125=CARTESIAN_POINT('Ctrl Pts',(-32.815219994237,8.33900374759826,-59.2033586635242));
#54126=CARTESIAN_POINT('Ctrl Pts',(-32.6923181777297,8.39620454756814,-59.5955480932275));
#54127=CARTESIAN_POINT('Ctrl Pts',(-32.3170499076978,8.58960686180279,-60.7566922032304));
#54128=CARTESIAN_POINT('Ctrl Pts',(-31.4950115977029,9.06913125042783,-62.8815100017806));
#54129=CARTESIAN_POINT('Ctrl Pts',(-30.825979501774,9.43523105888426,-63.9748521677351));
#54130=CARTESIAN_POINT('Ctrl Pts',(-30.33736888334,9.77553124130067,-64.7925772570574));
#54131=CARTESIAN_POINT('',(-34.9063163914144,8.66722257324563,-53.4437571318393));
#54132=CARTESIAN_POINT('Ctrl Pts',(-34.9063163914144,8.66722257324563,-53.4437571318393));
#54133=CARTESIAN_POINT('Ctrl Pts',(-34.5724735540937,8.60352804275007,-54.2895979904455));
#54134=CARTESIAN_POINT('Ctrl Pts',(-34.0106677638488,8.38266385056441,-55.6375787991562));
#54135=CARTESIAN_POINT('Ctrl Pts',(-33.3555720402961,8.20876541621131,-57.5526773984119));
#54136=CARTESIAN_POINT('Ctrl Pts',(-32.9982863465608,8.26644533317311,-58.6882956274082));
#54137=CARTESIAN_POINT('Ctrl Pts',(-32.815219994237,8.33900374759826,-59.2033586635242));
#54138=CARTESIAN_POINT('',(-36.4974177553682,8.64413762617978,-47.4049093964133));
#54139=CARTESIAN_POINT('Ctrl Pts',(-36.4973970222996,8.64418876114758,-47.4049059587411));
#54140=CARTESIAN_POINT('Ctrl Pts',(-36.4930289916103,8.64553623909837,-47.4512937213671));
#54141=CARTESIAN_POINT('Ctrl Pts',(-36.4886315292324,8.64694889881603,-47.4972561440451));
#54142=CARTESIAN_POINT('Ctrl Pts',(-36.484192549884,8.64843677203915,-47.5430220976373));
#54143=CARTESIAN_POINT('Ctrl Pts',(-36.4787175260311,8.65027191042287,-47.5994696879291));
#54144=CARTESIAN_POINT('Ctrl Pts',(-36.4731794617622,8.65222167439011,-47.6556192569373));
#54145=CARTESIAN_POINT('Ctrl Pts',(-36.4675493926941,8.65430341847232,-47.7119871384523));
#54146=CARTESIAN_POINT('Ctrl Pts',(-36.4658463631896,8.6549331215097,-47.7290377579324));
#54147=CARTESIAN_POINT('Ctrl Pts',(-36.4641348729266,8.65557487828422,-47.7461087665885));
#54148=CARTESIAN_POINT('Ctrl Pts',(-36.4624140181909,8.65622909617189,-47.7632151944437));
#54149=CARTESIAN_POINT('Ctrl Pts',(-36.4536224220762,8.65957140003995,-47.8506094419356));
#54150=CARTESIAN_POINT('Ctrl Pts',(-36.4445877356492,8.66324213430238,-47.9389321062188));
#54151=CARTESIAN_POINT('Ctrl Pts',(-36.4352616615615,8.66706716925153,-48.0267057038783));
#54152=CARTESIAN_POINT('Ctrl Pts',(-36.4318722169841,8.66845733019651,-48.0586059163179));
#54153=CARTESIAN_POINT('Ctrl Pts',(-36.4284441225271,8.66986751298689,-48.0904332878203));
#54154=CARTESIAN_POINT('Ctrl Pts',(-36.4249745171483,8.67128828565653,-48.1221167741548));
#54155=CARTESIAN_POINT('Ctrl Pts',(-36.4163577663833,8.67481676876961,-48.2008025828584));
#54156=CARTESIAN_POINT('Ctrl Pts',(-36.407485592542,8.67841162841733,-48.2786028353604));
#54157=CARTESIAN_POINT('Ctrl Pts',(-36.3982992396125,8.68193730465335,-48.3547699804819));
#54158=CARTESIAN_POINT('Ctrl Pts',(-36.3832550118477,8.68771120390653,-48.4795067381686));
#54159=CARTESIAN_POINT('Ctrl Pts',(-36.3674213410786,8.69348144139046,-48.6016400496475));
#54160=CARTESIAN_POINT('Ctrl Pts',(-36.3506717255914,8.69909693977363,-48.7215796362339));
#54161=CARTESIAN_POINT('Ctrl Pts',(-36.3447399773247,8.70108562559313,-48.7640553238337));
#54162=CARTESIAN_POINT('Ctrl Pts',(-36.3386935379683,8.70305534242297,-48.80625573984));
#54163=CARTESIAN_POINT('Ctrl Pts',(-36.3325273598475,8.7050007255993,-48.8481986924699));
#54164=CARTESIAN_POINT('Ctrl Pts',(-36.3139269188474,8.71086902591192,-48.974720729375));
#54165=CARTESIAN_POINT('Ctrl Pts',(-36.2942355210381,8.71651232896629,-49.0988978177763));
#54166=CARTESIAN_POINT('Ctrl Pts',(-36.273332807523,8.72179936887609,-49.2210928935335));
#54167=CARTESIAN_POINT('Ctrl Pts',(-36.2514155037859,8.72734303474937,-49.3492191575517));
#54168=CARTESIAN_POINT('Ctrl Pts',(-36.2281665678998,8.73249563709191,-49.4751662784035));
#54169=CARTESIAN_POINT('Ctrl Pts',(-36.2034673290701,8.73715372561922,-49.5993803218675));
#54170=CARTESIAN_POINT('Ctrl Pts',(-36.1770276647907,8.74214004514491,-49.7323470756462));
#54171=CARTESIAN_POINT('Ctrl Pts',(-36.1489261982809,8.74656032064097,-49.863327691379));
#54172=CARTESIAN_POINT('Ctrl Pts',(-36.1190381533995,8.75033147847292,-49.9929025197663));
#54173=CARTESIAN_POINT('Ctrl Pts',(-36.1146844987613,8.75088080576588,-50.0117770916841));
#54174=CARTESIAN_POINT('Ctrl Pts',(-36.1102929679145,8.75141642102278,-50.0306218921998));
#54175=CARTESIAN_POINT('Ctrl Pts',(-36.1058632068143,8.751938125806,-50.0494387730954));
#54176=CARTESIAN_POINT('Ctrl Pts',(-36.0835767301713,8.75456286361976,-50.144107981453));
#54177=CARTESIAN_POINT('Ctrl Pts',(-36.0602596436235,8.75682996775874,-50.2382269535845));
#54178=CARTESIAN_POINT('Ctrl Pts',(-36.0358615729958,8.75871909889858,-50.3320618854742));
#54179=CARTESIAN_POINT('Ctrl Pts',(-35.9999440738256,8.76150017397549,-50.4702005169957));
#54180=CARTESIAN_POINT('Ctrl Pts',(-35.9616833399972,8.76346229475952,-50.6077212978283));
#54181=CARTESIAN_POINT('Ctrl Pts',(-35.9209301557936,8.76454314369576,-50.7455436566489));
#54182=CARTESIAN_POINT('Ctrl Pts',(-35.8822140489112,8.76556996561794,-50.8764768654072));
#54183=CARTESIAN_POINT('Ctrl Pts',(-35.8412488566998,8.76580268314493,-51.0076821423615));
#54184=CARTESIAN_POINT('Ctrl Pts',(-35.7979164514549,8.76518430437887,-51.1399924693141));
#54185=CARTESIAN_POINT('Ctrl Pts',(-35.7818028154709,8.76495435336922,-51.1891935333535));
#54186=CARTESIAN_POINT('Ctrl Pts',(-35.7653619105376,8.76460658281126,-51.2385478748913));
#54187=CARTESIAN_POINT('Ctrl Pts',(-35.7485878674312,8.76413739810438,-51.2881000964566));
#54188=CARTESIAN_POINT('Ctrl Pts',(-35.7079903302002,8.76300184935893,-51.4080293315912));
#54189=CARTESIAN_POINT('Ctrl Pts',(-35.6654412007548,8.76115656530288,-51.529114700737));
#54190=CARTESIAN_POINT('Ctrl Pts',(-35.620851257772,8.75854559565368,-51.6520184108547));
#54191=CARTESIAN_POINT('Ctrl Pts',(-35.5961416953814,8.75709872415909,-51.7201256271918));
#54192=CARTESIAN_POINT('Ctrl Pts',(-35.5708054769911,8.75541638233675,-51.7887919529377));
#54193=CARTESIAN_POINT('Ctrl Pts',(-35.5448277903592,8.75348544289058,-51.8581361380061));
#54194=CARTESIAN_POINT('Ctrl Pts',(-35.5034267713903,8.75040807646563,-51.9686509795348));
#54195=CARTESIAN_POINT('Ctrl Pts',(-35.4603963380976,8.74670139246173,-52.0808858519023));
#54196=CARTESIAN_POINT('Ctrl Pts',(-35.4156751384311,8.74227587473622,-52.1953420239112));
#54197=CARTESIAN_POINT('Ctrl Pts',(-35.373287056294,8.73808123751165,-52.3038269853255));
#54198=CARTESIAN_POINT('Ctrl Pts',(-35.329379885665,8.73324135910154,-52.414307454948));
#54199=CARTESIAN_POINT('Ctrl Pts',(-35.2839046009633,8.72764503042221,-52.5272398205582));
#54200=CARTESIAN_POINT('Ctrl Pts',(-35.2414710308672,8.72242302451609,-52.6326184560888));
#54201=CARTESIAN_POINT('Ctrl Pts',(-35.197671958818,8.71654270599691,-52.7401319985077));
#54202=CARTESIAN_POINT('Ctrl Pts',(-35.1524723942141,8.70987655801072,-52.8501776988826));
#54203=CARTESIAN_POINT('Ctrl Pts',(-35.1380366349633,8.70774753512516,-52.8853239055136));
#54204=CARTESIAN_POINT('Ctrl Pts',(-35.1234580703044,8.70553803581093,-52.9207286095553));
#54205=CARTESIAN_POINT('Ctrl Pts',(-35.1087357173717,8.70324293979444,-52.9564053679361));
#54206=CARTESIAN_POINT('Ctrl Pts',(-35.0659132069259,8.69656725598293,-53.0601773917032));
#54207=CARTESIAN_POINT('Ctrl Pts',(-35.0218735461726,8.68917045117481,-53.166249305713));
#54208=CARTESIAN_POINT('Ctrl Pts',(-34.9765945533639,8.68090166712676,-53.2749698162118));
#54209=CARTESIAN_POINT('Ctrl Pts',(-34.9534600464532,8.67667687700144,-53.3305186534418));
#54210=CARTESIAN_POINT('Ctrl Pts',(-34.9300021434374,8.67222379725344,-53.3867592998611));
#54211=CARTESIAN_POINT('Ctrl Pts',(-34.9062189727919,8.66751773911485,-53.4437408417599));
#54212=CARTESIAN_POINT('',(-37.4912550961874,8.66275191199404,-41.3740808902194));
#54213=CARTESIAN_POINT('Ctrl Pts',(-37.491189835617,8.6629355512308,-41.3740675237284));
#54214=CARTESIAN_POINT('Ctrl Pts',(-37.356700123897,8.65117444483456,-41.870984084739));
#54215=CARTESIAN_POINT('Ctrl Pts',(-37.1655465363814,8.62975442365193,-42.611977051936));
#54216=CARTESIAN_POINT('Ctrl Pts',(-36.88503216533,8.59955674721597,-43.9209841884754));
#54217=CARTESIAN_POINT('Ctrl Pts',(-36.6512741057588,8.59103223488232,-45.4978226844016));
#54218=CARTESIAN_POINT('Ctrl Pts',(-36.5532891736331,8.62548607044055,-46.792631727622));
#54219=CARTESIAN_POINT('Ctrl Pts',(-36.4974177553682,8.64413762617978,-47.4049093964133));
#54220=CARTESIAN_POINT('',(-38.9091460669097,8.64371781494149,-35.3259112856609));
#54221=CARTESIAN_POINT('Ctrl Pts',(-38.9090921504208,8.64388899039054,-35.3258962859625));
#54222=CARTESIAN_POINT('Ctrl Pts',(-38.9089923803477,8.64391395683976,-35.3265391752867));
#54223=CARTESIAN_POINT('Ctrl Pts',(-38.9088925687444,8.64393892778801,-35.3271821637191));
#54224=CARTESIAN_POINT('Ctrl Pts',(-38.9087927155238,8.64396390325458,-35.3278252515927));
#54225=CARTESIAN_POINT('Ctrl Pts',(-38.9010416619146,8.64590261068036,-35.377744608754));
#54226=CARTESIAN_POINT('Ctrl Pts',(-38.893040948649,8.6478815213966,-35.4291730896422));
#54227=CARTESIAN_POINT('Ctrl Pts',(-38.8847602428943,8.64987340469648,-35.4819038201963));
#54228=CARTESIAN_POINT('Ctrl Pts',(-38.8774468694352,8.65163260094019,-35.5284746725773));
#54229=CARTESIAN_POINT('Ctrl Pts',(-38.8699150880467,8.65340194442179,-35.5760616904033));
#54230=CARTESIAN_POINT('Ctrl Pts',(-38.8621452295201,8.65515861579911,-35.6244816485022));
#54231=CARTESIAN_POINT('Ctrl Pts',(-38.8578352844873,8.65613304243134,-35.6513402273532));
#54232=CARTESIAN_POINT('Ctrl Pts',(-38.8534521080782,8.65710349341095,-35.6784543186067));
#54233=CARTESIAN_POINT('Ctrl Pts',(-38.8489925569198,8.65806538151594,-35.7057855665315));
#54234=CARTESIAN_POINT('Ctrl Pts',(-38.837160129509,8.66061753772527,-35.7783029557562));
#54235=CARTESIAN_POINT('Ctrl Pts',(-38.8247903422569,8.66310890245544,-35.8523421507106));
#54236=CARTESIAN_POINT('Ctrl Pts',(-38.8117921403903,8.66555150832271,-35.9284109044899));
#54237=CARTESIAN_POINT('Ctrl Pts',(-38.8030160035092,8.66720070900891,-35.9797710697189));
#54238=CARTESIAN_POINT('Ctrl Pts',(-38.7939533509191,8.66882771198339,-36.0320571416344));
#54239=CARTESIAN_POINT('Ctrl Pts',(-38.7845753678349,8.67043697660535,-36.0854391578441));
#54240=CARTESIAN_POINT('Ctrl Pts',(-38.7626357657024,8.6742018187057,-36.2103253072602));
#54241=CARTESIAN_POINT('Ctrl Pts',(-38.7389709088127,8.67787156150978,-36.3412193387587));
#54242=CARTESIAN_POINT('Ctrl Pts',(-38.7132264474225,8.68142472654518,-36.4794520117829));
#54243=CARTESIAN_POINT('Ctrl Pts',(-38.7083652398284,8.6820956542679,-36.5055538482001));
#54244=CARTESIAN_POINT('Ctrl Pts',(-38.7034298482699,8.68276236529588,-36.5319172136502));
#54245=CARTESIAN_POINT('Ctrl Pts',(-38.6984178331563,8.68342462471417,-36.558550866477));
#54246=CARTESIAN_POINT('Ctrl Pts',(-38.6811269220411,8.68570934821904,-36.6504340937338));
#54247=CARTESIAN_POINT('Ctrl Pts',(-38.6629336867529,8.68791838048242,-36.7452218008698));
#54248=CARTESIAN_POINT('Ctrl Pts',(-38.6436861704223,8.690012614542,-36.8431203416096));
#54249=CARTESIAN_POINT('Ctrl Pts',(-38.6125355094802,8.6934019752264,-37.0015617839719));
#54250=CARTESIAN_POINT('Ctrl Pts',(-38.5786256817257,8.69649257073304,-37.1681471984866));
#54251=CARTESIAN_POINT('Ctrl Pts',(-38.5412800152023,8.6991051969997,-37.3439169337678));
#54252=CARTESIAN_POINT('Ctrl Pts',(-38.5374413725623,8.69937374056909,-37.3619837474971));
#54253=CARTESIAN_POINT('Ctrl Pts',(-38.5335664272518,8.69963719321634,-37.3801474087064));
#54254=CARTESIAN_POINT('Ctrl Pts',(-38.5296547036981,8.69989534537905,-37.3984080931803));
#54255=CARTESIAN_POINT('Ctrl Pts',(-38.4929974502891,8.70231452176423,-37.5695312640755));
#54256=CARTESIAN_POINT('Ctrl Pts',(-38.4531125120698,8.70427049130661,-37.7491723002855));
#54257=CARTESIAN_POINT('Ctrl Pts',(-38.4096004714822,8.70558653496202,-37.9374917606443));
#54258=CARTESIAN_POINT('Ctrl Pts',(-38.3846707945306,8.70634054563908,-38.0453870293346));
#54259=CARTESIAN_POINT('Ctrl Pts',(-38.3585500110649,8.70688401621914,-38.1561316054534));
#54260=CARTESIAN_POINT('Ctrl Pts',(-38.3311593377478,8.70717887644011,-38.2697606369798));
#54261=CARTESIAN_POINT('Ctrl Pts',(-38.3244562750184,8.70725103481807,-38.2975680047425));
#54262=CARTESIAN_POINT('Ctrl Pts',(-38.3176771765432,8.70730828039793,-38.3255479458308));
#54263=CARTESIAN_POINT('Ctrl Pts',(-38.3108174593195,8.70734996070891,-38.3537140754484));
#54264=CARTESIAN_POINT('Ctrl Pts',(-38.2765890091585,8.70755793611093,-38.4942567439596));
#54265=CARTESIAN_POINT('Ctrl Pts',(-38.2403549331725,8.70738074668867,-38.6394344676793));
#54266=CARTESIAN_POINT('Ctrl Pts',(-38.2015342101401,8.70671971787683,-38.7909302440284));
#54267=CARTESIAN_POINT('Ctrl Pts',(-38.1708049037257,8.706196467527,-38.910849703747));
#54268=CARTESIAN_POINT('Ctrl Pts',(-38.1384610683968,8.70536846681098,-39.0347278181911));
#54269=CARTESIAN_POINT('Ctrl Pts',(-38.1057102218041,8.70427431951171,-39.1582853361838));
#54270=CARTESIAN_POINT('Ctrl Pts',(-38.0887946401576,8.7037092001362,-39.2221019241832));
#54271=CARTESIAN_POINT('Ctrl Pts',(-38.0717710110007,8.70307368167698,-39.2858329237427));
#54272=CARTESIAN_POINT('Ctrl Pts',(-38.0548093062264,8.70237725162869,-39.3488880213126));
#54273=CARTESIAN_POINT('Ctrl Pts',(-37.9738109041856,8.6990515410474,-39.6499993902266));
#54274=CARTESIAN_POINT('Ctrl Pts',(-37.8941771573195,8.69432620811437,-39.9357008070417));
#54275=CARTESIAN_POINT('Ctrl Pts',(-37.8166126392952,8.68890321160458,-40.211615336106));
#54276=CARTESIAN_POINT('Ctrl Pts',(-37.7987960992563,8.68765755138637,-40.2749927975999));
#54277=CARTESIAN_POINT('Ctrl Pts',(-37.7810885840085,8.6863750335467,-40.3378537397244));
#54278=CARTESIAN_POINT('Ctrl Pts',(-37.763498260598,8.68506409032027,-40.4002661241927));
#54279=CARTESIAN_POINT('Ctrl Pts',(-37.7002374816639,8.68034949311207,-40.6247222620632));
#54280=CARTESIAN_POINT('Ctrl Pts',(-37.6384910072925,8.67526723033651,-40.8433800677456));
#54281=CARTESIAN_POINT('Ctrl Pts',(-37.5783484419992,8.67010156626611,-41.0592716010482));
#54282=CARTESIAN_POINT('Ctrl Pts',(-37.5489627761302,8.66757762207411,-41.1647562346124));
#54283=CARTESIAN_POINT('Ctrl Pts',(-37.5199593500415,8.66503352278262,-41.2695805547653));
#54284=CARTESIAN_POINT('Ctrl Pts',(-37.4913443196371,8.66250084268668,-41.3740991647216));
#54285=CARTESIAN_POINT('',(-39.8378651641511,8.40808204040271,-29.2047428884228));
#54286=CARTESIAN_POINT('Ctrl Pts',(-39.8378651639228,8.40808204093907,-29.204742888344));
#54287=CARTESIAN_POINT('Ctrl Pts',(-39.7403557200732,8.42558824320743,-29.6064705490188));
#54288=CARTESIAN_POINT('Ctrl Pts',(-39.5863221729383,8.46001992220811,-30.3835625396964));
#54289=CARTESIAN_POINT('Ctrl Pts',(-39.4599526712302,8.4939877818819,-31.1842583062903));
#54290=CARTESIAN_POINT('Ctrl Pts',(-39.3117522083446,8.53693747852479,-32.2573499658343));
#54291=CARTESIAN_POINT('Ctrl Pts',(-39.1834328367189,8.5752710622992,-33.3490981603829));
#54292=CARTESIAN_POINT('Ctrl Pts',(-39.0384531936711,8.61284501735072,-34.4653792758384));
#54293=CARTESIAN_POINT('Ctrl Pts',(-38.959857971873,8.63186531179917,-35.008020879665));
#54294=CARTESIAN_POINT('Ctrl Pts',(-38.9091460669097,8.64371781494149,-35.3259112856608));
#54295=CARTESIAN_POINT('',(-43.6350081753485,8.95468720513522,-22.9398480277775));
#54296=CARTESIAN_POINT('Ctrl Pts',(-43.6350081753485,8.95468720513522,-22.9398480277775));
#54297=CARTESIAN_POINT('Ctrl Pts',(-43.4741574413301,8.94820825817609,-23.1065847254121));
#54298=CARTESIAN_POINT('Ctrl Pts',(-43.1335328486735,8.92374576231794,-23.4666708399978));
#54299=CARTESIAN_POINT('Ctrl Pts',(-42.181557989294,8.79178703405004,-24.5033719122517));
#54300=CARTESIAN_POINT('Ctrl Pts',(-41.0217226392209,8.48128348309427,-26.0202735195218));
#54301=CARTESIAN_POINT('Ctrl Pts',(-40.2577289267292,8.36214502734256,-27.6878442174315));
#54302=CARTESIAN_POINT('Ctrl Pts',(-39.9631870435311,8.38841260911053,-28.7076954825739));
#54303=CARTESIAN_POINT('Ctrl Pts',(-39.8378651639228,8.4080820409391,-29.204742888344));
#54304=CARTESIAN_POINT('',(-56.9472987453291,10.4971210956015,-16.8490842893495));
#54305=CARTESIAN_POINT('Ctrl Pts',(-56.9472987452347,10.4971210960165,-16.8490842892202));
#54306=CARTESIAN_POINT('Ctrl Pts',(-56.2481469214632,10.4104471933364,-17.0815737981202));
#54307=CARTESIAN_POINT('Ctrl Pts',(-54.1344740653502,10.1093354912827,-17.7283592068575));
#54308=CARTESIAN_POINT('Ctrl Pts',(-51.3563456833993,9.61325730669952,-18.4697257428994));
#54309=CARTESIAN_POINT('Ctrl Pts',(-48.9121891096784,9.10710294010294,-19.2319251368394));
#54310=CARTESIAN_POINT('Ctrl Pts',(-47.2414265358552,8.840217651377,-19.9343653479424));
#54311=CARTESIAN_POINT('Ctrl Pts',(-46.0257479434454,8.82194194637927,-20.7196929414398));
#54312=CARTESIAN_POINT('Ctrl Pts',(-44.8748647635386,8.90526226846306,-21.6754872735224));
#54313=CARTESIAN_POINT('Ctrl Pts',(-44.0874700808914,8.96460650876973,-22.4409005690892));
#54314=CARTESIAN_POINT('Ctrl Pts',(-43.6350081753485,8.95468720513522,-22.9398480277775));
#54315=CARTESIAN_POINT('',(-69.6237422477832,12.3291004120271,-10.9554808154416));
#54316=CARTESIAN_POINT('Ctrl Pts',(-69.6237422477832,12.3291004120271,-10.9554808154416));
#54317=CARTESIAN_POINT('Ctrl Pts',(-69.0619467479908,12.2684092204603,-11.3706412385527));
#54318=CARTESIAN_POINT('Ctrl Pts',(-67.3257727339187,11.9872729690017,-12.5677786432507));
#54319=CARTESIAN_POINT('Ctrl Pts',(-65.1428673887983,11.4234020038613,-13.7075202041218));
#54320=CARTESIAN_POINT('Ctrl Pts',(-62.7668261595333,11.0221069854903,-14.6746180957437));
#54321=CARTESIAN_POINT('Ctrl Pts',(-61.0303852735734,10.8460095502133,-15.3378639972945));
#54322=CARTESIAN_POINT('Ctrl Pts',(-59.1522514841506,10.7106003736308,-16.0390772817491));
#54323=CARTESIAN_POINT('Ctrl Pts',(-57.6974034262523,10.5819199165458,-16.5733557441422));
#54324=CARTESIAN_POINT('Ctrl Pts',(-56.9472987452347,10.4971210960165,-16.8490842892202));
#54325=CARTESIAN_POINT('',(-76.0152010859362,13.203464721645,-5.1323536644963));
#54326=CARTESIAN_POINT('Ctrl Pts',(-76.0152010859361,13.203464721645,-5.1323536644963));
#54327=CARTESIAN_POINT('Ctrl Pts',(-75.6055079654791,13.12190451308,-5.716816608525));
#54328=CARTESIAN_POINT('Ctrl Pts',(-74.9215487758576,12.957479513477,-6.54678203039554));
#54329=CARTESIAN_POINT('Ctrl Pts',(-73.5802384751692,12.6798652978959,-7.873047892913));
#54330=CARTESIAN_POINT('Ctrl Pts',(-71.872722792672,12.4627641836395,-9.26669786648776));
#54331=CARTESIAN_POINT('Ctrl Pts',(-70.451678034269,12.4119687385728,-10.3168853345243));
#54332=CARTESIAN_POINT('Ctrl Pts',(-69.6237422477832,12.3291004120271,-10.9554808154415));
#54333=CARTESIAN_POINT('',(-77.8900123568112,13.4547375618153,-1.34395683259202));
#54334=CARTESIAN_POINT('Ctrl Pts',(-77.8897919792404,13.4547521615023,-1.34470326410749));
#54335=CARTESIAN_POINT('Ctrl Pts',(-77.687905838974,13.4682199621307,-2.0282002152612));
#54336=CARTESIAN_POINT('Ctrl Pts',(-77.4243415558115,13.4409012933351,-2.69552577166936));
#54337=CARTESIAN_POINT('Ctrl Pts',(-76.9525567732676,13.3724546737323,-3.64049244562797));
#54338=CARTESIAN_POINT('Ctrl Pts',(-76.7857287407807,13.3453290176752,-3.94159347054734));
#54339=CARTESIAN_POINT('Ctrl Pts',(-76.4200308904728,13.2814819277456,-4.54406678801877));
#54340=CARTESIAN_POINT('Ctrl Pts',(-76.2223690395977,13.2448574973167,-4.84142100893202));
#54341=CARTESIAN_POINT('Ctrl Pts',(-76.0153375294591,13.2031298898674,-5.13240265603379));
#54342=CARTESIAN_POINT('',(-71.7129439767344,8.64375557957816,1.03298829038523));
#54343=CARTESIAN_POINT('Ctrl Pts',(-71.7139042075071,8.64435208932012,1.03275752880096));
#54344=CARTESIAN_POINT('Ctrl Pts',(-71.7747188119592,8.68227215256098,1.01813579272073));
#54345=CARTESIAN_POINT('Ctrl Pts',(-71.8355664916663,8.72108772894506,1.00379664885951));
#54346=CARTESIAN_POINT('Ctrl Pts',(-71.8965306070675,8.76083117390857,0.989646569940123));
#54347=CARTESIAN_POINT('Ctrl Pts',(-71.966691596487,8.80657020256874,0.973361850137095));
#54348=CARTESIAN_POINT('Ctrl Pts',(-72.0370070497349,8.85353814249846,0.957327521923361));
#54349=CARTESIAN_POINT('Ctrl Pts',(-72.1076057540138,8.90179697013866,0.941404592495416));
#54350=CARTESIAN_POINT('Ctrl Pts',(-72.177854073707,8.94981628701864,0.925560689291656));
#54351=CARTESIAN_POINT('Ctrl Pts',(-72.2483828085012,8.99911375717801,0.909827250443446));
#54352=CARTESIAN_POINT('Ctrl Pts',(-72.319318686479,9.04976146747853,0.894069297918034));
#54353=CARTESIAN_POINT('Ctrl Pts',(-72.3888099009981,9.09937769838638,0.878632268159006));
#54354=CARTESIAN_POINT('Ctrl Pts',(-72.4586921083569,9.15028999732531,0.863171759399451));
#54355=CARTESIAN_POINT('Ctrl Pts',(-72.5290521981716,9.20255582626718,0.847568109351788));
#54356=CARTESIAN_POINT('Ctrl Pts',(-72.6359128789326,9.28193551546284,0.823869778794765));
#54357=CARTESIAN_POINT('Ctrl Pts',(-72.7438735159213,9.3644356615039,0.799841815292893));
#54358=CARTESIAN_POINT('Ctrl Pts',(-72.8530365481291,9.44985698853578,0.775079198820834));
#54359=CARTESIAN_POINT('Ctrl Pts',(-72.9033286761307,9.48921115657477,0.763670898299317));
#54360=CARTESIAN_POINT('Ctrl Pts',(-72.9538763340886,9.52918586174015,0.75210656838282));
#54361=CARTESIAN_POINT('Ctrl Pts',(-73.0046912038893,9.56976373539415,0.740346307564975));
#54362=CARTESIAN_POINT('Ctrl Pts',(-73.1234537853114,9.66460079869218,0.712860673174829));
#54363=CARTESIAN_POINT('Ctrl Pts',(-73.2436726461032,9.76273123797388,0.684305087434254));
#54364=CARTESIAN_POINT('Ctrl Pts',(-73.3655479475731,9.86396463519217,0.654162545478233));
#54365=CARTESIAN_POINT('Ctrl Pts',(-73.4834530575551,9.96190026849052,0.625001922434837));
#54366=CARTESIAN_POINT('Ctrl Pts',(-73.6029476879116,10.0626889841494,0.594338940577086));
#54367=CARTESIAN_POINT('Ctrl Pts',(-73.7243030596086,10.1661070351483,0.561682029959349));
#54368=CARTESIAN_POINT('Ctrl Pts',(-73.7942839346597,10.2257441620739,0.542850072629904));
#54369=CARTESIAN_POINT('Ctrl Pts',(-73.8648429610062,10.286308900022,0.523372952508207));
#54370=CARTESIAN_POINT('Ctrl Pts',(-73.9360196572315,10.3477822481166,0.503164180801907));
#54371=CARTESIAN_POINT('Ctrl Pts',(-73.9704193189414,10.3774922865248,0.493397291537105));
#54372=CARTESIAN_POINT('Ctrl Pts',(-74.0049632394888,10.4074145442767,0.483459525796313));
#54373=CARTESIAN_POINT('Ctrl Pts',(-74.0396557889533,10.4375468077449,0.473341248310394));
#54374=CARTESIAN_POINT('Ctrl Pts',(-74.0616239408447,10.4566272774976,0.466934113057424));
#54375=CARTESIAN_POINT('Ctrl Pts',(-74.0836491924182,10.4757897854284,0.460455326897042));
#54376=CARTESIAN_POINT('Ctrl Pts',(-74.1057326637109,10.4950337600684,0.453902493490168));
#54377=CARTESIAN_POINT('Ctrl Pts',(-74.1209340570077,10.5082805555209,0.449391780635923));
#54378=CARTESIAN_POINT('Ctrl Pts',(-74.1361639292525,10.5215667293953,0.444845719375119));
#54379=CARTESIAN_POINT('Ctrl Pts',(-74.15142479311,10.5348939807602,0.440262869550269));
#54380=CARTESIAN_POINT('Ctrl Pts',(-74.2209214739893,10.5955851541924,0.419392959775233));
#54381=CARTESIAN_POINT('Ctrl Pts',(-74.2910599577422,10.6571271073302,0.397761489779669));
#54382=CARTESIAN_POINT('Ctrl Pts',(-74.3618601395729,10.7194002313636,0.375310769785536));
#54383=CARTESIAN_POINT('Ctrl Pts',(-74.4443416020322,10.7919477617423,0.34915591861849));
#54384=CARTESIAN_POINT('Ctrl Pts',(-74.5278728361943,10.8653701096654,0.321829534180452));
#54385=CARTESIAN_POINT('Ctrl Pts',(-74.6124874497988,10.9396747980141,0.29321819202761));
#54386=CARTESIAN_POINT('Ctrl Pts',(-74.6981797801607,11.0149258879875,0.264242433829161));
#54387=CARTESIAN_POINT('Ctrl Pts',(-74.7836188958127,11.0899283290314,0.234411023652205));
#54388=CARTESIAN_POINT('Ctrl Pts',(-74.8688498737947,11.164552430703,0.203648851738809));
#54389=CARTESIAN_POINT('Ctrl Pts',(-74.905368038679,11.1965259609111,0.190468455447126));
#54390=CARTESIAN_POINT('Ctrl Pts',(-74.9418483580553,11.2284304875774,0.177116693959281));
#54391=CARTESIAN_POINT('Ctrl Pts',(-74.9782954785082,11.2602569521105,0.163585454925456));
#54392=CARTESIAN_POINT('Ctrl Pts',(-75.0074345983226,11.2857019022679,0.15276736036695));
#54393=CARTESIAN_POINT('Ctrl Pts',(-75.0365610563992,11.3111070185523,0.141831372080102));
#54394=CARTESIAN_POINT('Ctrl Pts',(-75.0656646015123,11.3364528632712,0.130777364319412));
#54395=CARTESIAN_POINT('Ctrl Pts',(-75.1693891430163,11.4267850242597,0.0913810680159116));
#54396=CARTESIAN_POINT('Ctrl Pts',(-75.2728226806968,11.5163646344423,0.0504861477426313));
#54397=CARTESIAN_POINT('Ctrl Pts',(-75.3762211738556,11.6050891055634,0.00797700848348162));
#54398=CARTESIAN_POINT('Ctrl Pts',(-75.5209764363984,11.7293011101946,-0.0515347061067087));
#54399=CARTESIAN_POINT('Ctrl Pts',(-75.6656005855099,11.8517654908376,-0.114186880414224));
#54400=CARTESIAN_POINT('Ctrl Pts',(-75.8105815039629,11.9720103355759,-0.180199616753054));
#54401=CARTESIAN_POINT('Ctrl Pts',(-75.8688769667546,12.0203596559357,-0.206742716742249));
#54402=CARTESIAN_POINT('Ctrl Pts',(-75.9272301710115,12.0683429779132,-0.233828803928773));
#54403=CARTESIAN_POINT('Ctrl Pts',(-75.9856730522913,12.1159454171049,-0.261471969112078));
#54404=CARTESIAN_POINT('Ctrl Pts',(-76.0738442188497,12.1877619070289,-0.303176451646275));
#54405=CARTESIAN_POINT('Ctrl Pts',(-76.1622194677579,12.2587114608792,-0.346148840494859));
#54406=CARTESIAN_POINT('Ctrl Pts',(-76.2508921194158,12.3286689947587,-0.390466393683425));
#54407=CARTESIAN_POINT('Ctrl Pts',(-76.3045126820762,12.3709724813333,-0.417265323153464));
#54408=CARTESIAN_POINT('Ctrl Pts',(-76.3582418720366,12.412917464529,-0.444556260698553));
#54409=CARTESIAN_POINT('Ctrl Pts',(-76.4120993155164,12.4544814707452,-0.472356374618462));
#54410=CARTESIAN_POINT('Ctrl Pts',(-76.4246540554797,12.4641704804003,-0.478836875337829));
#54411=CARTESIAN_POINT('Ctrl Pts',(-76.4372157038024,12.4738388656321,-0.485345020926855));
#54412=CARTESIAN_POINT('Ctrl Pts',(-76.4497845907488,12.4834862511291,-0.491881065292419));
#54413=CARTESIAN_POINT('Ctrl Pts',(-76.5663072516948,12.5729244833353,-0.552474917777949));
#54414=CARTESIAN_POINT('Ctrl Pts',(-76.6834519541958,12.6605584945839,-0.615466015597185));
#54415=CARTESIAN_POINT('Ctrl Pts',(-76.8014105707122,12.7461545044742,-0.681003990962555));
#54416=CARTESIAN_POINT('Ctrl Pts',(-76.9250297873023,12.8358580971271,-0.749687003792275));
#54417=CARTESIAN_POINT('Ctrl Pts',(-77.0495441480684,12.9233233001143,-0.821168132964172));
#54418=CARTESIAN_POINT('Ctrl Pts',(-77.1751446629466,13.0082520782237,-0.895608320462843));
#54419=CARTESIAN_POINT('Ctrl Pts',(-77.2934431354488,13.0882433484153,-0.965720775673853));
#54420=CARTESIAN_POINT('Ctrl Pts',(-77.4127053358055,13.1659845002992,-1.03845878994031));
#54421=CARTESIAN_POINT('Ctrl Pts',(-77.5330572832168,13.2411990194525,-1.11393705810681));
#54422=CARTESIAN_POINT('Ctrl Pts',(-77.6092830790908,13.288836691356,-1.16174177739831));
#54423=CARTESIAN_POINT('Ctrl Pts',(-77.6859470912346,13.3354581966371,-1.21064851708965));
#54424=CARTESIAN_POINT('Ctrl Pts',(-77.7627810117474,13.3808245309148,-1.26048464802789));
#54425=CARTESIAN_POINT('Ctrl Pts',(-77.805172502908,13.4058544466824,-1.28798067959899));
#54426=CARTESIAN_POINT('Ctrl Pts',(-77.8476154631687,13.4305028627614,-1.31575900541072));
#54427=CARTESIAN_POINT('Ctrl Pts',(-77.8900628058563,13.4547342196409,-1.34378595877275));
#54428=CARTESIAN_POINT('',(-66.3007096452781,7.3256579779933,6.6269806053999));
#54429=CARTESIAN_POINT('Ctrl Pts',(-66.3007095462964,7.32565791266264,6.62698056598248));
#54430=CARTESIAN_POINT('Ctrl Pts',(-66.3009135695284,7.3256802261172,6.62643125788398));
#54431=CARTESIAN_POINT('Ctrl Pts',(-66.3011176225372,7.32570254169686,6.62588191975181));
#54432=CARTESIAN_POINT('Ctrl Pts',(-66.3013217053874,7.32572485941033,6.62533255152024));
#54433=CARTESIAN_POINT('Ctrl Pts',(-66.3194179281466,7.32770379254521,6.57661954164251));
#54434=CARTESIAN_POINT('Ctrl Pts',(-66.3378230918283,7.32965372278552,6.52699894618457));
#54435=CARTESIAN_POINT('Ctrl Pts',(-66.3565849496956,7.33157745912018,6.47668360260689));
#54436=CARTESIAN_POINT('Ctrl Pts',(-66.374078920144,7.33337119334559,6.42976846553077));
#54437=CARTESIAN_POINT('Ctrl Pts',(-66.3918830071351,7.33514214755358,6.38224911349161));
#54438=CARTESIAN_POINT('Ctrl Pts',(-66.410035606402,7.3368925923503,6.3343426080647));
#54439=CARTESIAN_POINT('Ctrl Pts',(-66.4217701751073,7.33802415011952,6.30337392026969));
#54440=CARTESIAN_POINT('Ctrl Pts',(-66.4336503754913,7.33914713718827,6.27224433285713));
#54441=CARTESIAN_POINT('Ctrl Pts',(-66.4456864922457,7.34026218757265,6.24102425000606));
#54442=CARTESIAN_POINT('Ctrl Pts',(-66.4747433527868,7.34295407434778,6.16565462606573));
#54443=CARTESIAN_POINT('Ctrl Pts',(-66.5047091948074,7.34559978471336,6.08976624501636));
#54444=CARTESIAN_POINT('Ctrl Pts',(-66.5357273196607,7.34820719314405,6.01308254286435));
#54445=CARTESIAN_POINT('Ctrl Pts',(-66.5568756309281,7.3499849371358,5.96079921465153));
#54446=CARTESIAN_POINT('Ctrl Pts',(-66.578513037914,7.35174485098548,5.90814543700593));
#54447=CARTESIAN_POINT('Ctrl Pts',(-66.6006836819377,7.35348934292209,5.85501943010007));
#54448=CARTESIAN_POINT('Ctrl Pts',(-66.6428593479286,7.35680792533058,5.75395674918312));
#54449=CARTESIAN_POINT('Ctrl Pts',(-66.686966030636,7.36007054666283,5.65117826481152));
#54450=CARTESIAN_POINT('Ctrl Pts',(-66.7332927314322,7.3632907199729,5.54643924423697));
#54451=CARTESIAN_POINT('Ctrl Pts',(-66.7810584598513,7.36661092022778,5.43844675770848));
#54452=CARTESIAN_POINT('Ctrl Pts',(-66.8310605834434,7.36988089902069,5.32897366717206));
#54453=CARTESIAN_POINT('Ctrl Pts',(-66.883383161277,7.37312728448175,5.21861412315586));
#54454=CARTESIAN_POINT('Ctrl Pts',(-66.9042716248249,7.3744233216262,5.17455587129235));
#54455=CARTESIAN_POINT('Ctrl Pts',(-66.9255296182242,7.37571585460846,5.13035673764271));
#54456=CARTESIAN_POINT('Ctrl Pts',(-66.9471612143753,7.37700769457503,5.08605616894808));
#54457=CARTESIAN_POINT('Ctrl Pts',(-67.0020202838865,7.38028388085499,4.97370717905229));
#54458=CARTESIAN_POINT('Ctrl Pts',(-67.0592848107264,7.3835531223658,4.86070546692605));
#54459=CARTESIAN_POINT('Ctrl Pts',(-67.1189977790173,7.38688847113522,4.74763793427717));
#54460=CARTESIAN_POINT('Ctrl Pts',(-67.1763135110444,7.39008991902428,4.63910960973153));
#54461=CARTESIAN_POINT('Ctrl Pts',(-67.2358851065306,7.39335216145908,4.53052082135333));
#54462=CARTESIAN_POINT('Ctrl Pts',(-67.297716666954,7.39677274401974,4.42239841323215));
#54463=CARTESIAN_POINT('Ctrl Pts',(-67.3585623242391,7.40013878545192,4.31600001499786));
#54464=CARTESIAN_POINT('Ctrl Pts',(-67.4215966129306,7.40365803772726,4.21005340898495));
#54465=CARTESIAN_POINT('Ctrl Pts',(-67.4867880504236,7.40745792272589,4.10506590900433));
#54466=CARTESIAN_POINT('Ctrl Pts',(-67.5511198678568,7.41120770210489,4.00146278348265));
#54467=CARTESIAN_POINT('Ctrl Pts',(-67.6175524583477,7.41523077998971,3.89879381993956));
#54468=CARTESIAN_POINT('Ctrl Pts',(-67.6860185912183,7.41968423904816,3.79754912249489));
#54469=CARTESIAN_POINT('Ctrl Pts',(-67.7359642288322,7.42293301100205,3.72369171655007));
#54470=CARTESIAN_POINT('Ctrl Pts',(-67.7869912854423,7.42641156134627,3.65059231891243));
#54471=CARTESIAN_POINT('Ctrl Pts',(-67.8390603750945,7.43019232082122,3.57844119038534));
#54472=CARTESIAN_POINT('Ctrl Pts',(-67.8857580036338,7.43358305614492,3.51373319143344));
#54473=CARTESIAN_POINT('Ctrl Pts',(-67.9332935903729,7.43721706882084,3.44978792357554));
#54474=CARTESIAN_POINT('Ctrl Pts',(-67.9816311052487,7.44114802956374,3.3867439779933));
#54475=CARTESIAN_POINT('Ctrl Pts',(-68.0194296228557,7.44422192546497,3.33744546330498));
#54476=CARTESIAN_POINT('Ctrl Pts',(-68.0577180817216,7.44747752520659,3.28869812900676));
#54477=CARTESIAN_POINT('Ctrl Pts',(-68.0964849977637,7.45094195228621,3.24056752849838));
#54478=CARTESIAN_POINT('Ctrl Pts',(-68.167468735921,7.45728545364744,3.15243851818121));
#54479=CARTESIAN_POINT('Ctrl Pts',(-68.240236923429,7.46434767010371,3.06631689289534));
#54480=CARTESIAN_POINT('Ctrl Pts',(-68.3143503194014,7.47226730576452,2.98259175686538));
#54481=CARTESIAN_POINT('Ctrl Pts',(-68.3809814871828,7.47938740282066,2.90731921654876));
#54482=CARTESIAN_POINT('Ctrl Pts',(-68.4486998362414,7.48720099887561,2.83398386620116));
#54483=CARTESIAN_POINT('Ctrl Pts',(-68.5172226611057,7.49581109283069,2.76284316012924));
#54484=CARTESIAN_POINT('Ctrl Pts',(-68.5837159569218,7.50416617050726,2.69380952027606));
#54485=CARTESIAN_POINT('Ctrl Pts',(-68.6509665695429,7.51327156880274,2.62684268767755));
#54486=CARTESIAN_POINT('Ctrl Pts',(-68.7187552419876,7.5232183054159,2.56214960643483));
#54487=CARTESIAN_POINT('Ctrl Pts',(-68.7852864741979,7.53298053588124,2.4986565440199));
#54488=CARTESIAN_POINT('Ctrl Pts',(-68.8523359727839,7.54355343171551,2.43735377662181));
#54489=CARTESIAN_POINT('Ctrl Pts',(-68.9197363662121,7.55501595279508,2.37840660705263));
#54490=CARTESIAN_POINT('Ctrl Pts',(-68.949043521386,7.56000010595616,2.3527750972386));
#54491=CARTESIAN_POINT('Ctrl Pts',(-68.9784175370779,7.56515234688882,2.32758855806634));
#54492=CARTESIAN_POINT('Ctrl Pts',(-69.0078470239477,7.57047856294424,2.30285869971681));
#54493=CARTESIAN_POINT('Ctrl Pts',(-69.0811794028085,7.58375042512104,2.24123685256458));
#54494=CARTESIAN_POINT('Ctrl Pts',(-69.154831024795,7.59809903352262,2.18246657147294));
#54495=CARTESIAN_POINT('Ctrl Pts',(-69.2286605473917,7.6136124418366,2.1264662081964));
#54496=CARTESIAN_POINT('Ctrl Pts',(-69.3059090789679,7.62984426848056,2.06787249556368));
#54497=CARTESIAN_POINT('Ctrl Pts',(-69.3833525322979,7.64735154983253,2.0123112110714));
#54498=CARTESIAN_POINT('Ctrl Pts',(-69.4608738698136,7.66622374537447,1.95965407767665));
#54499=CARTESIAN_POINT('Ctrl Pts',(-69.5449564724437,7.68669324924739,1.90254014021424));
#54500=CARTESIAN_POINT('Ctrl Pts',(-69.629130994274,7.70876903418113,1.8488426881589));
#54501=CARTESIAN_POINT('Ctrl Pts',(-69.7132966457926,7.73254554360505,1.79835787559971));
#54502=CARTESIAN_POINT('Ctrl Pts',(-69.7971367364602,7.75623008319924,1.74806834316057));
#54503=CARTESIAN_POINT('Ctrl Pts',(-69.880969193409,7.78160254817844,1.70096571478774));
#54504=CARTESIAN_POINT('Ctrl Pts',(-69.9647281914062,7.80873119754363,1.65681886174829));
#54505=CARTESIAN_POINT('Ctrl Pts',(-70.0380592877499,7.83248236037801,1.61816824257998));
#54506=CARTESIAN_POINT('Ctrl Pts',(-70.1112816378291,7.85755983506915,1.58186156351898));
#54507=CARTESIAN_POINT('Ctrl Pts',(-70.1841143970553,7.8839044258334,1.54766345052146));
#54508=CARTESIAN_POINT('Ctrl Pts',(-70.241950136846,7.9048243925149,1.52050708317151));
#54509=CARTESIAN_POINT('Ctrl Pts',(-70.2995407757624,7.9265426198367,1.49468000367399));
#54510=CARTESIAN_POINT('Ctrl Pts',(-70.3567496590864,7.94900631970774,1.47006601912511));
#54511=CARTESIAN_POINT('Ctrl Pts',(-70.4224156098662,7.97479078051802,1.44181340162984));
#54512=CARTESIAN_POINT('Ctrl Pts',(-70.4875795354592,8.00155856095457,1.41515741744729));
#54513=CARTESIAN_POINT('Ctrl Pts',(-70.5520542732033,8.02916527010112,1.38994245160169));
#54514=CARTESIAN_POINT('Ctrl Pts',(-70.6158157737203,8.05646658626165,1.36500642062193));
#54515=CARTESIAN_POINT('Ctrl Pts',(-70.6789036055966,8.08458833367319,1.34147963066587));
#54516=CARTESIAN_POINT('Ctrl Pts',(-70.7411232251305,8.11334882868581,1.31923720824191));
#54517=CARTESIAN_POINT('Ctrl Pts',(-70.7928520977186,8.1372600642932,1.30074504380507));
#54518=CARTESIAN_POINT('Ctrl Pts',(-70.8439806675348,8.16161202433244,1.28314112432323));
#54519=CARTESIAN_POINT('Ctrl Pts',(-70.8943876832028,8.18627849626928,1.26636748743511));
#54520=CARTESIAN_POINT('Ctrl Pts',(-70.9685642174178,8.22257648724013,1.24168421202093));
#54521=CARTESIAN_POINT('Ctrl Pts',(-71.0412299653039,8.25958269162281,1.21873568845334));
#54522=CARTESIAN_POINT('Ctrl Pts',(-71.1125632075137,8.29718424520714,1.19715207673234));
#54523=CARTESIAN_POINT('Ctrl Pts',(-71.1877147737129,8.33679853380312,1.17441313798763));
#54524=CARTESIAN_POINT('Ctrl Pts',(-71.2613866892902,8.37707311139465,1.153190021763));
#54525=CARTESIAN_POINT('Ctrl Pts',(-71.3337438157902,8.41790617984398,1.13308174347315));
#54526=CARTESIAN_POINT('Ctrl Pts',(-71.4105556377512,8.46125315249983,1.11173549098008));
#54527=CARTESIAN_POINT('Ctrl Pts',(-71.4858851171286,8.50522892886088,1.09164653976952));
#54528=CARTESIAN_POINT('Ctrl Pts',(-71.5598924747369,8.54975360065063,1.07235492453254));
#54529=CARTESIAN_POINT('Ctrl Pts',(-71.6070899451594,8.57814877577616,1.06005188509195));
#54530=CARTESIAN_POINT('Ctrl Pts',(-71.6537489985828,8.60676808056893,1.04807346027955));
#54531=CARTESIAN_POINT('Ctrl Pts',(-71.6999058441912,8.63560026715401,1.03630157777965));
#54532=CARTESIAN_POINT('Ctrl Pts',(-71.704120708006,8.63823311041569,1.03522661520525));
#54533=CARTESIAN_POINT('Ctrl Pts',(-71.708331426215,8.64086748855088,1.03415473800599));
#54534=CARTESIAN_POINT('Ctrl Pts',(-71.7125380276667,8.6435033979355,1.03308584761069));
#54535=CARTESIAN_POINT('',(-63.8800558890744,6.98826998322039,12.652871638431));
#54536=CARTESIAN_POINT('Ctrl Pts',(-63.8800459600055,6.98833961342996,12.652871806017));
#54537=CARTESIAN_POINT('Ctrl Pts',(-63.8800561878002,6.98834112621968,12.6528492302221));
#54538=CARTESIAN_POINT('Ctrl Pts',(-63.8800664155777,6.98834263900889,12.6528266544218));
#54539=CARTESIAN_POINT('Ctrl Pts',(-63.880076643338,6.98834415179758,12.6528040786163));
#54540=CARTESIAN_POINT('Ctrl Pts',(-63.9572793151289,6.99976320410498,12.4823940898988));
#54541=CARTESIAN_POINT('Ctrl Pts',(-64.0340116487795,7.01124392269474,12.3117675918103));
#54542=CARTESIAN_POINT('Ctrl Pts',(-64.1102406561908,7.02272416958815,12.1407419422998));
#54543=CARTESIAN_POINT('Ctrl Pts',(-64.1453347460234,7.02800941243021,12.0620056487097));
#54544=CARTESIAN_POINT('Ctrl Pts',(-64.1803219866163,7.03329450837554,11.9831849600398));
#54545=CARTESIAN_POINT('Ctrl Pts',(-64.2151980126629,7.03857457831673,11.904262701183));
#54546=CARTESIAN_POINT('Ctrl Pts',(-64.3118605224935,7.05320883773364,11.6855215059444));
#54547=CARTESIAN_POINT('Ctrl Pts',(-64.4076718527601,7.0678064597728,11.4660006269974));
#54548=CARTESIAN_POINT('Ctrl Pts',(-64.5025055426427,7.08225064094446,11.2455495972412));
#54549=CARTESIAN_POINT('Ctrl Pts',(-64.5155997988649,7.08424503565182,11.2151106016516));
#54550=CARTESIAN_POINT('Ctrl Pts',(-64.5286753465173,7.0862364629838,11.1846538725359));
#54551=CARTESIAN_POINT('Ctrl Pts',(-64.5417317838301,7.0882245749091,11.1541790127706));
#54552=CARTESIAN_POINT('Ctrl Pts',(-64.6301515191858,7.1016883036492,10.9477996635737));
#54553=CARTESIAN_POINT('Ctrl Pts',(-64.7176988502198,7.11500064672635,10.740587896499));
#54554=CARTESIAN_POINT('Ctrl Pts',(-64.8042231407219,7.12804626582424,10.5324087104427));
#54555=CARTESIAN_POINT('Ctrl Pts',(-64.8363675374695,7.13289280722514,10.4550686442905));
#54556=CARTESIAN_POINT('Ctrl Pts',(-64.8683702418261,7.13770246224527,10.3775951715722));
#54557=CARTESIAN_POINT('Ctrl Pts',(-64.9002217457112,7.14246913199823,10.299981827171));
#54558=CARTESIAN_POINT('Ctrl Pts',(-64.9478661518172,7.1495992552823,10.1838855287595));
#54559=CARTESIAN_POINT('Ctrl Pts',(-64.9951724628551,7.15663301464725,10.0674761822453));
#54560=CARTESIAN_POINT('Ctrl Pts',(-65.0421056966384,7.16354976945968,9.95073637091178));
#54561=CARTESIAN_POINT('Ctrl Pts',(-65.0825059421805,7.16950372937786,9.85024644805254));
#54562=CARTESIAN_POINT('Ctrl Pts',(-65.1226458394789,7.17537320271517,9.7495018816085));
#54563=CARTESIAN_POINT('Ctrl Pts',(-65.1624544957306,7.18113925044134,9.64878744287005));
#54564=CARTESIAN_POINT('Ctrl Pts',(-65.2419384276758,7.19265202651099,9.44769601330832));
#54565=CARTESIAN_POINT('Ctrl Pts',(-65.3201024156781,7.20374940290162,9.24672378317048));
#54566=CARTESIAN_POINT('Ctrl Pts',(-65.3963637810109,7.2143106093483,9.04815217590113));
#54567=CARTESIAN_POINT('Ctrl Pts',(-65.468296331599,7.2242723312986,8.86085206498778));
#54568=CARTESIAN_POINT('Ctrl Pts',(-65.5385340583308,7.23375700647539,8.67568850949559));
#54569=CARTESIAN_POINT('Ctrl Pts',(-65.6065923143366,7.24270648257226,8.49458419430487));
#54570=CARTESIAN_POINT('Ctrl Pts',(-65.6502509006398,7.24844746827295,8.37840786480911));
#54571=CARTESIAN_POINT('Ctrl Pts',(-65.6930128012289,7.25396914188262,8.26390206970707));
#54572=CARTESIAN_POINT('Ctrl Pts',(-65.7347567854724,7.25926556663905,8.15157432823398));
#54573=CARTESIAN_POINT('Ctrl Pts',(-65.7364420781083,7.25947939447078,8.14703942053546));
#54574=CARTESIAN_POINT('Ctrl Pts',(-65.7381257216343,7.25969285723204,8.14250805592864));
#54575=CARTESIAN_POINT('Ctrl Pts',(-65.739807721741,7.25990595645158,8.13798023872227));
#54576=CARTESIAN_POINT('Ctrl Pts',(-65.8100377537922,7.26880367587444,7.94892629855544));
#54577=CARTESIAN_POINT('Ctrl Pts',(-65.8773985543478,7.27706623739923,7.76605796002971));
#54578=CARTESIAN_POINT('Ctrl Pts',(-65.9423265821899,7.28481922328194,7.58967481592044));
#54579=CARTESIAN_POINT('Ctrl Pts',(-66.0095897680272,7.29285104786611,7.40694799369743));
#54580=CARTESIAN_POINT('Ctrl Pts',(-66.0742418673935,7.30033681706775,7.23118091907675));
#54581=CARTESIAN_POINT('Ctrl Pts',(-66.1368236734351,7.30742582948383,7.06269520960938));
#54582=CARTESIAN_POINT('Ctrl Pts',(-66.1929759980861,7.31378653640203,6.91151925519911));
#54583=CARTESIAN_POINT('Ctrl Pts',(-66.2474625884719,7.31982822145605,6.76620507781348));
#54584=CARTESIAN_POINT('Ctrl Pts',(-66.3007095158743,7.32565790933545,6.62698064789046));
#54585=CARTESIAN_POINT('',(-60.9536795918073,6.58767285120433,18.6650422826135));
#54586=CARTESIAN_POINT('Ctrl Pts',(-60.9536795918073,6.58767285120433,18.6650422826135));
#54587=CARTESIAN_POINT('Ctrl Pts',(-61.1064136681965,6.60882453290174,18.397171129156));
#54588=CARTESIAN_POINT('Ctrl Pts',(-61.4026533876799,6.64953999991258,17.8502351016645));
#54589=CARTESIAN_POINT('Ctrl Pts',(-61.8813511258638,6.71394676359331,16.8972049262099));
#54590=CARTESIAN_POINT('Ctrl Pts',(-62.313674056402,6.7713543457067,16.0028732107663));
#54591=CARTESIAN_POINT('Ctrl Pts',(-62.7048717197328,6.82345654645031,15.1819379428255));
#54592=CARTESIAN_POINT('Ctrl Pts',(-63.2386855526803,6.89569253577236,14.0502307887768));
#54593=CARTESIAN_POINT('Ctrl Pts',(-63.6251462417326,6.95055614069076,13.2159876874408));
#54594=CARTESIAN_POINT('Ctrl Pts',(-63.88006477921,6.98820763880422,12.6528714883805));
#54595=CARTESIAN_POINT('',(-48.943686428043,5.01441858224854,24.6839747939812));
#54596=CARTESIAN_POINT('Ctrl Pts',(-48.943686427953,5.01441858311083,24.6839747939811));
#54597=CARTESIAN_POINT('Ctrl Pts',(-48.9436933030855,5.01441930127938,24.6839740301331));
#54598=CARTESIAN_POINT('Ctrl Pts',(-48.9437001782249,5.01442001944909,24.6839732662801));
#54599=CARTESIAN_POINT('Ctrl Pts',(-48.9437070533713,5.01442073761994,24.6839725024221));
#54600=CARTESIAN_POINT('Ctrl Pts',(-49.2104058457392,5.04227982433237,24.6543411359102));
#54601=CARTESIAN_POINT('Ctrl Pts',(-49.4876048491357,5.0718742454339,24.6172984586111));
#54602=CARTESIAN_POINT('Ctrl Pts',(-49.7724012808886,5.10302368190886,24.5737464914054));
#54603=CARTESIAN_POINT('Ctrl Pts',(-50.0079486615118,5.12878653337579,24.5377258441904));
#54604=CARTESIAN_POINT('Ctrl Pts',(-50.2486931821281,5.15561239316509,24.4972525288513));
#54605=CARTESIAN_POINT('Ctrl Pts',(-50.4929944974496,5.18337221375705,24.4528377619485));
#54606=CARTESIAN_POINT('Ctrl Pts',(-50.7766538286848,5.21560426348613,24.4012675808382));
#54607=CARTESIAN_POINT('Ctrl Pts',(-51.0651079819501,5.24909696850875,24.3443836308993));
#54608=CARTESIAN_POINT('Ctrl Pts',(-51.3558112857037,5.28357192459843,24.2829878673439));
#54609=CARTESIAN_POINT('Ctrl Pts',(-51.6520246136125,5.31870032300662,24.220428401361));
#54610=CARTESIAN_POINT('Ctrl Pts',(-51.9505734679519,5.35484840513919,24.1531844876066));
#54611=CARTESIAN_POINT('Ctrl Pts',(-52.2487678361982,5.39166710815415,24.0821063528286));
#54612=CARTESIAN_POINT('Ctrl Pts',(-52.55816891618,5.42986952808365,24.0083569665047));
#54613=CARTESIAN_POINT('Ctrl Pts',(-52.867188802127,5.46879371681604,23.9304798136703));
#54614=CARTESIAN_POINT('Ctrl Pts',(-53.172820278291,5.50799417252183,23.8494259008386));
#54615=CARTESIAN_POINT('Ctrl Pts',(-53.2063458833143,5.51229418445523,23.8405348615343));
#54616=CARTESIAN_POINT('Ctrl Pts',(-53.2398307108533,5.51659746965907,23.8316055983123));
#54617=CARTESIAN_POINT('Ctrl Pts',(-53.273270786351,5.52090340344408,23.822639366649));
#54618=CARTESIAN_POINT('Ctrl Pts',(-53.4433076524457,5.54279831472997,23.7770476653738));
#54619=CARTESIAN_POINT('Ctrl Pts',(-53.6121875240046,5.56476198960391,23.7305001411357));
#54620=CARTESIAN_POINT('Ctrl Pts',(-53.7793893479847,5.58669844287257,23.6831595754526));
#54621=CARTESIAN_POINT('Ctrl Pts',(-54.093173328354,5.62786610156178,23.5943165785321));
#54622=CARTESIAN_POINT('Ctrl Pts',(-54.4010372363093,5.6689398394008,23.5026837491855));
#54623=CARTESIAN_POINT('Ctrl Pts',(-54.6974294149276,5.70897076501432,23.4097505788098));
#54624=CARTESIAN_POINT('Ctrl Pts',(-54.9414822833493,5.74193270843367,23.3332282936825));
#54625=CARTESIAN_POINT('Ctrl Pts',(-55.1777570043168,5.77418559781669,23.2558242895775));
#54626=CARTESIAN_POINT('Ctrl Pts',(-55.4031331947367,5.80518387641173,23.1783707257999));
#54627=CARTESIAN_POINT('Ctrl Pts',(-55.6070057675119,5.83322454387087,23.1083071698912));
#54628=CARTESIAN_POINT('Ctrl Pts',(-55.8019601413752,5.86023797808104,23.0382030434586));
#54629=CARTESIAN_POINT('Ctrl Pts',(-55.9856699657615,5.88582111046705,22.9686751793201));
#54630=CARTESIAN_POINT('Ctrl Pts',(-56.0107942755779,5.88931988113044,22.9591664902485));
#54631=CARTESIAN_POINT('Ctrl Pts',(-56.0357087956219,5.89279198396761,22.949668578276));
#54632=CARTESIAN_POINT('Ctrl Pts',(-56.0604194770111,5.89623806282833,22.9401792214321));
#54633=CARTESIAN_POINT('Ctrl Pts',(-56.2634514356021,5.92455230190299,22.8622112093225));
#54634=CARTESIAN_POINT('Ctrl Pts',(-56.4527203540863,5.95110528147132,22.7848206242314));
#54635=CARTESIAN_POINT('Ctrl Pts',(-56.6315152700827,5.97627685995714,22.706775556212));
#54636=CARTESIAN_POINT('Ctrl Pts',(-56.8341077358789,6.00479876800473,22.6183427130007));
#54637=CARTESIAN_POINT('Ctrl Pts',(-57.0232522057511,6.03154794669356,22.529069618797));
#54638=CARTESIAN_POINT('Ctrl Pts',(-57.2037695117562,6.0571386150431,22.4371655163732));
#54639=CARTESIAN_POINT('Ctrl Pts',(-57.3334050691406,6.07551613589554,22.3711660850317));
#54640=CARTESIAN_POINT('Ctrl Pts',(-57.4585922263825,6.09329753291716,22.3038098301435));
#54641=CARTESIAN_POINT('Ctrl Pts',(-57.5811269320388,6.11072246502127,22.2344337090417));
#54642=CARTESIAN_POINT('Ctrl Pts',(-57.7960199612812,6.14128112531378,22.1127665883611));
#54643=CARTESIAN_POINT('Ctrl Pts',(-58.002734874994,6.17074052332906,21.9848890384924));
#54644=CARTESIAN_POINT('Ctrl Pts',(-58.2027480597424,6.19925187141741,21.8478966424791));
#54645=CARTESIAN_POINT('Ctrl Pts',(-58.2856305930849,6.21106655634201,21.7911290006634));
#54646=CARTESIAN_POINT('Ctrl Pts',(-58.3673628401942,6.22271872520401,21.7327962746785));
#54647=CARTESIAN_POINT('Ctrl Pts',(-58.4480523143857,6.23422017683554,21.6726921818843));
#54648=CARTESIAN_POINT('Ctrl Pts',(-58.5904224605179,6.25451357155549,21.5666433005403));
#54649=CARTESIAN_POINT('Ctrl Pts',(-58.7295450374508,6.27433754426476,21.4550796143134));
#54650=CARTESIAN_POINT('Ctrl Pts',(-58.866025069094,6.29376041498173,21.3368706761723));
#54651=CARTESIAN_POINT('Ctrl Pts',(-58.8669089202096,6.29388619840766,21.3361051495191));
#54652=CARTESIAN_POINT('Ctrl Pts',(-58.8677926605737,6.29401196502538,21.335339344183));
#54653=CARTESIAN_POINT('Ctrl Pts',(-58.8686762903519,6.29413771485699,21.3345732598584));
#54654=CARTESIAN_POINT('Ctrl Pts',(-59.0693160286427,6.32269086451823,21.1606237595298));
#54655=CARTESIAN_POINT('Ctrl Pts',(-59.2642396750474,6.35037577232071,20.9722889479987));
#54656=CARTESIAN_POINT('Ctrl Pts',(-59.4520298320428,6.37697681306191,20.7716602375005));
#54657=CARTESIAN_POINT('Ctrl Pts',(-59.6398199890382,6.40357785380311,20.5710315270023));
#54658=CARTESIAN_POINT('Ctrl Pts',(-59.8204767928905,6.42909479775789,20.3581090997196));
#54659=CARTESIAN_POINT('Ctrl Pts',(-59.9926310538925,6.45333012417932,20.134997670789));
#54660=CARTESIAN_POINT('Ctrl Pts',(-60.1295309743094,6.47260245725467,19.9575757662313));
#54661=CARTESIAN_POINT('Ctrl Pts',(-60.2610708473564,6.49106748603937,19.773713601681));
#54662=CARTESIAN_POINT('Ctrl Pts',(-60.3891143826253,6.50898792976107,19.5828383420744));
#54663=CARTESIAN_POINT('Ctrl Pts',(-60.5104434499889,6.52596864431983,19.4019723797108));
#54664=CARTESIAN_POINT('Ctrl Pts',(-60.6286331300441,6.54246035334563,19.2148094425513));
#54665=CARTESIAN_POINT('Ctrl Pts',(-60.7453139889917,6.55869185993184,19.020871129382));
#54666=CARTESIAN_POINT('Ctrl Pts',(-60.8151920342546,6.56841261415106,18.9047249992618));
#54667=CARTESIAN_POINT('Ctrl Pts',(-60.8845297938964,6.57804014476984,18.7861489951842));
#54668=CARTESIAN_POINT('Ctrl Pts',(-60.9536863008776,6.58762473125413,18.665042306171));
#54669=CARTESIAN_POINT('',(-43.998256547978,4.57019747403691,24.6840336608423));
#54670=CARTESIAN_POINT('Ctrl Pts',(-43.9982565479099,4.57019747493893,24.6840336608423));
#54671=CARTESIAN_POINT('Ctrl Pts',(-44.7983004349469,4.63056911424585,24.7634007046597));
#54672=CARTESIAN_POINT('Ctrl Pts',(-45.6065458290174,4.69707310585867,24.8079761534353));
#54673=CARTESIAN_POINT('Ctrl Pts',(-47.2553606707774,4.84445121892603,24.8169837372541));
#54674=CARTESIAN_POINT('Ctrl Pts',(-48.1045754985842,4.92676600513598,24.7772030223014));
#54675=CARTESIAN_POINT('Ctrl Pts',(-48.943686427953,5.01441858311083,24.6839747939812));
#54676=CARTESIAN_POINT('',(-30.3134449265951,4.07585591331178,18.6659931355377));
#54677=CARTESIAN_POINT('Ctrl Pts',(-30.3134449302137,4.07585425011609,18.665993135544));
#54678=CARTESIAN_POINT('Ctrl Pts',(-30.5181570460434,4.07629984775709,18.8492527201676));
#54679=CARTESIAN_POINT('Ctrl Pts',(-30.7306280520902,4.07692382601424,19.032878104075));
#54680=CARTESIAN_POINT('Ctrl Pts',(-30.9534488453249,4.07782080148265,19.2181909065929));
#54681=CARTESIAN_POINT('Ctrl Pts',(-31.1681448217793,4.07868507012316,19.396746563399));
#54682=CARTESIAN_POINT('Ctrl Pts',(-31.3924496744848,4.07980188235618,19.5768689665312));
#54683=CARTESIAN_POINT('Ctrl Pts',(-31.6286796916658,4.08130139885299,19.7597442125536));
#54684=CARTESIAN_POINT('Ctrl Pts',(-31.7324682166588,4.08196021692897,19.8400911230304));
#54685=CARTESIAN_POINT('Ctrl Pts',(-31.8385587306746,4.08269424598024,19.920968736235));
#54686=CARTESIAN_POINT('Ctrl Pts',(-31.945633483405,4.08350482910259,20.0014046313493));
#54687=CARTESIAN_POINT('Ctrl Pts',(-32.0868798312397,4.08457409989452,20.1075106566261));
#54688=CARTESIAN_POINT('Ctrl Pts',(-32.2298388402814,4.08577749941939,20.2128481180817));
#54689=CARTESIAN_POINT('Ctrl Pts',(-32.3714856621259,4.08709818275659,20.31518127585));
#54690=CARTESIAN_POINT('Ctrl Pts',(-32.6205108244127,4.08942003776253,20.4950902274858));
#54691=CARTESIAN_POINT('Ctrl Pts',(-32.8654802639302,4.09209932738748,20.6657155719101));
#54692=CARTESIAN_POINT('Ctrl Pts',(-33.1064729800666,4.0951370942871,20.8281355915901));
#54693=CARTESIAN_POINT('Ctrl Pts',(-33.3420167258229,4.09810617570061,20.9868832103339));
#54694=CARTESIAN_POINT('Ctrl Pts',(-33.5737828997118,4.10141821376346,21.1378098526377));
#54695=CARTESIAN_POINT('Ctrl Pts',(-33.801596834306,4.10506508715158,21.2813307553833));
#54696=CARTESIAN_POINT('Ctrl Pts',(-34.0187745948657,4.10854169536209,21.4181509560761));
#54697=CARTESIAN_POINT('Ctrl Pts',(-34.2323606929839,4.11232238479546,21.5482409335746));
#54698=CARTESIAN_POINT('Ctrl Pts',(-34.4422091994987,4.11638534088304,21.6719655411268));
#54699=CARTESIAN_POINT('Ctrl Pts',(-34.6983862296924,4.12134528099226,21.8230049888265));
#54700=CARTESIAN_POINT('Ctrl Pts',(-34.9489931041619,4.12672608777494,21.9645581634061));
#54701=CARTESIAN_POINT('Ctrl Pts',(-35.1937750867211,4.13247990804728,22.0972961327151));
#54702=CARTESIAN_POINT('Ctrl Pts',(-35.4313178144435,4.13806356313507,22.2261084700136));
#54703=CARTESIAN_POINT('Ctrl Pts',(-35.6633753700192,4.14399822754493,22.3466194588185));
#54704=CARTESIAN_POINT('Ctrl Pts',(-35.8897221244981,4.15022593205858,22.4594474749716));
#54705=CARTESIAN_POINT('Ctrl Pts',(-36.1280821148351,4.15678416873891,22.5782637791943));
#54706=CARTESIAN_POINT('Ctrl Pts',(-36.3601091602886,4.16366732082402,22.688560022379));
#54707=CARTESIAN_POINT('Ctrl Pts',(-36.5855452007813,4.17080074833602,22.7910624884676));
#54708=CARTESIAN_POINT('Ctrl Pts',(-36.9014638915004,4.18079730024053,22.9347060904907));
#54709=CARTESIAN_POINT('Ctrl Pts',(-37.2044390322616,4.19128489538215,23.0630439489659));
#54710=CARTESIAN_POINT('Ctrl Pts',(-37.4937605320397,4.20203012125431,23.1780823421347));
#54711=CARTESIAN_POINT('Ctrl Pts',(-37.6593150137322,4.20817871477847,23.2439091872548));
#54712=CARTESIAN_POINT('Ctrl Pts',(-37.8203989701946,4.21441160013928,23.3053814950684));
#54713=CARTESIAN_POINT('Ctrl Pts',(-37.9768795174009,4.22068493286446,23.362875825288));
#54714=CARTESIAN_POINT('Ctrl Pts',(-37.9980459759114,4.22153349991782,23.370652838961));
#54715=CARTESIAN_POINT('Ctrl Pts',(-38.0191282062722,4.22238280724491,23.3783570687426));
#54716=CARTESIAN_POINT('Ctrl Pts',(-38.0401258778123,4.22323274137395,23.385989447289));
#54717=CARTESIAN_POINT('Ctrl Pts',(-38.4250493867617,4.23881349882616,23.5259041004981));
#54718=CARTESIAN_POINT('Ctrl Pts',(-38.7814993652197,4.25460815954868,23.6416161168415));
#54719=CARTESIAN_POINT('Ctrl Pts',(-39.1025011525761,4.26968007837109,23.7382724472324));
#54720=CARTESIAN_POINT('Ctrl Pts',(-39.1939361781236,4.2739732048796,23.7658043002834));
#54721=CARTESIAN_POINT('Ctrl Pts',(-39.2824949682192,4.27820734981913,23.7917900658136));
#54722=CARTESIAN_POINT('Ctrl Pts',(-39.3680159669074,4.28236034493513,23.81634868312));
#54723=CARTESIAN_POINT('Ctrl Pts',(-39.5018516789771,4.28885955643987,23.8547815836366));
#54724=CARTESIAN_POINT('Ctrl Pts',(-39.6282476293091,4.29515990196685,23.8897193222904));
#54725=CARTESIAN_POINT('Ctrl Pts',(-39.7465823943656,4.30117637238633,23.92161762482));
#54726=CARTESIAN_POINT('Ctrl Pts',(-39.8741179109594,4.30766063474704,23.9559960806325));
#54727=CARTESIAN_POINT('Ctrl Pts',(-39.9922928698564,4.31381067584175,23.98684415462));
#54728=CARTESIAN_POINT('Ctrl Pts',(-40.1070321775967,4.31989179764076,24.0158116417197));
#54729=CARTESIAN_POINT('Ctrl Pts',(-40.1989532767345,4.32476356661657,24.0390183640358));
#54730=CARTESIAN_POINT('Ctrl Pts',(-40.2886693510511,4.32959237034955,24.0610181045133));
#54731=CARTESIAN_POINT('Ctrl Pts',(-40.3792268216836,4.3345384269169,24.0826590548447));
#54732=CARTESIAN_POINT('Ctrl Pts',(-40.5550100507714,4.34413933326496,24.124666810839));
#54733=CARTESIAN_POINT('Ctrl Pts',(-40.7339621950764,4.35418390708394,24.1653227568943));
#54734=CARTESIAN_POINT('Ctrl Pts',(-40.9199894723898,4.36493764138614,24.2052754880848));
#54735=CARTESIAN_POINT('Ctrl Pts',(-40.9494216450215,4.3666390357676,24.2115965808756));
#54736=CARTESIAN_POINT('Ctrl Pts',(-40.9790309204839,4.3683582876528,24.2179000708525));
#54737=CARTESIAN_POINT('Ctrl Pts',(-41.0088327685384,4.37009657042689,24.224188526569));
#54738=CARTESIAN_POINT('Ctrl Pts',(-41.2587538625024,4.38467397286592,24.2769241062269));
#54739=CARTESIAN_POINT('Ctrl Pts',(-41.522215837609,4.4005938813599,24.3286024290861));
#54740=CARTESIAN_POINT('Ctrl Pts',(-41.7959610673191,4.41781281081743,24.3778619523168));
#54741=CARTESIAN_POINT('Ctrl Pts',(-41.9123878923407,4.42513620888773,24.3988125635764));
#54742=CARTESIAN_POINT('Ctrl Pts',(-42.030674852438,4.43269397282911,24.4193256463625));
#54743=CARTESIAN_POINT('Ctrl Pts',(-42.1505713508101,4.44047982652793,24.439296481844));
#54744=CARTESIAN_POINT('Ctrl Pts',(-42.2409398060512,4.44634818449541,24.4543489110379));
#54745=CARTESIAN_POINT('Ctrl Pts',(-42.3322226369957,4.45234608023781,24.4690932928778));
#54746=CARTESIAN_POINT('Ctrl Pts',(-42.42431198011,4.45847033217187,24.4834847584958));
#54747=CARTESIAN_POINT('Ctrl Pts',(-42.784797503065,4.48244383536452,24.5398204302896));
#54748=CARTESIAN_POINT('Ctrl Pts',(-43.1576489772132,4.5083540926368,24.590748313527));
#54749=CARTESIAN_POINT('Ctrl Pts',(-43.5419429082308,4.5363561170648,24.635085509321));
#54750=CARTESIAN_POINT('Ctrl Pts',(-43.6923106007685,4.54731283394157,24.6524339014944));
#54751=CARTESIAN_POINT('Ctrl Pts',(-43.8444299906764,4.55858966891662,24.6687732511125));
#54752=CARTESIAN_POINT('Ctrl Pts',(-43.9982463104202,4.57019670241406,24.6840326452309));
#54753=CARTESIAN_POINT('Ctrl Pts',(-43.9982497229159,4.57019695992218,24.6840329837686));
#54754=CARTESIAN_POINT('Ctrl Pts',(-43.9982531354125,4.57019721743047,24.6840333223057));
#54755=CARTESIAN_POINT('Ctrl Pts',(-43.9982565479099,4.57019747493892,24.6840336608423));
#54756=CARTESIAN_POINT('',(-25.4568055127478,4.0805540095759,12.6479974296003));
#54757=CARTESIAN_POINT('Ctrl Pts',(-25.4568055127484,4.08055401005756,12.6479974296003));
#54758=CARTESIAN_POINT('Ctrl Pts',(-27.0327363192644,4.07841070070495,15.0082590047032));
#54759=CARTESIAN_POINT('Ctrl Pts',(-28.2185108053635,4.07131231245263,16.7905674249077));
#54760=CARTESIAN_POINT('Ctrl Pts',(-30.3134449229829,4.07585757700934,18.6659931355318));
#54761=CARTESIAN_POINT('',(-21.1401509099359,4.08071597508933,6.62997962237056));
#54762=CARTESIAN_POINT('Ctrl Pts',(-21.1401574799756,4.08071597981543,6.62998826233523));
#54763=CARTESIAN_POINT('Ctrl Pts',(-21.4692458061929,4.08095270291158,7.06232595293004));
#54764=CARTESIAN_POINT('Ctrl Pts',(-21.7882670410954,4.08118452196195,7.48072007481999));
#54765=CARTESIAN_POINT('Ctrl Pts',(-22.1061108542803,4.08137642561277,7.90235762953136));
#54766=CARTESIAN_POINT('Ctrl Pts',(-22.284711446525,4.08148425878198,8.13928128152719));
#54767=CARTESIAN_POINT('Ctrl Pts',(-22.4629415192341,4.0815794918012,8.37723040795624));
#54768=CARTESIAN_POINT('Ctrl Pts',(-22.6423690871753,4.08165601858648,8.61922908722337));
#54769=CARTESIAN_POINT('Ctrl Pts',(-22.7822570470729,4.08171568152453,8.80789965735382));
#54770=CARTESIAN_POINT('Ctrl Pts',(-22.9228728197913,4.0817639754497,8.99903144132748));
#54771=CARTESIAN_POINT('Ctrl Pts',(-23.0649499739826,4.08179806827018,9.19403707854816));
#54772=CARTESIAN_POINT('Ctrl Pts',(-23.089242443057,4.08180389748876,9.22737930333079));
#54773=CARTESIAN_POINT('Ctrl Pts',(-23.1135776064206,4.0818093117026,9.26083472002905));
#54774=CARTESIAN_POINT('Ctrl Pts',(-23.1379446185742,4.08181430925493,9.29438788392053));
#54775=CARTESIAN_POINT('Ctrl Pts',(-23.2474269721439,4.08183676353811,9.44514413295864));
#54776=CARTESIAN_POINT('Ctrl Pts',(-23.3579353512576,4.08184894949124,9.59840224218975));
#54777=CARTESIAN_POINT('Ctrl Pts',(-23.4683481026768,4.08185062199027,9.75258737280672));
#54778=CARTESIAN_POINT('Ctrl Pts',(-23.6195577047054,4.08185291246768,9.96374298608199));
#54779=CARTESIAN_POINT('Ctrl Pts',(-23.7705834817783,4.08183546777614,10.1766325430206));
#54780=CARTESIAN_POINT('Ctrl Pts',(-23.9185172660665,4.08179797831881,10.3871359698167));
#54781=CARTESIAN_POINT('Ctrl Pts',(-24.0197941038079,4.08177231268939,10.5312485638547));
#54782=CARTESIAN_POINT('Ctrl Pts',(-24.1196208989452,4.08173725990457,10.6742407070177));
#54783=CARTESIAN_POINT('Ctrl Pts',(-24.2170854846451,4.08169283385564,10.8148087558425));
#54784=CARTESIAN_POINT('Ctrl Pts',(-24.2619861753325,4.08167236734191,10.8795666618601));
#54785=CARTESIAN_POINT('Ctrl Pts',(-24.3063859262931,4.08164991286656,10.9438105322975));
#54786=CARTESIAN_POINT('Ctrl Pts',(-24.3501981466148,4.08162547894153,11.0074159299064));
#54787=CARTESIAN_POINT('Ctrl Pts',(-24.3825541098732,4.08160743413177,11.0543894430712));
#54788=CARTESIAN_POINT('Ctrl Pts',(-24.4145897119851,4.08158830987438,11.1010148268432));
#54789=CARTESIAN_POINT('Ctrl Pts',(-24.4463194375088,4.08156817329577,11.147301956624));
#54790=CARTESIAN_POINT('Ctrl Pts',(-24.5269242714908,4.08151701919503,11.2648877960821));
#54791=CARTESIAN_POINT('Ctrl Pts',(-24.6061395773467,4.08145979701039,11.3811447622533));
#54792=CARTESIAN_POINT('Ctrl Pts',(-24.6840716542324,4.08139685593094,11.4960646524234));
#54793=CARTESIAN_POINT('Ctrl Pts',(-24.7705692911081,4.08132699696077,11.6236154546984));
#54794=CARTESIAN_POINT('Ctrl Pts',(-24.8554863518349,4.08125009280203,11.7495191699868));
#54795=CARTESIAN_POINT('Ctrl Pts',(-24.939014259396,4.08116678926922,11.8738119545452));
#54796=CARTESIAN_POINT('Ctrl Pts',(-25.033126716636,4.08107292961922,12.013854961889));
#54797=CARTESIAN_POINT('Ctrl Pts',(-25.1254766313393,4.08097094742442,12.1518534862534));
#54798=CARTESIAN_POINT('Ctrl Pts',(-25.2163841921841,4.08086196114674,12.2879118774981));
#54799=CARTESIAN_POINT('Ctrl Pts',(-25.2975937607871,4.08076460149357,12.4094555990007));
#54800=CARTESIAN_POINT('Ctrl Pts',(-25.3776540492092,4.08066165823048,12.5294527346467));
#54801=CARTESIAN_POINT('Ctrl Pts',(-25.4568055127484,4.08055401005756,12.6479974296003));
#54802=CARTESIAN_POINT('',(-16.686777128013,4.07896401785927,0.570989604234123));
#54803=CARTESIAN_POINT('Ctrl Pts',(-16.6867771273137,4.07896172090824,0.570989650428049));
#54804=CARTESIAN_POINT('Ctrl Pts',(-16.7841459689088,4.08162687912007,0.704986248288088));
#54805=CARTESIAN_POINT('Ctrl Pts',(-16.880846010462,4.08355025119849,0.838584067301125));
#54806=CARTESIAN_POINT('Ctrl Pts',(-16.9766362404799,4.08495392785334,0.971294459765536));
#54807=CARTESIAN_POINT('Ctrl Pts',(-17.0096954643441,4.08543836620115,1.01709560851285));
#54808=CARTESIAN_POINT('Ctrl Pts',(-17.0426464502949,4.08586064648245,1.0627911508977));
#54809=CARTESIAN_POINT('Ctrl Pts',(-17.0754929950314,4.08622882894667,1.10837987529852));
#54810=CARTESIAN_POINT('Ctrl Pts',(-17.1731007695106,4.08732293096634,1.24385269187051));
#54811=CARTESIAN_POINT('Ctrl Pts',(-17.2697875086632,4.08794300664813,1.37838378599298));
#54812=CARTESIAN_POINT('Ctrl Pts',(-17.3656435015793,4.08826316038151,1.51193079495319));
#54813=CARTESIAN_POINT('Ctrl Pts',(-17.4642655981198,4.08859255274855,1.6493315521692));
#54814=CARTESIAN_POINT('Ctrl Pts',(-17.5620082347372,4.0886040867082,1.7856907594135));
#54815=CARTESIAN_POINT('Ctrl Pts',(-17.6589529261752,4.08843757506459,1.92093947295767));
#54816=CARTESIAN_POINT('Ctrl Pts',(-17.7610551734985,4.0882622048327,2.06338355520294));
#54817=CARTESIAN_POINT('Ctrl Pts',(-17.8622722619584,4.08788904084334,2.20459606314489));
#54818=CARTESIAN_POINT('Ctrl Pts',(-17.9626819456571,4.08743203252299,2.34446843489057));
#54819=CARTESIAN_POINT('Ctrl Pts',(-17.9857716705684,4.08732694110143,2.37663280855774));
#54820=CARTESIAN_POINT('Ctrl Pts',(-18.0088224426463,4.08721631990852,2.40873151016149));
#54821=CARTESIAN_POINT('Ctrl Pts',(-18.0318289356247,4.08710273253635,2.440754419878));
#54822=CARTESIAN_POINT('Ctrl Pts',(-18.0826477931075,4.08685183030264,2.51148956784678));
#54823=CARTESIAN_POINT('Ctrl Pts',(-18.1332504270625,4.08658646050215,2.58185461834398));
#54824=CARTESIAN_POINT('Ctrl Pts',(-18.1836567657045,4.08631176891754,2.65186612027432));
#54825=CARTESIAN_POINT('Ctrl Pts',(-18.2770994146918,4.08580254904538,2.78165257920393));
#54826=CARTESIAN_POINT('Ctrl Pts',(-18.3694162091785,4.08527202707044,2.90959746665377));
#54827=CARTESIAN_POINT('Ctrl Pts',(-18.4612811429612,4.08475867356178,3.03657594574594));
#54828=CARTESIAN_POINT('Ctrl Pts',(-18.4688691213433,4.08471627092602,3.04706427806888));
#54829=CARTESIAN_POINT('Ctrl Pts',(-18.4764540006169,4.08467398512724,3.05754599355073));
#54830=CARTESIAN_POINT('Ctrl Pts',(-18.4840361525888,4.08463183770619,3.06802157368569));
#54831=CARTESIAN_POINT('Ctrl Pts',(-18.5451231850346,4.08429226908686,3.15242005395425));
#54832=CARTESIAN_POINT('Ctrl Pts',(-18.6060211115761,4.08396170556085,3.23640371253096));
#54833=CARTESIAN_POINT('Ctrl Pts',(-18.6669509110043,4.08364541281635,3.32026056370214));
#54834=CARTESIAN_POINT('Ctrl Pts',(-18.7190814341725,4.0833747980039,3.39200709107969));
#54835=CARTESIAN_POINT('Ctrl Pts',(-18.7712351265386,4.08311462674048,3.46366056109551));
#54836=CARTESIAN_POINT('Ctrl Pts',(-18.8235118219749,4.08286882610003,3.53534797170876));
#54837=CARTESIAN_POINT('Ctrl Pts',(-18.8441314456826,4.08277187435756,3.56362381085831));
#54838=CARTESIAN_POINT('Ctrl Pts',(-18.8647718882406,4.08267706144966,3.59190722809431));
#54839=CARTESIAN_POINT('Ctrl Pts',(-18.8854405400068,4.08258452488808,3.62020769046226));
#54840=CARTESIAN_POINT('Ctrl Pts',(-18.9139413939724,4.08245692241754,3.6592323619423));
#54841=CARTESIAN_POINT('Ctrl Pts',(-18.94249588657,4.08233365051722,3.69828944962005));
#54842=CARTESIAN_POINT('Ctrl Pts',(-18.9711233744466,4.08221500263331,3.73740362574907));
#54843=CARTESIAN_POINT('Ctrl Pts',(-19.0606946304323,4.08184377061924,3.8597862077566));
#54844=CARTESIAN_POINT('Ctrl Pts',(-19.1509291277118,4.08151777088175,3.98265901523723));
#54845=CARTESIAN_POINT('Ctrl Pts',(-19.242528424724,4.08124251797849,4.10691573705344));
#54846=CARTESIAN_POINT('Ctrl Pts',(-19.2635485518487,4.08117935318131,4.1354300616593));
#54847=CARTESIAN_POINT('Ctrl Pts',(-19.2846407111546,4.08111887286734,4.16401739825223));
#54848=CARTESIAN_POINT('Ctrl Pts',(-19.3058137050309,4.08106116769549,4.19268882867069));
#54849=CARTESIAN_POINT('Ctrl Pts',(-19.3322323911041,4.0809891658412,4.2284637183211));
#54850=CARTESIAN_POINT('Ctrl Pts',(-19.3587769939038,4.08092148536531,4.26436962064455));
#54851=CARTESIAN_POINT('Ctrl Pts',(-19.3854337817106,4.08085764253541,4.30038893000356));
#54852=CARTESIAN_POINT('Ctrl Pts',(-19.39842995467,4.08082651678742,4.31794967954701));
#54853=CARTESIAN_POINT('Ctrl Pts',(-19.4114573113798,4.08079638090457,4.33554349027692));
#54854=CARTESIAN_POINT('Ctrl Pts',(-19.4245173432076,4.08076723479642,4.35317245358558));
#54855=CARTESIAN_POINT('Ctrl Pts',(-19.489472938666,4.08062227321939,4.44085216402782));
#54856=CARTESIAN_POINT('Ctrl Pts',(-19.5537417608887,4.08050583169764,4.52738438607107));
#54857=CARTESIAN_POINT('Ctrl Pts',(-19.6173542232542,4.08041287513929,4.61284247073614));
#54858=CARTESIAN_POINT('Ctrl Pts',(-19.6961025636338,4.08029780060161,4.7186343563062));
#54859=CARTESIAN_POINT('Ctrl Pts',(-19.7738497167904,4.08021869702705,4.82278679314521));
#54860=CARTESIAN_POINT('Ctrl Pts',(-19.8506921953251,4.08016901437943,4.92546814305012));
#54861=CARTESIAN_POINT('Ctrl Pts',(-19.885211075738,4.08014669613301,4.97159426112431));
#54862=CARTESIAN_POINT('Ctrl Pts',(-19.919553701739,4.08013009809011,5.01743162922105));
#54863=CARTESIAN_POINT('Ctrl Pts',(-19.9537115876116,4.08011650017662,5.06297116675175));
#54864=CARTESIAN_POINT('Ctrl Pts',(-19.9695992615268,4.08011017545218,5.08415272714558));
#54865=CARTESIAN_POINT('Ctrl Pts',(-19.9854469188514,4.08010450048555,5.1052697797261));
#54866=CARTESIAN_POINT('Ctrl Pts',(-20.0012608379634,4.08009922299098,5.1263311055391));
#54867=CARTESIAN_POINT('Ctrl Pts',(-20.0876094687218,4.08007040632468,5.24133211401896));
#54868=CARTESIAN_POINT('Ctrl Pts',(-20.1728585866075,4.08007004066717,5.35454628879534));
#54869=CARTESIAN_POINT('Ctrl Pts',(-20.2571125809195,4.08009030729853,5.46618501499764));
#54870=CARTESIAN_POINT('Ctrl Pts',(-20.3344593924838,4.08010891246175,5.56867154503511));
#54871=CARTESIAN_POINT('Ctrl Pts',(-20.4109698888398,4.08014488839819,5.66983361846497));
#54872=CARTESIAN_POINT('Ctrl Pts',(-20.4867385357516,4.08019174670546,5.76985765191063));
#54873=CARTESIAN_POINT('Ctrl Pts',(-20.5985299989913,4.08026088293725,5.91743628124831));
#54874=CARTESIAN_POINT('Ctrl Pts',(-20.7086941885613,4.08035370311237,6.06252104066088));
#54875=CARTESIAN_POINT('Ctrl Pts',(-20.8175153853736,4.08044838230245,6.20569714733634));
#54876=CARTESIAN_POINT('Ctrl Pts',(-20.8837484074139,4.08050600792197,6.29283996975399));
#54877=CARTESIAN_POINT('Ctrl Pts',(-20.9494899802706,4.08056430624765,6.37928395918526));
#54878=CARTESIAN_POINT('Ctrl Pts',(-21.0147749929071,4.08061833242126,6.46512326211024));
#54879=CARTESIAN_POINT('Ctrl Pts',(-21.056753592743,4.08065307152953,6.52031837661131));
#54880=CARTESIAN_POINT('Ctrl Pts',(-21.0985432473107,4.08068604483045,6.57526325140479));
#54881=CARTESIAN_POINT('Ctrl Pts',(-21.1401509099359,4.08071597508933,6.62997962237056));
#54882=CARTESIAN_POINT('Ctrl Pts',(-10.8670147648799,2.7042092247722,-5.65154550519047));
#54883=CARTESIAN_POINT('Ctrl Pts',(-10.8825819667526,2.70903278193244,-5.64047515756788));
#54884=CARTESIAN_POINT('Ctrl Pts',(-10.8981033350986,2.71386799061846,-5.62937871312437));
#54885=CARTESIAN_POINT('Ctrl Pts',(-10.9135792074401,2.71871360214693,-5.61825800418583));
#54886=CARTESIAN_POINT('Ctrl Pts',(-11.0107587992363,2.74914126011334,-5.54842633775175));
#54887=CARTESIAN_POINT('Ctrl Pts',(-11.1061434441261,2.77997495059204,-5.477637425274));
#54888=CARTESIAN_POINT('Ctrl Pts',(-11.1997509871659,2.81085934490754,-5.40635622923117));
#54889=CARTESIAN_POINT('Ctrl Pts',(-11.2928171879274,2.84156513151862,-5.33548725985091));
#54890=CARTESIAN_POINT('Ctrl Pts',(-11.3841265997849,2.87232103418462,-5.26413206407766));
#54891=CARTESIAN_POINT('Ctrl Pts',(-11.4737096205386,2.90282774713705,-5.19274952618222));
#54892=CARTESIAN_POINT('Ctrl Pts',(-11.5164512601376,2.91738303807718,-5.15869165804243));
#54893=CARTESIAN_POINT('Ctrl Pts',(-11.5588001080816,2.93188233724435,-5.12462755866404));
#54894=CARTESIAN_POINT('Ctrl Pts',(-11.6007606569768,2.94629714755178,-5.09060688784509));
#54895=CARTESIAN_POINT('Ctrl Pts',(-11.6698696768522,2.97003833870074,-5.03457484637507));
#54896=CARTESIAN_POINT('Ctrl Pts',(-11.737965114793,2.99357278208341,-4.97856686204584));
#54897=CARTESIAN_POINT('Ctrl Pts',(-11.8054490598404,3.01696025884261,-4.92223728584462));
#54898=CARTESIAN_POINT('Ctrl Pts',(-11.8794776799778,3.04261588155053,-4.86044479881427));
#54899=CARTESIAN_POINT('Ctrl Pts',(-11.952770434535,3.06809557782894,-4.7982654510355));
#54900=CARTESIAN_POINT('Ctrl Pts',(-12.0258886104834,3.09350467545653,-4.73519326240181));
#54901=CARTESIAN_POINT('Ctrl Pts',(-12.102122512934,3.11999651069141,-4.66943342890923));
#54902=CARTESIAN_POINT('Ctrl Pts',(-12.1781669364099,3.14641306799247,-4.60270275829058));
#54903=CARTESIAN_POINT('Ctrl Pts',(-12.2546871001548,3.17288172182397,-4.53437800091278));
#54904=CARTESIAN_POINT('Ctrl Pts',(-12.3317459488349,3.19953670909201,-4.46557225243795));
#54905=CARTESIAN_POINT('Ctrl Pts',(-12.4092877338435,3.22624611123961,-4.39514937721361));
#54906=CARTESIAN_POINT('Ctrl Pts',(-12.4880146031307,3.25312461003796,-4.32242993472665));
#54907=CARTESIAN_POINT('Ctrl Pts',(-12.5192375769084,3.26378458763852,-4.29358949859024));
#54908=CARTESIAN_POINT('Ctrl Pts',(-12.5506471645991,3.27447086295421,-4.26438740435322));
#54909=CARTESIAN_POINT('Ctrl Pts',(-12.5822878884511,3.28518907137685,-4.23477968801371));
#54910=CARTESIAN_POINT('Ctrl Pts',(-12.6568047736437,3.31043146185554,-4.16505072702003));
#54911=CARTESIAN_POINT('Ctrl Pts',(-12.7326033668085,3.33585402022417,-4.09307337513168));
#54912=CARTESIAN_POINT('Ctrl Pts',(-12.8102719529775,3.36149876026795,-4.01825763687434));
#54913=CARTESIAN_POINT('Ctrl Pts',(-12.8439067468809,3.37260435119765,-3.98585828391655));
#54914=CARTESIAN_POINT('Ctrl Pts',(-12.8778922944557,3.38375105078127,-3.95292636620954));
#54915=CARTESIAN_POINT('Ctrl Pts',(-12.9122764856802,3.3949393291939,-3.91941291420406));
#54916=CARTESIAN_POINT('Ctrl Pts',(-12.9370845594558,3.40301163295904,-3.89523307573123));
#54917=CARTESIAN_POINT('Ctrl Pts',(-12.9621001530937,3.41110553892594,-3.87075050495877));
#54918=CARTESIAN_POINT('Ctrl Pts',(-12.9873408891014,3.41922107952233,-3.84594638986787));
#54919=CARTESIAN_POINT('Ctrl Pts',(-13.0760628982132,3.44774746902704,-3.75875911749837));
#54920=CARTESIAN_POINT('Ctrl Pts',(-13.1675146048207,3.47651397214489,-3.66771261218589));
#54921=CARTESIAN_POINT('Ctrl Pts',(-13.2613154033226,3.50517803164381,-3.57289531261814));
#54922=CARTESIAN_POINT('Ctrl Pts',(-13.3558400529778,3.53406328875359,-3.47734631766253));
#54923=CARTESIAN_POINT('Ctrl Pts',(-13.4527501050739,3.56284323316075,-3.3779680079072));
#54924=CARTESIAN_POINT('Ctrl Pts',(-13.5516154260481,3.591163592317,-3.27488416648269));
#54925=CARTESIAN_POINT('Ctrl Pts',(-13.6339391159868,3.61474553635114,-3.18904777698334));
#54926=CARTESIAN_POINT('Ctrl Pts',(-13.7176176631479,3.63800835248907,-3.10064273411202));
#54927=CARTESIAN_POINT('Ctrl Pts',(-13.8023830403473,3.66075569667637,-3.00975812175573));
#54928=CARTESIAN_POINT('Ctrl Pts',(-13.8961548674793,3.68591998069561,-2.90921688144739));
#54929=CARTESIAN_POINT('Ctrl Pts',(-13.9912484919101,3.71045810812311,-2.8056379406839));
#54930=CARTESIAN_POINT('Ctrl Pts',(-14.0880081563311,3.73427239190452,-2.69847830019729));
#54931=CARTESIAN_POINT('Ctrl Pts',(-14.0986567235059,3.73689319471615,-2.68668519780301));
#54932=CARTESIAN_POINT('Ctrl Pts',(-14.1093254421708,3.73950518591304,-2.67484873235818));
#54933=CARTESIAN_POINT('Ctrl Pts',(-14.1200147504619,3.74210820192807,-2.66296818424889));
#54934=CARTESIAN_POINT('Ctrl Pts',(-14.215122794505,3.76526851829853,-2.55726109244567));
#54935=CARTESIAN_POINT('Ctrl Pts',(-14.3118634807218,3.78772128016114,-2.44806304643595));
#54936=CARTESIAN_POINT('Ctrl Pts',(-14.4105259337003,3.80933210165384,-2.33487331767942));
#54937=CARTESIAN_POINT('Ctrl Pts',(-14.5090268780975,3.83090754663789,-2.22186887838165));
#54938=CARTESIAN_POINT('Ctrl Pts',(-14.6094437433893,3.85164325824876,-2.10488521430534));
#54939=CARTESIAN_POINT('Ctrl Pts',(-14.712027927971,3.87137351965582,-1.98344311485669));
#54940=CARTESIAN_POINT('Ctrl Pts',(-14.7480030930743,3.87829270914438,-1.94085468277071));
#54941=CARTESIAN_POINT('Ctrl Pts',(-14.784252937188,3.88508861678897,-1.89771585291644));
#54942=CARTESIAN_POINT('Ctrl Pts',(-14.8207338105388,3.89174386471088,-1.85407313434892));
#54943=CARTESIAN_POINT('Ctrl Pts',(-14.8955878522407,3.90539957412038,-1.76452391100031));
#54944=CARTESIAN_POINT('Ctrl Pts',(-14.971414188907,3.91846034565269,-1.67285267325724));
#54945=CARTESIAN_POINT('Ctrl Pts',(-15.0478385606804,3.93080581904371,-1.57947261102481));
#54946=CARTESIAN_POINT('Ctrl Pts',(-15.1270962517208,3.9436089823942,-1.4826306226641));
#54947=CARTESIAN_POINT('Ctrl Pts',(-15.2069966171596,3.95564252009211,-1.38395112278974));
#54948=CARTESIAN_POINT('Ctrl Pts',(-15.2871330839331,3.96682523634334,-1.2838979026888));
#54949=CARTESIAN_POINT('Ctrl Pts',(-15.3511514963117,3.97575874401229,-1.20396864498479));
#54950=CARTESIAN_POINT('Ctrl Pts',(-15.4153207078596,3.98415025880874,-1.12316291197415));
#54951=CARTESIAN_POINT('Ctrl Pts',(-15.4794409402304,3.99198113393681,-1.04171785846541));
#54952=CARTESIAN_POINT('Ctrl Pts',(-15.5573651090663,4.00149785608596,-0.94273914510455));
#54953=CARTESIAN_POINT('Ctrl Pts',(-15.6352162293308,4.01018564820184,-0.842816346832298));
#54954=CARTESIAN_POINT('Ctrl Pts',(-15.7126525047195,4.01805069496177,-0.742364156738377));
#54955=CARTESIAN_POINT('Ctrl Pts',(-15.8133014664812,4.02827340759379,-0.611799914219101));
#54956=CARTESIAN_POINT('Ctrl Pts',(-15.9132436882516,4.03708677559505,-0.480700346086931));
#54957=CARTESIAN_POINT('Ctrl Pts',(-16.0122412921091,4.04463271570221,-0.349301786997184));
#54958=CARTESIAN_POINT('Ctrl Pts',(-16.0416708873646,4.04687594134125,-0.310240170750923));
#54959=CARTESIAN_POINT('Ctrl Pts',(-16.0710172335301,4.04900741347074,-0.271152030394429));
#54960=CARTESIAN_POINT('Ctrl Pts',(-16.100274661319,4.05103144399587,-0.232043298691982));
#54961=CARTESIAN_POINT('Ctrl Pts',(-16.1836574145965,4.05679986762905,-0.120584637661964));
#54962=CARTESIAN_POINT('Ctrl Pts',(-16.2663166502409,4.06169446575746,-0.00896259225158377));
#54963=CARTESIAN_POINT('Ctrl Pts',(-16.3481339461205,4.06582084985792,0.102612874254018));
#54964=CARTESIAN_POINT('Ctrl Pts',(-16.3647111828591,4.06665690836331,0.125219499205496));
#54965=CARTESIAN_POINT('Ctrl Pts',(-16.3812539136449,4.06746147727406,0.147824366621108));
#54966=CARTESIAN_POINT('Ctrl Pts',(-16.3977612396738,4.06823550038658,0.170425963319117));
#54967=CARTESIAN_POINT('Ctrl Pts',(-16.4465477097304,4.07052308199341,0.237223706249112));
#54968=CARTESIAN_POINT('Ctrl Pts',(-16.4950247902217,4.07254398783715,0.30399644028247));
#54969=CARTESIAN_POINT('Ctrl Pts',(-16.5431702873596,4.07432687884092,0.370874939270894));
#54970=CARTESIAN_POINT('Ctrl Pts',(-16.5745169579264,4.07548768722953,0.41441833170452));
#54971=CARTESIAN_POINT('Ctrl Pts',(-16.6057230998384,4.07654732854821,0.458000668758363));
#54972=CARTESIAN_POINT('Ctrl Pts',(-16.6367834831488,4.07750677533081,0.501329112044902));
#54973=CARTESIAN_POINT('Ctrl Pts',(-16.6533361456736,4.07801808256884,0.524419654498255));
#54974=CARTESIAN_POINT('Ctrl Pts',(-16.6698474196488,4.07850097957143,0.547438993526175));
#54975=CARTESIAN_POINT('Ctrl Pts',(-16.6863165610272,4.07895589513591,0.570348816731394));
#54976=CARTESIAN_POINT('Ctrl Pts',(-16.6864700870274,4.07896013587715,0.570562383027311));
#54977=CARTESIAN_POINT('Ctrl Pts',(-16.6866236098607,4.07896437475301,0.570775948118517));
#54978=CARTESIAN_POINT('Ctrl Pts',(-16.6867771295269,4.07896861176448,0.57098951200485));
#54979=CARTESIAN_POINT('',(-34.5094710129489,4.11696067448647,0.612674457278041));
#54980=CARTESIAN_POINT('',(-35.0820169555422,4.13115532855471,-2.69386316078375));
#54981=CARTESIAN_POINT('Origin',(-42.4365979192343,4.31984058958519,0.26838881652106));
#54982=CARTESIAN_POINT('',(-35.2886576356463,4.13442741082932,6.62929523481876));
#54983=CARTESIAN_POINT('Ctrl Pts',(-35.2883365499271,4.13441961266498,6.62833239954248));
#54984=CARTESIAN_POINT('Ctrl Pts',(-34.6423025074559,4.11873027055746,4.6907194393648));
#54985=CARTESIAN_POINT('Ctrl Pts',(-34.3775118580705,4.11384875218964,2.64941339379631));
#54986=CARTESIAN_POINT('Ctrl Pts',(-34.5094662196082,4.1169605614472,0.612748436480715));
#54987=CARTESIAN_POINT('',(-38.96547857039,4.2626731672903,12.6510864480354));
#54988=CARTESIAN_POINT('Ctrl Pts',(-38.9640138900455,4.26260658610796,12.6495838748125));
#54989=CARTESIAN_POINT('Ctrl Pts',(-37.3069065807585,4.18728739522815,10.9493640627874));
#54990=CARTESIAN_POINT('Ctrl Pts',(-36.0425989591165,4.1527392094223,8.88970910721889));
#54991=CARTESIAN_POINT('Ctrl Pts',(-35.2888843457993,4.13443291690738,6.6299750673985));
#54992=CARTESIAN_POINT('',(-61.2151481505771,6.62152250824553,12.6564237477171));
#54993=CARTESIAN_POINT('Ctrl Pts',(-61.2151481505771,6.62152250824553,12.6564237477171));
#54994=CARTESIAN_POINT('Ctrl Pts',(-58.2965417115554,6.22483785549351,15.6153467534928));
#54995=CARTESIAN_POINT('Ctrl Pts',(-50.1081788357534,4.96418169793774,19.0244081704428));
#54996=CARTESIAN_POINT('Ctrl Pts',(-41.8770097886242,4.39504138626396,15.6375182081803));
#54997=CARTESIAN_POINT('Ctrl Pts',(-38.96547857039,4.2626731672903,12.6510864480354));
#54998=CARTESIAN_POINT('',(-64.9284491122907,7.16443381643712,6.63636663678025));
#54999=CARTESIAN_POINT('Ctrl Pts',(-64.9279798115614,7.16341862632849,6.63807904463546));
#55000=CARTESIAN_POINT('Ctrl Pts',(-64.8508885627514,7.15299985198849,6.86358669794533));
#55001=CARTESIAN_POINT('Ctrl Pts',(-64.7684102394653,7.14156243532073,7.08720349281578));
#55002=CARTESIAN_POINT('Ctrl Pts',(-64.6809064278057,7.12914354033835,7.30871875086926));
#55003=CARTESIAN_POINT('Ctrl Pts',(-64.5974607138085,7.11730058699488,7.51996096442497));
#55004=CARTESIAN_POINT('Ctrl Pts',(-64.5094459744822,7.1045662353132,7.72929139412695));
#55005=CARTESIAN_POINT('Ctrl Pts',(-64.4171380221575,7.09100102588375,7.93652647044922));
#55006=CARTESIAN_POINT('Ctrl Pts',(-64.3852592526469,7.08631624874512,8.00809559386943));
#55007=CARTESIAN_POINT('Ctrl Pts',(-64.3528680238246,7.08153255014063,8.07941484428056));
#55008=CARTESIAN_POINT('Ctrl Pts',(-64.3199742825305,7.07665281288929,8.1504768514447));
#55009=CARTESIAN_POINT('Ctrl Pts',(-64.3071410638109,7.07474902411438,8.17820110063947));
#55010=CARTESIAN_POINT('Ctrl Pts',(-64.2942313488762,7.07283061818773,8.2058861961849));
#55011=CARTESIAN_POINT('Ctrl Pts',(-64.2812457042831,7.0708977660961,8.23353171912382));
#55012=CARTESIAN_POINT('Ctrl Pts',(-64.1910552011233,7.05747333410678,8.42554094947833));
#55013=CARTESIAN_POINT('Ctrl Pts',(-64.0972054525586,7.04334975225786,8.6156411800766));
#55014=CARTESIAN_POINT('Ctrl Pts',(-63.9998442582977,7.0285858672386,8.80367434032654));
#55015=CARTESIAN_POINT('Ctrl Pts',(-63.9029115746634,7.01388696171829,8.99087992026658));
#55016=CARTESIAN_POINT('Ctrl Pts',(-63.8024983496159,6.99855324463019,9.1760363662355));
#55017=CARTESIAN_POINT('Ctrl Pts',(-63.6987070211235,6.98267230296273,9.35899039531681));
#55018=CARTESIAN_POINT('Ctrl Pts',(-63.6417591017022,6.97395879481566,9.45937307137728));
#55019=CARTESIAN_POINT('Ctrl Pts',(-63.5837934413672,6.9650810994762,9.5590927750825));
#55020=CARTESIAN_POINT('Ctrl Pts',(-63.5248214191519,6.95605724044794,9.65812507941458));
#55021=CARTESIAN_POINT('Ctrl Pts',(-63.5210198925743,6.95547553341739,9.6645090208637));
#55022=CARTESIAN_POINT('Ctrl Pts',(-63.5172141827313,6.95489321973694,9.67089010615184));
#55023=CARTESIAN_POINT('Ctrl Pts',(-63.5134042920641,6.95431030451018,9.67726832887461));
#55024=CARTESIAN_POINT('Ctrl Pts',(-63.4053691505814,6.93778087243555,9.85813236263684));
#55025=CARTESIAN_POINT('Ctrl Pts',(-63.2939758134642,6.92076945837511,10.0366929411969));
#55026=CARTESIAN_POINT('Ctrl Pts',(-63.179268520996,6.90337495979145,10.2128406339241));
#55027=CARTESIAN_POINT('Ctrl Pts',(-63.0644443776627,6.88596274165252,10.3891677660735));
#55028=CARTESIAN_POINT('Ctrl Pts',(-62.9462992983965,6.86816729533639,10.5630773346187));
#55029=CARTESIAN_POINT('Ctrl Pts',(-62.8248362353091,6.85006129639097,10.7344780991604));
#55030=CARTESIAN_POINT('Ctrl Pts',(-62.7237908235596,6.83499887270372,10.8770668038006));
#55031=CARTESIAN_POINT('Ctrl Pts',(-62.6204482553076,6.81972118356617,11.0179197159958));
#55032=CARTESIAN_POINT('Ctrl Pts',(-62.514791071203,6.80425173418117,11.1569917197539));
#55033=CARTESIAN_POINT('Ctrl Pts',(-62.3870909877244,6.78555494612483,11.3250778431912));
#55034=CARTESIAN_POINT('Ctrl Pts',(-62.256009986916,6.76657955576061,11.4905618395803));
#55035=CARTESIAN_POINT('Ctrl Pts',(-62.1214919444444,6.74732763669793,11.6533667143777));
#55036=CARTESIAN_POINT('Ctrl Pts',(-62.0878954759279,6.74251938584335,11.6940279427896));
#55037=CARTESIAN_POINT('Ctrl Pts',(-62.0540845042587,6.73769366259078,11.7345221212631));
#55038=CARTESIAN_POINT('Ctrl Pts',(-62.0200579664813,6.73285005326746,11.7748481636997));
#55039=CARTESIAN_POINT('Ctrl Pts',(-61.9835559126172,6.7276540592003,11.8181080270094));
#55040=CARTESIAN_POINT('Ctrl Pts',(-61.9468057712324,6.72243747786662,11.8611743977494));
#55041=CARTESIAN_POINT('Ctrl Pts',(-61.9098067959039,6.71720001308234,11.9040458787038));
#55042=CARTESIAN_POINT('Ctrl Pts',(-61.7985120786369,6.70144546428232,12.0330053785082));
#55043=CARTESIAN_POINT('Ctrl Pts',(-61.6849649179537,6.68550281059298,12.1602033116016));
#55044=CARTESIAN_POINT('Ctrl Pts',(-61.5691520865945,6.66935638985563,12.2856216372723));
#55045=CARTESIAN_POINT('Ctrl Pts',(-61.4549290846619,6.65343162033362,12.4093182733649));
#55046=CARTESIAN_POINT('Ctrl Pts',(-61.3386809921953,6.63733318178291,12.5311923351786));
#55047=CARTESIAN_POINT('Ctrl Pts',(-61.2204712761571,6.62104377694539,12.6511854446751));
#55048=CARTESIAN_POINT('Ctrl Pts',(-61.2199200988289,6.62096782421546,12.6517449374453));
#55049=CARTESIAN_POINT('Ctrl Pts',(-61.2193688737375,6.62089186653554,12.6523043884547));
#55050=CARTESIAN_POINT('Ctrl Pts',(-61.2188176008955,6.62081590390381,12.652863797695));
#55051=CARTESIAN_POINT('',(-65.7394232394244,7.26094188381232,0.668649941455471));
#55052=CARTESIAN_POINT('Ctrl Pts',(-65.7395827156737,7.26124220258481,0.671033071149472));
#55053=CARTESIAN_POINT('Ctrl Pts',(-65.9020867768559,7.22064705772462,2.65598726978187));
#55054=CARTESIAN_POINT('Ctrl Pts',(-65.5865610442786,7.25403397826185,4.71036142108621));
#55055=CARTESIAN_POINT('Ctrl Pts',(-64.9284491122907,7.16443381643712,6.63636663678025));
#55056=CARTESIAN_POINT('',(-64.0795635270123,7.11304235593188,-4.92051130426413));
#55057=CARTESIAN_POINT('Ctrl Pts',(-64.0835337535963,7.11077786349443,-4.91454011088298));
#55058=CARTESIAN_POINT('Ctrl Pts',(-64.1323411238627,7.10143308976583,-4.82718197003987));
#55059=CARTESIAN_POINT('Ctrl Pts',(-64.1802005667353,7.09364154317148,-4.73875740081963));
#55060=CARTESIAN_POINT('Ctrl Pts',(-64.2272039770873,7.0873437062873,-4.64918122502579));
#55061=CARTESIAN_POINT('Ctrl Pts',(-64.2731661376042,7.08118538314411,-4.56158939840107));
#55062=CARTESIAN_POINT('Ctrl Pts',(-64.3183102368122,7.07645513160571,-4.47289638639061));
#55063=CARTESIAN_POINT('Ctrl Pts',(-64.362691913154,7.07305727552395,-4.38303080249611));
#55064=CARTESIAN_POINT('Ctrl Pts',(-64.407348532143,7.06963836986447,-4.29260850503057));
#55065=CARTESIAN_POINT('Ctrl Pts',(-64.4512334822151,7.06756810463911,-4.20099882935125));
#55066=CARTESIAN_POINT('Ctrl Pts',(-64.4943671378015,7.0667116387588,-4.10813965798429));
#55067=CARTESIAN_POINT('Ctrl Pts',(-64.538733872391,7.06583068874702,-4.0126258844766));
#55068=CARTESIAN_POINT('Ctrl Pts',(-64.5823058216986,7.06623345912329,-3.91578975174785));
#55069=CARTESIAN_POINT('Ctrl Pts',(-64.625064292327,7.06773963749489,-3.81757984118512));
#55070=CARTESIAN_POINT('Ctrl Pts',(-64.6366297318445,7.06814703314313,-3.79101572970186));
#55071=CARTESIAN_POINT('Ctrl Pts',(-64.6481354299698,7.06863499482074,-3.76435122011603));
#55072=CARTESIAN_POINT('Ctrl Pts',(-64.6595805256827,7.06919962896058,-3.73758555155824));
#55073=CARTESIAN_POINT('Ctrl Pts',(-64.7044712102175,7.07141427300421,-3.63260353884933));
#55074=CARTESIAN_POINT('Ctrl Pts',(-64.7484339464594,7.07480847542174,-3.52606497812548));
#55075=CARTESIAN_POINT('Ctrl Pts',(-64.791404704864,7.07913848472074,-3.41808155276295));
#55076=CARTESIAN_POINT('Ctrl Pts',(-64.8142018012916,7.0814356664133,-3.3607935585087));
#55077=CARTESIAN_POINT('Ctrl Pts',(-64.8367187512787,7.08399620397509,-3.30309898433251));
#55078=CARTESIAN_POINT('Ctrl Pts',(-64.858940198642,7.08678381264196,-3.24501532835008));
#55079=CARTESIAN_POINT('Ctrl Pts',(-64.9045049237743,7.09249975997003,-3.12591571362922));
#55080=CARTESIAN_POINT('Ctrl Pts',(-64.9488302632029,7.09916995637793,-3.00517924810612));
#55081=CARTESIAN_POINT('Ctrl Pts',(-64.9917455430339,7.10648781659526,-2.88297777630594));
#55082=CARTESIAN_POINT('Ctrl Pts',(-65.0375600701317,7.11430005285572,-2.75252068355919));
#55083=CARTESIAN_POINT('Ctrl Pts',(-65.0817671166487,7.12284975587435,-2.62039419187577));
#55084=CARTESIAN_POINT('Ctrl Pts',(-65.1241037097651,7.13177696281216,-2.48682213043831));
#55085=CARTESIAN_POINT('Ctrl Pts',(-65.1318590972489,7.1334122845009,-2.46235386274833));
#55086=CARTESIAN_POINT('Ctrl Pts',(-65.1395515909995,7.13506032430707,-2.43783711801167));
#55087=CARTESIAN_POINT('Ctrl Pts',(-65.147179412765,7.13671894382896,-2.41327330962486));
#55088=CARTESIAN_POINT('Ctrl Pts',(-65.1548093866202,7.13837803130856,-2.38870257088207));
#55089=CARTESIAN_POINT('Ctrl Pts',(-65.162374652527,7.14004770064065,-2.36408474166654));
#55090=CARTESIAN_POINT('Ctrl Pts',(-65.1698737946742,7.14172531456448,-2.33942154267057));
#55091=CARTESIAN_POINT('Ctrl Pts',(-65.2102039449649,7.15074746941242,-2.20678363520819));
#55092=CARTESIAN_POINT('Ctrl Pts',(-65.2488912851349,7.16005021608417,-2.07258936172927));
#55093=CARTESIAN_POINT('Ctrl Pts',(-65.2858205099729,7.16927502780963,-1.93704689908791));
#55094=CARTESIAN_POINT('Ctrl Pts',(-65.3077327593675,7.17474864324654,-1.8566217004009));
#55095=CARTESIAN_POINT('Ctrl Pts',(-65.3290254015679,7.18019570057733,-1.77572190701815));
#55096=CARTESIAN_POINT('Ctrl Pts',(-65.3496700473213,7.18554871571595,-1.69439082134555));
#55097=CARTESIAN_POINT('Ctrl Pts',(-65.385357852192,7.19480231890289,-1.55379611460786));
#55098=CARTESIAN_POINT('Ctrl Pts',(-65.4191095339481,7.20377199941432,-1.4119135129394));
#55099=CARTESIAN_POINT('Ctrl Pts',(-65.4507698563869,7.21212018115951,-1.26909214155907));
#55100=CARTESIAN_POINT('Ctrl Pts',(-65.4750302946932,7.21851716427901,-1.15965203475376));
#55101=CARTESIAN_POINT('Ctrl Pts',(-65.498062302265,7.22455029649033,-1.04966052491815));
#55102=CARTESIAN_POINT('Ctrl Pts',(-65.5197944063732,7.23008731297395,-0.939268302285297));
#55103=CARTESIAN_POINT('Ctrl Pts',(-65.524236410554,7.23121906948712,-0.916704324493633));
#55104=CARTESIAN_POINT('Ctrl Pts',(-65.5286241098133,7.23233015301656,-0.894123582617326));
#55105=CARTESIAN_POINT('Ctrl Pts',(-65.5329569904809,7.2334191756638,-0.871526032417236));
#55106=CARTESIAN_POINT('Ctrl Pts',(-65.5570702056107,7.23947977123251,-0.745766836359672));
#55107=CARTESIAN_POINT('Ctrl Pts',(-65.5794867225205,7.24485641788753,-0.619490657946675));
#55108=CARTESIAN_POINT('Ctrl Pts',(-65.6001882638281,7.24934156066612,-0.492123250458605));
#55109=CARTESIAN_POINT('Ctrl Pts',(-65.6185807063574,7.25332642003314,-0.378962704220613));
#55110=CARTESIAN_POINT('Ctrl Pts',(-65.6356193472249,7.25660864722147,-0.264940523657192));
#55111=CARTESIAN_POINT('Ctrl Pts',(-65.6512872325861,7.25903990662824,-0.149619654441558));
#55112=CARTESIAN_POINT('Ctrl Pts',(-65.6531503494619,7.25932901523006,-0.135906491968494));
#55113=CARTESIAN_POINT('Ctrl Pts',(-65.6549940787113,7.25960607744851,-0.122174923828413));
#55114=CARTESIAN_POINT('Ctrl Pts',(-65.6568183790756,7.25987084800059,-0.10842604919408));
#55115=CARTESIAN_POINT('Ctrl Pts',(-65.6645280546458,7.26098979480182,-0.0503219316038178));
#55116=CARTESIAN_POINT('Ctrl Pts',(-65.6718710057134,7.26188323443358,0.00675034893310512));
#55117=CARTESIAN_POINT('Ctrl Pts',(-65.6788643662617,7.26255350370653,0.0633737642326929));
#55118=CARTESIAN_POINT('Ctrl Pts',(-65.686925212884,7.26332608475218,0.128640335691545));
#55119=CARTESIAN_POINT('Ctrl Pts',(-65.6945220442716,7.26380328978071,0.193312839132918));
#55120=CARTESIAN_POINT('Ctrl Pts',(-65.7016657796718,7.26396077863301,0.258338263786383));
#55121=CARTESIAN_POINT('Ctrl Pts',(-65.7058603841224,7.2640532517446,0.296519400176069));
#55122=CARTESIAN_POINT('Ctrl Pts',(-65.7098984505169,7.26403499039114,0.334820379179476));
#55123=CARTESIAN_POINT('Ctrl Pts',(-65.713780714574,7.26388377792568,0.37383220486236));
#55124=CARTESIAN_POINT('Ctrl Pts',(-65.7167673931564,7.26376744811778,0.403844533367242));
#55125=CARTESIAN_POINT('Ctrl Pts',(-65.7196618187443,7.2635723487753,0.434277416501284));
#55126=CARTESIAN_POINT('Ctrl Pts',(-65.7224634125073,7.2632854179205,0.46542151022431));
#55127=CARTESIAN_POINT('Ctrl Pts',(-65.7245218275605,7.26307460120662,0.488304010957459));
#55128=CARTESIAN_POINT('Ctrl Pts',(-65.7265301305615,7.26281402466057,0.511575469365943));
#55129=CARTESIAN_POINT('Ctrl Pts',(-65.7284858187154,7.26251260512385,0.534798711637291));
#55130=CARTESIAN_POINT('Ctrl Pts',(-65.7303609092576,7.26222360765695,0.557064880123483));
#55131=CARTESIAN_POINT('Ctrl Pts',(-65.7321876345632,7.26189704344469,0.579287553385808));
#55132=CARTESIAN_POINT('Ctrl Pts',(-65.7339633481816,7.26154152718023,0.601031873391619));
#55133=CARTESIAN_POINT('Ctrl Pts',(-65.7355811316233,7.26121763017347,0.620842275525464));
#55134=CARTESIAN_POINT('Ctrl Pts',(-65.7371565718029,7.26086969558048,0.640255744443095));
#55135=CARTESIAN_POINT('Ctrl Pts',(-65.7386872986922,7.26050504824662,0.658895929602836));
#55136=CARTESIAN_POINT('Ctrl Pts',(-65.7388367302922,7.26046945088766,0.660715609333391));
#55137=CARTESIAN_POINT('Ctrl Pts',(-65.7389857354748,7.26043369499359,0.662527878289384));
#55138=CARTESIAN_POINT('Ctrl Pts',(-65.7391343118341,7.26039778787535,0.664332358598316));
#55139=CARTESIAN_POINT('',(-59.0504798555313,7.75485996799304,-10.7041909447736));
#55140=CARTESIAN_POINT('Ctrl Pts',(-59.0504798555313,7.75485996799304,-10.7041909447736));
#55141=CARTESIAN_POINT('Ctrl Pts',(-60.0796098167125,7.87873199265082,-9.96197480208937));
#55142=CARTESIAN_POINT('Ctrl Pts',(-62.0660466287397,7.97403730548955,-8.03642045404962));
#55143=CARTESIAN_POINT('Ctrl Pts',(-63.5230316254146,7.22290795330965,-5.91353180077074));
#55144=CARTESIAN_POINT('Ctrl Pts',(-64.0795059534616,7.11307519407537,-4.92059789448709));
#55145=CARTESIAN_POINT('',(-41.3402244866054,4.38233490926977,-11.3195856097259));
#55146=CARTESIAN_POINT('Ctrl Pts',(-41.3402244866054,4.38233490926977,-11.3195856097259));
#55147=CARTESIAN_POINT('Ctrl Pts',(-41.9985023915937,4.44701923023704,-11.7653170427634));
#55148=CARTESIAN_POINT('Ctrl Pts',(-43.3908039796773,4.61571635395792,-12.5174764940247));
#55149=CARTESIAN_POINT('Ctrl Pts',(-46.1914722110254,5.3927514423487,-13.3156545423547));
#55150=CARTESIAN_POINT('Ctrl Pts',(-49.9948035131066,7.02745080169609,-13.706606972641));
#55151=CARTESIAN_POINT('Ctrl Pts',(-54.1289712559167,7.53905427079786,-13.0742974757744));
#55152=CARTESIAN_POINT('Ctrl Pts',(-56.7102378337881,7.56456386339554,-12.0170276546053));
#55153=CARTESIAN_POINT('Ctrl Pts',(-57.9084119982073,7.63003527898566,-11.4010944726287));
#55154=CARTESIAN_POINT('Ctrl Pts',(-58.5678160077699,7.69080724613176,-11.0134367986666));
#55155=CARTESIAN_POINT('Ctrl Pts',(-58.8883897060344,7.73532762094072,-10.8209468457134));
#55156=CARTESIAN_POINT('Ctrl Pts',(-59.0486785764031,7.75464303119201,-10.7054892315628));
#55157=CARTESIAN_POINT('',(-36.1360059330621,4.15901206247279,-5.40582646581216));
#55158=CARTESIAN_POINT('Ctrl Pts',(-36.1360059330621,4.15901206247279,-5.40582646581216));
#55159=CARTESIAN_POINT('Ctrl Pts',(-36.735234866715,4.17590258588924,-6.60510917508678));
#55160=CARTESIAN_POINT('Ctrl Pts',(-37.85694008542,4.21051024093903,-8.27236172411371));
#55161=CARTESIAN_POINT('Ctrl Pts',(-39.7542446236388,4.26982122872605,-10.1775780089158));
#55162=CARTESIAN_POINT('Ctrl Pts',(-40.8013703910201,4.32944548953245,-10.9546239517306));
#55163=CARTESIAN_POINT('Ctrl Pts',(-41.3379913976662,4.38211560392107,-11.3180733508353));
#55164=CARTESIAN_POINT('Ctrl Pts',(-35.0820169555422,4.1311553285547,-2.69386316078375));
#55165=CARTESIAN_POINT('Ctrl Pts',(-35.3472499758451,4.13782412394816,-3.62262376308943));
#55166=CARTESIAN_POINT('Ctrl Pts',(-35.7008401684657,4.14674629646921,-4.53483852841008));
#55167=CARTESIAN_POINT('Ctrl Pts',(-36.135822819044,4.15900690108209,-5.40545997363959));
#55168=CARTESIAN_POINT('',(3.02589869591714,2.03453539417915,-29.481040542818));
#55169=CARTESIAN_POINT('',(1.7019170311789,1.9841758627661,-32.7826729204701));
#55170=CARTESIAN_POINT('Ctrl Pts',(3.02620767763066,2.03445931614535,-29.482369472598));
#55171=CARTESIAN_POINT('Ctrl Pts',(3.20555263301232,2.02375902210562,-30.2475171721583));
#55172=CARTESIAN_POINT('Ctrl Pts',(3.02661590274896,1.96081108314947,-31.598486221152));
#55173=CARTESIAN_POINT('Ctrl Pts',(2.12920577407486,1.97332831724216,-32.5206340925411));
#55174=CARTESIAN_POINT('Ctrl Pts',(1.7019170311789,1.9841758627661,-32.7826729204701));
#55175=CARTESIAN_POINT('',(-3.02596826212615,2.03432873875274,-29.4800060173015));
#55176=CARTESIAN_POINT('Ctrl Pts',(-3.0255268228659,2.03435552877844,-29.4781858978988));
#55177=CARTESIAN_POINT('Ctrl Pts',(-2.89748980529269,2.04212655242135,-28.9515397139976));
#55178=CARTESIAN_POINT('Ctrl Pts',(-2.34728642075398,2.07624236465954,-27.9637381387751));
#55179=CARTESIAN_POINT('Ctrl Pts',(-0.86527131205636,2.14132533286026,-27.1055607008419));
#55180=CARTESIAN_POINT('Ctrl Pts',(0.863471086326564,2.14121820993117,-27.1043323065609));
#55181=CARTESIAN_POINT('Ctrl Pts',(2.10137698734444,2.08724640507052,-27.8170592929481));
#55182=CARTESIAN_POINT('Ctrl Pts',(2.75995282450495,2.0506331663776,-28.6996503464524));
#55183=CARTESIAN_POINT('Ctrl Pts',(2.9604184742133,2.03838594914446,-29.2034367727384));
#55184=CARTESIAN_POINT('Ctrl Pts',(3.02523930059986,2.0345171033467,-29.4782510284727));
#55185=CARTESIAN_POINT('Ctrl Pts',(1.7019170311789,1.9841758627661,-32.7826729204701));
#55186=CARTESIAN_POINT('Ctrl Pts',(1.28857863702931,1.99466925188967,-33.036156566229));
#55187=CARTESIAN_POINT('Ctrl Pts',(0.321543600862733,2.02241016559728,-33.3511773448253));
#55188=CARTESIAN_POINT('Ctrl Pts',(-1.19853457360234,2.00220690733558,-33.1534394779125));
#55189=CARTESIAN_POINT('Ctrl Pts',(-2.44599217953573,1.95940735428246,-32.3264040160697));
#55190=CARTESIAN_POINT('Ctrl Pts',(-3.02438609187982,1.98457308078909,-31.2166546642125));
#55191=CARTESIAN_POINT('Ctrl Pts',(-3.14100419297298,2.01861532274412,-30.2293427451567));
#55192=CARTESIAN_POINT('Ctrl Pts',(-3.08328115399646,2.03085086602267,-29.7168832273726));
#55193=CARTESIAN_POINT('Ctrl Pts',(-3.02628868373051,2.03430929303555,-29.4813271629984));
#55194=CARTESIAN_POINT('',(2.75100840866463,2.05012843941995,-23.4599303049991));
#55195=CARTESIAN_POINT('',(1.61567592638144,2.10484535966067,-24.6418414854819));
#55196=CARTESIAN_POINT('Ctrl Pts',(2.75100552264243,2.05012860052275,-23.459935693484));
#55197=CARTESIAN_POINT('Ctrl Pts',(2.4917371536323,2.06460141183357,-23.9440137803207));
#55198=CARTESIAN_POINT('Ctrl Pts',(2.09220096563961,2.08654257832164,-24.3598140131154));
#55199=CARTESIAN_POINT('Ctrl Pts',(1.61567592638144,2.10484535966067,-24.6418414854819));
#55200=CARTESIAN_POINT('',(-2.75095635228815,2.0500785577562,-23.4601289752605));
#55201=CARTESIAN_POINT('Ctrl Pts',(-2.75104415575314,2.04996283861984,-23.459954551535));
#55202=CARTESIAN_POINT('Ctrl Pts',(-3.14697228957638,2.02797021966844,-22.7225859102412));
#55203=CARTESIAN_POINT('Ctrl Pts',(-3.28470830566268,2.01818671464134,-20.9006764566282));
#55204=CARTESIAN_POINT('Ctrl Pts',(-1.71693918475569,2.11168339882122,-19.2349389943924));
#55205=CARTESIAN_POINT('Ctrl Pts',(-5.68372511193975E-5,2.14348108036939,
-18.8971771498333));
#55206=CARTESIAN_POINT('Ctrl Pts',(1.71728341750388,2.11146607039885,-19.2336854760647));
#55207=CARTESIAN_POINT('Ctrl Pts',(3.28527599025147,2.01819903914408,-20.9040176508014));
#55208=CARTESIAN_POINT('Ctrl Pts',(3.14638608131475,2.02805776491796,-22.7217197351585));
#55209=CARTESIAN_POINT('Ctrl Pts',(2.75100840866463,2.05012843941995,-23.4599303049991));
#55210=CARTESIAN_POINT('Ctrl Pts',(1.61567592638144,2.10484535966067,-24.6418414854819));
#55211=CARTESIAN_POINT('Ctrl Pts',(1.04038344114352,2.12694168555298,-24.9823236681931));
#55212=CARTESIAN_POINT('Ctrl Pts',(-0.182315527702726,2.1513398143738,-25.2447478054221));
#55213=CARTESIAN_POINT('Ctrl Pts',(-1.8215791399191,2.10154489826223,-24.6600514792354));
#55214=CARTESIAN_POINT('Ctrl Pts',(-2.51542689144179,2.06305029395261,-23.8984874041331));
#55215=CARTESIAN_POINT('Ctrl Pts',(-2.75069164890588,2.04998241903505,-23.4606108465542));
#55216=CARTESIAN_POINT('Ctrl Pts',(-36.0549975098271,1.0528127756878,-2.38156518037249));
#55217=CARTESIAN_POINT('Ctrl Pts',(-36.3055439100197,1.05947580029909,-3.26356670979119));
#55218=CARTESIAN_POINT('Ctrl Pts',(-36.6408912827729,1.0685194404478,-4.1293438871194));
#55219=CARTESIAN_POINT('Ctrl Pts',(-37.6383467540235,1.09756433969661,-6.1123912328036));
#55220=CARTESIAN_POINT('Ctrl Pts',(-39.0798375037675,1.14868878793061,-8.2395365565181));
#55221=CARTESIAN_POINT('Ctrl Pts',(-41.0527618672285,1.2073272187152,-9.94414705234827));
#55222=CARTESIAN_POINT('Ctrl Pts',(-42.7057446504772,1.37815356390123,-11.0289708344873));
#55223=CARTESIAN_POINT('Ctrl Pts',(-43.9254694159358,1.53436264077785,-11.7104906826344));
#55224=CARTESIAN_POINT('Ctrl Pts',(-46.4982294500662,2.17389001321762,-12.6997150872518));
#55225=CARTESIAN_POINT('Ctrl Pts',(-49.146908121031,3.18680258560818,-13.126588408564));
#55226=CARTESIAN_POINT('Ctrl Pts',(-52.2274475031305,3.91643241459121,-12.9928561969852));
#55227=CARTESIAN_POINT('Ctrl Pts',(-54.304794246108,4.12355684923066,-12.5232019348578));
#55228=CARTESIAN_POINT('Ctrl Pts',(-56.2616035231788,4.24838602596462,-11.771250103581));
#55229=CARTESIAN_POINT('Ctrl Pts',(-57.2017281607085,4.31931888732918,-11.2901555467756));
#55230=CARTESIAN_POINT('Ctrl Pts',(-58.0855152875449,4.42766154699302,-10.7543378595292));
#55231=CARTESIAN_POINT('Ctrl Pts',(-58.6455973785906,4.50104299766934,-10.3873810885685));
#55232=CARTESIAN_POINT('Ctrl Pts',(-59.7051812089351,4.62670775817537,-9.58743591765393));
#55233=CARTESIAN_POINT('Ctrl Pts',(-61.3073010844994,4.69820828480475,-8.09568859876704));
#55234=CARTESIAN_POINT('Ctrl Pts',(-62.4948759707816,4.24202197752351,-6.47656645464623));
#55235=CARTESIAN_POINT('Ctrl Pts',(-63.1244186765201,4.05382187176954,-5.31872941631596));
#55236=CARTESIAN_POINT('Ctrl Pts',(-63.553812419201,3.95238147285607,-4.49832460967661));
#55237=CARTESIAN_POINT('Ctrl Pts',(-64.1594826858112,3.94362994185027,-3.07561996126338));
#55238=CARTESIAN_POINT('Ctrl Pts',(-64.6533034252321,4.13724389424319,-1.12169408361937));
#55239=CARTESIAN_POINT('Ctrl Pts',(-64.8054164174362,4.18825541443859,0.14378394163381));
#55240=CARTESIAN_POINT('Ctrl Pts',(-64.8433184824513,4.17721322512098,0.712263787109276));
#55241=CARTESIAN_POINT('Ctrl Pts',(-64.8578491520905,4.17264647741419,0.9518443795634));
#55242=CARTESIAN_POINT('Ctrl Pts',(-64.8752061422976,4.16523924168687,1.43110149180136));
#55243=CARTESIAN_POINT('Ctrl Pts',(-64.8689819333809,4.15580967855481,2.33145574074262));
#55244=CARTESIAN_POINT('Ctrl Pts',(-64.735236304878,4.14969563886838,3.99635849634215));
#55245=CARTESIAN_POINT('Ctrl Pts',(-64.4136362028236,4.12346149799371,5.39715323956259));
#55246=CARTESIAN_POINT('Ctrl Pts',(-63.8396954291777,4.03789832143775,7.10460988677013));
#55247=CARTESIAN_POINT('Ctrl Pts',(-62.9522024951476,3.89240808333474,9.15158202965359));
#55248=CARTESIAN_POINT('Ctrl Pts',(-61.6207408360306,3.67379600611113,10.9504902331086));
#55249=CARTESIAN_POINT('Ctrl Pts',(-58.7632410796701,3.26700669501724,13.8580023828708));
#55250=CARTESIAN_POINT('Ctrl Pts',(-55.2909382628842,2.70208941668797,15.8250391551239));
#55251=CARTESIAN_POINT('Ctrl Pts',(-48.0383621414291,1.75314527999541,16.7544202746464));
#55252=CARTESIAN_POINT('Ctrl Pts',(-42.9494969015026,1.3477622455303,14.9599652046533));
#55253=CARTESIAN_POINT('Ctrl Pts',(-40.0709952890308,1.20105054797173,12.2933217048773));
#55254=CARTESIAN_POINT('Ctrl Pts',(-39.1374904320878,1.1557136830438,11.3477424017553));
#55255=CARTESIAN_POINT('Ctrl Pts',(-37.7188277175619,1.09649931876771,9.64176435135193));
#55256=CARTESIAN_POINT('Ctrl Pts',(-36.7050062286424,1.06766764201769,7.63136101756027));
#55257=CARTESIAN_POINT('Ctrl Pts',(-35.6516839503182,1.04076735648636,4.50019397537972));
#55258=CARTESIAN_POINT('Ctrl Pts',(-35.4031603226107,1.03589678751514,2.5790344470455));
#55259=CARTESIAN_POINT('Ctrl Pts',(-35.5943183545488,1.04064036797772,-0.357304714959154));
#55260=CARTESIAN_POINT('Ctrl Pts',(-35.7726531517491,1.04530411699111,-1.38762491439351));
#55261=CARTESIAN_POINT('Ctrl Pts',(-36.0549975098271,1.0528127756878,-2.3815651803725));
#55262=CARTESIAN_POINT('Ctrl Pts',(-36.0555939497443,0.904484667441714,
-2.38244503347954));
#55263=CARTESIAN_POINT('Ctrl Pts',(-36.3062567268876,0.911222945188725,
-3.26462769997687));
#55264=CARTESIAN_POINT('Ctrl Pts',(-36.6417190294816,0.920392628576229,
-4.13054503564706));
#55265=CARTESIAN_POINT('Ctrl Pts',(-37.6400317392652,0.949603777841035,
-6.11448651724083));
#55266=CARTESIAN_POINT('Ctrl Pts',(-39.0812931660259,1.00146080909335,-8.24071227119904));
#55267=CARTESIAN_POINT('Ctrl Pts',(-41.0571520775041,1.058676413563,-9.94781725293408));
#55268=CARTESIAN_POINT('Ctrl Pts',(-42.7190199509979,1.22650923997694,-11.0365782464944));
#55269=CARTESIAN_POINT('Ctrl Pts',(-43.9458025053604,1.38117579517859,-11.7205907593239));
#55270=CARTESIAN_POINT('Ctrl Pts',(-46.5493430056267,2.00732942103926,-12.7149357794429));
#55271=CARTESIAN_POINT('Ctrl Pts',(-49.2086162954305,2.99676762410914,-13.1287136767877));
#55272=CARTESIAN_POINT('Ctrl Pts',(-52.2577461319444,3.70830093718569,-12.9861164884077));
#55273=CARTESIAN_POINT('Ctrl Pts',(-54.3176790478885,3.91571550975409,-12.5183560303513));
#55274=CARTESIAN_POINT('Ctrl Pts',(-56.2712243588391,4.04550672280604,-11.766236506535));
#55275=CARTESIAN_POINT('Ctrl Pts',(-57.2153673507245,4.12163827308303,-11.2822410862027));
#55276=CARTESIAN_POINT('Ctrl Pts',(-58.102252377271,4.23385380952422,-10.7429529768583));
#55277=CARTESIAN_POINT('Ctrl Pts',(-58.6604423297125,4.30678598655203,-10.37617396621));
#55278=CARTESIAN_POINT('Ctrl Pts',(-59.7153301961589,4.43155309898789,-9.57750241559074));
#55279=CARTESIAN_POINT('Ctrl Pts',(-61.2908741299189,4.50077347501871,-8.10847394371011));
#55280=CARTESIAN_POINT('Ctrl Pts',(-62.4722805388144,4.0598548345074,-6.51133116997329));
#55281=CARTESIAN_POINT('Ctrl Pts',(-63.1141505984817,3.87574923768064,-5.33689586275052));
#55282=CARTESIAN_POINT('Ctrl Pts',(-63.5512241737457,3.77783013568088,-4.50433690621057));
#55283=CARTESIAN_POINT('Ctrl Pts',(-64.1634629023857,3.77430690726006,-3.06490045526055));
#55284=CARTESIAN_POINT('Ctrl Pts',(-64.6550498983541,3.97353574719654,-1.10801283943642));
#55285=CARTESIAN_POINT('Ctrl Pts',(-64.8051375979326,4.02693314861109,0.147101311648772));
#55286=CARTESIAN_POINT('Ctrl Pts',(-64.8427246461288,4.01690539467727,0.709043311905127));
#55287=CARTESIAN_POINT('Ctrl Pts',(-64.8573586797898,4.01277167274026,0.949436098755388));
#55288=CARTESIAN_POINT('Ctrl Pts',(-64.8747862570427,4.00596589881556,1.42891266008647));
#55289=CARTESIAN_POINT('Ctrl Pts',(-64.8686835673502,3.99696796876503,2.3306272191874));
#55290=CARTESIAN_POINT('Ctrl Pts',(-64.7348567544036,3.98971137788843,3.99538790298088));
#55291=CARTESIAN_POINT('Ctrl Pts',(-64.4142860107865,3.96181921816279,5.39245691306954));
#55292=CARTESIAN_POINT('Ctrl Pts',(-63.8425047226651,3.8763093951887,7.09608474134876));
#55293=CARTESIAN_POINT('Ctrl Pts',(-62.958566432785,3.7311154604734,9.13944093727611));
#55294=CARTESIAN_POINT('Ctrl Pts',(-61.6293277697593,3.51429001249069,10.9391823544689));
#55295=CARTESIAN_POINT('Ctrl Pts',(-58.7777794785863,3.10978159513787,13.8465999095765));
#55296=CARTESIAN_POINT('Ctrl Pts',(-55.3120622199062,2.54885112777169,15.8174374982029));
#55297=CARTESIAN_POINT('Ctrl Pts',(-48.0528651919166,1.60552999596159,16.7577861953313));
#55298=CARTESIAN_POINT('Ctrl Pts',(-42.956881702099,1.20109260351356,14.9644289431498));
#55299=CARTESIAN_POINT('Ctrl Pts',(-40.0748747688297,1.0539287969232,12.296583589382));
#55300=CARTESIAN_POINT('Ctrl Pts',(-39.1403720142934,1.00843546237801,11.350577888442));
#55301=CARTESIAN_POINT('Ctrl Pts',(-37.7203617502752,0.948875201418379,
9.64381909341719));
#55302=CARTESIAN_POINT('Ctrl Pts',(-36.705921936741,0.919660734901868,7.63269341173704));
#55303=CARTESIAN_POINT('Ctrl Pts',(-35.6520519680447,0.892335839803674,
4.50068627822135));
#55304=CARTESIAN_POINT('Ctrl Pts',(-35.4034621866083,0.887355587669725,
2.57923003175189));
#55305=CARTESIAN_POINT('Ctrl Pts',(-35.5946982044237,0.892169363420933,
-0.357746184990163));
#55306=CARTESIAN_POINT('Ctrl Pts',(-35.7731184447994,0.896891204899179,
-1.38830064150969));
#55307=CARTESIAN_POINT('Ctrl Pts',(-36.0555939497443,0.904484667441719,
-2.38244503347954));
#55308=CARTESIAN_POINT('Ctrl Pts',(-35.9922681759013,0.608882116610321,
-2.40252489470072));
#55309=CARTESIAN_POINT('Ctrl Pts',(-36.2443785607268,0.615769948902191,
-3.28909825742476));
#55310=CARTESIAN_POINT('Ctrl Pts',(-36.5816919949173,0.625189340318007,
-4.15917917294117));
#55311=CARTESIAN_POINT('Ctrl Pts',(-37.5863972856988,0.654732027487002,
-6.1538645640023));
#55312=CARTESIAN_POINT('Ctrl Pts',(-39.0342187194187,0.708039659060072,
-8.28751826776375));
#55313=CARTESIAN_POINT('Ctrl Pts',(-41.0238977934904,0.762443843619788,
-10.0080550546168));
#55314=CARTESIAN_POINT('Ctrl Pts',(-42.7093426314559,0.924341288012181,
-11.1127801661199));
#55315=CARTESIAN_POINT('Ctrl Pts',(-43.9550916538701,1.07596757220897,-11.8065547998463));
#55316=CARTESIAN_POINT('Ctrl Pts',(-46.6258628903611,1.67564312080215,-12.8347074267587));
#55317=CARTESIAN_POINT('Ctrl Pts',(-49.3209792563777,2.61889807843932,-13.2552065788425));
#55318=CARTESIAN_POINT('Ctrl Pts',(-52.3365683940236,3.29462450617091,-13.1079278924267));
#55319=CARTESIAN_POINT('Ctrl Pts',(-54.3811675813475,3.50259527469106,-12.6377569789553));
#55320=CARTESIAN_POINT('Ctrl Pts',(-56.3432172769078,3.64215593963216,-11.8721821586535));
#55321=CARTESIAN_POINT('Ctrl Pts',(-57.3004435327768,3.72851730538224,-11.3729256118978));
#55322=CARTESIAN_POINT('Ctrl Pts',(-58.1983366806673,3.84837683953258,-10.8187721359246));
#55323=CARTESIAN_POINT('Ctrl Pts',(-58.7575257930806,3.92041942928577,-10.4498241116935));
#55324=CARTESIAN_POINT('Ctrl Pts',(-59.8115950408937,4.04339107950324,-9.64752989021953));
#55325=CARTESIAN_POINT('Ctrl Pts',(-61.3488447008931,4.10808603220261,-8.21282218706084));
#55326=CARTESIAN_POINT('Ctrl Pts',(-62.5172938429767,3.69736142138752,-6.63867657150117));
#55327=CARTESIAN_POINT('Ctrl Pts',(-63.180538680225,3.52130030141665,-5.41964915825797));
#55328=CARTESIAN_POINT('Ctrl Pts',(-63.6308402479908,3.43032212436478,-4.55486496656474));
#55329=CARTESIAN_POINT('Ctrl Pts',(-64.2552005173933,3.43711541496265,-3.07145772521243));
#55330=CARTESIAN_POINT('Ctrl Pts',(-64.7398338150334,3.64746919653615,-1.09596732690597));
#55331=CARTESIAN_POINT('Ctrl Pts',(-64.883657444038,3.70557613317877,0.145685389858161));
#55332=CARTESIAN_POINT('Ctrl Pts',(-64.9199369800284,3.69755989799623,0.697703834262555));
#55333=CARTESIAN_POINT('Ctrl Pts',(-64.9344053541345,3.69428520684122,0.941028798737093));
#55334=CARTESIAN_POINT('Ctrl Pts',(-64.9514652230736,3.68867191422421,1.42351021989472));
#55335=CARTESIAN_POINT('Ctrl Pts',(-64.9451323226112,3.68052822707428,2.33266296731874));
#55336=CARTESIAN_POINT('Ctrl Pts',(-64.8115806130686,3.67100337684105,4.00597005240495));
#55337=CARTESIAN_POINT('Ctrl Pts',(-64.4930085401915,3.6398247492517,5.40357234851391));
#55338=CARTESIAN_POINT('Ctrl Pts',(-63.9225371750656,3.55442398498814,7.10889226910018));
#55339=CARTESIAN_POINT('Ctrl Pts',(-63.0407763459327,3.40982158427969,9.15635693290283));
#55340=CARTESIAN_POINT('Ctrl Pts',(-61.7073917428413,3.19653576750585,10.9664076276178));
#55341=CARTESIAN_POINT('Ctrl Pts',(-58.8512171752399,2.79654951543426,13.8877565738267));
#55342=CARTESIAN_POINT('Ctrl Pts',(-55.3788151857701,2.24352248023264,15.8731131092571));
#55343=CARTESIAN_POINT('Ctrl Pts',(-48.0711268741737,1.31134848387323,16.8333529503183));
#55344=CARTESIAN_POINT('Ctrl Pts',(-42.9393497504966,0.908782583618137,
15.0329488636439));
#55345=CARTESIAN_POINT('Ctrl Pts',(-40.037135888014,0.76072091085068,12.3510345169592));
#55346=CARTESIAN_POINT('Ctrl Pts',(-39.0963650953478,0.714916638110273,
11.3999947936465));
#55347=CARTESIAN_POINT('Ctrl Pts',(-37.6670519522153,0.654669347149692,
9.68416817237497));
#55348=CARTESIAN_POINT('Ctrl Pts',(-36.6464607599348,0.624695100829358,
7.66263154429121));
#55349=CARTESIAN_POINT('Ctrl Pts',(-35.586343168216,0.59652792171092,4.51480593811151));
#55350=CARTESIAN_POINT('Ctrl Pts',(-35.3363720722281,0.591329963871329,
2.58396879028904));
#55351=CARTESIAN_POINT('Ctrl Pts',(-35.5287065927405,0.596283167752303,
-0.367726615960636));
#55352=CARTESIAN_POINT('Ctrl Pts',(-35.7081613409452,0.601120118890534,
-1.40343256371961));
#55353=CARTESIAN_POINT('Ctrl Pts',(-35.9922681759013,0.608882116610323,
-2.40252489470072));
#55354=CARTESIAN_POINT('Ctrl Pts',(-35.6788452868189,0.190821093669241,
-2.49451532637507));
#55355=CARTESIAN_POINT('Ctrl Pts',(-35.9371748016095,0.197823785522891,
-3.40120776118929));
#55356=CARTESIAN_POINT('Ctrl Pts',(-36.282732356387,0.207442112280784,-4.29073825142866));
#55357=CARTESIAN_POINT('Ctrl Pts',(-37.3127391006884,0.237223038563802,
-6.33180135183161));
#55358=CARTESIAN_POINT('Ctrl Pts',(-38.7939215560336,0.291757553947807,
-8.50810321664163));
#55359=CARTESIAN_POINT('Ctrl Pts',(-40.831367727429,0.343809372406078,-10.2771054693631));
#55360=CARTESIAN_POINT('Ctrl Pts',(-42.5704878635999,0.502424780495082,
-11.4310756317738));
#55361=CARTESIAN_POINT('Ctrl Pts',(-43.8601407661417,0.65251648547724,-12.1548977466516));
#55362=CARTESIAN_POINT('Ctrl Pts',(-46.6405321830093,1.24431899385572,-13.3013571802195));
#55363=CARTESIAN_POINT('Ctrl Pts',(-49.4150466416309,2.17965774129795,-13.8276699904443));
#55364=CARTESIAN_POINT('Ctrl Pts',(-52.487289380987,2.84182050128404,-13.7124729474502));
#55365=CARTESIAN_POINT('Ctrl Pts',(-54.5834122822819,3.04709747487405,-13.2191083636475));
#55366=CARTESIAN_POINT('Ctrl Pts',(-56.6086890147239,3.18486064563698,-12.396446266628));
#55367=CARTESIAN_POINT('Ctrl Pts',(-57.6010557122091,3.27180967339437,-11.848924443058));
#55368=CARTESIAN_POINT('Ctrl Pts',(-58.5304988833242,3.39304237564432,-11.251201716693));
#55369=CARTESIAN_POINT('Ctrl Pts',(-59.1071788251335,3.46491928745013,-10.8706615658623));
#55370=CARTESIAN_POINT('Ctrl Pts',(-60.1895627849156,3.5861844069988,-10.0428303353042));
#55371=CARTESIAN_POINT('Ctrl Pts',(-61.7323526812202,3.64882218416258,-8.60872134074377));
#55372=CARTESIAN_POINT('Ctrl Pts',(-62.8852363599739,3.25177729002768,-6.99767453874843));
#55373=CARTESIAN_POINT('Ctrl Pts',(-63.5663559032184,3.07268589980912,-5.68650329864844));
#55374=CARTESIAN_POINT('Ctrl Pts',(-64.0280889424921,2.98137593833669,-4.7548806456604));
#55375=CARTESIAN_POINT('Ctrl Pts',(-64.6668361058713,2.99356768937731,-3.17739735347249));
#55376=CARTESIAN_POINT('Ctrl Pts',(-65.1359228942973,3.2101415043566,-1.13275347647021));
#55377=CARTESIAN_POINT('Ctrl Pts',(-65.2645995616865,3.2700027911371,0.11596751667424));
#55378=CARTESIAN_POINT('Ctrl Pts',(-65.2970672831498,3.26337755333429,0.665229271993136));
#55379=CARTESIAN_POINT('Ctrl Pts',(-65.3101975596581,3.2605905741402,0.917050306601995));
#55380=CARTESIAN_POINT('Ctrl Pts',(-65.3252187606999,3.2556972790431,1.41248776916539));
#55381=CARTESIAN_POINT('Ctrl Pts',(-65.3170768123695,3.24806453671255,2.34819404964879));
#55382=CARTESIAN_POINT('Ctrl Pts',(-65.1849806435554,3.23714367305903,4.06366048664381));
#55383=CARTESIAN_POINT('Ctrl Pts',(-64.8682585802219,3.20411847574444,5.48964402016827));
#55384=CARTESIAN_POINT('Ctrl Pts',(-64.2891191680327,3.11906713455525,7.22967412462136));
#55385=CARTESIAN_POINT('Ctrl Pts',(-63.3933532975505,2.97528454618844,9.32178548398929));
#55386=CARTESIAN_POINT('Ctrl Pts',(-62.0251967524475,2.76420001016156,11.176124232464));
#55387=CARTESIAN_POINT('Ctrl Pts',(-59.1061532670881,2.36758918865814,14.1656659960127));
#55388=CARTESIAN_POINT('Ctrl Pts',(-55.5571056026393,1.82037527149572,16.1958610845329));
#55389=CARTESIAN_POINT('Ctrl Pts',(-48.0605713766001,0.895007067307973,
17.1791038904439));
#55390=CARTESIAN_POINT('Ctrl Pts',(-42.8024300701058,0.493573724953808,
15.3372352360987));
#55391=CARTESIAN_POINT('Ctrl Pts',(-39.8257879925702,0.344597652056968,
12.594654996906));
#55392=CARTESIAN_POINT('Ctrl Pts',(-38.8613094672086,0.298515741742694,
11.6219453892284));
#55393=CARTESIAN_POINT('Ctrl Pts',(-37.3959267257012,0.237691755664316,
9.86716981758532));
#55394=CARTESIAN_POINT('Ctrl Pts',(-36.34967000299,0.207126063084511,7.79970934891721));
#55395=CARTESIAN_POINT('Ctrl Pts',(-35.2628987004346,0.178306255067115,
4.58036202846229));
#55396=CARTESIAN_POINT('Ctrl Pts',(-35.0066880334485,0.172944297082686,
2.60569473777376));
#55397=CARTESIAN_POINT('Ctrl Pts',(-35.2038137596613,0.178003560438737,
-0.413421569693999));
#55398=CARTESIAN_POINT('Ctrl Pts',(-35.387730024456,0.182929659049877,-1.47275052239072));
#55399=CARTESIAN_POINT('Ctrl Pts',(-35.6788452868189,0.19082109366924,-2.49451532637507));
#55400=CARTESIAN_POINT('Ctrl Pts',(-35.3280864353835,0.0555127849838203,
-2.59511145651185));
#55401=CARTESIAN_POINT('Ctrl Pts',(-35.5930227147958,0.0623741059613249,
-3.52382056888469));
#55402=CARTESIAN_POINT('Ctrl Pts',(-35.9474295279237,0.0717571238130431,
-4.43479293536763));
#55403=CARTESIAN_POINT('Ctrl Pts',(-37.0036313064953,0.101206985431967,
-6.52566825268797));
#55404=CARTESIAN_POINT('Ctrl Pts',(-38.5220700933842,0.154518393969504,
-8.75194826360237));
#55405=CARTESIAN_POINT('Ctrl Pts',(-40.6072512998611,0.209107862145042,
-10.5688352699363));
#55406=CARTESIAN_POINT('Ctrl Pts',(-42.3874676158688,0.376237052150697,
-11.7654874351406));
#55407=CARTESIAN_POINT('Ctrl Pts',(-43.7107791876456,0.531145971673501,
-12.515371429476));
#55408=CARTESIAN_POINT('Ctrl Pts',(-46.5430769526905,1.17496549761945,-13.7574803436035));
#55409=CARTESIAN_POINT('Ctrl Pts',(-49.3605442991523,2.20753320357867,-14.3726106319492));
#55410=CARTESIAN_POINT('Ctrl Pts',(-52.5532731257945,2.9243401122523,-14.2847163631391));
#55411=CARTESIAN_POINT('Ctrl Pts',(-54.7393178368275,3.12348754878638,-13.7687183927178));
#55412=CARTESIAN_POINT('Ctrl Pts',(-56.8359906168391,3.23569223062666,-12.9035548079215));
#55413=CARTESIAN_POINT('Ctrl Pts',(-57.8576327536343,3.29986469632328,-12.3254963884192));
#55414=CARTESIAN_POINT('Ctrl Pts',(-58.8145013408182,3.40586009857496,-11.6988424821367));
#55415=CARTESIAN_POINT('Ctrl Pts',(-59.4122362997243,3.47946714478885,-11.3058944870703));
#55416=CARTESIAN_POINT('Ctrl Pts',(-60.532919917232,3.60139924350621,-10.4502770318816));
#55417=CARTESIAN_POINT('Ctrl Pts',(-62.1418004651168,3.67048433387294,-8.96072780586377));
#55418=CARTESIAN_POINT('Ctrl Pts',(-63.3061607182308,3.22908091298505,-7.27825424542751));
#55419=CARTESIAN_POINT('Ctrl Pts',(-63.9855192119155,3.0237769607437,-5.91821784636985));
#55420=CARTESIAN_POINT('Ctrl Pts',(-64.4473654457923,2.91464681574267,-4.94982855292355));
#55421=CARTESIAN_POINT('Ctrl Pts',(-65.0922321521348,2.91163642890028,-3.31422240884912));
#55422=CARTESIAN_POINT('Ctrl Pts',(-65.5562709582115,3.11313222367988,-1.20317387586483));
#55423=CARTESIAN_POINT('Ctrl Pts',(-65.6765118300283,3.16440593553937,0.0764583233013215));
#55424=CARTESIAN_POINT('Ctrl Pts',(-65.7065113328794,3.15556766719144,0.637330258957667));
#55425=CARTESIAN_POINT('Ctrl Pts',(-65.7184356601194,3.1516252764093,0.896477679082247));
#55426=CARTESIAN_POINT('Ctrl Pts',(-65.7317238609617,3.14520008550437,1.40543165819501));
#55427=CARTESIAN_POINT('Ctrl Pts',(-65.7218096180503,3.13643053510135,2.36692751924055));
#55428=CARTESIAN_POINT('Ctrl Pts',(-65.5903053362458,3.12832565018766,4.12841315210705));
#55429=CARTESIAN_POINT('Ctrl Pts',(-65.2714249136872,3.09979578088586,5.59308771296452));
#55430=CARTESIAN_POINT('Ctrl Pts',(-64.6778956707148,3.01523526234882,7.37918415885639));
#55431=CARTESIAN_POINT('Ctrl Pts',(-63.7590738429973,2.87171165703166,9.52742689805567));
#55432=CARTESIAN_POINT('Ctrl Pts',(-62.3499639442105,2.65618062577662,11.4286796347776));
#55433=CARTESIAN_POINT('Ctrl Pts',(-59.3509400735407,2.2550704713425,14.4935263716135));
#55434=CARTESIAN_POINT('Ctrl Pts',(-55.7061987517473,1.6997474464948,16.5669811264171));
#55435=CARTESIAN_POINT('Ctrl Pts',(-48.0174632092897,0.759785836285453,
17.5572025721814));
#55436=CARTESIAN_POINT('Ctrl Pts',(-42.6326410688909,0.35574578981809,15.6677377197388));
#55437=CARTESIAN_POINT('Ctrl Pts',(-39.5809054933731,0.207174781350006,
12.8596900461973));
#55438=CARTESIAN_POINT('Ctrl Pts',(-38.592216719327,0.16130623594675,11.8636454473681));
#55439=CARTESIAN_POINT('Ctrl Pts',(-37.0897327714284,0.101038920786803,
10.0669225154591));
#55440=CARTESIAN_POINT('Ctrl Pts',(-36.0165024752287,0.0711941104908416,
7.9496729397282));
#55441=CARTESIAN_POINT('Ctrl Pts',(-34.9015558309501,0.0431888394733598,
4.6523117895337));
#55442=CARTESIAN_POINT('Ctrl Pts',(-34.6386449346511,0.0380442549261144,
2.62945113732801));
#55443=CARTESIAN_POINT('Ctrl Pts',(-34.8408722523068,0.042968270696446,
-0.463365540987003));
#55444=CARTESIAN_POINT('Ctrl Pts',(-35.029525914519,0.0477806632471993,
-1.54853574050673));
#55445=CARTESIAN_POINT('Ctrl Pts',(-35.3280864353835,0.0555127849838172,
-2.59511145651185));
#55446=CARTESIAN_POINT('Ctrl Pts',(-35.11517701784,0.0508510909662703,-2.65562493453964));
#55447=CARTESIAN_POINT('Ctrl Pts',(-35.3840062951942,0.0575422421921914,
-3.5976188055133));
#55448=CARTESIAN_POINT('Ctrl Pts',(-35.7436259783105,0.0666559496806185,
-4.521538758328));
#55449=CARTESIAN_POINT('Ctrl Pts',(-36.8151557983613,0.095692551513825,
-6.64222332188911));
#55450=CARTESIAN_POINT('Ctrl Pts',(-38.3559078896116,0.147573716864128,
-8.89963534126349));
#55451=CARTESIAN_POINT('Ctrl Pts',(-40.469472385245,0.204977053081564,-10.7437628031316));
#55452=CARTESIAN_POINT('Ctrl Pts',(-42.2712014812638,0.381060117365087,
-11.9612747311747));
#55453=CARTESIAN_POINT('Ctrl Pts',(-43.6118086922819,0.540518683561826,
-12.724156531761));
#55454=CARTESIAN_POINT('Ctrl Pts',(-46.4621628306032,1.23462273661855,-14.0012119190018));
#55455=CARTESIAN_POINT('Ctrl Pts',(-49.295584910841,2.34465836914774,-14.632672959566));
#55456=CARTESIAN_POINT('Ctrl Pts',(-52.5620566289039,3.10483667886162,-14.5433464527275));
#55457=CARTESIAN_POINT('Ctrl Pts',(-54.8001566067438,3.30035269345341,-14.0186136905654));
#55458=CARTESIAN_POINT('Ctrl Pts',(-56.9350672575427,3.39429553816601,-13.1429311762582));
#55459=CARTESIAN_POINT('Ctrl Pts',(-57.9716624173195,3.44148099145208,-12.5594172014826));
#55460=CARTESIAN_POINT('Ctrl Pts',(-58.9428583166749,3.53537179799872,-11.9255218957174));
#55461=CARTESIAN_POINT('Ctrl Pts',(-59.5517785065692,3.61039741065779,-11.5258146157856));
#55462=CARTESIAN_POINT('Ctrl Pts',(-60.6939165981419,3.73345458801685,-10.6556781858428));
#55463=CARTESIAN_POINT('Ctrl Pts',(-62.3504191551611,3.80834832178581,-9.12254403970273));
#55464=CARTESIAN_POINT('Ctrl Pts',(-63.5361674281905,3.32898348528657,-7.40198206074098));
#55465=CARTESIAN_POINT('Ctrl Pts',(-64.2149763686856,3.10273760294942,-6.03098199576973));
#55466=CARTESIAN_POINT('Ctrl Pts',(-64.6776127435176,2.97884271655914,-5.05337165230659));
#55467=CARTESIAN_POINT('Ctrl Pts',(-65.3270688519725,2.96185205497302,-3.39714199807037));
#55468=CARTESIAN_POINT('Ctrl Pts',(-65.7950910047088,3.14840094628669,-1.25128635775172));
#55469=CARTESIAN_POINT('Ctrl Pts',(-65.9145204535827,3.19168477671591,0.0517785197280895));
#55470=CARTESIAN_POINT('Ctrl Pts',(-65.9441051213068,3.18047187028911,0.622955634058679));
#55471=CARTESIAN_POINT('Ctrl Pts',(-65.9557016612563,3.17533523586427,0.88586519906267));
#55472=CARTESIAN_POINT('Ctrl Pts',(-65.9685107144033,3.16731893908496,1.40252832323383));
#55473=CARTESIAN_POINT('Ctrl Pts',(-65.9579083168253,3.15739901945015,2.37829097111894));
#55474=CARTESIAN_POINT('Ctrl Pts',(-65.8257155275689,3.15229864335318,4.16664556351419));
#55475=CARTESIAN_POINT('Ctrl Pts',(-65.5034203203996,3.12833741358611,5.65528760646102));
#55476=CARTESIAN_POINT('Ctrl Pts',(-64.9002921012009,3.04408997663893,7.4699894353198));
#55477=CARTESIAN_POINT('Ctrl Pts',(-63.9662479404238,2.90055300510061,9.65247467963668));
#55478=CARTESIAN_POINT('Ctrl Pts',(-62.5336778099795,2.68044822146662,11.5812656319969));
#55479=CARTESIAN_POINT('Ctrl Pts',(-59.4862509442383,2.27438763852615,14.691094912035));
#55480=CARTESIAN_POINT('Ctrl Pts',(-55.783918038216,1.71016553075871,16.7906541149307));
#55481=CARTESIAN_POINT('Ctrl Pts',(-47.9845453946372,0.754692999391247,
17.7848020910906));
#55482=CARTESIAN_POINT('Ctrl Pts',(-42.5252504170977,0.347888964974057,
15.8667796976236));
#55483=CARTESIAN_POINT('Ctrl Pts',(-39.4298897457784,0.19996339908082,13.0192697191585));
#55484=CARTESIAN_POINT('Ctrl Pts',(-38.4270467968691,0.154379143867951,
12.0091830811851));
#55485=CARTESIAN_POINT('Ctrl Pts',(-36.9028760126082,0.0948092812359606,
10.1871843261409));
#55486=CARTESIAN_POINT('Ctrl Pts',(-35.8138531895274,0.0658148084159087,
8.03995386779416));
#55487=CARTESIAN_POINT('Ctrl Pts',(-34.682418296982,0.0387556318332189,
4.69562286008841));
#55488=CARTESIAN_POINT('Ctrl Pts',(-34.4155737946825,0.0338633837576097,
2.64375559367379));
#55489=CARTESIAN_POINT('Ctrl Pts',(-34.6207976535155,0.038627270703424,
-0.493388346484037));
#55490=CARTESIAN_POINT('Ctrl Pts',(-34.8122294213517,0.043310735981189,
-1.59407843213931));
#55491=CARTESIAN_POINT('Ctrl Pts',(-35.11517701784,0.0508510909662663,-2.65562493453964));
#55492=CARTESIAN_POINT('',(-36.055003997507,1.05060622379088,-2.38157894671781));
#55493=CARTESIAN_POINT('Ctrl Pts',(-35.11517701784,0.0508510909662703,-2.65562493453964));
#55494=CARTESIAN_POINT('Ctrl Pts',(-35.3280864353835,0.0555127849838203,
-2.59511145651185));
#55495=CARTESIAN_POINT('Ctrl Pts',(-35.6788452868189,0.190821093669241,
-2.49451532637507));
#55496=CARTESIAN_POINT('Ctrl Pts',(-35.9918225445504,0.608287708528165,
-2.40265568865918));
#55497=CARTESIAN_POINT('Ctrl Pts',(-36.0552784362427,0.903015554155871,
-2.38254505299135));
#55498=CARTESIAN_POINT('Ctrl Pts',(-36.055003997507,1.05060622379088,-2.38157894671781));
#55499=CARTESIAN_POINT('',(-64.8720027515639,4.16096914635678,1.63199606547109));
#55500=CARTESIAN_POINT('Ctrl Pts',(-36.055003997507,1.05060622379089,-2.38157894671782));
#55501=CARTESIAN_POINT('Ctrl Pts',(-36.1322935555675,1.05266199109914,-2.65366126311645));
#55502=CARTESIAN_POINT('Ctrl Pts',(-36.2176393940941,1.05494437214152,-2.92418923910143));
#55503=CARTESIAN_POINT('Ctrl Pts',(-36.3109765306706,1.05747450348401,-3.19257913391778));
#55504=CARTESIAN_POINT('Ctrl Pts',(-36.4042248382911,1.06000222690042,-3.46071360206248));
#55505=CARTESIAN_POINT('Ctrl Pts',(-36.5054492155598,1.0627772292734,-3.72671372010584));
#55506=CARTESIAN_POINT('Ctrl Pts',(-36.6145331160612,1.0658205868793,-3.99000253341186));
#55507=CARTESIAN_POINT('Ctrl Pts',(-36.7235075599445,1.06886089072907,-4.2530271582997));
#55508=CARTESIAN_POINT('Ctrl Pts',(-36.8403257011726,1.07216901153767,-4.51334558411149));
#55509=CARTESIAN_POINT('Ctrl Pts',(-36.9648203194525,1.07576596220024,-4.7703927225219));
#55510=CARTESIAN_POINT('Ctrl Pts',(-36.9953298241032,1.07664745558915,-4.83338645649311));
#55511=CARTESIAN_POINT('Ctrl Pts',(-37.026300123263,1.07754629545318,-4.89618378526105));
#55512=CARTESIAN_POINT('Ctrl Pts',(-37.0577282953327,1.07846279106366,-4.95877651989893));
#55513=CARTESIAN_POINT('Ctrl Pts',(-37.191989322685,1.0823780567035,-5.22617243585101));
#55514=CARTESIAN_POINT('Ctrl Pts',(-37.3339878357898,1.0867584845706,-5.48861222280936));
#55515=CARTESIAN_POINT('Ctrl Pts',(-37.4834941556401,1.09151956863047,-5.74597365794833));
#55516=CARTESIAN_POINT('Ctrl Pts',(-37.6350344703111,1.0963454260078,-6.00683642886125));
#55517=CARTESIAN_POINT('Ctrl Pts',(-37.7942884884527,1.10156236749132,-6.26248241688958));
#55518=CARTESIAN_POINT('Ctrl Pts',(-37.9610686654377,1.10708239086208,-6.51277093542689));
#55519=CARTESIAN_POINT('Ctrl Pts',(-38.1283425215666,1.11261875382703,-6.76380032271606));
#55520=CARTESIAN_POINT('Ctrl Pts',(-38.3031875375309,1.11845999561527,-7.00944112260689));
#55521=CARTESIAN_POINT('Ctrl Pts',(-38.4854614009836,1.12451733021712,-7.24952794553518));
#55522=CARTESIAN_POINT('Ctrl Pts',(-38.6673538937057,1.13056199108684,-7.48911243595516));
#55523=CARTESIAN_POINT('Ctrl Pts',(-38.8566446481855,1.13682184145623,-7.72316674673868));
#55524=CARTESIAN_POINT('Ctrl Pts',(-39.0532324665159,1.14320865145002,-7.95149404526017));
#55525=CARTESIAN_POINT('Ctrl Pts',(-39.1059157316391,1.1449202427737,-8.01268312454808));
#55526=CARTESIAN_POINT('Ctrl Pts',(-39.1591232574712,1.1466409520596,-8.0734606948525));
#55527=CARTESIAN_POINT('Ctrl Pts',(-39.2128535191938,1.14836908120523,-8.13382248951383));
#55528=CARTESIAN_POINT('Ctrl Pts',(-39.377032041595,1.15364956338699,-8.31826436526975));
#55529=CARTESIAN_POINT('Ctrl Pts',(-39.5461034134596,1.15899932279134,-8.49883113714326));
#55530=CARTESIAN_POINT('Ctrl Pts',(-39.7197596703417,1.16498249252869,-8.67513434098695));
#55531=CARTESIAN_POINT('Ctrl Pts',(-39.9019313933737,1.17125905497346,-8.86008280755486));
#55532=CARTESIAN_POINT('Ctrl Pts',(-40.0891487598253,1.17823267106649,-9.04033867429534));
#55533=CARTESIAN_POINT('Ctrl Pts',(-40.2810101475514,1.18655459897303,-9.21549445643098));
#55534=CARTESIAN_POINT('Ctrl Pts',(-40.4638745846345,1.19448628694898,-9.38243666341536));
#55535=CARTESIAN_POINT('Ctrl Pts',(-40.6509571307088,1.20364279891409,-9.54474595128902));
#55536=CARTESIAN_POINT('Ctrl Pts',(-40.8418740647712,1.21458800384062,-9.70210900822495));
#55537=CARTESIAN_POINT('Ctrl Pts',(-41.0328375236401,1.22553587601896,-9.85951041317748));
#55538=CARTESIAN_POINT('Ctrl Pts',(-41.2276369488457,1.23827331304294,-10.011962966512));
#55539=CARTESIAN_POINT('Ctrl Pts',(-41.425857428129,1.25336459621525,-10.1591951341152));
#55540=CARTESIAN_POINT('Ctrl Pts',(-41.6242463092005,1.26846870045974,-10.3065523854654));
#55541=CARTESIAN_POINT('Ctrl Pts',(-41.8260617492356,1.2859306520565,-10.4486801988254));
#55542=CARTESIAN_POINT('Ctrl Pts',(-42.0308613301175,1.30631617171648,-10.5853513426465));
#55543=CARTESIAN_POINT('Ctrl Pts',(-42.0607832486186,1.30929456578956,-10.6053194637201));
#55544=CARTESIAN_POINT('Ctrl Pts',(-42.0907688260537,1.31233536695569,-10.625171186479));
#55545=CARTESIAN_POINT('Ctrl Pts',(-42.120816641723,1.31544033955858,-10.644905885882));
#55546=CARTESIAN_POINT('Ctrl Pts',(-42.3559034005757,1.33973288559832,-10.7993053460842));
#55547=CARTESIAN_POINT('Ctrl Pts',(-42.5950137384494,1.36687278436907,-10.9466772342795));
#55548=CARTESIAN_POINT('Ctrl Pts',(-42.8376128379884,1.39836730966744,-11.086802603462));
#55549=CARTESIAN_POINT('Ctrl Pts',(-43.0805446382786,1.42990502660273,-11.2271201407756));
#55550=CARTESIAN_POINT('Ctrl Pts',(-43.3269744463138,1.46580932213761,-11.3601711739332));
#55551=CARTESIAN_POINT('Ctrl Pts',(-43.5763500708487,1.50759367980925,-11.4857858807722));
#55552=CARTESIAN_POINT('Ctrl Pts',(-43.6977164532822,1.52792933347377,-11.5469201739812));
#55553=CARTESIAN_POINT('Ctrl Pts',(-43.819780379753,1.54965772931728,-11.6062938729776));
#55554=CARTESIAN_POINT('Ctrl Pts',(-43.9424772606944,1.57295333338661,-11.6638917675623));
#55555=CARTESIAN_POINT('Ctrl Pts',(-44.1747498761995,1.6170533206515,-11.7729280651448));
#55556=CARTESIAN_POINT('Ctrl Pts',(-44.4093065880691,1.66676967748696,-11.8756041239089));
#55557=CARTESIAN_POINT('Ctrl Pts',(-44.6456367997568,1.72160486396264,-11.9718184735828));
#55558=CARTESIAN_POINT('Ctrl Pts',(-44.8824535709107,1.77655294577602,-12.0682309105104));
#55559=CARTESIAN_POINT('Ctrl Pts',(-45.1210507987122,1.83664095634219,-12.1581549600952));
#55560=CARTESIAN_POINT('Ctrl Pts',(-45.3609076348146,1.9013682763762,-12.2415404290646));
#55561=CARTESIAN_POINT('Ctrl Pts',(-45.5273868230638,1.94629404072762,-12.2994163912901));
#55562=CARTESIAN_POINT('Ctrl Pts',(-45.6944726686526,1.99345476140644,-12.3541435226089));
#55563=CARTESIAN_POINT('Ctrl Pts',(-45.8619903777366,2.042683047791,-12.4057197872398));
#55564=CARTESIAN_POINT('Ctrl Pts',(-46.0944304045427,2.11099000034794,-12.4772846886398));
#55565=CARTESIAN_POINT('Ctrl Pts',(-46.3276914891466,2.18327765523928,-12.5427863991036));
#55566=CARTESIAN_POINT('Ctrl Pts',(-46.5617698195259,2.25813907221755,-12.6023525500692));
#55567=CARTESIAN_POINT('Ctrl Pts',(-46.7972329711181,2.33344337375536,-12.6622710978983));
#55568=CARTESIAN_POINT('Ctrl Pts',(-47.0335235344732,2.41135198051783,-12.7161838131883));
#55569=CARTESIAN_POINT('Ctrl Pts',(-47.2706600841618,2.49043283361392,-12.7641729127843));
#55570=CARTESIAN_POINT('Ctrl Pts',(-47.5087361286878,2.56982699165316,-12.8123521370631));
#55571=CARTESIAN_POINT('Ctrl Pts',(-47.7476653612993,2.65040270290849,-12.8545608454763));
#55572=CARTESIAN_POINT('Ctrl Pts',(-47.9874819513711,2.73071082024241,-12.890832108857));
#55573=CARTESIAN_POINT('Ctrl Pts',(-48.227129692856,2.81096239473197,-12.92707783459));
#55574=CARTESIAN_POINT('Ctrl Pts',(-48.4676640406405,2.89094675197924,-12.9573945421757));
#55575=CARTESIAN_POINT('Ctrl Pts',(-48.7091270187202,2.96921780361185,-12.9817638440304));
#55576=CARTESIAN_POINT('Ctrl Pts',(-48.9494154580997,3.04710812450067,-13.0060146072655));
#55577=CARTESIAN_POINT('Ctrl Pts',(-49.1906240098808,3.12330176716413,-13.0243756948092));
#55578=CARTESIAN_POINT('Ctrl Pts',(-49.4327945273407,3.19637364319789,-13.036777533859));
#55579=CARTESIAN_POINT('Ctrl Pts',(-49.5681239803724,3.23720758582381,-13.0437079154463));
#55580=CARTESIAN_POINT('Ctrl Pts',(-49.7037538009874,3.27706666778437,-13.0487764279543));
#55581=CARTESIAN_POINT('Ctrl Pts',(-49.8396904754171,3.31570220099547,-13.0519638705386));
#55582=CARTESIAN_POINT('Ctrl Pts',(-50.1782233791656,3.41191905565005,-13.0599017886765));
#55583=CARTESIAN_POINT('Ctrl Pts',(-50.518582222015,3.50054751812004,-13.056172132156));
#55584=CARTESIAN_POINT('Ctrl Pts',(-50.8602747909478,3.5807299233009,-13.0404229903288));
#55585=CARTESIAN_POINT('Ctrl Pts',(-51.1751659120314,3.65462303586533,-13.0259091689087));
#55586=CARTESIAN_POINT('Ctrl Pts',(-51.4911898131278,3.72134309963386,-13.0011868511954));
#55587=CARTESIAN_POINT('Ctrl Pts',(-51.8079187282795,3.78021885210975,-12.9659530059506));
#55588=CARTESIAN_POINT('Ctrl Pts',(-51.8348765969948,3.78522996644075,-12.9629541342689));
#55589=CARTESIAN_POINT('Ctrl Pts',(-51.8618395452152,3.79018425432501,-12.9598790993903));
#55590=CARTESIAN_POINT('Ctrl Pts',(-51.8888072932649,3.79508130187158,-12.9567277064462));
#55591=CARTESIAN_POINT('Ctrl Pts',(-52.099829761794,3.83340066987668,-12.9320680753509));
#55592=CARTESIAN_POINT('Ctrl Pts',(-52.3111643310852,3.86821518154434,-12.9027265467538));
#55593=CARTESIAN_POINT('Ctrl Pts',(-52.5223516668009,3.89997784147055,-12.8686708631832));
#55594=CARTESIAN_POINT('Ctrl Pts',(-52.7330469211624,3.93166649216386,-12.8346945317519));
#55595=CARTESIAN_POINT('Ctrl Pts',(-52.9435952878337,3.9603174966052,-12.7960259885999));
#55596=CARTESIAN_POINT('Ctrl Pts',(-53.15354205119,3.9863807001654,-12.7526850506438));
#55597=CARTESIAN_POINT('Ctrl Pts',(-53.3633141711024,4.01242222314546,-12.7093801656877));
#55598=CARTESIAN_POINT('Ctrl Pts',(-53.5724853493314,4.03588024875905,-12.6614106889577));
#55599=CARTESIAN_POINT('Ctrl Pts',(-53.780608504578,4.05720350070397,-12.6088479826448));
#55600=CARTESIAN_POINT('Ctrl Pts',(-53.9887349759261,4.07852709239997,-12.5562844388312));
#55601=CARTESIAN_POINT('Ctrl Pts',(-54.1958130568032,4.09771584239852,-12.4991275895464));
#55602=CARTESIAN_POINT('Ctrl Pts',(-54.4014072013379,4.11521849584678,-12.4374996534384));
#55603=CARTESIAN_POINT('Ctrl Pts',(-54.5862926290981,4.13095817353576,-12.3820792651044));
#55604=CARTESIAN_POINT('Ctrl Pts',(-54.7699779948038,4.14533431612562,-12.3230438550149));
#55605=CARTESIAN_POINT('Ctrl Pts',(-54.9521578365331,4.15867326758291,-12.2605165051515));
#55606=CARTESIAN_POINT('Ctrl Pts',(-55.1517001248123,4.17328347292599,-12.192030055974));
#55607=CARTESIAN_POINT('Ctrl Pts',(-55.3494514939048,4.1866493698181,-12.1193573255133));
#55608=CARTESIAN_POINT('Ctrl Pts',(-55.5455657376014,4.19972898490674,-12.0424636765534));
#55609=CARTESIAN_POINT('Ctrl Pts',(-55.6748708970455,4.20835284456439,-11.9917649340675));
#55610=CARTESIAN_POINT('Ctrl Pts',(-55.8034640727799,4.21685225070397,-11.9392302238067));
#55611=CARTESIAN_POINT('Ctrl Pts',(-55.9313849198071,4.22550180155907,-11.8848380394075));
#55612=CARTESIAN_POINT('Ctrl Pts',(-56.1506171346802,4.24032550102394,-11.7916200899119));
#55613=CARTESIAN_POINT('Ctrl Pts',(-56.3678647316653,4.25559019800313,-11.6929433272729));
#55614=CARTESIAN_POINT('Ctrl Pts',(-56.5826783791045,4.2721750813338,-11.5889779895733));
#55615=CARTESIAN_POINT('Ctrl Pts',(-56.7974907879464,4.28875986903743,-11.4850132513289));
#55616=CARTESIAN_POINT('Ctrl Pts',(-57.0098689485361,4.30666482786843,-11.3757601408548));
#55617=CARTESIAN_POINT('Ctrl Pts',(-57.2193847947822,4.32676913145603,-11.2614365003806));
#55618=CARTESIAN_POINT('Ctrl Pts',(-57.415690155682,4.34560580964584,-11.1543212443999));
#55619=CARTESIAN_POINT('Ctrl Pts',(-57.6094827608094,4.36637322822266,-11.0427552658619));
#55620=CARTESIAN_POINT('Ctrl Pts',(-57.8004311760719,4.38979452405874,-10.9269537836621));
#55621=CARTESIAN_POINT('Ctrl Pts',(-57.9483123118011,4.40793328590039,-10.8372706371259));
#55622=CARTESIAN_POINT('Ctrl Pts',(-58.0948414911701,4.42652998500644,-10.7448297287611));
#55623=CARTESIAN_POINT('Ctrl Pts',(-58.2396322283765,4.44497959030501,-10.6498619680056));
#55624=CARTESIAN_POINT('Ctrl Pts',(-58.3740970612243,4.4621134425144,-10.5616669334177));
#55625=CARTESIAN_POINT('Ctrl Pts',(-58.5070626671158,4.47912043310067,-10.4712931632196));
#55626=CARTESIAN_POINT('Ctrl Pts',(-58.6382418504244,4.49551596420629,-10.3789591096853));
#55627=CARTESIAN_POINT('Ctrl Pts',(-58.7793571620321,4.5131533699485,-10.2796312406754));
#55628=CARTESIAN_POINT('Ctrl Pts',(-58.918404907508,4.5300831784743,-10.1780449583785));
#55629=CARTESIAN_POINT('Ctrl Pts',(-59.0556314028655,4.54572602503811,-10.0740454574417));
#55630=CARTESIAN_POINT('Ctrl Pts',(-59.1833292612958,4.5602826746177,-9.97726740074885));
#55631=CARTESIAN_POINT('Ctrl Pts',(-59.3094499076329,4.57372488341918,-9.87839907259325));
#55632=CARTESIAN_POINT('Ctrl Pts',(-59.4341673742325,4.58558578894325,-9.77728339330231));
#55633=CARTESIAN_POINT('Ctrl Pts',(-59.5962054154582,4.60099596324107,-9.64590976091361));
#55634=CARTESIAN_POINT('Ctrl Pts',(-59.7558736542354,4.613736854791,-9.51073085320083));
#55635=CARTESIAN_POINT('Ctrl Pts',(-59.9127949926263,4.6227019676806,-9.37199436529526));
#55636=CARTESIAN_POINT('Ctrl Pts',(-60.0695888566196,4.63165979779797,-9.23337057939951));
#55637=CARTESIAN_POINT('Ctrl Pts',(-60.2236400109866,4.63684798123959,-9.09119519083188));
#55638=CARTESIAN_POINT('Ctrl Pts',(-60.374604228999,4.63716271647514,-8.94575635226619));
#55639=CARTESIAN_POINT('Ctrl Pts',(-60.5255583550716,4.63747743067068,-8.80032723626937));
#55640=CARTESIAN_POINT('Ctrl Pts',(-60.6734257119601,4.63291934821723,-8.65163533700792));
#55641=CARTESIAN_POINT('Ctrl Pts',(-60.8178979821347,4.62238488893667,-8.50000659817944));
#55642=CARTESIAN_POINT('Ctrl Pts',(-60.8461349302844,4.6203259403223,-8.47037092601109));
#55643=CARTESIAN_POINT('Ctrl Pts',(-60.8742423012993,4.61803869245437,-8.44062317532011));
#55644=CARTESIAN_POINT('Ctrl Pts',(-60.9022179651097,4.61551490577955,-8.41076593635432));
#55645=CARTESIAN_POINT('Ctrl Pts',(-61.1259061652568,4.59533517733165,-8.17203301152134));
#55646=CARTESIAN_POINT('Ctrl Pts',(-61.341181112213,4.56003280409024,-7.92628709053869));
#55647=CARTESIAN_POINT('Ctrl Pts',(-61.5476559471016,4.51576670901703,-7.67416287821696));
#55648=CARTESIAN_POINT('Ctrl Pts',(-61.7546563946079,4.47138792796869,-7.42139684594989));
#55649=CARTESIAN_POINT('Ctrl Pts',(-61.9528118061257,4.41799973000764,-7.1622202527666));
#55650=CARTESIAN_POINT('Ctrl Pts',(-62.1417816318185,4.3618081933155,-6.89729085245331));
#55651=CARTESIAN_POINT('Ctrl Pts',(-62.3315145775604,4.30538973738861,-6.63129158325373));
#55652=CARTESIAN_POINT('Ctrl Pts',(-62.5119875421368,4.24614525547315,-6.35949319617911));
#55653=CARTESIAN_POINT('Ctrl Pts',(-62.6829063613797,4.19035631611767,-6.0825760589589));
#55654=CARTESIAN_POINT('Ctrl Pts',(-62.7797254131915,4.158753990324,-5.92571296585504));
#55655=CARTESIAN_POINT('Ctrl Pts',(-62.8734796582814,4.12826047706972,-5.76720761562995));
#55656=CARTESIAN_POINT('Ctrl Pts',(-62.9641228638388,4.10001755239961,-5.60718528462863));
#55657=CARTESIAN_POINT('Ctrl Pts',(-63.0152047876007,4.08410126925475,-5.51700479661378));
#55658=CARTESIAN_POINT('Ctrl Pts',(-63.0653027666178,4.06889974586153,-5.42634434508404));
#55659=CARTESIAN_POINT('Ctrl Pts',(-63.114690027439,4.05526150059234,-5.33467778889543));
#55660=CARTESIAN_POINT('Ctrl Pts',(-63.1438918413464,4.04719744735773,-5.2804769753488));
#55661=CARTESIAN_POINT('Ctrl Pts',(-63.1728443241659,4.03967993925421,-5.22592394033852));
#55662=CARTESIAN_POINT('Ctrl Pts',(-63.2015963121648,4.0328843828772,-5.17090601533745));
#55663=CARTESIAN_POINT('Ctrl Pts',(-63.2894948262794,4.01210949565389,-5.00270916378545));
#55664=CARTESIAN_POINT('Ctrl Pts',(-63.3744719191724,3.99625727530115,-4.83215125581444));
#55665=CARTESIAN_POINT('Ctrl Pts',(-63.4562599252191,3.98469841004765,-4.65961827175044));
#55666=CARTESIAN_POINT('Ctrl Pts',(-63.5366571757962,3.97333609629173,-4.49001910650485));
#55667=CARTESIAN_POINT('Ctrl Pts',(-63.6139728247038,3.96612236725379,-4.31851180304446));
#55668=CARTESIAN_POINT('Ctrl Pts',(-63.6879982711723,3.962459471557,-4.14548861462962));
#55669=CARTESIAN_POINT('Ctrl Pts',(-63.7639445164335,3.9587015317103,-3.96797585205806));
#55670=CARTESIAN_POINT('Ctrl Pts',(-63.8364272308132,3.95868108869533,-3.78886772818592));
#55671=CARTESIAN_POINT('Ctrl Pts',(-63.9052732336969,3.96175264228226,-3.60861111381425));
#55672=CARTESIAN_POINT('Ctrl Pts',(-63.9741192365805,3.9648241958692,-3.42835449944258));
#55673=CARTESIAN_POINT('Ctrl Pts',(-64.0393284286319,3.97098774605804,-3.24694973670777));
#55674=CARTESIAN_POINT('Ctrl Pts',(-64.1007822541809,3.97959779261897,-3.06486232390459));
#55675=CARTESIAN_POINT('Ctrl Pts',(-64.1702270221536,3.98932741775323,-2.85909778410764));
#55676=CARTESIAN_POINT('Ctrl Pts',(-64.2348845570762,4.00218114911087,-2.652469780862));
#55677=CARTESIAN_POINT('Ctrl Pts',(-64.2948630613201,4.01668597766837,-2.44487228947275));
#55678=CARTESIAN_POINT('Ctrl Pts',(-64.3549604873855,4.03121956553977,-2.23686318608836));
#55679=CARTESIAN_POINT('Ctrl Pts',(-64.4103604314521,4.04741080449716,-2.02788033843582));
#55680=CARTESIAN_POINT('Ctrl Pts',(-64.4611227734419,4.06377790634833,-1.81779844513638));
#55681=CARTESIAN_POINT('Ctrl Pts',(-64.5118609248486,4.08013720852512,-1.60781666549011));
#55682=CARTESIAN_POINT('Ctrl Pts',(-64.5579659879566,4.09667220602219,-1.39673647437591));
#55683=CARTESIAN_POINT('Ctrl Pts',(-64.5994472931465,4.11190322805798,-1.18442030572762));
#55684=CARTESIAN_POINT('Ctrl Pts',(-64.6204216122818,4.11960453628521,-1.07706623240652));
#55685=CARTESIAN_POINT('Ctrl Pts',(-64.6402129899606,4.12697246390265,-0.969396004279037));
#55686=CARTESIAN_POINT('Ctrl Pts',(-64.6588176023091,4.13381573006831,-0.861391140572027));
#55687=CARTESIAN_POINT('Ctrl Pts',(-64.6983751695293,4.14836604459698,-0.631748642454824));
#55688=CARTESIAN_POINT('Ctrl Pts',(-64.732559846353,4.16054445540993,-0.400605174382738));
#55689=CARTESIAN_POINT('Ctrl Pts',(-64.7612370512181,4.16849178751679,-0.168417716141251));
#55690=CARTESIAN_POINT('Ctrl Pts',(-64.7898878583897,4.17643180401403,0.063556010903203));
#55691=CARTESIAN_POINT('Ctrl Pts',(-64.8130412472295,4.18014852773221,0.296571463029256));
#55692=CARTESIAN_POINT('Ctrl Pts',(-64.8306138183485,4.17778791313152,0.530161692369568));
#55693=CARTESIAN_POINT('Ctrl Pts',(-64.8336767293851,4.17737645640931,0.570876627402885));
#55694=CARTESIAN_POINT('Ctrl Pts',(-64.8365702175283,4.17678036573755,0.611609004456205));
#55695=CARTESIAN_POINT('Ctrl Pts',(-64.839294001694,4.17598982323856,0.652356328090951));
#55696=CARTESIAN_POINT('Ctrl Pts',(-64.8432954133527,4.17482846617806,0.712216730359264));
#55697=CARTESIAN_POINT('Ctrl Pts',(-64.8469308150517,4.17368838965138,0.772114743988323));
#55698=CARTESIAN_POINT('Ctrl Pts',(-64.8501981550959,4.1726021357397,0.832015202980184));
#55699=CARTESIAN_POINT('Ctrl Pts',(-64.8600001752284,4.16934337400467,1.01171657995577));
#55700=CARTESIAN_POINT('Ctrl Pts',(-64.8664934873315,4.16656901580476,1.19143948170663));
#55701=CARTESIAN_POINT('Ctrl Pts',(-64.8696864375022,4.1641759703485,1.37131271729487));
#55702=CARTESIAN_POINT('Ctrl Pts',(-64.8712285716237,4.16302017496955,1.45818806433278));
#55703=CARTESIAN_POINT('Ctrl Pts',(-64.8719999767219,4.16195332864408,1.54509863601051));
#55704=CARTESIAN_POINT('Ctrl Pts',(-64.8719999999995,4.16096914635678,1.63199606547182));
#55705=CARTESIAN_POINT('Ctrl Pts',(-64.8720055031283,4.16096914635646,1.63199606549839));
#55706=CARTESIAN_POINT('Ctrl Pts',(-64.8719930365275,4.15923636219392,1.78499063561214));
#55707=CARTESIAN_POINT('Ctrl Pts',(-64.8620592180002,4.15312946060718,2.41759877960346));
#55708=CARTESIAN_POINT('Ctrl Pts',(-64.7352335229478,4.14731569311366,3.99634452035672));
#55709=CARTESIAN_POINT('Ctrl Pts',(-64.4136487318254,4.12105688799969,5.39708413320686));
#55710=CARTESIAN_POINT('Ctrl Pts',(-63.8397399723428,4.03549450524408,7.10448416695828));
#55711=CARTESIAN_POINT('Ctrl Pts',(-62.9522997363556,3.89000867503392,9.15140293674327));
#55712=CARTESIAN_POINT('Ctrl Pts',(-61.6208708298335,3.67142317516158,10.9503238549484));
#55713=CARTESIAN_POINT('Ctrl Pts',(-58.7634589988956,3.26466779407872,13.8578351195001));
#55714=CARTESIAN_POINT('Ctrl Pts',(-55.2912534175913,2.6998098225271,15.8249286900159));
#55715=CARTESIAN_POINT('Ctrl Pts',(-48.0385774976576,1.75094933219347,16.7544728922648));
#55716=CARTESIAN_POINT('Ctrl Pts',(-42.9496055667091,1.34558036473629,14.9600338121896));
#55717=CARTESIAN_POINT('Ctrl Pts',(-40.071051319765,1.19886194165591,12.29337200187));
#55718=CARTESIAN_POINT('Ctrl Pts',(-39.1375314597392,1.15352274909741,11.3477862008985));
#55719=CARTESIAN_POINT('Ctrl Pts',(-37.7188484542204,1.09430323930076,9.64179625830726));
#55720=CARTESIAN_POINT('Ctrl Pts',(-36.7050175851536,1.06546586823309,7.63138184708971));
#55721=CARTESIAN_POINT('Ctrl Pts',(-35.6516869686853,1.03855926629819,4.50020178467594));
#55722=CARTESIAN_POINT('Ctrl Pts',(-35.4031623106733,1.03368706569832,2.57903751737137));
#55723=CARTESIAN_POINT('Ctrl Pts',(-35.594321537606,1.03843169037817,-0.357311618779464));
#55724=CARTESIAN_POINT('Ctrl Pts',(-35.7726576378221,1.04309630355831,-1.3876354762478));
#55725=CARTESIAN_POINT('Ctrl Pts',(-36.055003997507,1.05060622379088,-2.38157894671782));
#55726=CARTESIAN_POINT('Origin',(-50.184,-32.64,1.632));
#55727=CARTESIAN_POINT('',(-64.8718846268333,6.25079236928354,1.6329527449831));
#55728=CARTESIAN_POINT('',(-64.872,-32.64,1.632));
#55729=CARTESIAN_POINT('',(-36.065644266864,3.13140677366842,-2.41884872497431));
#55730=CARTESIAN_POINT('Ctrl Pts',(-36.065644266864,3.13140677366842,-2.41884872497431));
#55731=CARTESIAN_POINT('Ctrl Pts',(-35.7780846374424,3.12368828933858,-1.4166219279989));
#55732=CARTESIAN_POINT('Ctrl Pts',(-35.5953745209546,3.11887456876326,-0.372879642437447));
#55733=CARTESIAN_POINT('Ctrl Pts',(-35.4027861848181,3.11402573771371,2.58487032700104));
#55734=CARTESIAN_POINT('Ctrl Pts',(-35.6521037255763,3.11894001012135,4.4959742368839));
#55735=CARTESIAN_POINT('Ctrl Pts',(-36.9698692287106,3.1530828253069,8.42617802922758));
#55736=CARTESIAN_POINT('Ctrl Pts',(-38.1616212543277,3.1879695783913,10.3549179060355));
#55737=CARTESIAN_POINT('Ctrl Pts',(-42.4613671667828,3.39627919561991,14.7446124362785));
#55738=CARTESIAN_POINT('Ctrl Pts',(-50.2262334512378,3.97083149861718,17.9144169067269));
#55739=CARTESIAN_POINT('Ctrl Pts',(-57.9134779272454,5.23514997311662,14.7265287262636));
#55740=CARTESIAN_POINT('Ctrl Pts',(-62.2002402570179,5.85744949443928,10.3661404754207));
#55741=CARTESIAN_POINT('Ctrl Pts',(-63.3943845893009,6.06869311513403,8.42892326864068));
#55742=CARTESIAN_POINT('Ctrl Pts',(-64.6118270133895,6.24609538226257,4.81359831624348));
#55743=CARTESIAN_POINT('Ctrl Pts',(-64.8712207656872,6.23100612702719,3.22312584190541));
#55744=CARTESIAN_POINT('Ctrl Pts',(-64.8718846268333,6.25079236928354,1.6329527449831));
#55745=CARTESIAN_POINT('Ctrl Pts',(-64.8718846268333,6.25079236928354,1.6329527449831));
#55746=CARTESIAN_POINT('Ctrl Pts',(-64.8720137299782,6.25464026144678,1.32370682963648));
#55747=CARTESIAN_POINT('Ctrl Pts',(-64.8623577223499,6.2598071376853,1.01447223668158));
#55748=CARTESIAN_POINT('Ctrl Pts',(-64.8279255683366,6.27285046627563,0.470282225806653));
#55749=CARTESIAN_POINT('Ctrl Pts',(-64.7869366759734,6.27297083982397,0.00182753649455431));
#55750=CARTESIAN_POINT('Ctrl Pts',(-64.6604441900832,6.24060155475075,-0.928432328896818));
#55751=CARTESIAN_POINT('Ctrl Pts',(-64.3201724720767,6.12732012565137,-2.54924414126407));
#55752=CARTESIAN_POINT('Ctrl Pts',(-63.8282831273652,6.05945295552752,-3.88543452904561));
#55753=CARTESIAN_POINT('Ctrl Pts',(-62.9004728688998,6.33137887468648,-5.81565625714699));
#55754=CARTESIAN_POINT('Ctrl Pts',(-61.6122544655027,7.13811360863407,-7.83110990015508));
#55755=CARTESIAN_POINT('Ctrl Pts',(-59.8048511793193,7.01369953657289,-9.53478552281347));
#55756=CARTESIAN_POINT('Ctrl Pts',(-58.6631333960574,6.8704405564795,-10.363121955978));
#55757=CARTESIAN_POINT('Ctrl Pts',(-58.3493696503069,6.83776391263835,-10.5817734230167));
#55758=CARTESIAN_POINT('Ctrl Pts',(-57.7047601394273,6.7930417097451,-10.9951030826806));
#55759=CARTESIAN_POINT('Ctrl Pts',(-56.5377248070284,6.7584186916988,-11.6470045461552));
#55760=CARTESIAN_POINT('Ctrl Pts',(-54.0569552148524,6.75345765423783,-12.6904602333806));
#55761=CARTESIAN_POINT('Ctrl Pts',(-50.2178417525627,6.25049709636969,-13.2722316651482));
#55762=CARTESIAN_POINT('Ctrl Pts',(-46.7178274773985,4.51449035845978,-12.7648792404124));
#55763=CARTESIAN_POINT('Ctrl Pts',(-43.9411365965136,3.61830280145254,-11.7305732722043));
#55764=CARTESIAN_POINT('Ctrl Pts',(-42.5911117010961,3.45233648724814,-10.9642662180381));
#55765=CARTESIAN_POINT('Ctrl Pts',(-41.4467701567403,3.33147776885485,-10.1910309575598));
#55766=CARTESIAN_POINT('Ctrl Pts',(-40.4532021950847,3.27050850699576,-9.42430687806686));
#55767=CARTESIAN_POINT('Ctrl Pts',(-38.6732274933371,3.21130715662269,-7.64161528907957));
#55768=CARTESIAN_POINT('Ctrl Pts',(-37.6213539969012,3.17638521197561,-6.08089500182063));
#55769=CARTESIAN_POINT('Ctrl Pts',(-36.6477529660739,3.14707541849258,-4.14218022621547));
#55770=CARTESIAN_POINT('Ctrl Pts',(-36.3151556718838,3.13810399286304,-3.28846667783078));
#55771=CARTESIAN_POINT('Ctrl Pts',(-36.065644266864,3.13140677366842,-2.41884872497431));
#55772=CARTESIAN_POINT('Ctrl Pts',(-36.065644266864,3.13140677366842,-2.41884872497431));
#55773=CARTESIAN_POINT('Ctrl Pts',(-35.7780846374424,3.12368828933858,-1.4166219279989));
#55774=CARTESIAN_POINT('Ctrl Pts',(-35.5953745209546,3.11887456876326,-0.372879642437447));
#55775=CARTESIAN_POINT('Ctrl Pts',(-35.4027861848181,3.11402573771371,2.58487032700104));
#55776=CARTESIAN_POINT('Ctrl Pts',(-35.6521037255763,3.11894001012135,4.4959742368839));
#55777=CARTESIAN_POINT('Ctrl Pts',(-36.9698692287106,3.1530828253069,8.42617802922758));
#55778=CARTESIAN_POINT('Ctrl Pts',(-38.1616212543277,3.1879695783913,10.3549179060355));
#55779=CARTESIAN_POINT('Ctrl Pts',(-42.4613671667828,3.39627919561991,14.7446124362785));
#55780=CARTESIAN_POINT('Ctrl Pts',(-50.2262334512378,3.97083149861718,17.9144169067269));
#55781=CARTESIAN_POINT('Ctrl Pts',(-57.9134779272454,5.23514997311662,14.7265287262636));
#55782=CARTESIAN_POINT('Ctrl Pts',(-62.2002402570179,5.85744949443928,10.3661404754207));
#55783=CARTESIAN_POINT('Ctrl Pts',(-63.3943845893009,6.06869311513403,8.42892326864068));
#55784=CARTESIAN_POINT('Ctrl Pts',(-64.7103648856598,6.26045404234611,4.52097960892216));
#55785=CARTESIAN_POINT('Ctrl Pts',(-64.9627582385739,6.22177417224124,2.60127270216699));
#55786=CARTESIAN_POINT('Ctrl Pts',(-64.8279255683366,6.27285046627563,0.470282225806653));
#55787=CARTESIAN_POINT('Ctrl Pts',(-64.7869366759734,6.27297083982397,0.00182753649455431));
#55788=CARTESIAN_POINT('Ctrl Pts',(-64.6604441900832,6.24060155475075,-0.928432328896818));
#55789=CARTESIAN_POINT('Ctrl Pts',(-64.3201724720767,6.12732012565137,-2.54924414126407));
#55790=CARTESIAN_POINT('Ctrl Pts',(-63.8282831273652,6.05945295552752,-3.88543452904561));
#55791=CARTESIAN_POINT('Ctrl Pts',(-62.9004728688998,6.33137887468648,-5.81565625714699));
#55792=CARTESIAN_POINT('Ctrl Pts',(-61.6122544655027,7.13811360863407,-7.83110990015508));
#55793=CARTESIAN_POINT('Ctrl Pts',(-59.8048511793193,7.01369953657289,-9.53478552281347));
#55794=CARTESIAN_POINT('Ctrl Pts',(-58.6631333960574,6.8704405564795,-10.363121955978));
#55795=CARTESIAN_POINT('Ctrl Pts',(-58.3493696503069,6.83776391263835,-10.5817734230167));
#55796=CARTESIAN_POINT('Ctrl Pts',(-57.7047601394273,6.7930417097451,-10.9951030826806));
#55797=CARTESIAN_POINT('Ctrl Pts',(-56.5377248070284,6.7584186916988,-11.6470045461552));
#55798=CARTESIAN_POINT('Ctrl Pts',(-54.0569552148524,6.75345765423783,-12.6904602333806));
#55799=CARTESIAN_POINT('Ctrl Pts',(-50.2178417525627,6.25049709636969,-13.2722316651482));
#55800=CARTESIAN_POINT('Ctrl Pts',(-46.7178274773985,4.51449035845978,-12.7648792404124));
#55801=CARTESIAN_POINT('Ctrl Pts',(-43.9411365965136,3.61830280145254,-11.7305732722043));
#55802=CARTESIAN_POINT('Ctrl Pts',(-42.5911117010961,3.45233648724814,-10.9642662180381));
#55803=CARTESIAN_POINT('Ctrl Pts',(-41.4467701567403,3.33147776885485,-10.1910309575598));
#55804=CARTESIAN_POINT('Ctrl Pts',(-40.4532021950847,3.27050850699576,-9.42430687806686));
#55805=CARTESIAN_POINT('Ctrl Pts',(-38.6732274933371,3.21130715662269,-7.64161528907957));
#55806=CARTESIAN_POINT('Ctrl Pts',(-37.6213539969012,3.17638521197561,-6.08089500182063));
#55807=CARTESIAN_POINT('Ctrl Pts',(-36.6477529660739,3.14707541849258,-4.14218022621547));
#55808=CARTESIAN_POINT('Ctrl Pts',(-36.3151556718838,3.13810399286304,-3.28846667783078));
#55809=CARTESIAN_POINT('Ctrl Pts',(-36.065644266864,3.13140677366842,-2.41884872497431));
#55810=CARTESIAN_POINT('Ctrl Pts',(-36.0650646070859,3.4346612700204,-2.41682844638411));
#55811=CARTESIAN_POINT('Ctrl Pts',(-35.7778621348589,3.42677312832869,-1.41532929226861));
#55812=CARTESIAN_POINT('Ctrl Pts',(-35.5953276311515,3.42184355033732,-0.371937396594396));
#55813=CARTESIAN_POINT('Ctrl Pts',(-35.4029663176075,3.41686295257622,2.58412733083116));
#55814=CARTESIAN_POINT('Ctrl Pts',(-35.6520686551882,3.42197511366452,4.49482638811762));
#55815=CARTESIAN_POINT('Ctrl Pts',(-36.968521585772,3.4572178918651,8.42244597254387));
#55816=CARTESIAN_POINT('Ctrl Pts',(-38.1580037490657,3.49281635955522,10.3496423448272));
#55817=CARTESIAN_POINT('Ctrl Pts',(-42.4498664685835,3.70275922439794,14.7330424895737));
#55818=CARTESIAN_POINT('Ctrl Pts',(-50.1810892659201,4.27080024554784,17.9103274086348));
#55819=CARTESIAN_POINT('Ctrl Pts',(-57.8815423520458,5.51753858629548,14.7469836103004));
#55820=CARTESIAN_POINT('Ctrl Pts',(-62.1866799556937,6.13507517348564,10.3858739129262));
#55821=CARTESIAN_POINT('Ctrl Pts',(-63.3857030057778,6.34398363305886,8.44800531621039));
#55822=CARTESIAN_POINT('Ctrl Pts',(-64.7107997545463,6.53780208228581,4.52413466314126));
#55823=CARTESIAN_POINT('Ctrl Pts',(-64.9616943271868,6.50914304046526,2.5989830365699));
#55824=CARTESIAN_POINT('Ctrl Pts',(-64.8281749317427,6.55133949313081,0.475090785410251));
#55825=CARTESIAN_POINT('Ctrl Pts',(-64.7863724086547,6.54981290757855,-0.00354337177167986));
#55826=CARTESIAN_POINT('Ctrl Pts',(-64.6582750072647,6.51215776525242,-0.94161213829145));
#55827=CARTESIAN_POINT('Ctrl Pts',(-64.3145441725083,6.38690347009193,-2.568589975368));
#55828=CARTESIAN_POINT('Ctrl Pts',(-63.8287571100992,6.3086096976912,-3.88066143217033));
#55829=CARTESIAN_POINT('Ctrl Pts',(-62.9289673976073,6.54418319192483,-5.76366911909594));
#55830=CARTESIAN_POINT('Ctrl Pts',(-61.6371827042111,7.32609606241457,-7.81260292844509));
#55831=CARTESIAN_POINT('Ctrl Pts',(-59.7926587181835,7.21283514873646,-9.54588742378878));
#55832=CARTESIAN_POINT('Ctrl Pts',(-58.6482498454689,7.07001126275249,-10.3736593014408));
#55833=CARTESIAN_POINT('Ctrl Pts',(-58.3385085297827,7.03254425950593,-10.5890602215478));
#55834=CARTESIAN_POINT('Ctrl Pts',(-57.6985348409166,6.98190728715686,-10.998859774944));
#55835=CARTESIAN_POINT('Ctrl Pts',(-56.5373250194885,6.93691002365351,-11.6473031199624));
#55836=CARTESIAN_POINT('Ctrl Pts',(-54.0509279624105,6.92531201937256,-12.6932902933945));
#55837=CARTESIAN_POINT('Ctrl Pts',(-50.1679811065434,6.42171268884258,-13.2814410926045));
#55838=CARTESIAN_POINT('Ctrl Pts',(-46.6184476459557,4.72761566928903,-12.740305567001));
#55839=CARTESIAN_POINT('Ctrl Pts',(-43.8944244000067,3.90614836057661,-11.7049493454516));
#55840=CARTESIAN_POINT('Ctrl Pts',(-42.5674858734948,3.74857859214072,-10.9494179972056));
#55841=CARTESIAN_POINT('Ctrl Pts',(-41.4315976471264,3.62970738952218,-10.1792648565723));
#55842=CARTESIAN_POINT('Ctrl Pts',(-40.4473443265289,3.57455025905753,-9.41841100374971));
#55843=CARTESIAN_POINT('Ctrl Pts',(-38.6696727269255,3.51502557823487,-7.63715913873979));
#55844=CARTESIAN_POINT('Ctrl Pts',(-37.6188008298502,3.48053370900519,-6.076262128612));
#55845=CARTESIAN_POINT('Ctrl Pts',(-36.6466007134482,3.45067784482792,-4.13925470645933));
#55846=CARTESIAN_POINT('Ctrl Pts',(-36.3142661118821,3.44150569849757,-3.28581503386884));
#55847=CARTESIAN_POINT('Ctrl Pts',(-36.0650646070859,3.4346612700204,-2.41682844638411));
#55848=CARTESIAN_POINT('Ctrl Pts',(-35.8155534753675,3.95922815415782,-2.48463600652939));
#55849=CARTESIAN_POINT('Ctrl Pts',(-35.5240223169276,3.95107190238858,-1.46597111396737));
#55850=CARTESIAN_POINT('Ctrl Pts',(-35.3388157069111,3.94595107338873,-0.40527320525134));
#55851=CARTESIAN_POINT('Ctrl Pts',(-35.1436102274987,3.94076100294377,2.60032378867928));
#55852=CARTESIAN_POINT('Ctrl Pts',(-35.3963491893894,3.94620086831573,4.54302230566112));
#55853=CARTESIAN_POINT('Ctrl Pts',(-36.731867402577,3.98322862837942,8.53671442736042));
#55854=CARTESIAN_POINT('Ctrl Pts',(-37.9377019443431,4.01999998102908,10.495940394407));
#55855=CARTESIAN_POINT('Ctrl Pts',(-42.2899491029564,4.2324854098098,14.9509728434312));
#55856=CARTESIAN_POINT('Ctrl Pts',(-50.1129881046017,4.78982733568662,18.1867023470396));
#55857=CARTESIAN_POINT('Ctrl Pts',(-57.9483290593166,6.00736287403418,14.9823983499893));
#55858=CARTESIAN_POINT('Ctrl Pts',(-62.3399356821522,6.61691276101214,10.5486133037616));
#55859=CARTESIAN_POINT('Ctrl Pts',(-63.5613060337253,6.82198967979261,8.57896237194291));
#55860=CARTESIAN_POINT('Ctrl Pts',(-64.9230450981126,7.0192762223136,4.5726621091647));
#55861=CARTESIAN_POINT('Ctrl Pts',(-65.192622059577,7.00684276405108,2.60965408956806));
#55862=CARTESIAN_POINT('Ctrl Pts',(-65.0446288523742,7.03437779670717,0.466431163727447));
#55863=CARTESIAN_POINT('Ctrl Pts',(-64.9980055512648,7.03014036934465,-0.0365399369319378));
#55864=CARTESIAN_POINT('Ctrl Pts',(-64.8571340870366,6.98374035596922,-1.00071940981554));
#55865=CARTESIAN_POINT('Ctrl Pts',(-64.4848024323001,6.83851971166886,-2.65718050680847));
#55866=CARTESIAN_POINT('Ctrl Pts',(-63.9862452561701,6.74259812652883,-3.93751639334648));
#55867=CARTESIAN_POINT('Ctrl Pts',(-63.0899327077538,6.91582060101885,-5.74134045894053));
#55868=CARTESIAN_POINT('Ctrl Pts',(-61.7532719631801,7.65468816352199,-7.84153086863482));
#55869=CARTESIAN_POINT('Ctrl Pts',(-59.8421629477594,7.56060613887443,-9.64672021837555));
#55870=CARTESIAN_POINT('Ctrl Pts',(-58.6851925837328,7.41843354268482,-10.4808914644111));
#55871=CARTESIAN_POINT('Ctrl Pts',(-58.3767589854455,7.37274010456707,-10.687376889481));
#55872=CARTESIAN_POINT('Ctrl Pts',(-57.7367797264508,7.31190480666232,-11.0881951675255));
#55873=CARTESIAN_POINT('Ctrl Pts',(-56.5732669821134,7.24895695789893,-11.7252028912417));
#55874=CARTESIAN_POINT('Ctrl Pts',(-54.0603724547201,7.22580025282231,-12.7753953588624));
#55875=CARTESIAN_POINT('Ctrl Pts',(-50.0841495080587,6.72117303445737,-13.3797286087254));
#55876=CARTESIAN_POINT('Ctrl Pts',(-46.4191811247196,5.10039243267267,-12.8412071463471));
#55877=CARTESIAN_POINT('Ctrl Pts',(-43.7167587333486,4.40484600132639,-11.8767330810714));
#55878=CARTESIAN_POINT('Ctrl Pts',(-42.3981754693853,4.26102412055946,-11.1378753168652));
#55879=CARTESIAN_POINT('Ctrl Pts',(-41.2564486598985,4.14573262965561,-10.3613182181735));
#55880=CARTESIAN_POINT('Ctrl Pts',(-40.2650697587731,4.10017673244414,-9.60492248587169));
#55881=CARTESIAN_POINT('Ctrl Pts',(-38.4589390717363,4.04017090207336,-7.79283393642232));
#55882=CARTESIAN_POINT('Ctrl Pts',(-37.3917532046939,4.00650035743647,-6.20548621434273));
#55883=CARTESIAN_POINT('Ctrl Pts',(-36.4057350142359,3.97579715932729,-4.23644501702129));
#55884=CARTESIAN_POINT('Ctrl Pts',(-36.068510919692,3.96630521794014,-3.36851706138635));
#55885=CARTESIAN_POINT('Ctrl Pts',(-35.8155534753675,3.95922815415782,-2.48463600652939));
#55886=CARTESIAN_POINT('Ctrl Pts',(-35.300583251693,4.13600582362742,-2.63111698861473));
#55887=CARTESIAN_POINT('Ctrl Pts',(-34.9991934800771,4.12811190259441,-1.57610435146056));
#55888=CARTESIAN_POINT('Ctrl Pts',(-34.8077644827284,4.12317489235507,-0.477647028350931));
#55889=CARTESIAN_POINT('Ctrl Pts',(-34.6060333124814,4.11818868004728,2.6346991492121));
#55890=CARTESIAN_POINT('Ctrl Pts',(-34.8671273680138,4.12331427351438,4.64644201761164));
#55891=CARTESIAN_POINT('Ctrl Pts',(-36.2471277637543,4.1586388019116,8.78323323890242));
#55892=CARTESIAN_POINT('Ctrl Pts',(-37.4935827303532,4.19414050837293,10.81320828298));
#55893=CARTESIAN_POINT('Ctrl Pts',(-41.9963149144722,4.40389550232149,15.4313894678807));
#55894=CARTESIAN_POINT('Ctrl Pts',(-50.1022225688271,4.9674647626258,18.7736207894476));
#55895=CARTESIAN_POINT('Ctrl Pts',(-58.1850741698473,6.2085491891343,15.4255183205296));
#55896=CARTESIAN_POINT('Ctrl Pts',(-62.712974569855,6.82560512914881,10.841656335752));
#55897=CARTESIAN_POINT('Ctrl Pts',(-63.969610611664,7.03376995866941,8.80641509887463));
#55898=CARTESIAN_POINT('Ctrl Pts',(-65.3827943906313,7.23025660308972,4.66801890208108));
#55899=CARTESIAN_POINT('Ctrl Pts',(-65.6866084443025,7.20685314020845,2.63859554445347));
#55900=CARTESIAN_POINT('Ctrl Pts',(-65.5116379537911,7.24390206311906,0.433244296697788));
#55901=CARTESIAN_POINT('Ctrl Pts',(-65.4585912453259,7.24146200832042,-0.0918947338236302));
#55902=CARTESIAN_POINT('Ctrl Pts',(-65.2992289363671,7.19990543690473,-1.08988473989177));
#55903=CARTESIAN_POINT('Ctrl Pts',(-64.8836246369305,7.06430956710991,-2.79529312832537));
#55904=CARTESIAN_POINT('Ctrl Pts',(-64.3446567263413,6.97888693816536,-4.0813056792627));
#55905=CARTESIAN_POINT('Ctrl Pts',(-63.3883510078546,7.15506110909943,-5.84612212194586));
#55906=CARTESIAN_POINT('Ctrl Pts',(-61.9668081348504,7.89578816450023,-7.96758783776226));
#55907=CARTESIAN_POINT('Ctrl Pts',(-59.999382965377,7.80389026779883,-9.85943516852207));
#55908=CARTESIAN_POINT('Ctrl Pts',(-58.8198661566153,7.6612085250852,-10.7098022926259));
#55909=CARTESIAN_POINT('Ctrl Pts',(-58.5032990808582,7.6148790028951,-10.9062394845128));
#55910=CARTESIAN_POINT('Ctrl Pts',(-57.8503744210902,7.5524633917664,-11.2975303524532));
#55911=CARTESIAN_POINT('Ctrl Pts',(-56.664326473605,7.48518113024164,-11.9193059799705));
#55912=CARTESIAN_POINT('Ctrl Pts',(-54.1048100395427,7.45888940763357,-12.9741605614099));
#55913=CARTESIAN_POINT('Ctrl Pts',(-50.018244533416,6.94967066206464,-13.5982483167349));
#55914=CARTESIAN_POINT('Ctrl Pts',(-46.2497967424538,5.33227973346929,-13.1575362520759));
#55915=CARTESIAN_POINT('Ctrl Pts',(-43.4813240908299,4.60340874785693,-12.3181482587086));
#55916=CARTESIAN_POINT('Ctrl Pts',(-42.1142395829665,4.4453022212816,-11.574327561683));
#55917=CARTESIAN_POINT('Ctrl Pts',(-40.9360947918748,4.32903411911999,-10.7753888548978));
#55918=CARTESIAN_POINT('Ctrl Pts',(-39.9057722307278,4.27570940455937,-10.0065317563462));
#55919=CARTESIAN_POINT('Ctrl Pts',(-38.0354999795452,4.21604903461122,-8.12865768725083));
#55920=CARTESIAN_POINT('Ctrl Pts',(-36.9302316463433,4.18186405058577,-6.48531537837426));
#55921=CARTESIAN_POINT('Ctrl Pts',(-35.9107301048361,4.15202804468452,-4.44559361297825));
#55922=CARTESIAN_POINT('Ctrl Pts',(-35.5620948746067,4.14285526675692,-3.54653646505307));
#55923=CARTESIAN_POINT('Ctrl Pts',(-35.300583251693,4.13600582362742,-2.63111698861472));
#55924=CARTESIAN_POINT('Ctrl Pts',(-35.0820169555422,4.1311553285547,-2.69386316078375));
#55925=CARTESIAN_POINT('Ctrl Pts',(-34.7762954146415,4.123468523943,-1.62332480119136));
#55926=CARTESIAN_POINT('Ctrl Pts',(-34.5821230489298,4.11867398866152,-0.50868185551124));
#55927=CARTESIAN_POINT('Ctrl Pts',(-34.3775118580705,4.11384875218964,2.64941339379631));
#55928=CARTESIAN_POINT('Ctrl Pts',(-34.6423025074559,4.11873027055746,4.6907194393648));
#55929=CARTESIAN_POINT('Ctrl Pts',(-36.04198628679,4.1527224694396,8.88871095791407));
#55930=CARTESIAN_POINT('Ctrl Pts',(-37.3065050558491,4.18726914503329,10.9489520915154));
#55931=CARTESIAN_POINT('Ctrl Pts',(-41.8756295459123,4.39494595491279,15.6369502302462));
#55932=CARTESIAN_POINT('Ctrl Pts',(-50.1074923035213,4.9640760014635,19.0246939944322));
#55933=CARTESIAN_POINT('Ctrl Pts',(-58.2965417115554,6.22483785549351,15.6153467534928));
#55934=CARTESIAN_POINT('Ctrl Pts',(-62.8818624102576,6.84805526665328,10.9666861040641));
#55935=CARTESIAN_POINT('Ctrl Pts',(-64.1536744099658,7.05889697316184,8.903002529081));
#55936=CARTESIAN_POINT('Ctrl Pts',(-65.587111358284,7.2541543028841,4.709423159478));
#55937=CARTESIAN_POINT('Ctrl Pts',(-65.9028420963167,7.22055997092229,2.65197203401351));
#55938=CARTESIAN_POINT('Ctrl Pts',(-65.7186730629668,7.26645282243596,0.417296843035803));
#55939=CARTESIAN_POINT('Ctrl Pts',(-65.6635658897677,7.26567899418896,-0.115119959858279));
#55940=CARTESIAN_POINT('Ctrl Pts',(-65.4980339395569,7.22894983406278,-1.12644210521919));
#55941=CARTESIAN_POINT('Ctrl Pts',(-65.0673144851431,7.10361635805402,-2.85325522762648));
#55942=CARTESIAN_POINT('Ctrl Pts',(-64.5112907294815,7.02863116832091,-4.14935247202906));
#55943=CARTESIAN_POINT('Ctrl Pts',(-63.5261863279776,7.22128027561666,-5.90893413005372));
#55944=CARTESIAN_POINT('Ctrl Pts',(-62.068197594767,7.97414050458901,-8.03433541315561));
#55945=CARTESIAN_POINT('Ctrl Pts',(-60.0796098167125,7.87873199265082,-9.96197480208937));
#55946=CARTESIAN_POINT('Ctrl Pts',(-58.8895882593918,7.73549412644146,-10.8202271543694));
#55947=CARTESIAN_POINT('Ctrl Pts',(-58.5684317890665,7.6908639977441,-11.0130747863924));
#55948=CARTESIAN_POINT('Ctrl Pts',(-57.9084119982073,7.63003527898566,-11.4010944726287));
#55949=CARTESIAN_POINT('Ctrl Pts',(-56.7102378337881,7.56456386339554,-12.0170276546053));
#55950=CARTESIAN_POINT('Ctrl Pts',(-54.1289712559167,7.53905427079786,-13.0742974757744));
#55951=CARTESIAN_POINT('Ctrl Pts',(-49.9948035131066,7.02745080169609,-13.706606972641));
#55952=CARTESIAN_POINT('Ctrl Pts',(-46.1914722110254,5.3927514423487,-13.3156545423547));
#55953=CARTESIAN_POINT('Ctrl Pts',(-43.3908039796773,4.61571635395792,-12.5174764940247));
#55954=CARTESIAN_POINT('Ctrl Pts',(-41.9985023915937,4.44701923023704,-11.7653170427634));
#55955=CARTESIAN_POINT('Ctrl Pts',(-40.8028218808128,4.32952815033359,-10.9557009467549));
#55956=CARTESIAN_POINT('Ctrl Pts',(-39.754901868991,4.26984177464805,-10.1782379949765));
#55957=CARTESIAN_POINT('Ctrl Pts',(-37.85694008542,4.21051024093903,-8.27236172411371));
#55958=CARTESIAN_POINT('Ctrl Pts',(-36.735234866715,4.17590258588924,-6.60510917508678));
#55959=CARTESIAN_POINT('Ctrl Pts',(-35.7009394011684,4.14674880041722,-4.5350945305174));
#55960=CARTESIAN_POINT('Ctrl Pts',(-35.3472871931217,4.13782505970798,-3.62275408600405));
#55961=CARTESIAN_POINT('Ctrl Pts',(-35.0820169555422,4.1311553285547,-2.69386316078375));
#55962=CARTESIAN_POINT('Ctrl Pts',(-35.0820169555422,4.1311553285547,-2.69386316078375));
#55963=CARTESIAN_POINT('Ctrl Pts',(-35.300583251693,4.13600582362742,-2.63111698861473));
#55964=CARTESIAN_POINT('Ctrl Pts',(-35.8155534753675,3.95922815415782,-2.48463600652939));
#55965=CARTESIAN_POINT('Ctrl Pts',(-36.0650646070859,3.4346612700204,-2.41682844638411));
#55966=CARTESIAN_POINT('Ctrl Pts',(-36.065644266864,3.13140677366842,-2.41884872497431));
#55967=CARTESIAN_POINT('Ctrl Pts',(1.34046462259684,-0.994431239233107,
-23.5830172776492));
#55968=CARTESIAN_POINT('Ctrl Pts',(1.15566339708668,-0.981222287792037,
-23.7427314913969));
#55969=CARTESIAN_POINT('Ctrl Pts',(0.510597376526876,-0.937346932838556,
-24.1271727076141));
#55970=CARTESIAN_POINT('Ctrl Pts',(-0.795414560778026,-0.941634478778648,
-24.119095744646));
#55971=CARTESIAN_POINT('Ctrl Pts',(-1.58219675349064,-1.01297453127524,
-23.4267441649288));
#55972=CARTESIAN_POINT('Ctrl Pts',(-2.00978422295716,-1.0483911567391,-22.6184046246051));
#55973=CARTESIAN_POINT('Ctrl Pts',(-2.11303381784703,-1.05826233623046,
-22.0402329203993));
#55974=CARTESIAN_POINT('Ctrl Pts',(-1.91580205826814,-1.04028492443336,
-21.212120769873));
#55975=CARTESIAN_POINT('Ctrl Pts',(-1.54497027776593,-1.00976017368561,
-20.5983257098217));
#55976=CARTESIAN_POINT('Ctrl Pts',(-0.607145822015571,-0.940669573101927,
-19.9292256569487));
#55977=CARTESIAN_POINT('Ctrl Pts',(0.606887110287569,-0.939423264837247,
-19.9262432814847));
#55978=CARTESIAN_POINT('Ctrl Pts',(1.54458406111778,-1.00903316772747,-20.5984241362299));
#55979=CARTESIAN_POINT('Ctrl Pts',(2.14134596539594,-1.05914052353263,-21.578464777093));
#55980=CARTESIAN_POINT('Ctrl Pts',(2.07601143327058,-1.05435985255611,-22.4957984055296));
#55981=CARTESIAN_POINT('Ctrl Pts',(1.69261614119323,-1.02145958385162,-23.2155194332715));
#55982=CARTESIAN_POINT('Ctrl Pts',(1.53141254982529,-1.00807953562059,-23.4179907851037));
#55983=CARTESIAN_POINT('Ctrl Pts',(1.34046462259684,-0.994431239233105,
-23.5830172776492));
#55984=CARTESIAN_POINT('Ctrl Pts',(1.33240415293763,-1.28753222554999,-23.5899835278486));
#55985=CARTESIAN_POINT('Ctrl Pts',(1.1469157030279,-1.27577525109937,-23.7485337176985));
#55986=CARTESIAN_POINT('Ctrl Pts',(0.501623816284161,-1.23758746220324,
-24.1249425674433));
#55987=CARTESIAN_POINT('Ctrl Pts',(-0.780574636333104,-1.2409583285191,
-24.1189164938403));
#55988=CARTESIAN_POINT('Ctrl Pts',(-1.57425541223237,-1.3038793604076,-23.435400280391));
#55989=CARTESIAN_POINT('Ctrl Pts',(-2.00781896637476,-1.33644887563698,
-22.6230530338899));
#55990=CARTESIAN_POINT('Ctrl Pts',(-2.11303497262538,-1.34561536136995,
-22.0396719347269));
#55991=CARTESIAN_POINT('Ctrl Pts',(-1.91258908442446,-1.32903543096936,
-21.2060259117698));
#55992=CARTESIAN_POINT('Ctrl Pts',(-1.53633055206404,-1.30096043919022,
-20.5893234525047));
#55993=CARTESIAN_POINT('Ctrl Pts',(-0.596251688256806,-1.24026580005628,
-19.9304047255554));
#55994=CARTESIAN_POINT('Ctrl Pts',(0.595626544455079,-1.23930620689027,
-19.9281869876753));
#55995=CARTESIAN_POINT('Ctrl Pts',(1.53605999452011,-1.30033581584115,-20.5900175249093));
#55996=CARTESIAN_POINT('Ctrl Pts',(2.14157620787691,-1.34648816973293,-21.5740783667172));
#55997=CARTESIAN_POINT('Ctrl Pts',(2.07534233636514,-1.34187841054564,-22.5011424018098));
#55998=CARTESIAN_POINT('Ctrl Pts',(1.68697288849109,-1.31176837112141,-23.2237452080945));
#55999=CARTESIAN_POINT('Ctrl Pts',(1.52406216244111,-1.29968025051912,-23.4261597759772));
#56000=CARTESIAN_POINT('Ctrl Pts',(1.33240415293763,-1.28753222554998,-23.5899835278486));
#56001=CARTESIAN_POINT('Ctrl Pts',(1.4758309169534,-1.79544747755601,-23.7841728091566));
#56002=CARTESIAN_POINT('Ctrl Pts',(1.26838865034841,-1.78601872806586,-23.9621689855623));
#56003=CARTESIAN_POINT('Ctrl Pts',(0.551030494946323,-1.75703447393435,
-24.3824714148802));
#56004=CARTESIAN_POINT('Ctrl Pts',(-0.858786621919096,-1.75892874024821,
-24.3770422952472));
#56005=CARTESIAN_POINT('Ctrl Pts',(-1.74729745582464,-1.80824551117858,
-23.6127100620137));
#56006=CARTESIAN_POINT('Ctrl Pts',(-2.23527843187923,-1.8361855302437,-22.6984081072173));
#56007=CARTESIAN_POINT('Ctrl Pts',(-2.35403929323783,-1.84418965457546,
-22.0410059801487));
#56008=CARTESIAN_POINT('Ctrl Pts',(-2.12796028967623,-1.82989818874935,
-21.1014645536594));
#56009=CARTESIAN_POINT('Ctrl Pts',(-1.70448676238135,-1.80582090614153,
-20.4074451781338));
#56010=CARTESIAN_POINT('Ctrl Pts',(-0.655240694168969,-1.75868262352979,
-19.6708937823934));
#56011=CARTESIAN_POINT('Ctrl Pts',(0.655193324216905,-1.7581595208231,-19.6684797661189));
#56012=CARTESIAN_POINT('Ctrl Pts',(1.70386306074689,-1.80534861734831,-20.4079383197073));
#56013=CARTESIAN_POINT('Ctrl Pts',(2.38615076333066,-1.84508770821069,-21.5157914644901));
#56014=CARTESIAN_POINT('Ctrl Pts',(2.31069308799246,-1.8407737494664,-22.5596482740071));
#56015=CARTESIAN_POINT('Ctrl Pts',(1.87321043198864,-1.81518150600845,-23.3728871164866));
#56016=CARTESIAN_POINT('Ctrl Pts',(1.69017295239418,-1.80518983811954,-23.6002562748075));
#56017=CARTESIAN_POINT('Ctrl Pts',(1.4758309169534,-1.79544747755601,-23.7841728091566));
#56018=CARTESIAN_POINT('Ctrl Pts',(1.80304354213939,-1.98648318031429,-24.1734013935208));
#56019=CARTESIAN_POINT('Ctrl Pts',(1.55183159751857,-1.97512642852453,-24.3932594536731));
#56020=CARTESIAN_POINT('Ctrl Pts',(0.679721866652848,-1.93861163401404,
-24.9201620196685));
#56021=CARTESIAN_POINT('Ctrl Pts',(-1.05900238101113,-1.94168634007152,
-24.910084768943));
#56022=CARTESIAN_POINT('Ctrl Pts',(-2.13145659008938,-2.00220229591781,
-23.9590865594632));
#56023=CARTESIAN_POINT('Ctrl Pts',(-2.71931215681635,-2.03407334807429,
-22.8426999176217));
#56024=CARTESIAN_POINT('Ctrl Pts',(-2.86228855524459,-2.04307423559703,
-22.043277402193));
#56025=CARTESIAN_POINT('Ctrl Pts',(-2.59014207056062,-2.02683577645921,
-20.8988502028586));
#56026=CARTESIAN_POINT('Ctrl Pts',(-2.08038729224802,-1.99936686297598,
-20.051300417594));
#56027=CARTESIAN_POINT('Ctrl Pts',(-0.80844853421373,-1.94110132490594,
-19.1332915718003));
#56028=CARTESIAN_POINT('Ctrl Pts',(0.808258885423883,-1.94022830439346,
-19.1294522906829));
#56029=CARTESIAN_POINT('Ctrl Pts',(2.07969237177025,-1.99876909577637,-20.0515337319994));
#56030=CARTESIAN_POINT('Ctrl Pts',(2.90085466420141,-2.04396331371082,-21.404748876263));
#56031=CARTESIAN_POINT('Ctrl Pts',(2.81033956030822,-2.03937236813819,-22.6732842137794));
#56032=CARTESIAN_POINT('Ctrl Pts',(2.28328462136404,-2.00996084831922,-23.6670462324578));
#56033=CARTESIAN_POINT('Ctrl Pts',(2.06261108552529,-1.99821767075566,-23.946230600932));
#56034=CARTESIAN_POINT('Ctrl Pts',(1.80304354213939,-1.98648318031429,-24.1734013935208));
#56035=CARTESIAN_POINT('Ctrl Pts',(1.94662784270136,-1.99329185033283,-24.3399175880524));
#56036=CARTESIAN_POINT('Ctrl Pts',(1.67638127074653,-1.98030748769492,-24.5776542418215));
#56037=CARTESIAN_POINT('Ctrl Pts',(0.736629093141336,-1.93751000700026,
-25.1500576569261));
#56038=CARTESIAN_POINT('Ctrl Pts',(-1.14750345414621,-1.94155549971475,
-25.1379865951392));
#56039=CARTESIAN_POINT('Ctrl Pts',(-2.29979798593773,-2.01146084484187,
-24.1072334392769));
#56040=CARTESIAN_POINT('Ctrl Pts',(-2.93067378779831,-2.04663627148226,
-22.9044123516052));
#56041=CARTESIAN_POINT('Ctrl Pts',(-3.08401460891383,-2.05645871391943,
-22.0442241048096));
#56042=CARTESIAN_POINT('Ctrl Pts',(-2.79208955112528,-2.03860098114137,
-20.8121763806738));
#56043=CARTESIAN_POINT('Ctrl Pts',(-2.24515915919612,-2.00827757256358,
-19.898951478238));
#56044=CARTESIAN_POINT('Ctrl Pts',(-0.876173007874418,-1.94068884397439,
-18.9033970954646));
#56045=CARTESIAN_POINT('Ctrl Pts',(0.875895764425228,-1.93951554837252,
-18.8989606653587));
#56046=CARTESIAN_POINT('Ctrl Pts',(2.2444503085602,-2.00757360901504,-19.8990971193787));
#56047=CARTESIAN_POINT('Ctrl Pts',(3.12537961073622,-2.05736838288602,-21.3572403317401));
#56048=CARTESIAN_POINT('Ctrl Pts',(3.02843680266979,-2.05254349855045,-22.721972135133));
#56049=CARTESIAN_POINT('Ctrl Pts',(2.46280778521956,-2.01992324553137,-23.7929340812186));
#56050=CARTESIAN_POINT('Ctrl Pts',(2.22586312706117,-2.00670808783477,-24.0942735392203));
#56051=CARTESIAN_POINT('Ctrl Pts',(1.94662784270136,-1.99329185033284,-24.3399175880524));
#56052=CARTESIAN_POINT('',(1.34046462259684,-0.994431239233107,-23.5830172776492));
#56053=CARTESIAN_POINT('Ctrl Pts',(1.94661322350961,-1.99329115684075,-24.3399006340105));
#56054=CARTESIAN_POINT('Ctrl Pts',(1.80303402327035,-1.9864776228478,-24.1733900705544));
#56055=CARTESIAN_POINT('Ctrl Pts',(1.47582883074698,-1.79544008970153,-23.7841699845866));
#56056=CARTESIAN_POINT('Ctrl Pts',(1.33240415293763,-1.28753222554999,-23.5899835278486));
#56057=CARTESIAN_POINT('Ctrl Pts',(1.34046462259684,-0.994431239233107,
-23.5830172776492));
#56058=CARTESIAN_POINT('',(-2.04965785769565,-1.05238869753535,-22.0330650649484));
#56059=CARTESIAN_POINT('Ctrl Pts',(1.34046462259684,-0.994431239233107,
-23.5830172776492));
#56060=CARTESIAN_POINT('Ctrl Pts',(1.15566339708668,-0.981222287792037,
-23.7427314913969));
#56061=CARTESIAN_POINT('Ctrl Pts',(0.510597376526876,-0.937346932838556,
-24.1271727076141));
#56062=CARTESIAN_POINT('Ctrl Pts',(-0.795414560778026,-0.941634478778648,
-24.119095744646));
#56063=CARTESIAN_POINT('Ctrl Pts',(-1.58219675349064,-1.01297453127524,
-23.4267441649288));
#56064=CARTESIAN_POINT('Ctrl Pts',(-1.96798801478004,-1.04492922027809,
-22.6974189318937));
#56065=CARTESIAN_POINT('Ctrl Pts',(-2.04906955950107,-1.05226003620114,
-22.3656080815114));
#56066=CARTESIAN_POINT('Ctrl Pts',(-2.04965785769565,-1.05238869753535,
-22.0330650649484));
#56067=CARTESIAN_POINT('Ctrl Pts',(-2.04965785769565,-1.05238869753535,
-22.0330650649484));
#56068=CARTESIAN_POINT('Ctrl Pts',(-2.04981577269251,-1.05242323368449,
-21.9438016099532));
#56069=CARTESIAN_POINT('Ctrl Pts',(-2.0352872104395,-1.05117583667188,-21.7138001471288));
#56070=CARTESIAN_POINT('Ctrl Pts',(-1.91580205826814,-1.04028492443336,
-21.212120769873));
#56071=CARTESIAN_POINT('Ctrl Pts',(-1.54497027776593,-1.00976017368561,
-20.5983257098217));
#56072=CARTESIAN_POINT('Ctrl Pts',(-0.607145822015571,-0.940669573101927,
-19.9292256569487));
#56073=CARTESIAN_POINT('Ctrl Pts',(0.606887110287569,-0.939423264837247,
-19.9262432814847));
#56074=CARTESIAN_POINT('Ctrl Pts',(1.54458406111778,-1.00903316772747,-20.5984241362299));
#56075=CARTESIAN_POINT('Ctrl Pts',(2.14134596539594,-1.05914052353263,-21.578464777093));
#56076=CARTESIAN_POINT('Ctrl Pts',(2.07601143327058,-1.05435985255611,-22.4957984055296));
#56077=CARTESIAN_POINT('Ctrl Pts',(1.69261614119323,-1.02145958385162,-23.2155194332715));
#56078=CARTESIAN_POINT('Ctrl Pts',(1.53141254982529,-1.00807953562059,-23.4179907851037));
#56079=CARTESIAN_POINT('Ctrl Pts',(1.34046462259684,-0.994431239233105,
-23.5830172776492));
#56080=CARTESIAN_POINT('Origin',(0.,-32.64,-22.032));
#56081=CARTESIAN_POINT('',(-2.04798719608651,1.031471238741,-22.0314998033837));
#56082=CARTESIAN_POINT('',(-2.05,-32.64,-22.032));
#56083=CARTESIAN_POINT('',(1.06033811196866,1.10557153022754,-23.7864751603562));
#56084=CARTESIAN_POINT('Ctrl Pts',(1.06033811196866,1.10557153022754,-23.7864751603562));
#56085=CARTESIAN_POINT('Ctrl Pts',(1.3741706509286,1.08763482658183,-23.5968067003208));
#56086=CARTESIAN_POINT('Ctrl Pts',(1.6389112117965,1.06602766214671,-23.3172136393184));
#56087=CARTESIAN_POINT('Ctrl Pts',(2.07504458979883,1.02978963073027,-22.4955454402302));
#56088=CARTESIAN_POINT('Ctrl Pts',(2.16671526713221,1.02015496747681,-21.2738800000443));
#56089=CARTESIAN_POINT('Ctrl Pts',(1.12497802521023,1.11222339267956,-20.1511354024741));
#56090=CARTESIAN_POINT('Ctrl Pts',(-2.22411254650599E-5,1.14324344009484,
-19.9249469059644));
#56091=CARTESIAN_POINT('Ctrl Pts',(-1.12483654553001,1.11241940027572,-20.1519785870164));
#56092=CARTESIAN_POINT('Ctrl Pts',(-1.92005960293299,1.04196266266284,-21.0068804220012));
#56093=CARTESIAN_POINT('Ctrl Pts',(-2.04846270330842,1.03133303488674,-21.8009775414312));
#56094=CARTESIAN_POINT('Ctrl Pts',(-2.04798719608651,1.031471238741,-22.0314998033837));
#56095=CARTESIAN_POINT('Ctrl Pts',(-2.04798719608651,1.031471238741,-22.0314998033837));
#56096=CARTESIAN_POINT('Ctrl Pts',(-2.0472990346369,1.0316712495091,-22.3651152074008));
#56097=CARTESIAN_POINT('Ctrl Pts',(-1.96760078125492,1.03861898694433,-22.6990725582984));
#56098=CARTESIAN_POINT('Ctrl Pts',(-1.65476826134601,1.06448801082077,-23.2866051421743));
#56099=CARTESIAN_POINT('Ctrl Pts',(-1.19459273103418,1.10242309331756,-23.7986869773671));
#56100=CARTESIAN_POINT('Ctrl Pts',(-0.11883654419667,1.1509767800617,-24.1919960917867));
#56101=CARTESIAN_POINT('Ctrl Pts',(0.681458753251526,1.12722590296183,-24.0154554462922));
#56102=CARTESIAN_POINT('Ctrl Pts',(1.06033811196866,1.10557153022754,-23.7864751603562));
#56103=CARTESIAN_POINT('Ctrl Pts',(1.06033811196866,1.10557153022754,-23.7864751603562));
#56104=CARTESIAN_POINT('Ctrl Pts',(1.3741706509286,1.08763482658183,-23.5968067003208));
#56105=CARTESIAN_POINT('Ctrl Pts',(1.6389112117965,1.06602766214671,-23.3172136393184));
#56106=CARTESIAN_POINT('Ctrl Pts',(2.07504458979883,1.02978963073027,-22.4955454402302));
#56107=CARTESIAN_POINT('Ctrl Pts',(2.16671526713221,1.02015496747681,-21.2738800000443));
#56108=CARTESIAN_POINT('Ctrl Pts',(1.12497802521023,1.11222339267956,-20.1511354024741));
#56109=CARTESIAN_POINT('Ctrl Pts',(-2.22411254650599E-5,1.14324344009484,
-19.9249469059644));
#56110=CARTESIAN_POINT('Ctrl Pts',(-1.12483654553001,1.11241940027572,-20.1519785870164));
#56111=CARTESIAN_POINT('Ctrl Pts',(-2.16645281839403,1.02013223160363,-21.2717646077205));
#56112=CARTESIAN_POINT('Ctrl Pts',(-2.07546536871258,1.02969935292042,-22.4964914462192));
#56113=CARTESIAN_POINT('Ctrl Pts',(-1.65476826134601,1.06448801082077,-23.2866051421743));
#56114=CARTESIAN_POINT('Ctrl Pts',(-1.19459273103418,1.10242309331756,-23.7986869773671));
#56115=CARTESIAN_POINT('Ctrl Pts',(-0.11883654419667,1.1509767800617,-24.1919960917867));
#56116=CARTESIAN_POINT('Ctrl Pts',(0.681458753251526,1.12722590296183,-24.0154554462922));
#56117=CARTESIAN_POINT('Ctrl Pts',(1.06033811196866,1.10557153022754,-23.7864751603562));
#56118=CARTESIAN_POINT('Ctrl Pts',(1.06885567305814,1.40828367652872,-23.7813274701248));
#56119=CARTESIAN_POINT('Ctrl Pts',(1.38248586686808,1.39243884639632,-23.5895875529348));
#56120=CARTESIAN_POINT('Ctrl Pts',(1.64436283152676,1.3732095635864,-23.3087243380774));
#56121=CARTESIAN_POINT('Ctrl Pts',(2.07314889996122,1.34044977214445,-22.4906135360011));
#56122=CARTESIAN_POINT('Ctrl Pts',(2.16411028206747,1.33196913158902,-21.2847252513266));
#56123=CARTESIAN_POINT('Ctrl Pts',(1.13744447201766,1.4143568387895,-20.1592143027524));
#56124=CARTESIAN_POINT('Ctrl Pts',(-0.000256227932920122,1.44137426575786,
-19.92387643395));
#56125=CARTESIAN_POINT('Ctrl Pts',(-1.13694778952218,1.41450806520655,-20.1595508202468));
#56126=CARTESIAN_POINT('Ctrl Pts',(-2.16383403896832,1.33195045856082,-21.2825688856218));
#56127=CARTESIAN_POINT('Ctrl Pts',(-2.07325337832862,1.34033815950352,-22.4907608848192));
#56128=CARTESIAN_POINT('Ctrl Pts',(-1.6592835139715,1.37180588493616,-23.2775613318082));
#56129=CARTESIAN_POINT('Ctrl Pts',(-1.20487142745969,1.40556608560269,-23.7910434905851));
#56130=CARTESIAN_POINT('Ctrl Pts',(-0.122112202043455,1.4482379067298,-24.1940212246999));
#56131=CARTESIAN_POINT('Ctrl Pts',(0.690220598763919,1.42741260146251,-24.0128085558852));
#56132=CARTESIAN_POINT('Ctrl Pts',(1.06885567305814,1.40828367652872,-23.7813274701248));
#56133=CARTESIAN_POINT('Ctrl Pts',(1.21687788573647,1.93213443184209,-23.992953261104));
#56134=CARTESIAN_POINT('Ctrl Pts',(1.57324186146248,1.91959724479566,-23.7763501693715));
#56135=CARTESIAN_POINT('Ctrl Pts',(1.8683540783032,1.9042141351763,-23.4608590636703));
#56136=CARTESIAN_POINT('Ctrl Pts',(2.34973256394823,1.87701976965164,-22.5436171337775));
#56137=CARTESIAN_POINT('Ctrl Pts',(2.45226711834097,1.87047554852946,-21.1978834357668));
#56138=CARTESIAN_POINT('Ctrl Pts',(1.29873523523315,1.93739606097254,-19.9306130867953));
#56139=CARTESIAN_POINT('Ctrl Pts',(-2.48986141743091E-5,1.95795842159875,
-19.6634199435529));
#56140=CARTESIAN_POINT('Ctrl Pts',(-1.29846053070403,1.93745323324118,-19.9312506887653));
#56141=CARTESIAN_POINT('Ctrl Pts',(-2.45198106316624,1.87046011766442,-21.1955379468141));
#56142=CARTESIAN_POINT('Ctrl Pts',(-2.35021929528818,1.87691821348825,-22.5445287638371));
#56143=CARTESIAN_POINT('Ctrl Pts',(-1.88580976045264,1.90305993699306,-23.4266020673305));
#56144=CARTESIAN_POINT('Ctrl Pts',(-1.37432153671418,1.93016224431321,-24.003984576668));
#56145=CARTESIAN_POINT('Ctrl Pts',(-0.13951160354739,1.96345677777968,-24.4611199386481));
#56146=CARTESIAN_POINT('Ctrl Pts',(0.786651768838543,1.94727015168814,-24.2544508125171));
#56147=CARTESIAN_POINT('Ctrl Pts',(1.21687788573647,1.93213443184209,-23.992953261104));
#56148=CARTESIAN_POINT('Ctrl Pts',(1.49832696166209,2.10922709805227,-24.4473929779526));
#56149=CARTESIAN_POINT('Ctrl Pts',(1.93946239340197,2.09347121942612,-24.184968765879));
#56150=CARTESIAN_POINT('Ctrl Pts',(2.30810979033992,2.07439966898151,-23.79924586829));
#56151=CARTESIAN_POINT('Ctrl Pts',(2.91131182915358,2.04195622182916,-22.6683467986794));
#56152=CARTESIAN_POINT('Ctrl Pts',(3.03948394883541,2.03353491233303,-20.9920377381179));
#56153=CARTESIAN_POINT('Ctrl Pts',(1.59432559617741,2.11523562113408,-19.4424175335459));
#56154=CARTESIAN_POINT('Ctrl Pts',(-3.29269739570931E-5,2.14220011170132,
-19.126726079993));
#56155=CARTESIAN_POINT('Ctrl Pts',(-1.59401433946836,2.11538707819239,-19.4435006465808));
#56156=CARTESIAN_POINT('Ctrl Pts',(-3.03913212305212,2.03351582365801,-20.989134884764));
#56157=CARTESIAN_POINT('Ctrl Pts',(-2.91185846141516,2.04185422508344,-22.6696329552038));
#56158=CARTESIAN_POINT('Ctrl Pts',(-2.32998889963734,2.07301540754862,-23.757123907291));
#56159=CARTESIAN_POINT('Ctrl Pts',(-1.69011408984992,2.10650576808936,-24.4634914741773));
#56160=CARTESIAN_POINT('Ctrl Pts',(-0.169731804772517,2.14900999872136,
-25.0099387468857));
#56161=CARTESIAN_POINT('Ctrl Pts',(0.965759146868535,2.12824863485557,-24.764208810727));
#56162=CARTESIAN_POINT('Ctrl Pts',(1.49832696166209,2.10922709805227,-24.4473929779526));
#56163=CARTESIAN_POINT('Ctrl Pts',(1.61567592638144,2.10484535966067,-24.6418414854819));
#56164=CARTESIAN_POINT('Ctrl Pts',(2.09220096563961,2.08654257832164,-24.3598140131154));
#56165=CARTESIAN_POINT('Ctrl Pts',(2.4917371536323,2.06460141183357,-23.9440137803207));
#56166=CARTESIAN_POINT('Ctrl Pts',(3.14638574337583,2.02805778890562,-22.7217241578602));
#56167=CARTESIAN_POINT('Ctrl Pts',(3.28527751630146,2.01819894837187,-20.9040192764535));
#56168=CARTESIAN_POINT('Ctrl Pts',(1.71728341750388,2.11146607039885,-19.2336854760647));
#56169=CARTESIAN_POINT('Ctrl Pts',(-5.68372511193975E-5,2.14348108036939,
-18.8971771498333));
#56170=CARTESIAN_POINT('Ctrl Pts',(-1.71693918475569,2.11168339882122,-19.2349389943924));
#56171=CARTESIAN_POINT('Ctrl Pts',(-3.2848943379376,2.01817562027762,-20.9008741138759));
#56172=CARTESIAN_POINT('Ctrl Pts',(-3.14693139817671,2.02797312390453,-22.7231264087792));
#56173=CARTESIAN_POINT('Ctrl Pts',(-2.51542689144179,2.06305029395261,-23.8984874041331));
#56174=CARTESIAN_POINT('Ctrl Pts',(-1.8215791399191,2.10154489826223,-24.6600514792354));
#56175=CARTESIAN_POINT('Ctrl Pts',(-0.182315527702726,2.1513398143738,-25.2447478054221));
#56176=CARTESIAN_POINT('Ctrl Pts',(1.04038344114352,2.12694168555298,-24.9823236681931));
#56177=CARTESIAN_POINT('Ctrl Pts',(1.61567592638144,2.10484535966067,-24.6418414854819));
#56178=CARTESIAN_POINT('Ctrl Pts',(1.61567592638144,2.10484535966067,-24.6418414854819));
#56179=CARTESIAN_POINT('Ctrl Pts',(1.49832696166209,2.10922709805227,-24.4473929779526));
#56180=CARTESIAN_POINT('Ctrl Pts',(1.21687788573647,1.93213443184209,-23.992953261104));
#56181=CARTESIAN_POINT('Ctrl Pts',(1.06885567305814,1.40828367652872,-23.7813274701248));
#56182=CARTESIAN_POINT('Ctrl Pts',(1.06033811196866,1.10557153022754,-23.7864751603562));
#56183=CARTESIAN_POINT('Ctrl Pts',(1.32735269144094,-1.10555525796307,-31.754253126905));
#56184=CARTESIAN_POINT('Ctrl Pts',(1.06710073148761,-1.09683487190185,-31.975373592947));
#56185=CARTESIAN_POINT('Ctrl Pts',(0.428155187551756,-1.06165436373511,
-32.2864496159946));
#56186=CARTESIAN_POINT('Ctrl Pts',(-0.630282194184733,-1.0692102615866,
-32.2353219180946));
#56187=CARTESIAN_POINT('Ctrl Pts',(-1.53618081272622,-1.12324621261658,
-31.6799876467057));
#56188=CARTESIAN_POINT('Ctrl Pts',(-2.06354935994887,-1.09811456220838,
-30.7530725805608));
#56189=CARTESIAN_POINT('Ctrl Pts',(-2.07369689301627,-1.05472770793943,
-30.0461163773485));
#56190=CARTESIAN_POINT('Ctrl Pts',(-1.95022898432517,-1.04370742396877,
-29.5338952679768));
#56191=CARTESIAN_POINT('Ctrl Pts',(-1.81664117243763,-1.0312338635184,-29.1901382103174));
#56192=CARTESIAN_POINT('Ctrl Pts',(-1.37870319165073,-0.994208730015135,
-28.5976563596733));
#56193=CARTESIAN_POINT('Ctrl Pts',(-0.565632139754401,-0.938431810497882,
-28.1175164175936));
#56194=CARTESIAN_POINT('Ctrl Pts',(0.566051291595285,-0.938787274998903,
-28.1186849695365));
#56195=CARTESIAN_POINT('Ctrl Pts',(1.29716483238625,-0.988597635068523,
-28.5489950966502));
#56196=CARTESIAN_POINT('Ctrl Pts',(1.65332946690085,-1.01745671260863,-28.9696512040306));
#56197=CARTESIAN_POINT('Ctrl Pts',(1.80035161541673,-1.0302070446804,-29.1988189274931));
#56198=CARTESIAN_POINT('Ctrl Pts',(1.89755296929512,-1.0389008897144,-29.406736531242));
#56199=CARTESIAN_POINT('Ctrl Pts',(1.95792514729417,-1.04441107544017,-29.5794738833423));
#56200=CARTESIAN_POINT('Ctrl Pts',(1.98223924757779,-1.04664413680767,-29.6674728551243));
#56201=CARTESIAN_POINT('Ctrl Pts',(2.02810945191073,-1.0508832347292,-29.8577107402739));
#56202=CARTESIAN_POINT('Ctrl Pts',(2.06564184504211,-1.0616449129841,-30.159982754614));
#56203=CARTESIAN_POINT('Ctrl Pts',(1.99588940266396,-1.10355864373223,-30.9150513968238));
#56204=CARTESIAN_POINT('Ctrl Pts',(1.67008090765068,-1.11703921512503,-31.4630575374169));
#56205=CARTESIAN_POINT('Ctrl Pts',(1.32735269144094,-1.10555525796307,-31.754253126905));
#56206=CARTESIAN_POINT('Ctrl Pts',(1.32359268837332,-1.3930284764443,-31.7574477757783));
#56207=CARTESIAN_POINT('Ctrl Pts',(1.06075990223367,-1.38701669149454,-31.9795472988009));
#56208=CARTESIAN_POINT('Ctrl Pts',(0.419725709553912,-1.3602190366849,-32.2844089798952));
#56209=CARTESIAN_POINT('Ctrl Pts',(-0.618485714611421,-1.36594619964849,
-32.2352048569959));
#56210=CARTESIAN_POINT('Ctrl Pts',(-1.53434167017165,-1.40706476564176,
-31.6853452283511));
#56211=CARTESIAN_POINT('Ctrl Pts',(-2.06756518656419,-1.38208136621911,
-30.7392367955497));
#56212=CARTESIAN_POINT('Ctrl Pts',(-2.07107027760732,-1.34300067689607,
-30.0368863357017));
#56213=CARTESIAN_POINT('Ctrl Pts',(-1.94807632133963,-1.33142265611008,
-29.5305662158123));
#56214=CARTESIAN_POINT('Ctrl Pts',(-1.81175633221395,-1.32042474667762,
-29.1822460250395));
#56215=CARTESIAN_POINT('Ctrl Pts',(-1.3687168401187,-1.28652020920908,-28.5906178404563));
#56216=CARTESIAN_POINT('Ctrl Pts',(-0.555659683581034,-1.23798415259695,
-28.1189521130734));
#56217=CARTESIAN_POINT('Ctrl Pts',(0.556795084374633,-1.23819678242899,
-28.1201472467162));
#56218=CARTESIAN_POINT('Ctrl Pts',(1.28744457447514,-1.28184563228667,-28.5417785542487));
#56219=CARTESIAN_POINT('Ctrl Pts',(1.64696260849818,-1.30788994439935,-28.9617938965102));
#56220=CARTESIAN_POINT('Ctrl Pts',(1.79566840873594,-1.31945564515493,-29.1912135128309));
#56221=CARTESIAN_POINT('Ctrl Pts',(1.89426584711195,-1.32742070284596,-29.400029974807));
#56222=CARTESIAN_POINT('Ctrl Pts',(1.95553864001657,-1.33248283811966,-29.5737054711291));
#56223=CARTESIAN_POINT('Ctrl Pts',(1.98023234041262,-1.33453601106632,-29.6622637213054));
#56224=CARTESIAN_POINT('Ctrl Pts',(2.02679416400233,-1.33848243383651,-29.8536245299278));
#56225=CARTESIAN_POINT('Ctrl Pts',(2.06442657207142,-1.34907719838766,-30.1508642304607));
#56226=CARTESIAN_POINT('Ctrl Pts',(2.00034510775818,-1.38695750726818,-30.9054053055921));
#56227=CARTESIAN_POINT('Ctrl Pts',(1.6697196184884,-1.40094545171871,-31.4649628570855));
#56228=CARTESIAN_POINT('Ctrl Pts',(1.32359268837332,-1.3930284764443,-31.7574477757783));
#56229=CARTESIAN_POINT('Ctrl Pts',(1.46653971754463,-1.8915537217059,-31.9389064298716));
#56230=CARTESIAN_POINT('Ctrl Pts',(1.17208250986832,-1.88990990750113,-32.1922127295594));
#56231=CARTESIAN_POINT('Ctrl Pts',(0.460648793220428,-1.87680187973207,
-32.5388567043923));
#56232=CARTESIAN_POINT('Ctrl Pts',(-0.679806548016544,-1.87951434725149,
-32.4836938552306));
#56233=CARTESIAN_POINT('Ctrl Pts',(-1.70258640950013,-1.89979282381933,
-31.8577659411165));
#56234=CARTESIAN_POINT('Ctrl Pts',(-2.30312627589108,-1.87494954073869,
-30.7804042928418));
#56235=CARTESIAN_POINT('Ctrl Pts',(-2.3047574810545,-1.84291420533356,-30.0049321102413));
#56236=CARTESIAN_POINT('Ctrl Pts',(-2.16713537988374,-1.83047398511645,
-29.450084851244));
#56237=CARTESIAN_POINT('Ctrl Pts',(-2.01322265024838,-1.82185288488754,
-29.0528943526148));
#56238=CARTESIAN_POINT('Ctrl Pts',(-1.51600088272362,-1.79307985743714,
-28.3908970609083));
#56239=CARTESIAN_POINT('Ctrl Pts',(-0.612040482336112,-1.75621723925646,
-27.8627033356224));
#56240=CARTESIAN_POINT('Ctrl Pts',(0.612324780435475,-1.75625510817756,
-27.8650485172928));
#56241=CARTESIAN_POINT('Ctrl Pts',(1.42455024203057,-1.78983816998982,-28.3335961136323));
#56242=CARTESIAN_POINT('Ctrl Pts',(1.82755327624387,-1.81131968108437,-28.8054906524833));
#56243=CARTESIAN_POINT('Ctrl Pts',(1.99464262300472,-1.82096843430477,-29.0635047207685));
#56244=CARTESIAN_POINT('Ctrl Pts',(2.10562099039111,-1.82774616567129,-29.2985549129538));
#56245=CARTESIAN_POINT('Ctrl Pts',(2.1746649507395,-1.83208104982681,-29.4941944943251));
#56246=CARTESIAN_POINT('Ctrl Pts',(2.2025166171187,-1.83384404888901,-29.594055594785));
#56247=CARTESIAN_POINT('Ctrl Pts',(2.25497054882611,-1.83730258309225,-29.8091760872681));
#56248=CARTESIAN_POINT('Ctrl Pts',(2.29712794695441,-1.84758569353084,-30.1318884172415));
#56249=CARTESIAN_POINT('Ctrl Pts',(2.22692569402416,-1.87892699693054,-30.9729351466869));
#56250=CARTESIAN_POINT('Ctrl Pts',(1.85431314124951,-1.89371847585523,-31.6053250179881));
#56251=CARTESIAN_POINT('Ctrl Pts',(1.46653971754463,-1.8915537217059,-31.9389064298717));
#56252=CARTESIAN_POINT('Ctrl Pts',(1.78295981235903,-2.09034202746774,-32.3165923940998));
#56253=CARTESIAN_POINT('Ctrl Pts',(1.42887704568795,-2.08528185371715,-32.6294992152107));
#56254=CARTESIAN_POINT('Ctrl Pts',(0.5682747633569,-2.06094872479154,-33.0717163335162));
#56255=CARTESIAN_POINT('Ctrl Pts',(-0.837377841698829,-2.06620701234019,
-32.9989619534493));
#56256=CARTESIAN_POINT('Ctrl Pts',(-2.0651652506236,-2.10333070270456,-32.2093337878777));
#56257=CARTESIAN_POINT('Ctrl Pts',(-2.79217267385067,-2.07752992562671,
-30.9061146080709));
#56258=CARTESIAN_POINT('Ctrl Pts',(-2.80438461577025,-2.04051125226246,
-29.9635496597121));
#56259=CARTESIAN_POINT('Ctrl Pts',(-2.63548264699564,-2.02890333097792,
-29.2894223532697));
#56260=CARTESIAN_POINT('Ctrl Pts',(-2.45137426614447,-2.01824716085344,
-28.8045713252895));
#56261=CARTESIAN_POINT('Ctrl Pts',(-1.85198515728335,-1.98522456653967,
-27.9937075036918));
#56262=CARTESIAN_POINT('Ctrl Pts',(-0.753821627316684,-1.93883646088754,
-27.3319251834597));
#56263=CARTESIAN_POINT('Ctrl Pts',(0.754378094218889,-1.93902779172867,
-27.3349745231335));
#56264=CARTESIAN_POINT('Ctrl Pts',(1.74159121964216,-1.98078805737154,-27.921968319788));
#56265=CARTESIAN_POINT('Ctrl Pts',(2.22779548254146,-2.00605371647797,-28.5013840066074));
#56266=CARTESIAN_POINT('Ctrl Pts',(2.42910284089573,-2.01729978469252,-28.8172792473517));
#56267=CARTESIAN_POINT('Ctrl Pts',(2.56263060668496,-2.02507503169194,-29.1041603431301));
#56268=CARTESIAN_POINT('Ctrl Pts',(2.64567276448555,-2.03002288631674,-29.3426222472456));
#56269=CARTESIAN_POINT('Ctrl Pts',(2.67915108961055,-2.03203164657226,-29.4642451627364));
#56270=CARTESIAN_POINT('Ctrl Pts',(2.74228969748,-2.03589942781969,-29.7261453244971));
#56271=CARTESIAN_POINT('Ctrl Pts',(2.79358493531193,-2.0461853708987,-30.118560451381));
#56272=CARTESIAN_POINT('Ctrl Pts',(2.69905012072682,-2.08239625976544,-31.139014614668));
#56273=CARTESIAN_POINT('Ctrl Pts',(2.24925468688582,-2.09700581714128,-31.9045225036042));
#56274=CARTESIAN_POINT('Ctrl Pts',(1.78295981235902,-2.09034202746774,-32.3165923940998));
#56275=CARTESIAN_POINT('Ctrl Pts',(1.92217361622795,-2.10353486590704,-32.4807924448345));
#56276=CARTESIAN_POINT('Ctrl Pts',(1.54214210494487,-2.09550639469273,-32.8185779932545));
#56277=CARTESIAN_POINT('Ctrl Pts',(0.61600518091511,-2.06181102885638,-33.3002465007061));
#56278=CARTESIAN_POINT('Ctrl Pts',(-0.907207782595835,-2.0691118392714,
-33.2202856317455));
#56279=CARTESIAN_POINT('Ctrl Pts',(-2.22461176780362,-2.1206214736028,-32.3628055449923));
#56280=CARTESIAN_POINT('Ctrl Pts',(-3.00594215374136,-2.09423195572766,
-30.9643085677682));
#56281=CARTESIAN_POINT('Ctrl Pts',(-3.02268599780788,-2.05274388500329,
-29.9478114914885));
#56282=CARTESIAN_POINT('Ctrl Pts',(-2.84029263744146,-2.04183273360025,
-29.22012928383));
#56283=CARTESIAN_POINT('Ctrl Pts',(-2.64319201568411,-2.02946358499133,
-28.6985450532409));
#56284=CARTESIAN_POINT('Ctrl Pts',(-1.99960374430712,-1.99287484878532,
-27.8235216602912));
#56285=CARTESIAN_POINT('Ctrl Pts',(-0.816457589247531,-1.93849257916689,
-27.1049559716654));
#56286=CARTESIAN_POINT('Ctrl Pts',(0.817160570345912,-1.93883495609753,
-27.1081768085736));
#56287=CARTESIAN_POINT('Ctrl Pts',(1.88095619521476,-1.98740065419004,-27.7460109726621));
#56288=CARTESIAN_POINT('Ctrl Pts',(2.40323538999901,-2.01585893888295,-28.3714302885281));
#56289=CARTESIAN_POINT('Ctrl Pts',(2.61933802028281,-2.02845220565332,-28.7120950601187));
#56290=CARTESIAN_POINT('Ctrl Pts',(2.76258855495401,-2.0370663728381,-29.0211619117701));
#56291=CARTESIAN_POINT('Ctrl Pts',(2.85165863890266,-2.04253049221437,-29.2779504603529));
#56292=CARTESIAN_POINT('Ctrl Pts',(2.88755751178509,-2.04474699586185,-29.4088777844149));
#56293=CARTESIAN_POINT('Ctrl Pts',(2.95529437562388,-2.04895478990619,-29.690865199318));
#56294=CARTESIAN_POINT('Ctrl Pts',(3.01054093596492,-2.05929030439916,-30.1150007456908));
#56295=CARTESIAN_POINT('Ctrl Pts',(2.90557514872957,-2.09980733494611,-31.2138156516044));
#56296=CARTESIAN_POINT('Ctrl Pts',(2.42264063284103,-2.11410763399941,-32.0359595279482));
#56297=CARTESIAN_POINT('Ctrl Pts',(1.92217361622794,-2.10353486590704,-32.4807924448345));
#56298=CARTESIAN_POINT('',(1.32735269144094,-1.10555525796307,-31.754253126905));
#56299=CARTESIAN_POINT('Ctrl Pts',(1.92209690203547,-2.10352758862968,-32.4807019617002));
#56300=CARTESIAN_POINT('Ctrl Pts',(1.78290998961342,-2.09031072420672,-32.3165329245109));
#56301=CARTESIAN_POINT('Ctrl Pts',(1.46652846325438,-1.89151447256697,-31.9388921435421));
#56302=CARTESIAN_POINT('Ctrl Pts',(1.32359268837332,-1.3930284764443,-31.7574477757783));
#56303=CARTESIAN_POINT('Ctrl Pts',(1.32735269144094,-1.10555525796307,-31.754253126905));
#56304=CARTESIAN_POINT('',(-2.04999522160878,-1.06512573620563,-30.1923376809671));
#56305=CARTESIAN_POINT('Ctrl Pts',(1.32735269144094,-1.10555525796307,-31.754253126905));
#56306=CARTESIAN_POINT('Ctrl Pts',(1.06710073148761,-1.09683487190185,-31.975373592947));
#56307=CARTESIAN_POINT('Ctrl Pts',(0.428155187551756,-1.06165436373511,
-32.2864496159946));
#56308=CARTESIAN_POINT('Ctrl Pts',(-0.630282194184733,-1.0692102615866,
-32.2353219180946));
#56309=CARTESIAN_POINT('Ctrl Pts',(-1.53618081272622,-1.12324621261658,
-31.6799876467057));
#56310=CARTESIAN_POINT('Ctrl Pts',(-1.98079487593783,-1.10205821181136,
-30.8985237615705));
#56311=CARTESIAN_POINT('Ctrl Pts',(-2.05000335389775,-1.07367692784301,
-30.3739907004343));
#56312=CARTESIAN_POINT('Ctrl Pts',(-2.04999522160878,-1.06512573620563,
-30.1923376809671));
#56313=CARTESIAN_POINT('Ctrl Pts',(-2.04999522160878,-1.06512573620563,
-30.1923376809671));
#56314=CARTESIAN_POINT('Ctrl Pts',(-2.04998798795319,-1.05751946748649,
-30.0307576651865));
#56315=CARTESIAN_POINT('Ctrl Pts',(-2.03102354673217,-1.05091884457554,
-29.8690809921543));
#56316=CARTESIAN_POINT('Ctrl Pts',(-1.95022898432517,-1.04370742396877,
-29.5338952679768));
#56317=CARTESIAN_POINT('Ctrl Pts',(-1.81664117243763,-1.0312338635184,-29.1901382103174));
#56318=CARTESIAN_POINT('Ctrl Pts',(-1.37870319165073,-0.994208730015135,
-28.5976563596733));
#56319=CARTESIAN_POINT('Ctrl Pts',(-0.565632139754401,-0.938431810497882,
-28.1175164175936));
#56320=CARTESIAN_POINT('Ctrl Pts',(0.566051291595285,-0.938787274998903,
-28.1186849695365));
#56321=CARTESIAN_POINT('Ctrl Pts',(1.29716483238625,-0.988597635068523,
-28.5489950966502));
#56322=CARTESIAN_POINT('Ctrl Pts',(1.65332946690085,-1.01745671260863,-28.9696512040306));
#56323=CARTESIAN_POINT('Ctrl Pts',(1.80035161541673,-1.0302070446804,-29.1988189274931));
#56324=CARTESIAN_POINT('Ctrl Pts',(1.89755296929512,-1.0389008897144,-29.406736531242));
#56325=CARTESIAN_POINT('Ctrl Pts',(1.95792514729417,-1.04441107544017,-29.5794738833423));
#56326=CARTESIAN_POINT('Ctrl Pts',(1.98223924757779,-1.04664413680767,-29.6674728551243));
#56327=CARTESIAN_POINT('Ctrl Pts',(2.02810945191073,-1.0508832347292,-29.8577107402739));
#56328=CARTESIAN_POINT('Ctrl Pts',(2.06564184504211,-1.0616449129841,-30.159982754614));
#56329=CARTESIAN_POINT('Ctrl Pts',(1.99588940266396,-1.10355864373223,-30.9150513968238));
#56330=CARTESIAN_POINT('Ctrl Pts',(1.67008090765068,-1.11703921512503,-31.4630575374169));
#56331=CARTESIAN_POINT('Ctrl Pts',(1.32735269144094,-1.10555525796307,-31.754253126905));
#56332=CARTESIAN_POINT('Origin',(0.,-32.64,-30.192));
#56333=CARTESIAN_POINT('',(-2.04996075587217,1.01995056002153,-30.1919211569379));
#56334=CARTESIAN_POINT('',(-2.05,-32.64,-30.192));
#56335=CARTESIAN_POINT('',(1.11427248149542,0.985616400927087,-31.9127256716229));
#56336=CARTESIAN_POINT('Ctrl Pts',(1.11427248149542,0.985616400927087,-31.9127256716229));
#56337=CARTESIAN_POINT('Ctrl Pts',(1.39531085079306,0.975440411623561,-31.7307365688176));
#56338=CARTESIAN_POINT('Ctrl Pts',(1.99044683757195,0.965060884489212,-31.0938116474192));
#56339=CARTESIAN_POINT('Ctrl Pts',(2.11292571169222,1.02591892089202,-30.2033470929722));
#56340=CARTESIAN_POINT('Ctrl Pts',(1.94993402071046,1.04016458736943,-29.5342274298653));
#56341=CARTESIAN_POINT('Ctrl Pts',(1.81641479649524,1.0523146735164,-29.1904822889767));
#56342=CARTESIAN_POINT('Ctrl Pts',(1.37906269670218,1.08848337424274,-28.5984740900847));
#56343=CARTESIAN_POINT('Ctrl Pts',(0.564594594180929,1.14119196261678,-28.1173646277202));
#56344=CARTESIAN_POINT('Ctrl Pts',(-0.565690606478501,1.14128987332371,
-28.118282602635));
#56345=CARTESIAN_POINT('Ctrl Pts',(-1.54155256487553,1.0776718216566,-28.6932848560635));
#56346=CARTESIAN_POINT('Ctrl Pts',(-1.90806784508456,1.04384068155644,-29.3576617301976));
#56347=CARTESIAN_POINT('Ctrl Pts',(-2.03072544333898,1.03276938773931,-29.8679570181404));
#56348=CARTESIAN_POINT('Ctrl Pts',(-2.04987917115497,1.02693726153892,-30.0302127515688));
#56349=CARTESIAN_POINT('Ctrl Pts',(-2.04996075587217,1.01995056002153,-30.1919211569379));
#56350=CARTESIAN_POINT('Ctrl Pts',(-2.04999999848379,1.019950560016,-30.1919211555564));
#56351=CARTESIAN_POINT('Ctrl Pts',(-2.05000005380476,1.01988841535769,-30.1933595318955));
#56352=CARTESIAN_POINT('Ctrl Pts',(-2.0499985952739,1.01982617935423,-30.1947978635202));
#56353=CARTESIAN_POINT('Ctrl Pts',(-2.04999562318249,1.0197638529079,-30.1962361459661));
#56354=CARTESIAN_POINT('Ctrl Pts',(-2.04975068589453,1.01462737874599,-30.3147685035087));
#56355=CARTESIAN_POINT('Ctrl Pts',(-2.03922196734261,1.00887663384279,-30.4329535298336));
#56356=CARTESIAN_POINT('Ctrl Pts',(-2.01860478544297,1.00335286719046,-30.5493999443016));
#56357=CARTESIAN_POINT('Ctrl Pts',(-2.01084599258605,1.0012741271641,-30.593221821277));
#56358=CARTESIAN_POINT('Ctrl Pts',(-2.00165893224459,0.999227532176541,
-30.6367977614767));
#56359=CARTESIAN_POINT('Ctrl Pts',(-1.99105581950972,0.997257917428783,
-30.6800540170888));
#56360=CARTESIAN_POINT('Ctrl Pts',(-1.97431541280555,0.994148250225161,
-30.748347859619));
#56361=CARTESIAN_POINT('Ctrl Pts',(-1.9540381171472,0.991230469561293,-30.8158565688041));
#56362=CARTESIAN_POINT('Ctrl Pts',(-1.93032221771434,0.988582488966841,
-30.8821855806943));
#56363=CARTESIAN_POINT('Ctrl Pts',(-1.90661593400946,0.985935582009134,
-30.9484876991607));
#56364=CARTESIAN_POINT('Ctrl Pts',(-1.87947397032055,0.983558256381658,
-31.0136105978385));
#56365=CARTESIAN_POINT('Ctrl Pts',(-1.84904444368859,0.981528330881211,
-31.0771749235402));
#56366=CARTESIAN_POINT('Ctrl Pts',(-1.81862281036336,0.979498931935937,
-31.1407227608908));
#56367=CARTESIAN_POINT('Ctrl Pts',(-1.78491552685566,0.977816752912453,
-31.20271238098));
#56368=CARTESIAN_POINT('Ctrl Pts',(-1.74811795368169,0.976559552065531,
-31.2627864493053));
#56369=CARTESIAN_POINT('Ctrl Pts',(-1.71130007460099,0.975301657460817,
-31.3228936681435));
#56370=CARTESIAN_POINT('Ctrl Pts',(-1.67138876382225,0.974469210191225,
-31.3810828009535));
#56371=CARTESIAN_POINT('Ctrl Pts',(-1.62862354828288,0.974140097309977,
-31.4370242318841));
#56372=CARTESIAN_POINT('Ctrl Pts',(-1.6015032683714,0.973931384847071,-31.4725004301529));
#56373=CARTESIAN_POINT('Ctrl Pts',(-1.57323611092066,0.973925097132324,
-31.5070732670964));
#56374=CARTESIAN_POINT('Ctrl Pts',(-1.54389146947895,0.974141098580752,
-31.5406656852127));
#56375=CARTESIAN_POINT('Ctrl Pts',(-1.49368685948395,0.974510647089232,
-31.5981376517272));
#56376=CARTESIAN_POINT('Ctrl Pts',(-1.44029009238857,0.975530846253287,
-31.6527802833411));
#56377=CARTESIAN_POINT('Ctrl Pts',(-1.38403878501658,0.977004899514149,
-31.7042620942052));
#56378=CARTESIAN_POINT('Ctrl Pts',(-1.32772589645034,0.978480566496798,
-31.7558002648508));
#56379=CARTESIAN_POINT('Ctrl Pts',(-1.26855250415855,0.980411081834956,
-31.8041704474619));
#56380=CARTESIAN_POINT('Ctrl Pts',(-1.20689100633097,0.982599001932101,
-31.8490799916834));
#56381=CARTESIAN_POINT('Ctrl Pts',(-1.14520292035325,0.984787865450183,
-31.8940089006908));
#56382=CARTESIAN_POINT('Ctrl Pts',(-1.08102489983426,0.987234355758579,
-31.9354739805255));
#56383=CARTESIAN_POINT('Ctrl Pts',(-1.01475894042778,0.98974077374038,-31.9732255030798));
#56384=CARTESIAN_POINT('Ctrl Pts',(-0.948445088105803,0.992249003205265,
-32.0110043100874));
#56385=CARTESIAN_POINT('Ctrl Pts',(-0.880040613676623,0.994817246998847,
-32.0450640170226));
#56386=CARTESIAN_POINT('Ctrl Pts',(-0.809972632927784,0.997247377040431,
-32.0752005559441));
#56387=CARTESIAN_POINT('Ctrl Pts',(-0.791398111670701,0.997891587157983,
-32.083189537171));
#56388=CARTESIAN_POINT('Ctrl Pts',(-0.772706805174443,0.998526091438893,
-32.0909030798375));
#56389=CARTESIAN_POINT('Ctrl Pts',(-0.753906908629067,0.999147198916575,
-32.0983379482981));
#56390=CARTESIAN_POINT('Ctrl Pts',(-0.67836183054658,1.00164304312433,-32.128214055171));
#56391=CARTESIAN_POINT('Ctrl Pts',(-0.601050728001295,1.00392256437619,
-32.1535899336801));
#56392=CARTESIAN_POINT('Ctrl Pts',(-0.522511154750602,1.00588453382231,
-32.1742921311354));
#56393=CARTESIAN_POINT('Ctrl Pts',(-0.447881594202448,1.0077488286168,-32.1939636907648));
#56394=CARTESIAN_POINT('Ctrl Pts',(-0.372143322601374,1.00932640255769,
-32.209415691935));
#56395=CARTESIAN_POINT('Ctrl Pts',(-0.295771013314592,1.01053040534075,
-32.2205510857957));
#56396=CARTESIAN_POINT('Ctrl Pts',(-0.219414607426094,1.01173415740812,
-32.2316841608761));
#56397=CARTESIAN_POINT('Ctrl Pts',(-0.142424777405172,1.01256449388275,
-32.2385023728595));
#56398=CARTESIAN_POINT('Ctrl Pts',(-0.0652837489749921,1.012934618705,-32.2409602319518));
#56399=CARTESIAN_POINT('Ctrl Pts',(0.0118274848913055,1.01330460057211,
-32.2434171417328));
#56400=CARTESIAN_POINT('Ctrl Pts',(0.0890894474301462,1.01321472621786,
-32.241517046982));
#56401=CARTESIAN_POINT('Ctrl Pts',(0.16601789719275,1.0125783001148,-32.2352665165885));
#56402=CARTESIAN_POINT('Ctrl Pts',(0.178178240097014,1.01247769806614,-32.2342784738923));
#56403=CARTESIAN_POINT('Ctrl Pts',(0.190330250549795,1.01236343921683,-32.2331818318135));
#56404=CARTESIAN_POINT('Ctrl Pts',(0.202472019062823,1.01223518113576,-32.2319767355283));
#56405=CARTESIAN_POINT('Ctrl Pts',(0.27220735997383,1.01149854042331,-32.2250553549908));
#56406=CARTESIAN_POINT('Ctrl Pts',(0.341638885368904,1.0103001079684,-32.2145487493329));
#56407=CARTESIAN_POINT('Ctrl Pts',(0.410365860739164,1.00877460508166,-32.2005068733614));
#56408=CARTESIAN_POINT('Ctrl Pts',(0.479101969682676,1.00724889946096,-32.1864631312739));
#56409=CARTESIAN_POINT('Ctrl Pts',(0.547132845704916,1.00539603646965,-32.1688832655349));
#56410=CARTESIAN_POINT('Ctrl Pts',(0.614066975647822,1.00335079113749,-32.1478685409349));
#56411=CARTESIAN_POINT('Ctrl Pts',(0.68100394653689,1.00130545899712,-32.1268529243878));
#56412=CARTESIAN_POINT('Ctrl Pts',(0.746843602335305,0.999067728184644,
-32.1024023210015));
#56413=CARTESIAN_POINT('Ctrl Pts',(0.811211060810975,0.996772390891678,
-32.0746674201297));
#56414=CARTESIAN_POINT('Ctrl Pts',(0.875645346513367,0.994474670546324,
-32.0469037244826));
#56415=CARTESIAN_POINT('Ctrl Pts',(0.938603927258259,0.992119224042631,
-32.0158491368998));
#56416=CARTESIAN_POINT('Ctrl Pts',(0.999734427064827,0.989841263837853,
-31.9817013927863));
#56417=CARTESIAN_POINT('Ctrl Pts',(1.0386837119197,0.98838986198142,-31.9599441649404));
#56418=CARTESIAN_POINT('Ctrl Pts',(1.07689136950961,0.986969916451226,-31.9369321707182));
#56419=CARTESIAN_POINT('Ctrl Pts',(1.11427248149541,0.985616400927093,-31.9127256716229));
#56420=CARTESIAN_POINT('Ctrl Pts',(1.11427248149542,0.985616400927087,-31.9127256716229));
#56421=CARTESIAN_POINT('Ctrl Pts',(1.39531085079306,0.975440411623561,-31.7307365688176));
#56422=CARTESIAN_POINT('Ctrl Pts',(1.99044683757195,0.965060884489212,-31.0938116474192));
#56423=CARTESIAN_POINT('Ctrl Pts',(2.11292571169222,1.02591892089202,-30.2033470929722));
#56424=CARTESIAN_POINT('Ctrl Pts',(1.94993402071046,1.04016458736943,-29.5342274298653));
#56425=CARTESIAN_POINT('Ctrl Pts',(1.81641479649524,1.0523146735164,-29.1904822889767));
#56426=CARTESIAN_POINT('Ctrl Pts',(1.37906269670218,1.08848337424274,-28.5984740900847));
#56427=CARTESIAN_POINT('Ctrl Pts',(0.564594594180929,1.14119196261678,-28.1173646277202));
#56428=CARTESIAN_POINT('Ctrl Pts',(-0.565690606478501,1.14128987332371,
-28.118282602635));
#56429=CARTESIAN_POINT('Ctrl Pts',(-1.54155256487553,1.0776718216566,-28.6932848560635));
#56430=CARTESIAN_POINT('Ctrl Pts',(-1.90806784508456,1.04384068155644,-29.3576617301976));
#56431=CARTESIAN_POINT('Ctrl Pts',(-2.03106003574106,1.0327391868317,-29.8693490307722));
#56432=CARTESIAN_POINT('Ctrl Pts',(-2.06937685224897,1.02092745047005,-30.1968502518399));
#56433=CARTESIAN_POINT('Ctrl Pts',(-1.99066291316253,0.987995197249567,
-30.8469392317313));
#56434=CARTESIAN_POINT('Ctrl Pts',(-1.60389855123596,0.962274733835357,
-31.594329399779));
#56435=CARTESIAN_POINT('Ctrl Pts',(-0.782446503162938,1.00260836621067,
-32.1715806038486));
#56436=CARTESIAN_POINT('Ctrl Pts',(0.209646108503345,1.02217499482138,-32.310885465022));
#56437=CARTESIAN_POINT('Ctrl Pts',(0.842409601437768,0.995460159152721,
-32.0887730979989));
#56438=CARTESIAN_POINT('Ctrl Pts',(1.11427248149542,0.985616400927087,-31.9127256716229));
#56439=CARTESIAN_POINT('Ctrl Pts',(1.11956381130215,1.29420809400475,-31.9092992200441));
#56440=CARTESIAN_POINT('Ctrl Pts',(1.39818435418416,1.28711878983686,-31.7274836751049));
#56441=CARTESIAN_POINT('Ctrl Pts',(1.98135604782,1.28207482701826,-31.1022476003622));
#56442=CARTESIAN_POINT('Ctrl Pts',(2.1128795676757,1.33532002180968,-30.2176795236496));
#56443=CARTESIAN_POINT('Ctrl Pts',(1.94985285160701,1.35063254955861,-29.5389616589331));
#56444=CARTESIAN_POINT('Ctrl Pts',(1.81913793522182,1.3612658092768,-29.1996370764735));
#56445=CARTESIAN_POINT('Ctrl Pts',(1.38765007217341,1.3937566224756,-28.6077703469072));
#56446=CARTESIAN_POINT('Ctrl Pts',(0.573031934016957,1.4401444299264,-28.1188124687556));
#56447=CARTESIAN_POINT('Ctrl Pts',(-0.57399177348583,1.44023865387881,-28.1195341194796));
#56448=CARTESIAN_POINT('Ctrl Pts',(-1.55039175852058,1.38391592875038,-28.7058296242747));
#56449=CARTESIAN_POINT('Ctrl Pts',(-1.9095164692758,1.35344936800592,-29.3666716185023));
#56450=CARTESIAN_POINT('Ctrl Pts',(-2.03050637137044,1.34331472964374,-29.8743021354302));
#56451=CARTESIAN_POINT('Ctrl Pts',(-2.06837339171471,1.3316298126124,-30.2064485213252));
#56452=CARTESIAN_POINT('Ctrl Pts',(-1.98506648137687,1.30187139856525,-30.8552545286718));
#56453=CARTESIAN_POINT('Ctrl Pts',(-1.60212643522416,1.27750805182646,-31.5889934734217));
#56454=CARTESIAN_POINT('Ctrl Pts',(-0.792039056601329,1.30634155677681,
-32.1675382972107));
#56455=CARTESIAN_POINT('Ctrl Pts',(0.213298425973278,1.32138237766697,-32.3124702863081));
#56456=CARTESIAN_POINT('Ctrl Pts',(0.850039819185237,1.3010659428227,-32.085178754963));
#56457=CARTESIAN_POINT('Ctrl Pts',(1.11956381130215,1.29420809400475,-31.9092992200441));
#56458=CARTESIAN_POINT('Ctrl Pts',(1.27454163485273,1.8276996776529,-32.1285752398414));
#56459=CARTESIAN_POINT('Ctrl Pts',(1.59048771051817,1.82546583320247,-31.9272465850611));
#56460=CARTESIAN_POINT('Ctrl Pts',(2.24506867253542,1.82887441364011,-31.2405221593139));
#56461=CARTESIAN_POINT('Ctrl Pts',(2.39580868742134,1.87009241788133,-30.2391853142947));
#56462=CARTESIAN_POINT('Ctrl Pts',(2.21207475359764,1.88703580700542,-29.456927089891));
#56463=CARTESIAN_POINT('Ctrl Pts',(2.06558631312181,1.89524681774927,-29.0798299199868));
#56464=CARTESIAN_POINT('Ctrl Pts',(1.57974170165877,1.92187683611202,-28.4135771845243));
#56465=CARTESIAN_POINT('Ctrl Pts',(0.655063819144604,1.95814863714053,-27.8622104435215));
#56466=CARTESIAN_POINT('Ctrl Pts',(-0.65717394110681,1.95823512688616,-27.8629454348409));
#56467=CARTESIAN_POINT('Ctrl Pts',(-1.76474453532705,1.91360863385461,-28.527769477946));
#56468=CARTESIAN_POINT('Ctrl Pts',(-2.16726287994011,1.88851922966795,-29.2691704704899));
#56469=CARTESIAN_POINT('Ctrl Pts',(-2.30281338888132,1.87995898954312,-29.8386330483677));
#56470=CARTESIAN_POINT('Ctrl Pts',(-2.34544045465379,1.86847127655649,-30.2231880710558));
#56471=CARTESIAN_POINT('Ctrl Pts',(-2.25007163104386,1.84369961096044,-30.9597522307304));
#56472=CARTESIAN_POINT('Ctrl Pts',(-1.82100012358539,1.82146628356056,-31.7765943544781));
#56473=CARTESIAN_POINT('Ctrl Pts',(-0.906777259631241,1.83213318063528,
-32.4148810720433));
#56474=CARTESIAN_POINT('Ctrl Pts',(0.244785644071488,1.8398977864338,-32.5765442393965));
#56475=CARTESIAN_POINT('Ctrl Pts',(0.968910733677276,1.82986059036888,-32.3233308102765));
#56476=CARTESIAN_POINT('Ctrl Pts',(1.27454163485273,1.8276996776529,-32.1285752398414));
#56477=CARTESIAN_POINT('Ctrl Pts',(1.57644208397091,1.99566187679991,-32.5884753902851));
#56478=CARTESIAN_POINT('Ctrl Pts',(1.97100507309382,1.9885807024151,-32.345177614523));
#56479=CARTESIAN_POINT('Ctrl Pts',(2.79658360538242,1.98287648602251,-31.4952486579893));
#56480=CARTESIAN_POINT('Ctrl Pts',(2.96667415068578,2.03643433013976,-30.2472423249499));
#56481=CARTESIAN_POINT('Ctrl Pts',(2.74056010357048,2.05208677514991,-29.2806260191735));
#56482=CARTESIAN_POINT('Ctrl Pts',(2.55597801423823,2.06256996690073,-28.8141728220434));
#56483=CARTESIAN_POINT('Ctrl Pts',(1.94794652960207,2.09483464954365,-27.9954419169136));
#56484=CARTESIAN_POINT('Ctrl Pts',(0.802279448537956,2.14101584746524,-27.3312746370507));
#56485=CARTESIAN_POINT('Ctrl Pts',(-0.80422250876151,2.14111565459134,-27.3323492148327));
#56486=CARTESIAN_POINT('Ctrl Pts',(-2.17661844051394,2.08500434760299,-28.1331664227393));
#56487=CARTESIAN_POINT('Ctrl Pts',(-2.68307713098919,2.05482231865599,-29.0481824505078));
#56488=CARTESIAN_POINT('Ctrl Pts',(-2.85317444361622,2.04476692737883,-29.7536088239151));
#56489=CARTESIAN_POINT('Ctrl Pts',(-2.90642449768279,2.03282840777432,-30.22927942631));
#56490=CARTESIAN_POINT('Ctrl Pts',(-2.79629611681264,2.00277800636097,-31.1428048397418));
#56491=CARTESIAN_POINT('Ctrl Pts',(-2.26248035166364,1.97897801598921,-32.1646758668128));
#56492=CARTESIAN_POINT('Ctrl Pts',(-1.11307220412048,2.00775834857362,-32.9330684865351));
#56493=CARTESIAN_POINT('Ctrl Pts',(0.299068585902303,2.02244161902527,-33.1194515816353));
#56494=CARTESIAN_POINT('Ctrl Pts',(1.19476099588608,2.00251186126023,-32.823829851655));
#56495=CARTESIAN_POINT('Ctrl Pts',(1.57644208397091,1.99566187679991,-32.5884753902851));
#56496=CARTESIAN_POINT('Ctrl Pts',(1.7019170311789,1.9841758627661,-32.7826729204701));
#56497=CARTESIAN_POINT('Ctrl Pts',(2.12920577407486,1.97332831724216,-32.5206340925411));
#56498=CARTESIAN_POINT('Ctrl Pts',(3.02661590274896,1.96081108314947,-31.598486221152));
#56499=CARTESIAN_POINT('Ctrl Pts',(3.20555263301232,2.02375902210562,-30.2475171721583));
#56500=CARTESIAN_POINT('Ctrl Pts',(2.96141616799977,2.03832498497809,-29.2059464506088));
#56501=CARTESIAN_POINT('Ctrl Pts',(2.76077187221957,2.05058763177432,-28.7007479940497));
#56502=CARTESIAN_POINT('Ctrl Pts',(2.10137698734444,2.08724640507052,-27.8170592929481));
#56503=CARTESIAN_POINT('Ctrl Pts',(0.863471086326564,2.14121820993117,-27.1043323065609));
#56504=CARTESIAN_POINT('Ctrl Pts',(-0.86527131205636,2.14132533286026,-27.1055607008419));
#56505=CARTESIAN_POINT('Ctrl Pts',(-2.34826718848484,2.07619929406285,-27.9643060633081));
#56506=CARTESIAN_POINT('Ctrl Pts',(-2.89858207601554,2.04205880766061,-28.953501894721));
#56507=CARTESIAN_POINT('Ctrl Pts',(-3.08328115399646,2.03085086602267,-29.7168832273726));
#56508=CARTESIAN_POINT('Ctrl Pts',(-3.14100419297298,2.01861532274412,-30.2293427451567));
#56509=CARTESIAN_POINT('Ctrl Pts',(-3.02438609187982,1.98457308078909,-31.2166546642125));
#56510=CARTESIAN_POINT('Ctrl Pts',(-2.44599217953573,1.95940735428246,-32.3264040160697));
#56511=CARTESIAN_POINT('Ctrl Pts',(-1.19853457360234,2.00220690733558,-33.1534394779125));
#56512=CARTESIAN_POINT('Ctrl Pts',(0.321543600862733,2.02241016559728,-33.3511773448253));
#56513=CARTESIAN_POINT('Ctrl Pts',(1.28857863702931,1.99466925188967,-33.036156566229));
#56514=CARTESIAN_POINT('Ctrl Pts',(1.7019170311789,1.9841758627661,-32.7826729204701));
#56515=CARTESIAN_POINT('Ctrl Pts',(1.7019170311789,1.9841758627661,-32.7826729204701));
#56516=CARTESIAN_POINT('Ctrl Pts',(1.57644208397091,1.99566187679991,-32.5884753902851));
#56517=CARTESIAN_POINT('Ctrl Pts',(1.27454163485273,1.8276996776529,-32.1285752398414));
#56518=CARTESIAN_POINT('Ctrl Pts',(1.11956381130215,1.29420809400475,-31.9092992200441));
#56519=CARTESIAN_POINT('Ctrl Pts',(1.11427248149542,0.985616400927087,-31.9127256716229));
#56520=CARTESIAN_POINT('Ctrl Pts',(-2.6112,-1.7952,-17.9847266586119));
#56521=CARTESIAN_POINT('Ctrl Pts',(-2.6112,-1.7952,-17.8038186312799));
#56522=CARTESIAN_POINT('Ctrl Pts',(-2.6112,-1.7952,-17.6229797056178));
#56523=CARTESIAN_POINT('Ctrl Pts',(-2.61120000000001,-1.7952,-15.4299462974754));
#56524=CARTESIAN_POINT('Ctrl Pts',(-2.61119999999997,-1.79520000000006,
-13.4283436818382));
#56525=CARTESIAN_POINT('Ctrl Pts',(-2.6112,-1.7952,-11.3982797880253));
#56526=CARTESIAN_POINT('Ctrl Pts',(-2.6112,-1.7952,-11.3949488097292));
#56527=CARTESIAN_POINT('Ctrl Pts',(-2.6112,-1.7952,-11.3916190672592));
#56528=CARTESIAN_POINT('Ctrl Pts',(-2.77989728120026,-1.95404468986484,
-17.9847305491976));
#56529=CARTESIAN_POINT('Ctrl Pts',(-2.77989657069797,-1.95404498366009,
-17.8038217156034));
#56530=CARTESIAN_POINT('Ctrl Pts',(-2.77989885548672,-1.95404480761269,
-17.6228745058655));
#56531=CARTESIAN_POINT('Ctrl Pts',(-2.77986360351872,-1.95404717491004,
-15.4319102613121));
#56532=CARTESIAN_POINT('Ctrl Pts',(-2.78490918456105,-1.9809296830024,-13.4264720521715));
#56533=CARTESIAN_POINT('Ctrl Pts',(-2.77977307325551,-1.95384830245126,
-11.3904949845565));
#56534=CARTESIAN_POINT('Ctrl Pts',(-2.77976473793328,-1.95380467400608,
-11.3872330515971));
#56535=CARTESIAN_POINT('Ctrl Pts',(-2.77975642964883,-1.95376115846772,
-11.3839397041863));
#56536=CARTESIAN_POINT('Ctrl Pts',(-3.00527959091536,-2.05140295765447,
-17.9847344249878));
#56537=CARTESIAN_POINT('Ctrl Pts',(-3.00527820077576,-2.0514038959004,-17.80382478864));
#56538=CARTESIAN_POINT('Ctrl Pts',(-3.00528063959888,-2.05140328438882,
-17.6227699131191));
#56539=CARTESIAN_POINT('Ctrl Pts',(-3.00524011522215,-2.05141620495531,
-15.433862968178));
#56540=CARTESIAN_POINT('Ctrl Pts',(-3.03079562252321,-2.09655587208129,
-13.4246144926598));
#56541=CARTESIAN_POINT('Ctrl Pts',(-3.00496931991195,-2.05104808335724,
-11.3827398048443));
#56542=CARTESIAN_POINT('Ctrl Pts',(-3.00492672599342,-2.05097607451537,
-11.3795465922533));
#56543=CARTESIAN_POINT('Ctrl Pts',(-3.00488462572301,-2.05090371235558,
-11.376289460898));
#56544=CARTESIAN_POINT('Ctrl Pts',(-3.2365718826939,-2.06534153551084,-17.9847374128284));
#56545=CARTESIAN_POINT('Ctrl Pts',(-3.23657012621139,-2.06534337873604,
-17.8038271587737));
#56546=CARTESIAN_POINT('Ctrl Pts',(-3.23657277689822,-2.06534385547269,
-17.6226933437992));
#56547=CARTESIAN_POINT('Ctrl Pts',(-3.23652783128775,-2.06535065050216,
-15.4352998782646));
#56548=CARTESIAN_POINT('Ctrl Pts',(-3.28422590292882,-2.11198472512398,
-13.4234076931397));
#56549=CARTESIAN_POINT('Ctrl Pts',(-3.2360940577226,-2.06491840819467,-11.3767602403348));
#56550=CARTESIAN_POINT('Ctrl Pts',(-3.23601450622251,-2.06484630497268,
-11.3736192543818));
#56551=CARTESIAN_POINT('Ctrl Pts',(-3.23593596401738,-2.06477283942456,
-11.3703894647525));
#56552=CARTESIAN_POINT('',(-2.6112,-1.7952,-12.0768));
#56553=CARTESIAN_POINT('Ctrl Pts',(-3.23593596335381,-2.06477283939948,
-11.3703894654624));
#56554=CARTESIAN_POINT('Ctrl Pts',(-3.23474911227318,-2.06472795379312,
-11.3716587203814));
#56555=CARTESIAN_POINT('Ctrl Pts',(-3.23356208451618,-2.06468080653982,
-11.3729279078231));
#56556=CARTESIAN_POINT('Ctrl Pts',(-3.21770668024123,-2.06402110482042,
-11.3898827330855));
#56557=CARTESIAN_POINT('Ctrl Pts',(-3.20326350624142,-2.06308054430746,
-11.4057713990633));
#56558=CARTESIAN_POINT('Ctrl Pts',(-3.17469796288973,-2.0605365195,-11.4371598604922));
#56559=CARTESIAN_POINT('Ctrl Pts',(-3.16053710931684,-2.05894031541534,
-11.4527727770445));
#56560=CARTESIAN_POINT('Ctrl Pts',(-3.11874262004929,-2.05324512177431,
-11.4989707101412));
#56561=CARTESIAN_POINT('Ctrl Pts',(-3.09119467476536,-2.04821009397366,
-11.5295815571663));
#56562=CARTESIAN_POINT('Ctrl Pts',(-3.01139845824404,-2.02988905583392,
-11.6185972772731));
#56563=CARTESIAN_POINT('Ctrl Pts',(-2.95944916080578,-2.01321064940806,
-11.6770218573854));
#56564=CARTESIAN_POINT('Ctrl Pts',(-2.80388238880711,-1.94794876530532,
-11.8532974877227));
#56565=CARTESIAN_POINT('Ctrl Pts',(-2.7010964672983,-1.88292076974793,-11.9716088406924));
#56566=CARTESIAN_POINT('Ctrl Pts',(-2.61119999999998,-1.79520000000001,
-12.0768));
#56567=CARTESIAN_POINT('',(-2.6112,-1.7952,-17.2992));
#56568=CARTESIAN_POINT('Ctrl Pts',(-2.6112,-1.7952,-17.2992));
#56569=CARTESIAN_POINT('Ctrl Pts',(-2.70186167676372,-1.88058822619405,
-17.4015213914483));
#56570=CARTESIAN_POINT('Ctrl Pts',(-2.80486101159827,-1.94451507288388,
-17.5160105710852));
#56571=CARTESIAN_POINT('Ctrl Pts',(-3.01370491385484,-2.03227186506088,
-17.7451334738264));
#56572=CARTESIAN_POINT('Ctrl Pts',(-3.12339555017824,-2.05811702770554,
-17.8639679791454));
#56573=CARTESIAN_POINT('Ctrl Pts',(-3.23424858100826,-2.06519943732415,
-17.9822588144596));
#56574=CARTESIAN_POINT('Ctrl Pts',(-3.23541015404723,-2.06527153855177,
-17.983498128713));
#56575=CARTESIAN_POINT('Ctrl Pts',(-3.23657188269389,-2.06534153551084,
-17.9847374128283));
#56576=CARTESIAN_POINT('',(-2.6112,-1.7952,-17.2992));
#56577=CARTESIAN_POINT('Ctrl Pts',(3.29672665861269,-1.7952,-17.2992));
#56578=CARTESIAN_POINT('Ctrl Pts',(2.35555773128068,-1.7952,-17.2992));
#56579=CARTESIAN_POINT('Ctrl Pts',(0.157077029037056,-1.7952,-17.2992));
#56580=CARTESIAN_POINT('Ctrl Pts',(-2.04159461806908,-1.7952,-17.2992));
#56581=CARTESIAN_POINT('Ctrl Pts',(-3.29672665861176,-1.7952,-17.2992));
#56582=CARTESIAN_POINT('Ctrl Pts',(3.27462222013899,-1.9675756217075,-17.4822674903391));
#56583=CARTESIAN_POINT('Ctrl Pts',(2.33444703225756,-1.93319533298188,-17.4767078287549));
#56584=CARTESIAN_POINT('Ctrl Pts',(0.154267744829852,-1.85615680163965,
-17.4367287277564));
#56585=CARTESIAN_POINT('Ctrl Pts',(-2.0208154190802,-1.92172646467574,-17.4748531896899));
#56586=CARTESIAN_POINT('Ctrl Pts',(-3.27462222013808,-1.96757562170745,
-17.4822674903391));
#56587=CARTESIAN_POINT('Ctrl Pts',(3.25263565790317,-2.06631231538414,-17.7328313194308));
#56588=CARTESIAN_POINT('Ctrl Pts',(2.31339000270371,-2.00929176274259,-17.7003376499762));
#56589=CARTESIAN_POINT('Ctrl Pts',(0.151449899736544,-1.88860291849517,
-17.5858308525659));
#56590=CARTESIAN_POINT('Ctrl Pts',(-2.00006847092217,-1.99027036317821,
-17.6894981361277));
#56591=CARTESIAN_POINT('Ctrl Pts',(-3.25263565790227,-2.06631231538406,
-17.7328313194307));
#56592=CARTESIAN_POINT('Ctrl Pts',(3.2365718826948,-2.06534153551092,-17.9847374128284));
#56593=CARTESIAN_POINT('Ctrl Pts',(2.29676905143962,-2.00870599133178,-17.924480085149));
#56594=CARTESIAN_POINT('Ctrl Pts',(0.14883959757836,-1.89016258129227,-17.7348933106489));
#56595=CARTESIAN_POINT('Ctrl Pts',(-1.98326165214378,-1.9898130261557,-17.9043789347151));
#56596=CARTESIAN_POINT('Ctrl Pts',(-3.23657188269391,-2.06534153551084,
-17.9847374128283));
#56597=CARTESIAN_POINT('',(2.6112,-1.7952,-17.2992));
#56598=CARTESIAN_POINT('Ctrl Pts',(2.6112,-1.7952,-17.2992));
#56599=CARTESIAN_POINT('Ctrl Pts',(2.70179483356098,-1.88052135230686,-17.4014820850961));
#56600=CARTESIAN_POINT('Ctrl Pts',(2.80470828086409,-1.94441882305696,-17.5159947338438));
#56601=CARTESIAN_POINT('Ctrl Pts',(3.01348181545287,-2.03220905700659,-17.7451259671429));
#56602=CARTESIAN_POINT('Ctrl Pts',(3.12325136755414,-2.05810707767854,-17.8640229733036));
#56603=CARTESIAN_POINT('Ctrl Pts',(3.23424428254041,-2.06519917044408,-17.9822585773976));
#56604=CARTESIAN_POINT('Ctrl Pts',(3.23540799956588,-2.06527140871556,-17.9834980150053));
#56605=CARTESIAN_POINT('Ctrl Pts',(3.23657188269388,-2.06534153551087,-17.9847374128284));
#56606=CARTESIAN_POINT('',(2.6112,-1.7952,-17.2992));
#56607=CARTESIAN_POINT('Ctrl Pts',(2.6112,-1.7952,-11.3916190672592));
#56608=CARTESIAN_POINT('Ctrl Pts',(2.6112,-1.7952,-11.3949488317952));
#56609=CARTESIAN_POINT('Ctrl Pts',(2.6112,-1.7952,-11.3982785791877));
#56610=CARTESIAN_POINT('Ctrl Pts',(2.61119999999999,-1.7952,-11.602832033445));
#56611=CARTESIAN_POINT('Ctrl Pts',(2.6112,-1.7952,-12.0053665520704));
#56612=CARTESIAN_POINT('Ctrl Pts',(2.6112,-1.7952,-12.6092595592021));
#56613=CARTESIAN_POINT('Ctrl Pts',(2.6112,-1.7952,-13.2132104845282));
#56614=CARTESIAN_POINT('Ctrl Pts',(2.6112,-1.7952,-13.817202001388));
#56615=CARTESIAN_POINT('Ctrl Pts',(2.6112,-1.7952,-14.4211425787327));
#56616=CARTESIAN_POINT('Ctrl Pts',(2.6112,-1.7952,-15.0251107188001));
#56617=CARTESIAN_POINT('Ctrl Pts',(2.6112,-1.7952,-15.6291801268932));
#56618=CARTESIAN_POINT('Ctrl Pts',(2.6112,-1.7952,-16.2333316263011));
#56619=CARTESIAN_POINT('Ctrl Pts',(2.6112,-1.7952,-16.8375946102639));
#56620=CARTESIAN_POINT('Ctrl Pts',(2.6112,-1.7952,-17.2405176643803));
#56621=CARTESIAN_POINT('Ctrl Pts',(2.6112,-1.7952,-17.6229032948673));
#56622=CARTESIAN_POINT('Ctrl Pts',(2.6112,-1.7952,-17.8038125599604));
#56623=CARTESIAN_POINT('Ctrl Pts',(2.6112,-1.7952,-17.9847266586118));
#56624=CARTESIAN_POINT('Ctrl Pts',(2.77975642964883,-1.95376115846772,-11.3839397041863));
#56625=CARTESIAN_POINT('Ctrl Pts',(2.77976473798834,-1.95380467429445,-11.387233073422));
#56626=CARTESIAN_POINT('Ctrl Pts',(2.77977307189872,-1.95384850217605,-11.3905252176229));
#56627=CARTESIAN_POINT('Ctrl Pts',(2.78029059422271,-1.95655831630512,-11.5929254382172));
#56628=CARTESIAN_POINT('Ctrl Pts',(2.78108092408054,-1.96087507413405,-11.9996813082198));
#56629=CARTESIAN_POINT('Ctrl Pts',(2.78166904335597,-1.96461218616667,-12.6052412508096));
#56630=CARTESIAN_POINT('Ctrl Pts',(2.78190434852498,-1.96611094161964,-13.2119111458807));
#56631=CARTESIAN_POINT('Ctrl Pts',(2.78187541204246,-1.96583132347523,-13.817493293962));
#56632=CARTESIAN_POINT('Ctrl Pts',(2.78165383672433,-1.96424923733261,-14.4226530410535));
#56633=CARTESIAN_POINT('Ctrl Pts',(2.78128602574335,-1.96184656545489,-15.02729567872));
#56634=CARTESIAN_POINT('Ctrl Pts',(2.78083334812767,-1.95910495087451,-15.6315963053697));
#56635=CARTESIAN_POINT('Ctrl Pts',(2.78037226762904,-1.95651735366381,-16.2354433429288));
#56636=CARTESIAN_POINT('Ctrl Pts',(2.78000529832649,-1.9545750332871,-16.8389564677654));
#56637=CARTESIAN_POINT('Ctrl Pts',(2.77989762673263,-1.95404171479014,-17.2410103818547));
#56638=CARTESIAN_POINT('Ctrl Pts',(2.77989674977132,-1.95404389310532,-17.6226204503694));
#56639=CARTESIAN_POINT('Ctrl Pts',(2.77989657067412,-1.95404498366996,-17.8038156442568));
#56640=CARTESIAN_POINT('Ctrl Pts',(2.77989728120025,-1.95404468986484,-17.9847305491976));
#56641=CARTESIAN_POINT('Ctrl Pts',(3.00488462572301,-2.05090371235558,-11.376289460898));
#56642=CARTESIAN_POINT('Ctrl Pts',(3.00492672627241,-2.05097607499491,-11.3795466138381));
#56643=CARTESIAN_POINT('Ctrl Pts',(3.00496909004423,-2.05104893207522,-11.3828013386179));
#56644=CARTESIAN_POINT('Ctrl Pts',(3.00759032329905,-2.05555770794966,-11.583059109221));
#56645=CARTESIAN_POINT('Ctrl Pts',(3.01162939612273,-2.06287948227701,-11.994019831593));
#56646=CARTESIAN_POINT('Ctrl Pts',(3.01502559244183,-2.06919068355675,-12.6012395611528));
#56647=CARTESIAN_POINT('Ctrl Pts',(3.01638025343442,-2.07174063869622,-13.210615927018));
#56648=CARTESIAN_POINT('Ctrl Pts',(3.01615487636255,-2.07126503359285,-13.8177813034702));
#56649=CARTESIAN_POINT('Ctrl Pts',(3.01476443826533,-2.0685876908235,-14.4241546208859));
#56650=CARTESIAN_POINT('Ctrl Pts',(3.01260262607997,-2.06452689158505,-15.0294692549031));
#56651=CARTESIAN_POINT('Ctrl Pts',(3.01008433904802,-2.05990604728973,-15.6340008239812));
#56652=CARTESIAN_POINT('Ctrl Pts',(3.00765552944531,-2.05555450697557,-16.2375454125361));
#56653=CARTESIAN_POINT('Ctrl Pts',(3.00579999024632,-2.05229554923455,-16.8403123323523));
#56654=CARTESIAN_POINT('Ctrl Pts',(3.00527820611931,-2.051400250927,-17.2415009376399));
#56655=CARTESIAN_POINT('Ctrl Pts',(3.00527780370662,-2.05140286172455,-17.6223388317464));
#56656=CARTESIAN_POINT('Ctrl Pts',(3.0052782007291,-2.05140389593189,-17.8038187172666));
#56657=CARTESIAN_POINT('Ctrl Pts',(3.00527959091535,-2.05140295765448,-17.9847344249877));
#56658=CARTESIAN_POINT('Ctrl Pts',(3.23593596401738,-2.06477283942456,-11.3703894647525));
#56659=CARTESIAN_POINT('Ctrl Pts',(3.23601450674301,-2.06484630545954,-11.3736192757854));
#56660=CARTESIAN_POINT('Ctrl Pts',(3.2360935773066,-2.06492021722567,-11.3768457420933));
#56661=CARTESIAN_POINT('Ctrl Pts',(3.24098309020377,-2.06950210825037,-11.5754888699177));
#56662=CARTESIAN_POINT('Ctrl Pts',(3.24852404096208,-2.07718177263222,-11.9897144106618));
#56663=CARTESIAN_POINT('Ctrl Pts',(3.25495835163609,-2.0836979792605,-12.5981980422748));
#56664=CARTESIAN_POINT('Ctrl Pts',(3.25752083357516,-2.08636008311531,-13.2096246578577));
#56665=CARTESIAN_POINT('Ctrl Pts',(3.25707692954116,-2.08586417392827,-13.8179806012891));
#56666=CARTESIAN_POINT('Ctrl Pts',(3.25441336551011,-2.08309603063915,-14.42527398279));
#56667=CARTESIAN_POINT('Ctrl Pts',(3.25030484001515,-2.07889552730337,-15.0311078760445));
#56668=CARTESIAN_POINT('Ctrl Pts',(3.24554996678201,-2.07412283442935,-15.6358291186907));
#56669=CARTESIAN_POINT('Ctrl Pts',(3.24099557149147,-2.06963003990913,-16.2391544763694));
#56670=CARTESIAN_POINT('Ctrl Pts',(3.23753474759444,-2.0662687333896,-16.8413552372142));
#56671=CARTESIAN_POINT('Ctrl Pts',(3.23656829394497,-2.06534293239529,-17.2418783823923));
#56672=CARTESIAN_POINT('Ctrl Pts',(3.23656896082705,-2.06534377018181,-17.6221221200761));
#56673=CARTESIAN_POINT('Ctrl Pts',(3.23657012615242,-2.06534337879792,-17.8038210873795));
#56674=CARTESIAN_POINT('Ctrl Pts',(3.23657188269388,-2.06534153551086,-17.9847374128284));
#56675=CARTESIAN_POINT('',(2.6112,-1.7952,-12.0768));
#56676=CARTESIAN_POINT('Ctrl Pts',(2.6112,-1.7952,-12.0768));
#56677=CARTESIAN_POINT('Ctrl Pts',(2.70108906248718,-1.88293102006866,-11.97158933628));
#56678=CARTESIAN_POINT('Ctrl Pts',(2.80383287136991,-1.94791497263524,-11.8532683416248));
#56679=CARTESIAN_POINT('Ctrl Pts',(2.95935587549655,-2.0131643150658,-11.6768902688329));
#56680=CARTESIAN_POINT('Ctrl Pts',(3.01128269850091,-2.02984330840291,-11.6183900264733));
#56681=CARTESIAN_POINT('Ctrl Pts',(3.09123953787233,-2.04821304173687,-11.529435637509));
#56682=CARTESIAN_POINT('Ctrl Pts',(3.11894944687461,-2.05328114880983,-11.4988527223898));
#56683=CARTESIAN_POINT('Ctrl Pts',(3.17524764513357,-2.06093594854933,-11.4367604756888));
#56684=CARTESIAN_POINT('Ctrl Pts',(3.20350843291098,-2.06343538786481,-11.4052693925845));
#56685=CARTESIAN_POINT('Ctrl Pts',(3.23357666665279,-2.06468169900353,-11.3729269299378));
#56686=CARTESIAN_POINT('Ctrl Pts',(3.23475628359345,-2.06472837703521,-11.3716581976009));
#56687=CARTESIAN_POINT('Ctrl Pts',(3.2359359640172,-2.06477283942451,-11.3703894647503));
#56688=CARTESIAN_POINT('',(2.6112,-1.7952,-12.0768));
#56689=CARTESIAN_POINT('Ctrl Pts',(-3.29642266651177,-1.79519748712059,
-12.0768026712547));
#56690=CARTESIAN_POINT('Ctrl Pts',(-3.24358001593308,-1.7951975141813,-12.0768026674452));
#56691=CARTESIAN_POINT('Ctrl Pts',(-3.19073147951111,-1.79519754134527,
-12.0768026631509));
#56692=CARTESIAN_POINT('Ctrl Pts',(-2.30200704699003,-1.79519799153053,
-12.0768025940069));
#56693=CARTESIAN_POINT('Ctrl Pts',(-0.210367141271462,-1.7951990085787,
-12.0768020751207));
#56694=CARTESIAN_POINT('Ctrl Pts',(1.88431933586522,-1.79519823108613,-12.0768025301754));
#56695=CARTESIAN_POINT('Ctrl Pts',(3.1907250856176,-1.79519754057334,-12.0768026640128));
#56696=CARTESIAN_POINT('Ctrl Pts',(3.24358391077697,-1.79519751417976,-12.076802667445));
#56697=CARTESIAN_POINT('Ctrl Pts',(3.29642845573587,-1.79519748711763,-12.0768026712551));
#56698=CARTESIAN_POINT('Ctrl Pts',(-3.27408831410364,-1.9722276015856,-11.888615889407));
#56699=CARTESIAN_POINT('Ctrl Pts',(-3.22130116681679,-1.97032122721793,
-11.8888842560883));
#56700=CARTESIAN_POINT('Ctrl Pts',(-3.16852989305899,-1.96840757721836,
-11.889186770879));
#56701=CARTESIAN_POINT('Ctrl Pts',(-2.28147119761913,-1.93669289133901,
-11.8940577302633));
#56702=CARTESIAN_POINT('Ctrl Pts',(-0.206758859811364,-1.86504377040126,
-11.9306120492651));
#56703=CARTESIAN_POINT('Ctrl Pts',(1.86459196778903,-1.91981665684861,-11.8985544808556));
#56704=CARTESIAN_POINT('Ctrl Pts',(3.16852276150168,-1.96846195848408,-11.8891260506951));
#56705=CARTESIAN_POINT('Ctrl Pts',(3.22130505642342,-1.97032133571503,-11.8888842700037));
#56706=CARTESIAN_POINT('Ctrl Pts',(3.27409409724692,-1.97222781045467,-11.8886158599898));
#56707=CARTESIAN_POINT('Ctrl Pts',(-3.25188642042027,-2.07124454663285,
-11.6291452762124));
#56708=CARTESIAN_POINT('Ctrl Pts',(-3.19915094357724,-2.06808131163795,
-11.6308935276775));
#56709=CARTESIAN_POINT('Ctrl Pts',(-3.1464530232335,-2.06491642594862,-11.6326958363931));
#56710=CARTESIAN_POINT('Ctrl Pts',(-2.26099539435471,-2.01245733351299,
-11.66238937861));
#56711=CARTESIAN_POINT('Ctrl Pts',(-0.203136696371867,-1.90101534660559,
-11.7690581356509));
#56712=CARTESIAN_POINT('Ctrl Pts',(1.84488996298587,-1.98523478906184,-11.6813986289955));
#56713=CARTESIAN_POINT('Ctrl Pts',(3.1464452756991,-2.06498681864732,-11.6325557398156));
#56714=CARTESIAN_POINT('Ctrl Pts',(3.19915482816189,-2.06808150272424,-11.6308934784624));
#56715=CARTESIAN_POINT('Ctrl Pts',(3.25189219790266,-2.07124489320274,-11.6291450846441));
#56716=CARTESIAN_POINT('Ctrl Pts',(-3.23597709627681,-2.0647751983077,-11.3703832379468));
#56717=CARTESIAN_POINT('Ctrl Pts',(-3.18320926520253,-2.06164839985804,
-11.3736415239251));
#56718=CARTESIAN_POINT('Ctrl Pts',(-3.13049942170299,-2.05852190907284,
-11.3769735809423));
#56719=CARTESIAN_POINT('Ctrl Pts',(-2.24493355632026,-2.00672158959924,
-11.4319074741996));
#56720=CARTESIAN_POINT('Ctrl Pts',(-0.199619045096931,-1.89967482673457,
-11.6080442665278));
#56721=CARTESIAN_POINT('Ctrl Pts',(1.82862748588428,-1.98056379950097,-11.4653731295733));
#56722=CARTESIAN_POINT('Ctrl Pts',(3.13049602407356,-2.0585699244099,-11.3767617538477));
#56723=CARTESIAN_POINT('Ctrl Pts',(3.18321314808538,-2.06164860144816,-11.3736414048196));
#56724=CARTESIAN_POINT('Ctrl Pts',(3.23598287730504,-2.0647755408798,-11.370382880926));
#56725=CARTESIAN_POINT('',(-2.6112,-1.7952,-12.0768));
#56726=CARTESIAN_POINT('Origin',(0.,-1.7952,-14.688));
#56727=CARTESIAN_POINT('Ctrl Pts',(-27.803209900382,9.23603435870819,-72.5577790171547));
#56728=CARTESIAN_POINT('Ctrl Pts',(-27.8052592499116,10.4382360290543,-71.9219265766247));
#56729=CARTESIAN_POINT('Ctrl Pts',(-27.8073085994413,11.6404376994003,-71.2860741360946));
#56730=CARTESIAN_POINT('Ctrl Pts',(-27.8093579489709,12.8426393697465,-70.6502216955646));
#56731=CARTESIAN_POINT('Ctrl Pts',(-27.6551378439486,9.49096672380132,-73.0393005844633));
#56732=CARTESIAN_POINT('Ctrl Pts',(-27.6577399757294,10.6926691697792,-72.4025060111301));
#56733=CARTESIAN_POINT('Ctrl Pts',(-27.6603592487415,11.8943607952455,-71.7656911381846));
#56734=CARTESIAN_POINT('Ctrl Pts',(-27.6629613805351,13.0960632412153,-71.1288965648361));
#56735=CARTESIAN_POINT('Ctrl Pts',(-27.3490633632825,10.0377474084797,-74.0689767319683));
#56736=CARTESIAN_POINT('Ctrl Pts',(-27.3523402607163,11.2386401731222,-73.4306601269834));
#56737=CARTESIAN_POINT('Ctrl Pts',(-27.3556287080767,12.4395358745722,-72.7923490828472));
#56738=CARTESIAN_POINT('Ctrl Pts',(-27.3589056055191,13.6404286392169,-72.1540324778666));
#56739=CARTESIAN_POINT('Ctrl Pts',(-26.7423192852016,11.1383815330078,-76.1342058942393));
#56740=CARTESIAN_POINT('Ctrl Pts',(-26.7452350312789,12.3387016520456,-75.4948119055702));
#56741=CARTESIAN_POINT('Ctrl Pts',(-26.7481576407974,13.5390168090643,-74.8554085957215));
#56742=CARTESIAN_POINT('Ctrl Pts',(-26.7510733868799,14.7393369280985,-74.2160146070454));
#56743=CARTESIAN_POINT('Ctrl Pts',(-26.2567727580936,11.9678276411624,-77.6901374866193));
#56744=CARTESIAN_POINT('Ctrl Pts',(-26.2588779851847,13.1684233865823,-77.0512578239776));
#56745=CARTESIAN_POINT('Ctrl Pts',(-26.2610419402911,14.3690213682034,-76.4123829857732));
#56746=CARTESIAN_POINT('Ctrl Pts',(-26.2631471674262,15.5696171136249,-75.7735033231351));
#56747=CARTESIAN_POINT('Ctrl Pts',(-25.9521939343629,12.4413211944637,-78.5797217247913));
#56748=CARTESIAN_POINT('Ctrl Pts',(-25.9541384780474,13.6421291419706,-77.941240813488));
#56749=CARTESIAN_POINT('Ctrl Pts',(-25.9560830217321,14.8429370894773,-77.3027599021845));
#56750=CARTESIAN_POINT('Ctrl Pts',(-25.9580275654167,16.0437450369841,-76.6642789908811));
#56751=CARTESIAN_POINT('',(-25.9551107509796,14.2425337887163,-77.6219999999998));
#56752=CARTESIAN_POINT('',(-27.806283925825,11.0393375380009,-71.6039999999963));
#56753=CARTESIAN_POINT('Ctrl Pts',(-30.3753540341099,6.01695723880277,-66.3794227429406));
#56754=CARTESIAN_POINT('Ctrl Pts',(-30.362690827324,7.26996265932069,-65.8504120080144));
#56755=CARTESIAN_POINT('Ctrl Pts',(-30.350027620538,8.52296807983859,-65.3214012730881));
#56756=CARTESIAN_POINT('Ctrl Pts',(-30.3373644137521,9.7759735003565,-64.7923905381619));
#56757=CARTESIAN_POINT('Ctrl Pts',(-30.1088133612586,6.21732189962616,-66.8603832394881));
#56758=CARTESIAN_POINT('Ctrl Pts',(-30.106912725349,7.45664743997982,-66.2989301326288));
#56759=CARTESIAN_POINT('Ctrl Pts',(-30.104370068785,8.69572635844707,-65.7362566384473));
#56760=CARTESIAN_POINT('Ctrl Pts',(-30.1024695839643,9.93505195683909,-65.1748038187859));
#56761=CARTESIAN_POINT('Ctrl Pts',(-29.7096580135423,6.55735136704459,-67.5873569901587));
#56762=CARTESIAN_POINT('Ctrl Pts',(-29.7189274177172,7.7778112690182,-66.9861296374917));
#56763=CARTESIAN_POINT('Ctrl Pts',(-29.7274740067858,8.99846080978516,-66.3850583054978));
#56764=CARTESIAN_POINT('Ctrl Pts',(-29.7367435810634,10.2189206671305,-65.783830916114));
#56765=CARTESIAN_POINT('Ctrl Pts',(-28.7821722057447,7.57574471691707,-69.5467552476757));
#56766=CARTESIAN_POINT('Ctrl Pts',(-28.8019189087709,8.76527728138276,-68.8866094926591));
#56767=CARTESIAN_POINT('Ctrl Pts',(-28.821609300456,9.95439323841018,-68.2252261249033));
#56768=CARTESIAN_POINT('Ctrl Pts',(-28.8413560167341,11.1439259009176,-67.5650806611384));
#56769=CARTESIAN_POINT('Ctrl Pts',(-28.2846186462697,8.42885715791647,-71.0332031632364));
#56770=CARTESIAN_POINT('Ctrl Pts',(-28.2867169655075,9.61827756684128,-70.3734598241401));
#56771=CARTESIAN_POINT('Ctrl Pts',(-28.2831472841818,10.8081867183063,-69.7127753471578));
#56772=CARTESIAN_POINT('Ctrl Pts',(-28.2852469372896,11.9976070122136,-69.0530322295429));
#56773=CARTESIAN_POINT('Ctrl Pts',(-27.8032099026791,9.23603570625527,-72.5577783044281));
#56774=CARTESIAN_POINT('Ctrl Pts',(-27.8052594925831,10.4383783864874,-71.9218512828337));
#56775=CARTESIAN_POINT('Ctrl Pts',(-27.8073090824873,11.6407210667195,-71.2859242612392));
#56776=CARTESIAN_POINT('Ctrl Pts',(-27.8093586723913,12.8430637469518,-70.6499972396448));
#56777=CARTESIAN_POINT('',(-30.356361458725,7.89624424005172,-65.585999999999));
#56778=CARTESIAN_POINT('Ctrl Pts',(-33.2870419060249,4.35253527707242,-59.9326413364709));
#56779=CARTESIAN_POINT('Ctrl Pts',(-33.1297679354289,5.68135810058103,-59.6895471121553));
#56780=CARTESIAN_POINT('Ctrl Pts',(-32.972493964833,7.01018092408964,-59.4464528878397));
#56781=CARTESIAN_POINT('Ctrl Pts',(-32.815219994237,8.33900374759826,-59.2033586635242));
#56782=CARTESIAN_POINT('Ctrl Pts',(-33.1236843979303,4.41327697339383,-60.3703598245789));
#56783=CARTESIAN_POINT('Ctrl Pts',(-32.9800384987428,5.74096812205601,-60.1121164371264));
#56784=CARTESIAN_POINT('Ctrl Pts',(-32.8359640769173,7.06851339890597,-59.8537914806801));
#56785=CARTESIAN_POINT('Ctrl Pts',(-32.6923181777297,8.39620454756814,-59.5955480932275));
#56786=CARTESIAN_POINT('Ctrl Pts',(-32.6598069524929,4.6233160195265,-61.6572795724073));
#56787=CARTESIAN_POINT('Ctrl Pts',(-32.5452155833611,5.94541733829744,-61.3571538338168));
#56788=CARTESIAN_POINT('Ctrl Pts',(-32.4316412768296,7.26750554303185,-61.056817941821));
#56789=CARTESIAN_POINT('Ctrl Pts',(-32.3170499076978,8.58960686180279,-60.7566922032304));
#56790=CARTESIAN_POINT('Ctrl Pts',(-31.725539611122,5.1629429740609,-64.061279077029));
#56791=CARTESIAN_POINT('Ctrl Pts',(-31.6492324422371,6.46500946226312,-63.6680054128815));
#56792=CARTESIAN_POINT('Ctrl Pts',(-31.5713187665878,7.7670647622256,-63.2747836659281));
#56793=CARTESIAN_POINT('Ctrl Pts',(-31.4950115977029,9.06913125042783,-62.8815100017806));
#56794=CARTESIAN_POINT('Ctrl Pts',(-30.929578969617,5.6097190919677,-65.4015789370632));
#56795=CARTESIAN_POINT('Ctrl Pts',(-30.8937893171137,6.88505174727525,-64.926143571465));
#56796=CARTESIAN_POINT('Ctrl Pts',(-30.8617691542772,8.15989840357671,-64.4502875333333));
#56797=CARTESIAN_POINT('Ctrl Pts',(-30.825979501774,9.43523105888426,-63.9748521677351));
#56798=CARTESIAN_POINT('Ctrl Pts',(-30.3753540341099,6.01695723880277,-66.3794227429406));
#56799=CARTESIAN_POINT('Ctrl Pts',(-30.3626923171866,7.26981523963541,-65.8504742476462));
#56800=CARTESIAN_POINT('Ctrl Pts',(-30.3500306002633,8.52267324046804,-65.3215257523518));
#56801=CARTESIAN_POINT('Ctrl Pts',(-30.33736888334,9.77553124130067,-64.7925772570574));
#56802=CARTESIAN_POINT('',(-33.051130950131,6.34576951233522,-59.5679999999976));
#56803=CARTESIAN_POINT('',(-33.0511309501309,6.34576951233534,-59.5679999999975));
#56804=CARTESIAN_POINT('',(-33.0511309501309,6.34576951233534,-59.5679999999975));
#56805=CARTESIAN_POINT('Ctrl Pts',(-36.1829138277439,4.79791400485575,-53.6562428681641));
#56806=CARTESIAN_POINT('Ctrl Pts',(-35.7573813489674,6.08768352765237,-53.5854142893892));
#56807=CARTESIAN_POINT('Ctrl Pts',(-35.3318488701909,7.377453050449,-53.5145857106142));
#56808=CARTESIAN_POINT('Ctrl Pts',(-34.9063163914144,8.66722257324563,-53.4437571318393));
#56809=CARTESIAN_POINT('Ctrl Pts',(-35.8221894292354,4.71279832802143,-54.2735126527001));
#56810=CARTESIAN_POINT('Ctrl Pts',(-35.4055710113178,6.0086770499647,-54.27897609436));
#56811=CARTESIAN_POINT('Ctrl Pts',(-34.9890919720113,7.30764932080681,-54.2841345487856));
#56812=CARTESIAN_POINT('Ctrl Pts',(-34.5724735540937,8.60352804275007,-54.2895979904455));
#56813=CARTESIAN_POINT('Ctrl Pts',(-35.1345762789437,4.46191327643785,-55.4630423598499));
#56814=CARTESIAN_POINT('Ctrl Pts',(-34.7604641920181,5.76926615742872,-55.5213765022354));
#56815=CARTESIAN_POINT('Ctrl Pts',(-34.3847798507744,7.07531096957354,-55.5792446567707));
#56816=CARTESIAN_POINT('Ctrl Pts',(-34.0106677638488,8.38266385056441,-55.6375787991562));
#56817=CARTESIAN_POINT('Ctrl Pts',(-34.1112888063175,4.18758073788383,-57.6561452037581));
#56818=CARTESIAN_POINT('Ctrl Pts',(-33.8593807355069,5.52781101585105,-57.6216091426396));
#56819=CARTESIAN_POINT('Ctrl Pts',(-33.6074801111067,6.86853513824409,-57.5872134595304));
#56820=CARTESIAN_POINT('Ctrl Pts',(-33.3555720402961,8.20876541621131,-57.5526773984119));
#56821=CARTESIAN_POINT('Ctrl Pts',(-33.5340571648804,4.24789457701618,-59.2008344761412));
#56822=CARTESIAN_POINT('Ctrl Pts',(-33.3563722159371,5.58810392677528,-59.0303155049847));
#56823=CARTESIAN_POINT('Ctrl Pts',(-33.1759712955042,6.92623598341401,-58.8588145985647));
#56824=CARTESIAN_POINT('Ctrl Pts',(-32.9982863465608,8.26644533317311,-58.6882956274082));
#56825=CARTESIAN_POINT('Ctrl Pts',(-33.2870419060249,4.35253527707242,-59.9326413364709));
#56826=CARTESIAN_POINT('Ctrl Pts',(-33.1297679354289,5.68135810058103,-59.6895471121553));
#56827=CARTESIAN_POINT('Ctrl Pts',(-32.972493964833,7.01018092408964,-59.4464528878397));
#56828=CARTESIAN_POINT('Ctrl Pts',(-32.815219994237,8.33900374759826,-59.2033586635242));
#56829=CARTESIAN_POINT('',(-35.5446151095792,6.73256828905069,-53.5500000000017));
#56830=CARTESIAN_POINT('',(-35.5446151095792,6.73256828905069,-53.5500000000017));
#56831=CARTESIAN_POINT('',(-35.5446151095792,6.73256828905069,-53.5500000000017));
#56832=CARTESIAN_POINT('Ctrl Pts',(-38.0224713055506,4.8684211641347,-47.6590291921613));
#56833=CARTESIAN_POINT('Ctrl Pts',(-37.5141101402729,6.12702180277212,-47.5743024240645));
#56834=CARTESIAN_POINT('Ctrl Pts',(-37.0057489009982,7.38562239684713,-47.4895759845357));
#56835=CARTESIAN_POINT('Ctrl Pts',(-36.4973877357239,8.6442230354866,-47.4048492164237));
#56836=CARTESIAN_POINT('Ctrl Pts',(-37.9812710970613,4.87622981994569,-48.0222296824199));
#56837=CARTESIAN_POINT('Ctrl Pts',(-37.4764043002191,6.13527223994773,-47.9241769029098));
#56838=CARTESIAN_POINT('Ctrl Pts',(-36.9719750983327,7.39457818133208,-47.8241811391747));
#56839=CARTESIAN_POINT('Ctrl Pts',(-36.4671082813248,8.65362058919022,-47.7261284492034));
#56840=CARTESIAN_POINT('Ctrl Pts',(-37.8390117177081,4.91385054480188,-49.0952025625359));
#56841=CARTESIAN_POINT('Ctrl Pts',(-37.3492889481593,6.17608455138244,-48.9616650119934));
#56842=CARTESIAN_POINT('Ctrl Pts',(-36.8594199960831,7.43860904700498,-48.8252249030439));
#56843=CARTESIAN_POINT('Ctrl Pts',(-36.3696972332709,8.7008430401989,-48.6916874862603));
#56844=CARTESIAN_POINT('Ctrl Pts',(-37.4172803943982,4.97200440485067,-51.0816419245504));
#56845=CARTESIAN_POINT('Ctrl Pts',(-36.9598775494223,6.2431156660951,-50.9280798398504));
#56846=CARTESIAN_POINT('Ctrl Pts',(-36.5027094328069,7.51388912919058,-50.7775833348501));
#56847=CARTESIAN_POINT('Ctrl Pts',(-36.0453065770139,8.78500040600178,-50.6240211088788));
#56848=CARTESIAN_POINT('Ctrl Pts',(-36.8017946572527,4.93958146881401,-52.5177513156359));
#56849=CARTESIAN_POINT('Ctrl Pts',(-36.3599669126062,6.21923512189812,-52.3770542244419));
#56850=CARTESIAN_POINT('Ctrl Pts',(-35.9183025240337,7.50075084985685,-52.2181590441769));
#56851=CARTESIAN_POINT('Ctrl Pts',(-35.4764747718593,8.78040441713075,-52.0774627916075));
#56852=CARTESIAN_POINT('Ctrl Pts',(-36.1828876819812,4.79790801989533,-53.6562909659612));
#56853=CARTESIAN_POINT('Ctrl Pts',(-35.7573460862841,6.08770768960492,-53.5854637068186));
#56854=CARTESIAN_POINT('Ctrl Pts',(-35.3318044836858,7.37750728064934,-53.5146372164721));
#56855=CARTESIAN_POINT('Ctrl Pts',(-34.906262887989,8.66730695036257,-53.4438099572941));
#56856=CARTESIAN_POINT('',(-37.2599410472769,6.75628005534009,-47.5319999999999));
#56857=CARTESIAN_POINT('Ctrl Pts',(-38.8604541099244,4.82976572790842,-41.6539325852781));
#56858=CARTESIAN_POINT('Ctrl Pts',(-38.4040326949895,6.10748900320921,-41.5606441950923));
#56859=CARTESIAN_POINT('Ctrl Pts',(-37.9476112800546,7.38521227851001,-41.4673558049066));
#56860=CARTESIAN_POINT('Ctrl Pts',(-37.4911898651198,8.66293555381081,-41.3740674147208));
#56861=CARTESIAN_POINT('Ctrl Pts',(-38.7579547565586,4.82831575431509,-42.1355598788231));
#56862=CARTESIAN_POINT('Ctrl Pts',(-38.2908397454192,6.10259351827304,-42.0473364200289));
#56863=CARTESIAN_POINT('Ctrl Pts',(-37.8238151536734,7.37689668296498,-41.9592074712887));
#56864=CARTESIAN_POINT('Ctrl Pts',(-37.3567001425339,8.65117444692294,-41.8709840124945));
#56865=CARTESIAN_POINT('Ctrl Pts',(-38.6165637640568,4.82401373724133,-42.8556343306891));
#56866=CARTESIAN_POINT('Ctrl Pts',(-38.1329344749416,6.09261012024952,-42.7744054967877));
#56867=CARTESIAN_POINT('Ctrl Pts',(-37.6491758337013,7.36115804152699,-42.6932058475502));
#56868=CARTESIAN_POINT('Ctrl Pts',(-37.1655465445862,8.62975442453518,-42.6119770136488));
#56869=CARTESIAN_POINT('Ctrl Pts',(-38.4070763697413,4.82011917504479,-44.1382125964065));
#56870=CARTESIAN_POINT('Ctrl Pts',(-37.8997443650628,6.07993325028302,-44.0657708065558));
#56871=CARTESIAN_POINT('Ctrl Pts',(-37.3923641700085,7.33974267197774,-43.993425978326));
#56872=CARTESIAN_POINT('Ctrl Pts',(-36.88503216533,8.59955674721597,-43.9209841884754));
#56873=CARTESIAN_POINT('Ctrl Pts',(-38.2178923694507,4.82934361138434,-45.7021852706702));
#56874=CARTESIAN_POINT('Ctrl Pts',(-37.6956752256365,6.08323545488938,-45.6340690461451));
#56875=CARTESIAN_POINT('Ctrl Pts',(-37.173491249573,7.33714039137729,-45.5659389089267));
#56876=CARTESIAN_POINT('Ctrl Pts',(-36.6512741057588,8.59103223488232,-45.4978226844016));
#56877=CARTESIAN_POINT('Ctrl Pts',(-38.0970582995982,4.85566739849337,-47.0220693317479));
#56878=CARTESIAN_POINT('Ctrl Pts',(-37.5826091437923,6.11231335186017,-46.9455012979541));
#56879=CARTESIAN_POINT('Ctrl Pts',(-37.0677383294391,7.36884011707376,-46.8691997614158));
#56880=CARTESIAN_POINT('Ctrl Pts',(-36.5532891736331,8.62548607044055,-46.792631727622));
#56881=CARTESIAN_POINT('Ctrl Pts',(-38.0224643391855,4.8684224845004,-47.6590906035864));
#56882=CARTESIAN_POINT('Ctrl Pts',(-37.5141154779131,6.12699419839353,-47.5743635345287));
#56883=CARTESIAN_POINT('Ctrl Pts',(-37.0057666166406,7.38556591228666,-47.489636465471));
#56884=CARTESIAN_POINT('Ctrl Pts',(-36.4974177553682,8.64413762617978,-47.4049093964133));
#56885=CARTESIAN_POINT('',(-38.1758219875221,6.74635064085961,-41.5139999999995));
#56886=CARTESIAN_POINT('Ctrl Pts',(-40.1355634406229,4.76730425857361,-35.6660853079992));
#56887=CARTESIAN_POINT('Ctrl Pts',(-39.7267565272628,6.05944617662692,-35.5526924624031));
#56888=CARTESIAN_POINT('Ctrl Pts',(-39.3179496117989,7.35158809405154,-35.4392996166302));
#56889=CARTESIAN_POINT('Ctrl Pts',(-38.9091426984386,8.64373001210486,-35.3259067710341));
#56890=CARTESIAN_POINT('Ctrl Pts',(-40.069789899138,4.77667325925527,-36.0099761177602));
#56891=CARTESIAN_POINT('Ctrl Pts',(-39.6647601607778,6.07017700486549,-35.8984639074028));
#56892=CARTESIAN_POINT('Ctrl Pts',(-39.2599437298742,7.36374449671887,-35.7869696292885));
#56893=CARTESIAN_POINT('Ctrl Pts',(-38.854913990157,8.65724824192357,-35.6754574188171));
#56894=CARTESIAN_POINT('Ctrl Pts',(-39.9548410579829,4.79179797702963,-36.6038794519936));
#56895=CARTESIAN_POINT('Ctrl Pts',(-39.5552706371814,6.08724978139326,-36.4953741367376));
#56896=CARTESIAN_POINT('Ctrl Pts',(-39.1556935142984,7.382699722788,-36.3868668179017));
#56897=CARTESIAN_POINT('Ctrl Pts',(-38.7561230935397,8.67815152716346,-36.2783615026586));
#56898=CARTESIAN_POINT('Ctrl Pts',(-39.7443037262004,4.81133016772462,-37.6330866698068));
#56899=CARTESIAN_POINT('Ctrl Pts',(-39.3462971338669,6.10759749935179,-37.5287105189401));
#56900=CARTESIAN_POINT('Ctrl Pts',(-38.9483293158955,7.40387558580187,-37.4243359249927));
#56901=CARTESIAN_POINT('Ctrl Pts',(-38.5503227233153,8.70014291736062,-37.3199597741161));
#56902=CARTESIAN_POINT('Ctrl Pts',(-39.5813565519597,4.82173156565819,-38.3962454196463));
#56903=CARTESIAN_POINT('Ctrl Pts',(-39.1798326777781,6.11712296255223,-38.2944317819117));
#56904=CARTESIAN_POINT('Ctrl Pts',(-38.7782569657644,7.41249976037084,-38.1926219386844));
#56905=CARTESIAN_POINT('Ctrl Pts',(-38.3767330919126,8.70789115735774,-38.0908083009255));
#56906=CARTESIAN_POINT('Ctrl Pts',(-39.4305411403599,4.82773783061676,-39.0811836979273));
#56907=CARTESIAN_POINT('Ctrl Pts',(-39.0220576798717,6.12110969421629,-38.9813878108934));
#56908=CARTESIAN_POINT('Ctrl Pts',(-38.6136027152855,7.41449063362709,-38.8815873335481));
#56909=CARTESIAN_POINT('Ctrl Pts',(-38.205119254616,8.70786249716888,-38.7817914465434));
#56910=CARTESIAN_POINT('Ctrl Pts',(-39.2609912818215,4.83170251246378,-39.8388585382037));
#56911=CARTESIAN_POINT('Ctrl Pts',(-38.8419292709767,6.12186145082356,-39.7411109024355));
#56912=CARTESIAN_POINT('Ctrl Pts',(-38.4227884822824,7.41199667487817,-39.6433661601837));
#56913=CARTESIAN_POINT('Ctrl Pts',(-38.0037264719387,8.7021556133888,-39.5456185243971));
#56914=CARTESIAN_POINT('Ctrl Pts',(-39.0664816974284,4.83206157495894,-40.6998863785975));
#56915=CARTESIAN_POINT('Ctrl Pts',(-38.6309073172999,6.11693937633135,-40.6042764850154));
#56916=CARTESIAN_POINT('Ctrl Pts',(-38.1954185995026,7.40184291372179,-40.5086663461849));
#56917=CARTESIAN_POINT('Ctrl Pts',(-37.7598442188292,8.68672071493048,-40.4130564526044));
#56918=CARTESIAN_POINT('Ctrl Pts',(-38.9270107680783,4.83045995066367,-41.3378067172326));
#56919=CARTESIAN_POINT('Ctrl Pts',(-38.477464005224,6.11058667135808,-41.2437467144136));
#56920=CARTESIAN_POINT('Ctrl Pts',(-38.0278583234486,7.39069394777282,-41.1496860831278));
#56921=CARTESIAN_POINT('Ctrl Pts',(-37.5783115609693,8.67082066859093,-41.055626080313));
#56922=CARTESIAN_POINT('Ctrl Pts',(-38.8604527970962,4.82976571421489,-41.6539388208502));
#56923=CARTESIAN_POINT('Ctrl Pts',(-38.4040297947643,6.10749300631662,-41.5606501491508));
#56924=CARTESIAN_POINT('Ctrl Pts',(-37.9476067935945,7.3852202988019,-41.4673614774639));
#56925=CARTESIAN_POINT('Ctrl Pts',(-37.4911837912626,8.66294759090364,-41.3740728057645));
#56926=CARTESIAN_POINT('',(-39.5223544282476,6.70551108323309,-35.4960000000003));
#56927=CARTESIAN_POINT('Ctrl Pts',(-41.4215456143025,4.68791021227309,-29.7512571116587));
#56928=CARTESIAN_POINT('Ctrl Pts',(-40.8936521308426,5.92796748849508,-29.5690857038871));
#56929=CARTESIAN_POINT('Ctrl Pts',(-40.3657586473827,7.16802476471708,-29.3869142961156));
#56930=CARTESIAN_POINT('Ctrl Pts',(-39.8378651639228,8.40808204093907,-29.204742888344));
#56931=CARTESIAN_POINT('Ctrl Pts',(-41.3092811227302,4.69284109397027,-30.1101403746882));
#56932=CARTESIAN_POINT('Ctrl Pts',(-40.7860870227411,5.9370021984995,-29.9421436309555));
#56933=CARTESIAN_POINT('Ctrl Pts',(-40.2635498200622,7.18142713867819,-29.7744672927514));
#56934=CARTESIAN_POINT('Ctrl Pts',(-39.7403557200732,8.42558824320743,-29.6064705490188));
#56935=CARTESIAN_POINT('Ctrl Pts',(-41.1168122255416,4.70227545160565,-30.8154015426932));
#56936=CARTESIAN_POINT('Ctrl Pts',(-40.6066654279172,5.95485537606158,-30.6714196014921));
#56937=CARTESIAN_POINT('Ctrl Pts',(-40.0964689705627,7.20743999775218,-30.5275444808975));
#56938=CARTESIAN_POINT('Ctrl Pts',(-39.5863221729383,8.46001992220811,-30.3835625396964));
#56939=CARTESIAN_POINT('Ctrl Pts',(-40.9411342639833,4.71057860533754,-31.5583878958659));
#56940=CARTESIAN_POINT('Ctrl Pts',(-40.4474171521444,5.97172751091908,-31.43372866912));
#56941=CARTESIAN_POINT('Ctrl Pts',(-39.9536697830691,7.23283887630036,-31.3089175330362));
#56942=CARTESIAN_POINT('Ctrl Pts',(-39.4599526712302,8.4939877818819,-31.1842583062903));
#56943=CARTESIAN_POINT('Ctrl Pts',(-40.72104027405,4.72052127144792,-32.5727429381947));
#56944=CARTESIAN_POINT('Ctrl Pts',(-40.2513012525973,5.99266951177614,-32.4676364806858));
#56945=CARTESIAN_POINT('Ctrl Pts',(-39.7814912297972,7.26478923819657,-32.3624564233432));
#56946=CARTESIAN_POINT('Ctrl Pts',(-39.3117522083446,8.53693747852479,-32.2573499658343));
#56947=CARTESIAN_POINT('Ctrl Pts',(-40.5142429668683,4.72897579183149,-33.638548551572));
#56948=CARTESIAN_POINT('Ctrl Pts',(-40.0706647764219,6.01107660461561,-33.5420022229916));
#56949=CARTESIAN_POINT('Ctrl Pts',(-39.6270110271653,7.29317024951508,-33.4456444889633));
#56950=CARTESIAN_POINT('Ctrl Pts',(-39.1834328367189,8.5752710622992,-33.3490981603829));
#56951=CARTESIAN_POINT('Ctrl Pts',(-40.3021090297733,4.74530128710119,-34.7695223916763));
#56952=CARTESIAN_POINT('Ctrl Pts',(-39.8808239070379,6.0344697149634,-34.668233741174));
#56953=CARTESIAN_POINT('Ctrl Pts',(-39.4597383158449,7.32367658963407,-34.5666679306649));
#56954=CARTESIAN_POINT('Ctrl Pts',(-39.0384531931095,8.61284501749628,-34.4653792801627));
#56955=CARTESIAN_POINT('Ctrl Pts',(-40.197670469322,4.75763956421394,-35.3320435682359));
#56956=CARTESIAN_POINT('Ctrl Pts',(-39.7850494778165,6.0490278260316,-35.2239026652054));
#56957=CARTESIAN_POINT('Ctrl Pts',(-39.3724789621606,7.34047705027623,-35.116161791104));
#56958=CARTESIAN_POINT('Ctrl Pts',(-38.9598579706551,8.6318653120939,-35.0080208880735));
#56959=CARTESIAN_POINT('Ctrl Pts',(-40.1355627919428,4.76730435097372,-35.6660886995623));
#56960=CARTESIAN_POINT('Ctrl Pts',(-39.726757216146,6.05944217247997,-35.5526962331876));
#56961=CARTESIAN_POINT('Ctrl Pts',(-39.3179516403492,7.35157999398622,-35.439303766813));
#56962=CARTESIAN_POINT('Ctrl Pts',(-38.9091460645523,8.64371781549247,-35.3259113004384));
#56963=CARTESIAN_POINT('',(-40.6297053891126,6.54799612660609,-29.4780000000013));
#56964=CARTESIAN_POINT('Ctrl Pts',(-44.8643748763769,5.20597739807172,-23.9801519722228));
#56965=CARTESIAN_POINT('Ctrl Pts',(-44.4545859760341,6.45554733375955,-23.633383990741));
#56966=CARTESIAN_POINT('Ctrl Pts',(-44.0447970756913,7.70511726944739,-23.2866160092593));
#56967=CARTESIAN_POINT('Ctrl Pts',(-43.6350081753485,8.95468720513522,-22.9398480277775));
#56968=CARTESIAN_POINT('Ctrl Pts',(-44.74295142856,5.19893273360771,-24.0982573983942));
#56969=CARTESIAN_POINT('Ctrl Pts',(-44.3193209089096,6.44821626255224,-23.7681532567383));
#56970=CARTESIAN_POINT('Ctrl Pts',(-43.8977879609805,7.69892472923156,-23.436688867068));
#56971=CARTESIAN_POINT('Ctrl Pts',(-43.4741574413301,8.94820825817609,-23.1065847254121));
#56972=CARTESIAN_POINT('Ctrl Pts',(-44.4866987396665,5.17768472779144,-24.3599634571171));
#56973=CARTESIAN_POINT('Ctrl Pts',(-44.0364884211506,6.42690120872934,-24.0616242521564));
#56974=CARTESIAN_POINT('Ctrl Pts',(-43.5837431671894,7.67452928138004,-23.7650100449585));
#56975=CARTESIAN_POINT('Ctrl Pts',(-43.1335328486735,8.92374576231794,-23.4666708399978));
#56976=CARTESIAN_POINT('Ctrl Pts',(-43.7774989443756,5.08577719072335,-25.1469769549528));
#56977=CARTESIAN_POINT('Ctrl Pts',(-43.2443604259601,6.32042239432471,-24.933270807941));
#56978=CARTESIAN_POINT('Ctrl Pts',(-42.7146965077096,7.55714183044868,-24.7170780592635));
#56979=CARTESIAN_POINT('Ctrl Pts',(-42.181557989294,8.79178703405004,-24.5033719122517));
#56980=CARTESIAN_POINT('Ctrl Pts',(-42.7956488003254,4.84372654876611,-26.5306371507459));
#56981=CARTESIAN_POINT('Ctrl Pts',(-42.2045420756648,6.05642918637459,-26.3604342415932));
#56982=CARTESIAN_POINT('Ctrl Pts',(-41.6128293638815,7.2685808454858,-26.1904764286745));
#56983=CARTESIAN_POINT('Ctrl Pts',(-41.0217226392209,8.48128348309427,-26.0202735195218));
#56984=CARTESIAN_POINT('Ctrl Pts',(-41.9333999007591,4.68167633313014,-28.2389876838209));
#56985=CARTESIAN_POINT('Ctrl Pts',(-41.3748325386295,5.90841244052776,-28.0551638450349));
#56986=CARTESIAN_POINT('Ctrl Pts',(-40.8162962888588,7.13540891994494,-27.8716680562176));
#56987=CARTESIAN_POINT('Ctrl Pts',(-40.2577289267292,8.36214502734256,-27.6878442174315));
#56988=CARTESIAN_POINT('Ctrl Pts',(-41.5686373679341,4.67844271843895,-29.2605708183325));
#56989=CARTESIAN_POINT('Ctrl Pts',(-41.0326449179321,5.91472734108893,-29.0769717489468));
#56990=CARTESIAN_POINT('Ctrl Pts',(-40.4991794935331,7.15212798646055,-28.8912945519595));
#56991=CARTESIAN_POINT('Ctrl Pts',(-39.9631870435311,8.38841260911053,-28.7076954825739));
#56992=CARTESIAN_POINT('Ctrl Pts',(-41.4215456143024,4.68791021227308,-29.7512571116587));
#56993=CARTESIAN_POINT('Ctrl Pts',(-40.8936521308426,5.92796748849509,-29.5690857038871));
#56994=CARTESIAN_POINT('Ctrl Pts',(-40.3657586473827,7.16802476471709,-29.3869142961156));
#56995=CARTESIAN_POINT('Ctrl Pts',(-39.8378651639228,8.4080820409391,-29.204742888344));
#56996=CARTESIAN_POINT('',(-44.2496915258627,7.08033230160341,-23.4600000000002));
#56997=CARTESIAN_POINT('',(-44.2496915258627,7.08033230160347,-23.4600000000001));
#56998=CARTESIAN_POINT('',(-44.2496915258627,7.08033230160347,-23.4600000000001));
#56999=CARTESIAN_POINT('Ctrl Pts',(-57.8135230790975,6.69056632259502,-18.0349157107833));
#57000=CARTESIAN_POINT('Ctrl Pts',(-57.5247816344766,7.95941791373551,-17.6396385702623));
#57001=CARTESIAN_POINT('Ctrl Pts',(-57.2360401898557,9.22826950487599,-17.2443614297412));
#57002=CARTESIAN_POINT('Ctrl Pts',(-56.9472987452347,10.4971210960165,-16.8490842892202));
#57003=CARTESIAN_POINT('Ctrl Pts',(-57.1239745403965,6.58412560248485,-18.1969381440623));
#57004=CARTESIAN_POINT('Ctrl Pts',(-56.8293558324884,7.85914040842569,-17.8258953952808));
#57005=CARTESIAN_POINT('Ctrl Pts',(-56.5427656293713,9.13543238739557,-17.4526165469018));
#57006=CARTESIAN_POINT('Ctrl Pts',(-56.2481469214632,10.4104471933364,-17.0815737981202));
#57007=CARTESIAN_POINT('Ctrl Pts',(-55.0066008221098,6.23208146801642,-18.6635552175992));
#57008=CARTESIAN_POINT('Ctrl Pts',(-54.7175706740941,7.52475833001072,-18.3513974459225));
#57009=CARTESIAN_POINT('Ctrl Pts',(-54.423504213366,8.81665862928835,-18.0405169785343));
#57010=CARTESIAN_POINT('Ctrl Pts',(-54.1344740653502,10.1093354912827,-17.7283592068575));
#57011=CARTESIAN_POINT('Ctrl Pts',(-52.3438248091449,5.73435620824511,-19.2638310488358));
#57012=CARTESIAN_POINT('Ctrl Pts',(-52.0143059097852,7.02728121608903,-18.9991095830863));
#57013=CARTESIAN_POINT('Ctrl Pts',(-51.685864582759,8.32033229885559,-18.7344472086489));
#57014=CARTESIAN_POINT('Ctrl Pts',(-51.3563456833993,9.61325730669952,-18.4697257428994));
#57015=CARTESIAN_POINT('Ctrl Pts',(-50.0095424054025,5.30085549787886,-20.220604371564));
#57016=CARTESIAN_POINT('Ctrl Pts',(-49.643613283696,6.56955609994842,-19.8911383329522));
#57017=CARTESIAN_POINT('Ctrl Pts',(-49.2781182313849,7.83840233803338,-19.5613911754511));
#57018=CARTESIAN_POINT('Ctrl Pts',(-48.9121891096784,9.10710294010294,-19.2319251368394));
#57019=CARTESIAN_POINT('Ctrl Pts',(-48.2669654993335,5.10361702097977,-21.2264548583875));
#57020=CARTESIAN_POINT('Ctrl Pts',(-47.9253792124948,6.3492056772126,-20.7955041080243));
#57021=CARTESIAN_POINT('Ctrl Pts',(-47.5830128226939,7.59462899514417,-20.3653160983057));
#57022=CARTESIAN_POINT('Ctrl Pts',(-47.2414265358552,8.840217651377,-19.9343653479424));
#57023=CARTESIAN_POINT('Ctrl Pts',(-46.9594441235353,5.13430758608674,-22.1958151860038));
#57024=CARTESIAN_POINT('Ctrl Pts',(-46.648112214713,6.36337591783102,-21.7041817066266));
#57025=CARTESIAN_POINT('Ctrl Pts',(-46.3370798522678,7.59287361463498,-21.2113264208171));
#57026=CARTESIAN_POINT('Ctrl Pts',(-46.0257479434454,8.82194194637927,-20.7196929414398));
#57027=CARTESIAN_POINT('Ctrl Pts',(-45.8504881283735,5.21184561373662,-23.1088853518396));
#57028=CARTESIAN_POINT('Ctrl Pts',(-45.5253385580089,6.44309869251224,-22.6308162647746));
#57029=CARTESIAN_POINT('Ctrl Pts',(-45.2000143339031,7.67400918968744,-22.1535563605875));
#57030=CARTESIAN_POINT('Ctrl Pts',(-44.8748647635386,8.90526226846306,-21.6754872735224));
#57031=CARTESIAN_POINT('Ctrl Pts',(-45.2012130342128,5.23387305606066,-23.6826188427425));
#57032=CARTESIAN_POINT('Ctrl Pts',(-44.8305825688381,6.47688655683838,-23.2691414457344));
#57033=CARTESIAN_POINT('Ctrl Pts',(-44.458100546266,7.72159300799202,-22.8543779660973));
#57034=CARTESIAN_POINT('Ctrl Pts',(-44.0874700808914,8.96460650876973,-22.4409005690892));
#57035=CARTESIAN_POINT('Ctrl Pts',(-44.8643748763769,5.20597739807172,-23.9801519722228));
#57036=CARTESIAN_POINT('Ctrl Pts',(-44.4545859760341,6.45554733375955,-23.633383990741));
#57037=CARTESIAN_POINT('Ctrl Pts',(-44.0447970756913,7.70511726944739,-23.2866160092593));
#57038=CARTESIAN_POINT('Ctrl Pts',(-43.6350081753485,8.95468720513522,-22.9398480277775));
#57039=CARTESIAN_POINT('',(-57.3804109121661,8.59384370930575,-17.4420000000018));
#57040=CARTESIAN_POINT('',(-57.3804109121661,8.59384370930575,-17.4420000000018));
#57041=CARTESIAN_POINT('',(-57.3804109121661,8.59384370930575,-17.4420000000018));
#57042=CARTESIAN_POINT('Ctrl Pts',(-70.7282577522101,8.51486331985853,-11.892519184563));
#57043=CARTESIAN_POINT('Ctrl Pts',(-70.3600859174011,9.78627568391473,-11.5801730615225));
#57044=CARTESIAN_POINT('Ctrl Pts',(-69.9919140825922,11.0576880479709,-11.267826938482));
#57045=CARTESIAN_POINT('Ctrl Pts',(-69.6237422477832,12.3291004120271,-10.9554808154416));
#57046=CARTESIAN_POINT('Ctrl Pts',(-70.1991067619348,8.44172633189886,-12.218539623772));
#57047=CARTESIAN_POINT('Ctrl Pts',(-69.8208712427477,9.71815881129524,-11.9344438903904));
#57048=CARTESIAN_POINT('Ctrl Pts',(-69.4401822671779,10.9919767410639,-11.6547369719342));
#57049=CARTESIAN_POINT('Ctrl Pts',(-69.0619467479908,12.2684092204603,-11.3706412385527));
#57050=CARTESIAN_POINT('Ctrl Pts',(-68.595429397507,8.158930957405,-13.1757731414385));
#57051=CARTESIAN_POINT('Ctrl Pts',(-68.1715348548732,9.43443402361281,-12.9743515055776));
#57052=CARTESIAN_POINT('Ctrl Pts',(-67.7496672765525,10.7117699027939,-12.7692002791116));
#57053=CARTESIAN_POINT('Ctrl Pts',(-67.3257727339187,11.9872729690017,-12.5677786432507));
#57054=CARTESIAN_POINT('Ctrl Pts',(-66.4080850486133,7.61830551402404,-14.5220628619485));
#57055=CARTESIAN_POINT('Ctrl Pts',(-65.9863449158698,8.88672644030649,-14.2505530903174));
#57056=CARTESIAN_POINT('Ctrl Pts',(-65.5646075215418,10.1549810775789,-13.9790299757529));
#57057=CARTESIAN_POINT('Ctrl Pts',(-65.1428673887983,11.4234020038613,-13.7075202041218));
#57058=CARTESIAN_POINT('Ctrl Pts',(-63.7670026279933,7.28205441226018,-15.9847718406443));
#57059=CARTESIAN_POINT('Ctrl Pts',(-63.433848092195,8.52888773018001,-15.5476019176397));
#57060=CARTESIAN_POINT('Ctrl Pts',(-63.0999806953316,9.77527366757043,-15.1117880187483));
#57061=CARTESIAN_POINT('Ctrl Pts',(-62.7668261595333,11.0221069854903,-14.6746180957437));
#57062=CARTESIAN_POINT('Ctrl Pts',(-61.8892806965024,7.15471518367529,-16.8453028714865));
#57063=CARTESIAN_POINT('Ctrl Pts',(-61.6026532538942,8.38492602600039,-16.3432643430782));
#57064=CARTESIAN_POINT('Ctrl Pts',(-61.3170127161816,9.61579870788819,-15.8399025257027));
#57065=CARTESIAN_POINT('Ctrl Pts',(-61.0303852735734,10.8460095502133,-15.3378639972945));
#57066=CARTESIAN_POINT('Ctrl Pts',(-59.9765401917668,7.00460230079879,-17.5365065043827));
#57067=CARTESIAN_POINT('Ctrl Pts',(-59.7021139192336,8.24020918624605,-17.0371230534497));
#57068=CARTESIAN_POINT('Ctrl Pts',(-59.4266777566838,9.47499348818355,-16.5384607326821));
#57069=CARTESIAN_POINT('Ctrl Pts',(-59.1522514841506,10.7106003736308,-16.0390772817491));
#57070=CARTESIAN_POINT('Ctrl Pts',(-58.5497235666632,6.81245518627654,-17.8884040415039));
#57071=CARTESIAN_POINT('Ctrl Pts',(-58.2653553289422,8.06852593330302,-17.4497909528517));
#57072=CARTESIAN_POINT('Ctrl Pts',(-57.9817716639733,9.32584916951929,-17.0119688327944));
#57073=CARTESIAN_POINT('Ctrl Pts',(-57.6974034262523,10.5819199165458,-16.5733557441422));
#57074=CARTESIAN_POINT('Ctrl Pts',(-57.8135230790975,6.69056632259502,-18.0349157107833));
#57075=CARTESIAN_POINT('Ctrl Pts',(-57.5247816344766,7.95941791373551,-17.6396385702623));
#57076=CARTESIAN_POINT('Ctrl Pts',(-57.2360401898557,9.22826950487599,-17.2443614297412));
#57077=CARTESIAN_POINT('Ctrl Pts',(-56.9472987452347,10.4971210960165,-16.8490842892202));
#57078=CARTESIAN_POINT('',(-70.1759999999962,10.4219818659442,-11.4240000000019));
#57079=CARTESIAN_POINT('',(-70.1759999999966,10.4219818659428,-11.4240000000023));
#57080=CARTESIAN_POINT('',(-70.1759999999966,10.4219818659428,-11.4240000000023));
#57081=CARTESIAN_POINT('Ctrl Pts',(-77.5415210531587,9.45904311830585,-5.6796370336054));
#57082=CARTESIAN_POINT('Ctrl Pts',(-77.0327642242293,10.707186890519,-5.4971857604248));
#57083=CARTESIAN_POINT('Ctrl Pts',(-76.5240071582721,11.95533075251,-5.31473468722646));
#57084=CARTESIAN_POINT('Ctrl Pts',(-76.0152503292933,13.2034745247418,-5.13228341408748));
#57085=CARTESIAN_POINT('Ctrl Pts',(-77.1255245937012,9.37017154437904,-6.23165809536591));
#57086=CARTESIAN_POINT('Ctrl Pts',(-76.6182066545349,10.6210013196209,-6.06058457490718));
#57087=CARTESIAN_POINT('Ctrl Pts',(-76.1128620314122,11.8710836770426,-5.8878461381967));
#57088=CARTESIAN_POINT('Ctrl Pts',(-75.6055445028749,13.1219132967538,-5.71677227128412));
#57089=CARTESIAN_POINT('Ctrl Pts',(-76.405465217238,9.19639822407867,-7.09347041402827));
#57090=CARTESIAN_POINT('Ctrl Pts',(-75.9110410562668,10.4500649957193,-6.91088111986312));
#57091=CARTESIAN_POINT('Ctrl Pts',(-75.4159945623941,11.7038171731561,-6.72934984943679));
#57092=CARTESIAN_POINT('Ctrl Pts',(-74.9215702719211,12.9574839625689,-6.54676077543671));
#57093=CARTESIAN_POINT('Ctrl Pts',(-74.9141341563532,8.89641968768657,-8.65752098839668));
#57094=CARTESIAN_POINT('Ctrl Pts',(-74.4693520068755,10.1574090917317,-8.39661857717499));
#57095=CARTESIAN_POINT('Ctrl Pts',(-74.0250205308659,11.4188757945292,-8.13395067151794));
#57096=CARTESIAN_POINT('Ctrl Pts',(-73.5802384751692,12.6798652978959,-7.873047892913));
#57097=CARTESIAN_POINT('Ctrl Pts',(-72.9631668562262,8.69637264444927,-10.4087281112213));
#57098=CARTESIAN_POINT('Ctrl Pts',(-72.599764363485,9.95227518704734,-10.0271076573509));
#57099=CARTESIAN_POINT('Ctrl Pts',(-72.236097993674,11.2068584385996,-9.64834004665345));
#57100=CARTESIAN_POINT('Ctrl Pts',(-71.8726954460223,12.4627607066652,-9.2667201864336));
#57101=CARTESIAN_POINT('Ctrl Pts',(-71.5045506975364,8.62838606863837,-11.4414060938779));
#57102=CARTESIAN_POINT('Ctrl Pts',(-71.1537252528359,9.88821257086177,-11.0687855431255));
#57103=CARTESIAN_POINT('Ctrl Pts',(-70.8024466765253,11.1521393493876,-10.6895493100031));
#57104=CARTESIAN_POINT('Ctrl Pts',(-70.4516211375321,12.411966704841,-10.3169273825877));
#57105=CARTESIAN_POINT('Ctrl Pts',(-70.7282794573195,8.51445269903683,-11.8926709016604));
#57106=CARTESIAN_POINT('Ctrl Pts',(-70.3600672197069,9.78599878287807,-11.5802995099963));
#57107=CARTESIAN_POINT('Ctrl Pts',(-69.9918550365244,11.057544374204,-11.2679289129904));
#57108=CARTESIAN_POINT('Ctrl Pts',(-69.623642798923,12.3290904579427,-10.9555575214917));
#57109=CARTESIAN_POINT('',(-76.7782566939679,11.3314434017562,-5.40599999999698));
#57110=CARTESIAN_POINT('Ctrl Pts',(-79.5980561168786,9.7948810259695,-1.92025417907612));
#57111=CARTESIAN_POINT('Ctrl Pts',(-79.0286226813552,11.015051365124,-1.72806356741562));
#57112=CARTESIAN_POINT('Ctrl Pts',(-78.4591892458318,12.2352217042785,-1.53587295575512));
#57113=CARTESIAN_POINT('Ctrl Pts',(-77.8897558103085,13.455392043433,-1.34368234409463));
#57114=CARTESIAN_POINT('Ctrl Pts',(-79.3926541200977,9.78652201900712,-2.47576181499884));
#57115=CARTESIAN_POINT('Ctrl Pts',(-78.8328950227455,11.0133203526859,-2.29743332344463));
#57116=CARTESIAN_POINT('Ctrl Pts',(-78.273415546693,12.240356547761,-2.11844736719906));
#57117=CARTESIAN_POINT('Ctrl Pts',(-77.713656387765,13.46715482906,-1.94011902042602));
#57118=CARTESIAN_POINT('Ctrl Pts',(-78.8071962567564,9.7034726253451,-3.78882461998114));
#57119=CARTESIAN_POINT('Ctrl Pts',(-78.2719624773854,10.9425576600723,-3.61894133239815));
#57120=CARTESIAN_POINT('Ctrl Pts',(-77.7366705145668,12.1816470179848,-3.44939658013833));
#57121=CARTESIAN_POINT('Ctrl Pts',(-77.2014367480084,13.4207320517599,-3.27951321800603));
#57122=CARTESIAN_POINT('Ctrl Pts',(-78.0251745283461,9.56134461172776,-5.02766395488251));
#57123=CARTESIAN_POINT('Ctrl Pts',(-77.5136242019621,10.8076044886706,-4.83982958167015));
#57124=CARTESIAN_POINT('Ctrl Pts',(-77.0020491726152,12.0537106468992,-4.65168259079091));
#57125=CARTESIAN_POINT('Ctrl Pts',(-76.4904988516711,13.2999705576926,-4.46384828642048));
#57126=CARTESIAN_POINT('Ctrl Pts',(-77.5413122691002,9.45942207531784,-5.67964638243143));
#57127=CARTESIAN_POINT('Ctrl Pts',(-77.0325525411905,10.7075737063638,-5.4971953741327));
#57128=CARTESIAN_POINT('Ctrl Pts',(-76.5237928132806,11.9557253374098,-5.31474436583398));
#57129=CARTESIAN_POINT('Ctrl Pts',(-76.0150330853708,13.2038769684557,-5.13229335753524));
#57130=CARTESIAN_POINT('',(-78.744,11.6249350354095,-1.632));
#57131=CARTESIAN_POINT('Ctrl Pts',(-23.8932545728999,0.740547902948747,
-53.9987504226491));
#57132=CARTESIAN_POINT('Ctrl Pts',(-23.86567132551,2.06698974342288,-53.6996164276723));
#57133=CARTESIAN_POINT('Ctrl Pts',(-23.8380880426163,3.39343157051117,-53.4004823892113));
#57134=CARTESIAN_POINT('Ctrl Pts',(-23.8105047952247,4.71987341098465,-53.1013483942324));
#57135=CARTESIAN_POINT('Ctrl Pts',(-23.8111491297826,0.66280895354329,-53.6616057058667));
#57136=CARTESIAN_POINT('Ctrl Pts',(-23.7899322073168,1.99428207452091,-53.3842279343313));
#57137=CARTESIAN_POINT('Ctrl Pts',(-23.7689959243087,3.32586100308869,-53.107193880104));
#57138=CARTESIAN_POINT('Ctrl Pts',(-23.7477790154882,4.65733412921086,-52.8298161252807));
#57139=CARTESIAN_POINT('Ctrl Pts',(-23.5120480269356,0.444631858653941,
-52.5958478954493));
#57140=CARTESIAN_POINT('Ctrl Pts',(-23.5131370234285,1.78958247655091,-52.3846028150775));
#57141=CARTESIAN_POINT('Ctrl Pts',(-23.5140290283712,3.13446261342227,-52.1731322226411));
#57142=CARTESIAN_POINT('Ctrl Pts',(-23.5151180152861,4.47941322789233,-51.9618871313045));
#57143=CARTESIAN_POINT('Ctrl Pts',(-22.9082077797905,0.265131218620393,
-51.1308970104399));
#57144=CARTESIAN_POINT('Ctrl Pts',(-22.9352266775722,1.61785129599896,-50.9898559415293));
#57145=CARTESIAN_POINT('Ctrl Pts',(-22.9623772841048,2.97056451761134,-50.8489070392546));
#57146=CARTESIAN_POINT('Ctrl Pts',(-22.9893961882904,4.32328459465657,-50.7078659748253));
#57147=CARTESIAN_POINT('Ctrl Pts',(-21.9019816170089,0.165924669481705,
-49.7679496219043));
#57148=CARTESIAN_POINT('Ctrl Pts',(-21.9246701219479,1.52140639652562,-49.6589009921318));
#57149=CARTESIAN_POINT('Ctrl Pts',(-21.947364036065,2.87689968849961,-49.5498132146386));
#57150=CARTESIAN_POINT('Ctrl Pts',(-21.9700525412669,4.23238141610583,-49.4407645829627));
#57151=CARTESIAN_POINT('Ctrl Pts',(-20.8891826568043,0.111651161782249,
-48.9120914269852));
#57152=CARTESIAN_POINT('Ctrl Pts',(-20.8974190589084,1.46770925485864,-48.8080765082637));
#57153=CARTESIAN_POINT('Ctrl Pts',(-20.9056860401831,2.82376475946175,-48.7041166196569));
#57154=CARTESIAN_POINT('Ctrl Pts',(-20.9139224437741,4.17982285241228,-48.6001017036111));
#57155=CARTESIAN_POINT('Ctrl Pts',(-19.7609227539775,0.06610415987474,-48.291627810693));
#57156=CARTESIAN_POINT('Ctrl Pts',(-19.7587290709853,1.42205329907346,-48.1863874960513));
#57157=CARTESIAN_POINT('Ctrl Pts',(-19.7564713684224,2.77801680439355,-48.081155633946));
#57158=CARTESIAN_POINT('Ctrl Pts',(-19.7542776823175,4.13396594429077,-47.9759153197152));
#57159=CARTESIAN_POINT('Ctrl Pts',(-18.7367225861336,0.0329100024412727,
-47.8927011046375));
#57160=CARTESIAN_POINT('Ctrl Pts',(-18.7339401998428,1.3890343296589,-47.7896347298988));
#57161=CARTESIAN_POINT('Ctrl Pts',(-18.7313776034358,2.74516423171156,-47.6867008588423));
#57162=CARTESIAN_POINT('Ctrl Pts',(-18.7285952278316,4.10128855920025,-47.5836344905461));
#57163=CARTESIAN_POINT('Ctrl Pts',(-18.0840673956984,0.0167299223542211,
-47.6824848396237));
#57164=CARTESIAN_POINT('Ctrl Pts',(-18.0827609388197,1.37305600404991,-47.5821464675806));
#57165=CARTESIAN_POINT('Ctrl Pts',(-18.081454453813,2.7293820850321,-47.4818080785799));
#57166=CARTESIAN_POINT('Ctrl Pts',(-18.0801479969329,4.08570816672776,-47.3814697065359));
#57167=CARTESIAN_POINT('',(-18.0821908984155,2.05127053807155,-47.5319999999985));
#57168=CARTESIAN_POINT('',(-18.0821908984155,2.05127053807155,-47.5319999999985));
#57169=CARTESIAN_POINT('',(-23.8518695172951,2.73025015572333,-53.5499999999992));
#57170=CARTESIAN_POINT('',(-18.0821908984155,2.05127053807155,-47.5319999999985));
#57171=CARTESIAN_POINT('Ctrl Pts',(-24.7799130650367,2.95812473554076,-60.3565443657526));
#57172=CARTESIAN_POINT('Ctrl Pts',(-24.6861686425761,4.20890666796298,-59.8308481219162));
#57173=CARTESIAN_POINT('Ctrl Pts',(-24.5924242201155,5.45968860038519,-59.3051518780799));
#57174=CARTESIAN_POINT('Ctrl Pts',(-24.4986797976549,6.71047053280741,-58.7794556342435));
#57175=CARTESIAN_POINT('Ctrl Pts',(-24.7093254167293,2.61894304809241,-59.562121477931));
#57176=CARTESIAN_POINT('Ctrl Pts',(-24.6146095582202,3.8738857913977,-59.0466983423777));
#57177=CARTESIAN_POINT('Ctrl Pts',(-24.5199709784907,5.12912618706156,-58.5313692759599));
#57178=CARTESIAN_POINT('Ctrl Pts',(-24.4252551199817,6.38406893036685,-58.0159461404066));
#57179=CARTESIAN_POINT('Ctrl Pts',(-24.5694830832048,2.04316650995158,-58.1763047923767));
#57180=CARTESIAN_POINT('Ctrl Pts',(-24.4795102446963,3.31055333878821,-57.6893014217856));
#57181=CARTESIAN_POINT('Ctrl Pts',(-24.3895173433111,4.5779209632356,-57.2023296900593));
#57182=CARTESIAN_POINT('Ctrl Pts',(-24.2995445048026,5.84530779207223,-56.7153263194681));
#57183=CARTESIAN_POINT('Ctrl Pts',(-24.3518230181499,1.42202438632593,-56.4243962709067));
#57184=CARTESIAN_POINT('Ctrl Pts',(-24.2821550992614,2.71319822602082,-56.0014370835227));
#57185=CARTESIAN_POINT('Ctrl Pts',(-24.212420350588,4.00418313586032,-55.5780865162234));
#57186=CARTESIAN_POINT('Ctrl Pts',(-24.1427524316995,5.29535697555521,-55.1551273288394));
#57187=CARTESIAN_POINT('Ctrl Pts',(-24.1714172775178,1.07110956737089,-55.2893749713734));
#57188=CARTESIAN_POINT('Ctrl Pts',(-24.1195415474074,2.37885367803318,-54.9184414382784));
#57189=CARTESIAN_POINT('Ctrl Pts',(-24.0676400333205,3.68664518346435,-54.5475126821782));
#57190=CARTESIAN_POINT('Ctrl Pts',(-24.0157643032102,4.99438929412664,-54.1765791490832));
#57191=CARTESIAN_POINT('Ctrl Pts',(-24.0036588764749,0.844289079598309,
-54.4481403827476));
#57192=CARTESIAN_POINT('Ctrl Pts',(-23.9673653219391,2.16453830185569,-54.1222935195884));
#57193=CARTESIAN_POINT('Ctrl Pts',(-23.9311137308229,3.48457569165273,-53.7961224777469));
#57194=CARTESIAN_POINT('Ctrl Pts',(-23.8948201762871,4.80482491391012,-53.4702756145878));
#57195=CARTESIAN_POINT('Ctrl Pts',(-23.8932421744747,0.740634811882228,
-53.9986859556407));
#57196=CARTESIAN_POINT('Ctrl Pts',(-23.8656604030216,2.06704504110963,-53.699561985213));
#57197=CARTESIAN_POINT('Ctrl Pts',(-23.8380786315686,3.39345527033703,-53.4004380147853));
#57198=CARTESIAN_POINT('Ctrl Pts',(-23.8104968601155,4.71986549956443,-53.1013140443576));
#57199=CARTESIAN_POINT('',(-24.6392964313458,4.83429763417409,-59.5679999999981));
#57200=CARTESIAN_POINT('Ctrl Pts',(-24.8514816439886,6.03933586362476,-66.5177940910004));
#57201=CARTESIAN_POINT('Ctrl Pts',(-24.8457871534356,7.24924543830288,-65.8966616404837));
#57202=CARTESIAN_POINT('Ctrl Pts',(-24.8400921747285,8.45915509270137,-65.275529378494));
#57203=CARTESIAN_POINT('Ctrl Pts',(-24.8343976842069,9.66906466737436,-64.6543969279651));
#57204=CARTESIAN_POINT('Ctrl Pts',(-24.9519005131634,5.40013434801617,-65.2717689951452));
#57205=CARTESIAN_POINT('Ctrl Pts',(-24.9326786072616,6.59873041285434,-64.6288206915467));
#57206=CARTESIAN_POINT('Ctrl Pts',(-24.9184337609038,7.79651367564351,-63.9839502278183));
#57207=CARTESIAN_POINT('Ctrl Pts',(-24.8992115344816,8.99510979282575,-63.341002048006));
#57208=CARTESIAN_POINT('Ctrl Pts',(-24.955193873487,4.48978712507474,-63.5721497671119));
#57209=CARTESIAN_POINT('Ctrl Pts',(-24.8978913410139,5.69561205548002,-62.9450648497406));
#57210=CARTESIAN_POINT('Ctrl Pts',(-24.840394330803,6.90143304615417,-62.318020459864));
#57211=CARTESIAN_POINT('Ctrl Pts',(-24.7830918108543,8.10725797681316,-61.6909355398828));
#57212=CARTESIAN_POINT('Ctrl Pts',(-24.9193282160013,4.02246798717194,-62.6314379535427));
#57213=CARTESIAN_POINT('Ctrl Pts',(-24.8479165191087,5.2381550017438,-62.0258687577014));
#57214=CARTESIAN_POINT('Ctrl Pts',(-24.7768538140445,6.45354203486205,-61.4196009992347));
#57215=CARTESIAN_POINT('Ctrl Pts',(-24.7054420946769,7.66922906875258,-60.8140318483805));
#57216=CARTESIAN_POINT('Ctrl Pts',(-24.9088241241943,3.89449030749864,-62.3747837256354));
#57217=CARTESIAN_POINT('Ctrl Pts',(-24.8333191742452,5.11298267792579,-61.7753555460744));
#57218=CARTESIAN_POINT('Ctrl Pts',(-24.7581355545957,6.33163360070118,-61.1762619544598));
#57219=CARTESIAN_POINT('Ctrl Pts',(-24.682630583953,7.55012596091763,-60.5768337533516));
#57220=CARTESIAN_POINT('Ctrl Pts',(-24.9003852832803,3.80179791434547,-62.1865158010774));
#57221=CARTESIAN_POINT('Ctrl Pts',(-24.8221913397055,5.02260346864682,-61.592168571107));
#57222=CARTESIAN_POINT('Ctrl Pts',(-24.7442452372017,6.24340817620379,-60.9977988992182));
#57223=CARTESIAN_POINT('Ctrl Pts',(-24.666051277666,7.46421373055968,-60.403451670693));
#57224=CARTESIAN_POINT('Ctrl Pts',(-24.8848681816847,3.64819007810987,-61.8717738157264));
#57225=CARTESIAN_POINT('Ctrl Pts',(-24.802362419227,4.87306103722246,-61.2863881627958));
#57226=CARTESIAN_POINT('Ctrl Pts',(-24.7201086021799,6.09797862128327,-60.7010879047467));
#57227=CARTESIAN_POINT('Ctrl Pts',(-24.637602823497,7.32284957739323,-60.1157022463168));
#57228=CARTESIAN_POINT('Ctrl Pts',(-24.8483417886798,3.34833875688338,-61.2421817255175));
#57229=CARTESIAN_POINT('Ctrl Pts',(-24.758735472489,4.58246016741107,-60.6774045777714));
#57230=CARTESIAN_POINT('Ctrl Pts',(-24.6692623550833,5.81657910544939,-60.112615896231));
#57231=CARTESIAN_POINT('Ctrl Pts',(-24.5796560303146,7.05070051613632,-59.5478387492278));
#57232=CARTESIAN_POINT('Ctrl Pts',(-24.8095494386071,3.11146053772572,-60.716090603378));
#57233=CARTESIAN_POINT('Ctrl Pts',(-24.7166187762756,4.35508116577155,-60.173124017711));
#57234=CARTESIAN_POINT('Ctrl Pts',(-24.6236575971476,5.59875733363374,-59.6302142613489));
#57235=CARTESIAN_POINT('Ctrl Pts',(-24.5307269367814,6.84237795810284,-59.0872476720221));
#57236=CARTESIAN_POINT('Ctrl Pts',(-24.779910160927,2.95810970987412,-60.3565091331962));
#57237=CARTESIAN_POINT('Ctrl Pts',(-24.6861626398759,4.20893262287472,-59.8307976527483));
#57238=CARTESIAN_POINT('Ctrl Pts',(-24.5924151218147,5.45975553043318,-59.3050861667321));
#57239=CARTESIAN_POINT('Ctrl Pts',(-24.4986676007634,6.71057844343413,-58.7793746862846));
#57240=CARTESIAN_POINT('',(-24.8429480415422,7.85407743444482,-65.5860000000009));
#57241=CARTESIAN_POINT('Ctrl Pts',(-23.6734819284749,9.24326495191836,-72.5612011682599));
#57242=CARTESIAN_POINT('Ctrl Pts',(-23.6736392512832,10.4442582200649,-71.9230670560889));
#57243=CARTESIAN_POINT('Ctrl Pts',(-23.6737965740915,11.6452514882115,-71.284932943918));
#57244=CARTESIAN_POINT('Ctrl Pts',(-23.6739538968997,12.846244756358,-70.6467988317471));
#57245=CARTESIAN_POINT('Ctrl Pts',(-23.7649042668809,9.0816244028814,-72.257009894464));
#57246=CARTESIAN_POINT('Ctrl Pts',(-23.7650247809087,10.2820560268017,-71.6178191935096));
#57247=CARTESIAN_POINT('Ctrl Pts',(-23.7651416433926,11.482505712744,-70.9786611152447));
#57248=CARTESIAN_POINT('Ctrl Pts',(-23.7652621574204,12.6829373366643,-70.3394704142904));
#57249=CARTESIAN_POINT('Ctrl Pts',(-24.026191926212,8.5949110125477,-71.3440354252429));
#57250=CARTESIAN_POINT('Ctrl Pts',(-24.026490117635,9.79400808195901,-70.7023415912864));
#57251=CARTESIAN_POINT('Ctrl Pts',(-24.0267840819686,10.9930931283153,-70.0606258912063));
#57252=CARTESIAN_POINT('Ctrl Pts',(-24.0270822733915,12.1921901977266,-69.4189320572497));
#57253=CARTESIAN_POINT('Ctrl Pts',(-24.3676733444401,7.85042242107576,-69.9555629639005));
#57254=CARTESIAN_POINT('Ctrl Pts',(-24.3702647663561,9.04908783302253,-69.3130728922147));
#57255=CARTESIAN_POINT('Ctrl Pts',(-24.3726957523222,10.2477966114829,-68.6706626248404));
#57256=CARTESIAN_POINT('Ctrl Pts',(-24.3752871742381,11.4464620234297,-68.0281725531546));
#57257=CARTESIAN_POINT('Ctrl Pts',(-24.6786062061593,6.94797749971677,-68.2666525661597));
#57258=CARTESIAN_POINT('Ctrl Pts',(-24.6833099022124,8.14979165663938,-67.6300522330398));
#57259=CARTESIAN_POINT('Ctrl Pts',(-24.6880297408764,9.35159646931981,-66.9934315143023));
#57260=CARTESIAN_POINT('Ctrl Pts',(-24.6927334369296,10.5534106262424,-66.3568311811825));
#57261=CARTESIAN_POINT('Ctrl Pts',(-24.8079585801581,6.32785027214234,-67.080190599109));
#57262=CARTESIAN_POINT('Ctrl Pts',(-24.8075961665432,7.53482759926113,-66.4533978140702));
#57263=CARTESIAN_POINT('Ctrl Pts',(-24.8067625026745,8.74190348924563,-65.8267881673147));
#57264=CARTESIAN_POINT('Ctrl Pts',(-24.8064000890597,9.94888081636442,-65.1999953822759));
#57265=CARTESIAN_POINT('Ctrl Pts',(-24.8514914924163,6.0392731730085,-66.5176718854411));
#57266=CARTESIAN_POINT('Ctrl Pts',(-24.8457958585002,7.24914268063271,-65.8965572951477));
#57267=CARTESIAN_POINT('Ctrl Pts',(-24.8401002245841,8.45901218825693,-65.2754427048542));
#57268=CARTESIAN_POINT('Ctrl Pts',(-24.834404590668,9.66888169588114,-64.6543281145607));
#57269=CARTESIAN_POINT('',(-23.6737179126873,11.0447548541382,-71.6040000000035));
#57270=CARTESIAN_POINT('Ctrl Pts',(-21.0430574415816,12.4421901739772,-78.5797217830362));
#57271=CARTESIAN_POINT('Ctrl Pts',(-21.042167498106,13.642998643172,-77.9412405943464));
#57272=CARTESIAN_POINT('Ctrl Pts',(-21.0412775546305,14.8438071123667,-77.3027594056566));
#57273=CARTESIAN_POINT('Ctrl Pts',(-21.040387611155,16.0446155815615,-76.6642782169667));
#57274=CARTESIAN_POINT('Ctrl Pts',(-21.3778021402842,12.1976961752275,-78.1194288669213));
#57275=CARTESIAN_POINT('Ctrl Pts',(-21.3769081685314,13.3985041597138,-77.4809467730066));
#57276=CARTESIAN_POINT('Ctrl Pts',(-21.3760224274111,14.5993118579,-76.8424641268745));
#57277=CARTESIAN_POINT('Ctrl Pts',(-21.3751284556584,15.8001198423863,-76.2039820329599));
#57278=CARTESIAN_POINT('Ctrl Pts',(-21.9881636463861,11.644899047288,-77.0789580092169));
#57279=CARTESIAN_POINT('Ctrl Pts',(-21.9873817766374,12.8457004437947,-76.4404633549307));
#57280=CARTESIAN_POINT('Ctrl Pts',(-21.986615227335,14.0465025180761,-75.8019699506747));
#57281=CARTESIAN_POINT('Ctrl Pts',(-21.9858333575863,15.2473039145829,-75.1634752963886));
#57282=CARTESIAN_POINT('Ctrl Pts',(-22.84310382117,10.6110321918245,-75.1338794942987));
#57283=CARTESIAN_POINT('Ctrl Pts',(-22.8428530090605,11.811809075809,-74.4953382081582));
#57284=CARTESIAN_POINT('Ctrl Pts',(-22.8426022779187,13.0125856498721,-73.8567963290241));
#57285=CARTESIAN_POINT('Ctrl Pts',(-22.8423514658093,14.2133625338566,-73.2182550428836));
#57286=CARTESIAN_POINT('Ctrl Pts',(-23.3878046917012,9.75120273870573,-73.5170894484657));
#57287=CARTESIAN_POINT('Ctrl Pts',(-23.3880652364971,10.9520370262507,-72.8786561872709));
#57288=CARTESIAN_POINT('Ctrl Pts',(-23.3883718428281,12.1528739545353,-72.2402278077585));
#57289=CARTESIAN_POINT('Ctrl Pts',(-23.3886323876239,13.3537082420802,-71.6017945465636));
#57290=CARTESIAN_POINT('Ctrl Pts',(-23.6734819284749,9.24326495191836,-72.5612011682599));
#57291=CARTESIAN_POINT('Ctrl Pts',(-23.6736392512832,10.4442582200649,-71.9230670560889));
#57292=CARTESIAN_POINT('Ctrl Pts',(-23.6737965740915,11.6452514882115,-71.284932943918));
#57293=CARTESIAN_POINT('Ctrl Pts',(-23.6739538968997,12.846244756358,-70.6467988317471));
#57294=CARTESIAN_POINT('',(-21.0417225263683,14.2434028777694,-77.6220000000015));
#57295=CARTESIAN_POINT('Ctrl Pts',(-20.809321916529,12.6047206302969,-78.8857217870086));
#57296=CARTESIAN_POINT('Ctrl Pts',(-20.808440638843,13.8055291044742,-78.2472405956695));
#57297=CARTESIAN_POINT('Ctrl Pts',(-20.807559361157,15.0063375786514,-77.6087594043305));
#57298=CARTESIAN_POINT('Ctrl Pts',(-20.806678083471,16.2071460528287,-76.9702782129914));
#57299=CARTESIAN_POINT('Ctrl Pts',(-20.8889387648524,12.5520952777272,-78.7866380007792));
#57300=CARTESIAN_POINT('Ctrl Pts',(-20.8880519500474,13.7529037487349,-78.1481568111254));
#57301=CARTESIAN_POINT('Ctrl Pts',(-20.8871651385933,14.953712219749,-77.5096756214682));
#57302=CARTESIAN_POINT('Ctrl Pts',(-20.8862783237883,16.1545206907567,-76.8711944318144));
#57303=CARTESIAN_POINT('Ctrl Pts',(-20.966829204766,12.4978666722846,-78.6845402972071));
#57304=CARTESIAN_POINT('Ctrl Pts',(-20.965939552898,13.6986751416463,-78.0460591084285));
#57305=CARTESIAN_POINT('Ctrl Pts',(-20.965049904181,14.8994836110143,-77.4075779196465));
#57306=CARTESIAN_POINT('Ctrl Pts',(-20.964160252313,16.1002920803761,-76.7690967308679));
#57307=CARTESIAN_POINT('Ctrl Pts',(-21.0430574415815,12.4421901739772,-78.5797217830362));
#57308=CARTESIAN_POINT('Ctrl Pts',(-21.042167498106,13.642998643172,-77.9412405943464));
#57309=CARTESIAN_POINT('Ctrl Pts',(-21.0412775546305,14.8438071123667,-77.3027594056565));
#57310=CARTESIAN_POINT('Ctrl Pts',(-21.040387611155,16.0446155815615,-76.6642782169667));
#57311=CARTESIAN_POINT('',(-20.808,14.4059333415628,-77.928));
#57312=CARTESIAN_POINT('Ctrl Pts',(23.6734819284753,9.2432649519181,-72.5612011682563));
#57313=CARTESIAN_POINT('Ctrl Pts',(23.6736392516143,10.4442607414065,-71.9230657163991));
#57314=CARTESIAN_POINT('Ctrl Pts',(23.6737965747534,11.6452565308947,-71.2849302645419));
#57315=CARTESIAN_POINT('Ctrl Pts',(23.6739538978923,12.8462523203831,-70.6467948126847));
#57316=CARTESIAN_POINT('Ctrl Pts',(23.5615106118548,9.44235138733137,-72.9358619934788));
#57317=CARTESIAN_POINT('Ctrl Pts',(23.5617208320191,10.6432845725721,-72.2976087481736));
#57318=CARTESIAN_POINT('Ctrl Pts',(23.5619117889063,11.8442196676616,-71.6593590410948));
#57319=CARTESIAN_POINT('Ctrl Pts',(23.5621220091515,13.0451528528943,-71.0211057957747));
#57320=CARTESIAN_POINT('Ctrl Pts',(23.2106747185919,10.0332017364569,-74.0473320232884));
#57321=CARTESIAN_POINT('Ctrl Pts',(23.2107881218931,11.2340121859773,-73.4088478072317));
#57322=CARTESIAN_POINT('Ctrl Pts',(23.2109141600603,12.4348203100041,-72.7703592264185));
#57323=CARTESIAN_POINT('Ctrl Pts',(23.2110275633084,13.6356307595342,-72.1318750103799));
#57324=CARTESIAN_POINT('Ctrl Pts',(22.4162563803382,11.1958361188247,-76.2337986537702));
#57325=CARTESIAN_POINT('Ctrl Pts',(22.4156559127772,12.396613745026,-75.5952528536972));
#57326=CARTESIAN_POINT('Ctrl Pts',(22.4150306235993,13.5973972303885,-74.9567180648474));
#57327=CARTESIAN_POINT('Ctrl Pts',(22.4144301561425,14.7981748565652,-74.3181722647281));
#57328=CARTESIAN_POINT('Ctrl Pts',(21.6377011779931,12.0078686581778,-77.7620529729162));
#57329=CARTESIAN_POINT('Ctrl Pts',(21.6367967414816,13.208683760128,-77.1235782253732));
#57330=CARTESIAN_POINT('Ctrl Pts',(21.6359289318972,14.4094834349257,-76.4850743279567));
#57331=CARTESIAN_POINT('Ctrl Pts',(21.6350244952319,15.6102985369408,-75.8465995805361));
#57332=CARTESIAN_POINT('Ctrl Pts',(21.0430574415837,12.442190173977,-78.5797217830346));
#57333=CARTESIAN_POINT('Ctrl Pts',(21.0421674962392,13.6430011641255,-77.9412392539299));
#57334=CARTESIAN_POINT('Ctrl Pts',(21.0412775508946,14.843812154274,-77.3027567248251));
#57335=CARTESIAN_POINT('Ctrl Pts',(21.0403876055502,16.0446231444226,-76.6642741957204));
#57336=CARTESIAN_POINT('',(21.0417225263694,14.2434028777691,-77.6219999999999));
#57337=CARTESIAN_POINT('',(23.6737179126884,11.0447548541379,-71.6039999999999));
#57338=CARTESIAN_POINT('Ctrl Pts',(24.8514914924156,6.03927317300853,-66.5176718854405));
#57339=CARTESIAN_POINT('Ctrl Pts',(24.8457958585,7.24914268063269,-65.8965572951469));
#57340=CARTESIAN_POINT('Ctrl Pts',(24.8401002245844,8.45901218825685,-65.2754427048533));
#57341=CARTESIAN_POINT('Ctrl Pts',(24.8344045906688,9.66888169588101,-64.6543281145597));
#57342=CARTESIAN_POINT('Ctrl Pts',(24.7857582030557,6.47501525815644,-67.3670569474013));
#57343=CARTESIAN_POINT('Ctrl Pts',(24.7880943840847,7.68057023012441,-66.73749583644));
#57344=CARTESIAN_POINT('Ctrl Pts',(24.7897825180673,8.88611633876867,-66.1078291491835));
#57345=CARTESIAN_POINT('Ctrl Pts',(24.7921186990963,10.0916713107366,-65.4782680382222));
#57346=CARTESIAN_POINT('Ctrl Pts',(24.550338270654,7.4900405053709,-69.2911770386706));
#57347=CARTESIAN_POINT('Ctrl Pts',(24.5559989571534,8.68780867473477,-68.6470021875378));
#57348=CARTESIAN_POINT('Ctrl Pts',(24.5610779768368,9.88549730957243,-68.0027096389216));
#57349=CARTESIAN_POINT('Ctrl Pts',(24.5667386633363,11.0832654789363,-67.3585347877888));
#57350=CARTESIAN_POINT('Ctrl Pts',(24.0160972599616,8.6374991045811,-71.4212107028606));
#57351=CARTESIAN_POINT('Ctrl Pts',(24.0154309216262,9.83632107354304,-70.7789993845374));
#57352=CARTESIAN_POINT('Ctrl Pts',(24.0168080472231,11.0354101577888,-70.1372628915936));
#57353=CARTESIAN_POINT('Ctrl Pts',(24.0161417088878,12.2342321267508,-69.4950515732704));
#57354=CARTESIAN_POINT('Ctrl Pts',(23.6734819284753,9.2432649519181,-72.5612011682563));
#57355=CARTESIAN_POINT('Ctrl Pts',(23.673639251284,10.4442582200647,-71.9230670560853));
#57356=CARTESIAN_POINT('Ctrl Pts',(23.6737965740928,11.6452514882112,-71.2849329439144));
#57357=CARTESIAN_POINT('Ctrl Pts',(23.6739538969015,12.8462447563578,-70.6467988317435));
#57358=CARTESIAN_POINT('',(24.8429480415422,7.85407743444477,-65.5860000000001));
#57359=CARTESIAN_POINT('Ctrl Pts',(24.7799191277205,2.95792794530187,-60.3565375266123));
#57360=CARTESIAN_POINT('Ctrl Pts',(24.6861703694341,4.20876617277843,-59.8308217469595));
#57361=CARTESIAN_POINT('Ctrl Pts',(24.5924217855773,5.45960447146532,-59.3051063962421));
#57362=CARTESIAN_POINT('Ctrl Pts',(24.4986730273061,6.71044269894815,-58.7793906166268));
#57363=CARTESIAN_POINT('Ctrl Pts',(24.9089035260939,3.62528183199708,-61.9213719956554));
#57364=CARTESIAN_POINT('Ctrl Pts',(24.8198633370479,4.8453463929819,-61.3235933669262));
#57365=CARTESIAN_POINT('Ctrl Pts',(24.7272287916051,6.06394357005601,-60.7169759429534));
#57366=CARTESIAN_POINT('Ctrl Pts',(24.6381882876209,7.28400800246834,-60.1191965397671));
#57367=CARTESIAN_POINT('Ctrl Pts',(24.9834159830366,4.731838028036,-64.0136175321612));
#57368=CARTESIAN_POINT('Ctrl Pts',(24.9383372996939,5.93153728641096,-63.3748948329307));
#57369=CARTESIAN_POINT('Ctrl Pts',(24.8942407363303,7.13166149255805,-62.7389258132719));
#57370=CARTESIAN_POINT('Ctrl Pts',(24.8491621390411,8.33136078816702,-62.1002033553194));
#57371=CARTESIAN_POINT('Ctrl Pts',(24.9107202843689,5.66209961304811,-65.7828228049932));
#57372=CARTESIAN_POINT('Ctrl Pts',(24.8976557677923,6.8651069265034,-65.1478601922165));
#57373=CARTESIAN_POINT('Ctrl Pts',(24.8856952678506,8.06836234662063,-64.5146251843238));
#57374=CARTESIAN_POINT('Ctrl Pts',(24.8726308480082,9.27136968181508,-63.8796627229203));
#57375=CARTESIAN_POINT('Ctrl Pts',(24.8514884085996,6.03913854124118,-66.5178010814603));
#57376=CARTESIAN_POINT('Ctrl Pts',(24.8457930019507,7.24906150548085,-65.8966601719787));
#57377=CARTESIAN_POINT('Ctrl Pts',(24.8400975238651,8.45898445366638,-65.2755191507098));
#57378=CARTESIAN_POINT('Ctrl Pts',(24.8344021172099,9.66890741790464,-64.6543782412184));
#57379=CARTESIAN_POINT('',(24.639296431346,4.83429763417431,-59.5679999999998));
#57380=CARTESIAN_POINT('Ctrl Pts',(23.8932421744751,0.740634811882458,-53.9986859556419));
#57381=CARTESIAN_POINT('Ctrl Pts',(23.8656593284557,2.06709671711524,-53.6995503315557));
#57382=CARTESIAN_POINT('Ctrl Pts',(23.8380764824361,3.39355862234801,-53.4004147074695));
#57383=CARTESIAN_POINT('Ctrl Pts',(23.8104936364166,4.7200205275808,-53.1012790833832));
#57384=CARTESIAN_POINT('Ctrl Pts',(24.1789074622363,1.00880462386192,-55.1614948960392));
#57385=CARTESIAN_POINT('Ctrl Pts',(24.1277458282354,2.31879778942141,-54.7919563810276));
#57386=CARTESIAN_POINT('Ctrl Pts',(24.0798103811834,3.62982881878404,-54.4253709231687));
#57387=CARTESIAN_POINT('Ctrl Pts',(24.0286484958026,4.93982190347465,-54.0558321780592));
#57388=CARTESIAN_POINT('Ctrl Pts',(24.4015168304308,1.52786212045763,-56.7701588656369));
#57389=CARTESIAN_POINT('Ctrl Pts',(24.3255448890141,2.81314050207022,-56.3301388554163));
#57390=CARTESIAN_POINT('Ctrl Pts',(24.2496983734156,4.09850722836944,-55.8901826689679));
#57391=CARTESIAN_POINT('Ctrl Pts',(24.173726422226,5.38378560309834,-55.4501626537743));
#57392=CARTESIAN_POINT('Ctrl Pts',(24.6106655417996,2.23012064092564,-58.6108222610336));
#57393=CARTESIAN_POINT('Ctrl Pts',(24.5199407290614,3.49401760823125,-58.1162740526191));
#57394=CARTESIAN_POINT('Ctrl Pts',(24.4296363415329,4.75814275026669,-57.6224267085783));
#57395=CARTESIAN_POINT('Ctrl Pts',(24.3389114960358,6.02203969979325,-57.1278784455535));
#57396=CARTESIAN_POINT('Ctrl Pts',(24.6996147992407,2.59058304170841,-59.488342199932));
#57397=CARTESIAN_POINT('Ctrl Pts',(24.6057756690561,3.84681036908307,-58.9756997363143));
#57398=CARTESIAN_POINT('Ctrl Pts',(24.5118615880014,5.10287355736105,-58.4625429317005));
#57399=CARTESIAN_POINT('Ctrl Pts',(24.418022463657,6.35910089752518,-57.9499005081595));
#57400=CARTESIAN_POINT('Ctrl Pts',(24.7614059735443,2.86919605364059,-60.1482578252368));
#57401=CARTESIAN_POINT('Ctrl Pts',(24.667356476118,4.12105401998294,-59.6249836943641));
#57402=CARTESIAN_POINT('Ctrl Pts',(24.5734673948942,5.37318097339444,-59.1024871867851));
#57403=CARTESIAN_POINT('Ctrl Pts',(24.4794178849684,6.6250389187777,-58.5792129953211));
#57404=CARTESIAN_POINT('Ctrl Pts',(24.7799130650375,2.95812473554106,-60.3565443657544));
#57405=CARTESIAN_POINT('Ctrl Pts',(24.68616499036,4.2089553975436,-59.8308276411638));
#57406=CARTESIAN_POINT('Ctrl Pts',(24.5924169156826,5.45978605954612,-59.305110916573));
#57407=CARTESIAN_POINT('Ctrl Pts',(24.498668841005,6.71061672154866,-58.7793941919824));
#57408=CARTESIAN_POINT('',(23.8518695172954,2.73025015572356,-53.5500000000004));
#57409=CARTESIAN_POINT('Ctrl Pts',(18.0841396805929,0.0168146404897664,
-47.6825020134366));
#57410=CARTESIAN_POINT('Ctrl Pts',(18.0828330780895,1.3731194054854,-47.5821649137338));
#57411=CARTESIAN_POINT('Ctrl Pts',(18.081526479321,2.72942417022187,-47.4818278133018));
#57412=CARTESIAN_POINT('Ctrl Pts',(18.0802198768176,4.08572893521751,-47.3814907135991));
#57413=CARTESIAN_POINT('Ctrl Pts',(18.5443648070833,0.0282243501846493,
-47.8307394400169));
#57414=CARTESIAN_POINT('Ctrl Pts',(18.5421205699259,1.38438459857093,-47.7284998708658));
#57415=CARTESIAN_POINT('Ctrl Pts',(18.5397222302431,2.74055553971965,-47.6262903896664));
#57416=CARTESIAN_POINT('Ctrl Pts',(18.5374779933162,4.09671578808994,-47.5240508204702));
#57417=CARTESIAN_POINT('Ctrl Pts',(19.3713825374723,0.0528487038591615,
-48.1299992700489));
#57418=CARTESIAN_POINT('Ctrl Pts',(19.3683888317819,1.40882529369436,-48.0252908017089));
#57419=CARTESIAN_POINT('Ctrl Pts',(19.365563708298,2.76479677687121,-47.920635084255));
#57420=CARTESIAN_POINT('Ctrl Pts',(19.3625700023554,4.12077336671404,-47.8159266158361));
#57421=CARTESIAN_POINT('Ctrl Pts',(20.3970287176425,0.0913850843528481,
-48.6274441293917));
#57422=CARTESIAN_POINT('Ctrl Pts',(20.4001722793646,1.44737071048997,-48.5228840106449));
#57423=CARTESIAN_POINT('Ctrl Pts',(20.4031843891888,2.80336002413669,-48.4183208296279));
#57424=CARTESIAN_POINT('Ctrl Pts',(20.4063279511075,4.1593456502683,-48.3137607108857));
#57425=CARTESIAN_POINT('Ctrl Pts',(21.2030623279049,0.127765179000182,-49.1632061443352));
#57426=CARTESIAN_POINT('Ctrl Pts',(21.2157420402905,1.48366970427005,-49.0580958545386));
#57427=CARTESIAN_POINT('Ctrl Pts',(21.2284906751219,2.83956742651729,-48.9530453801162));
#57428=CARTESIAN_POINT('Ctrl Pts',(21.2411703874045,4.19547195179733,-48.8479350902301));
#57429=CARTESIAN_POINT('Ctrl Pts',(21.9415244226505,0.170818208138083,-49.8301345883609));
#57430=CARTESIAN_POINT('Ctrl Pts',(21.9642269284021,1.52612482082818,-49.7193172627231));
#57431=CARTESIAN_POINT('Ctrl Pts',(21.9868032115003,2.88143737386752,-49.6085370939327));
#57432=CARTESIAN_POINT('Ctrl Pts',(22.0095057174407,4.23674398654873,-49.4977197682393));
#57433=CARTESIAN_POINT('Ctrl Pts',(22.7299618914328,0.246693032010643,-50.877466594607));
#57434=CARTESIAN_POINT('Ctrl Pts',(22.7563638685511,1.59993105501455,-50.7426800809163));
#57435=CARTESIAN_POINT('Ctrl Pts',(22.7826599837655,2.95314572641759,-50.6077394381178));
#57436=CARTESIAN_POINT('Ctrl Pts',(22.8090619610422,4.30638374945642,-50.4729529246576));
#57437=CARTESIAN_POINT('Ctrl Pts',(23.4121500524248,0.405565211479381,-52.3094090691719));
#57438=CARTESIAN_POINT('Ctrl Pts',(23.4198394420821,1.75224322857291,-52.1135550169374));
#57439=CARTESIAN_POINT('Ctrl Pts',(23.427563745456,3.09892933740634,-51.9177173826107));
#57440=CARTESIAN_POINT('Ctrl Pts',(23.4352531350609,4.44560735448777,-51.7218633303516));
#57441=CARTESIAN_POINT('Ctrl Pts',(23.7490678075399,0.604114032031964,-53.4066787177267));
#57442=CARTESIAN_POINT('Ctrl Pts',(23.7328855382795,1.93947127745986,-53.1461836033946));
#57443=CARTESIAN_POINT('Ctrl Pts',(23.7165336536041,3.27471109737415,-52.8850050076064));
#57444=CARTESIAN_POINT('Ctrl Pts',(23.7003513845974,4.61006834297765,-52.6245098942964));
#57445=CARTESIAN_POINT('Ctrl Pts',(23.8932460088521,0.740622488142717,-53.9987038928088));
#57446=CARTESIAN_POINT('Ctrl Pts',(23.8656637224211,2.06704392239731,-53.6995764062096));
#57447=CARTESIAN_POINT('Ctrl Pts',(23.8380814401183,3.39346535950986,-53.4004489362454));
#57448=CARTESIAN_POINT('Ctrl Pts',(23.8104991536872,4.71988679376446,-53.1013214496463));
#57449=CARTESIAN_POINT('',(18.0821908984197,2.05127053807158,-47.5319999999999));
#57450=CARTESIAN_POINT('',(18.0821908984197,2.05127053807158,-47.5319999999999));
#57451=CARTESIAN_POINT('',(18.0821908984197,2.05127053807158,-47.5319999999999));
#57452=CARTESIAN_POINT('Ctrl Pts',(-3.2690524243696E-5,-0.0251265829928964,
-45.4192965823161));
#57453=CARTESIAN_POINT('Ctrl Pts',(-3.27354186043915E-5,1.33471801276171,
-45.4405652637787));
#57454=CARTESIAN_POINT('Ctrl Pts',(-3.27175351009904E-5,2.69456260844022,
-45.4618339363921));
#57455=CARTESIAN_POINT('Ctrl Pts',(-3.27624304691016E-5,4.05440720419482,
-45.4831026178549));
#57456=CARTESIAN_POINT('Ctrl Pts',(1.8682027887804,-0.0257296837108507,
-45.4578603912295));
#57457=CARTESIAN_POINT('Ctrl Pts',(1.87076844273175,1.33412472643363,-45.4782403258505));
#57458=CARTESIAN_POINT('Ctrl Pts',(1.86974641330836,2.69398348477606,-45.4991259855145));
#57459=CARTESIAN_POINT('Ctrl Pts',(1.87231212483236,4.05383789485077,-45.51950591202));
#57460=CARTESIAN_POINT('Ctrl Pts',(4.99153621662472,-0.0330411951959642,
-45.534798185463));
#57461=CARTESIAN_POINT('Ctrl Pts',(4.9932336251418,1.32683289940186,-45.5543492662237));
#57462=CARTESIAN_POINT('Ctrl Pts',(4.99497908362866,2.68670867600787,-45.5738691487411));
#57463=CARTESIAN_POINT('Ctrl Pts',(4.99667649137468,4.0465827705787,-45.5934202300024));
#57464=CARTESIAN_POINT('Ctrl Pts',(7.59438888123013,-0.0326758765092276,
-45.6867097257879));
#57465=CARTESIAN_POINT('Ctrl Pts',(7.59249880785721,1.32724755035341,-45.7021384549768));
#57466=CARTESIAN_POINT('Ctrl Pts',(7.59047347647672,2.68717345156613,-45.7176245959044));
#57467=CARTESIAN_POINT('Ctrl Pts',(7.58858340527433,4.04709687838906,-45.733053324172));
#57468=CARTESIAN_POINT('Ctrl Pts',(8.87729659300802,-0.0314509584309369,
-45.7887336658147));
#57469=CARTESIAN_POINT('Ctrl Pts',(8.87441777432724,1.3285062657543,-45.8007152975604));
#57470=CARTESIAN_POINT('Ctrl Pts',(8.87155087449128,2.68846580175383,-45.8126919130268));
#57471=CARTESIAN_POINT('Ctrl Pts',(8.86867205561924,4.04842302590197,-45.8246735448531));
#57472=CARTESIAN_POINT('Ctrl Pts',(10.1490597186576,-0.0297979816701636,
-45.9251950972821));
#57473=CARTESIAN_POINT('Ctrl Pts',(10.1465580226243,1.33020253676551,-45.9314329040811));
#57474=CARTESIAN_POINT('Ctrl Pts',(10.1440412110529,2.69020835929771,-45.9377490875431));
#57475=CARTESIAN_POINT('Ctrl Pts',(10.1415395152622,4.05020887764826,-45.9439868930844));
#57476=CARTESIAN_POINT('Ctrl Pts',(11.8978630897578,-0.0280707333736627,
-46.1680533783691));
#57477=CARTESIAN_POINT('Ctrl Pts',(11.8982432356438,1.33196096673256,-46.1620867040576));
#57478=CARTESIAN_POINT('Ctrl Pts',(11.898750185013,2.69199259656723,-46.1560178387715));
#57479=CARTESIAN_POINT('Ctrl Pts',(11.8991303288642,4.05202429667458,-46.1500511660999));
#57480=CARTESIAN_POINT('Ctrl Pts',(13.9971210552705,-0.0295760205187906,
-46.5641348045042));
#57481=CARTESIAN_POINT('Ctrl Pts',(14.0040786793423,1.33022743179417,-46.5331292464512));
#57482=CARTESIAN_POINT('Ctrl Pts',(14.0114201033648,2.69005785826174,-46.5023729377843));
#57483=CARTESIAN_POINT('Ctrl Pts',(14.0183777212778,4.04986131014184,-46.4713673757315));
#57484=CARTESIAN_POINT('Ctrl Pts',(16.2942313977893,-0.0209121707010144,
-47.1212911897684));
#57485=CARTESIAN_POINT('Ctrl Pts',(16.2992203099862,1.33750106368331,-47.0520421334878));
#57486=CARTESIAN_POINT('Ctrl Pts',(16.3037485306264,2.69589336048563,-46.9826958057665));
#57487=CARTESIAN_POINT('Ctrl Pts',(16.3087374502163,4.05430659520594,-46.9134467510469));
#57488=CARTESIAN_POINT('Ctrl Pts',(17.5354503382007,0.00240667102759995,
-47.4946713071985));
#57489=CARTESIAN_POINT('Ctrl Pts',(17.5350963620415,1.35941127856638,-47.4038531728718));
#57490=CARTESIAN_POINT('Ctrl Pts',(17.5354201549704,2.71645997318391,-47.3134407766488));
#57491=CARTESIAN_POINT('Ctrl Pts',(17.5350661679349,4.07346458001521,-47.222622635811));
#57492=CARTESIAN_POINT('Ctrl Pts',(18.0841700243305,0.0168314204591895,
-47.6825109969299));
#57493=CARTESIAN_POINT('Ctrl Pts',(18.0828633665264,1.37313536000937,-47.5821735769392));
#57494=CARTESIAN_POINT('Ctrl Pts',(18.0815566850005,2.72943929801651,-47.4818361427477));
#57495=CARTESIAN_POINT('Ctrl Pts',(18.0802500271968,4.08574323756672,-47.3814987227573));
#57496=CARTESIAN_POINT('',(0.,2.01462393409065,-45.4512));
#57497=CARTESIAN_POINT('Ctrl Pts',(70.7282577522084,8.51486331986405,-11.8925191845565));
#57498=CARTESIAN_POINT('Ctrl Pts',(70.3600859174044,9.78627568392211,-11.5801730615178));
#57499=CARTESIAN_POINT('Ctrl Pts',(69.9919140826003,11.0576880479802,-11.267826938479));
#57500=CARTESIAN_POINT('Ctrl Pts',(69.6237422477963,12.3291004120382,-10.9554808154403));
#57501=CARTESIAN_POINT('Ctrl Pts',(71.1586139886749,8.57802101438411,-11.6423301611079));
#57502=CARTESIAN_POINT('Ctrl Pts',(70.8002393926315,9.84354972351229,-11.2952769038158));
#57503=CARTESIAN_POINT('Ctrl Pts',(70.4411327279621,11.1095147323032,-10.9484903485044));
#57504=CARTESIAN_POINT('Ctrl Pts',(70.0827581319187,12.3750434414314,-10.6014370912123));
#57505=CARTESIAN_POINT('Ctrl Pts',(71.9827018728919,8.65468599963629,-11.0972577103214));
#57506=CARTESIAN_POINT('Ctrl Pts',(71.6283269336556,9.91255505994493,-10.7211921629858));
#57507=CARTESIAN_POINT('Ctrl Pts',(71.274046257563,11.1704252165446,-10.345117454098));
#57508=CARTESIAN_POINT('Ctrl Pts',(70.9196713183267,12.4282942768532,-9.96905190676241));
#57509=CARTESIAN_POINT('Ctrl Pts',(73.1303575054126,8.72650011278445,-10.21988802762));
#57510=CARTESIAN_POINT('Ctrl Pts',(72.7531257555003,9.98379326247583,-9.86275653492437));
#57511=CARTESIAN_POINT('Ctrl Pts',(72.3755917318045,11.2412341838258,-9.50577501726162));
#57512=CARTESIAN_POINT('Ctrl Pts',(71.9983599818921,12.4985273335172,-9.148643524566));
#57513=CARTESIAN_POINT('Ctrl Pts',(74.1065736572356,8.81331425878696,-9.37805983947955));
#57514=CARTESIAN_POINT('Ctrl Pts',(73.6947438271767,10.0724325673801,-9.06858889521421));
#57515=CARTESIAN_POINT('Ctrl Pts',(73.2830206497004,11.3316920464878,-8.7588620545661));
#57516=CARTESIAN_POINT('Ctrl Pts',(72.8711908196415,12.5908103550809,-8.44939111030075));
#57517=CARTESIAN_POINT('Ctrl Pts',(75.1777989853639,8.95359154800345,-8.37681652932542));
#57518=CARTESIAN_POINT('Ctrl Pts',(74.7248971875948,10.2125650956128,-8.12906705485955));
#57519=CARTESIAN_POINT('Ctrl Pts',(74.2723094444152,11.4717337582538,-7.88062467972502));
#57520=CARTESIAN_POINT('Ctrl Pts',(73.8194076466462,12.7307073058631,-7.63287520525915));
#57521=CARTESIAN_POINT('Ctrl Pts',(76.3760621018627,9.18465108771821,-7.13733271471052));
#57522=CARTESIAN_POINT('Ctrl Pts',(75.8808429490457,10.4390507692653,-6.95644970672696));
#57523=CARTESIAN_POINT('Ctrl Pts',(75.3855963914733,11.6934931005301,-6.77561572455319));
#57524=CARTESIAN_POINT('Ctrl Pts',(74.8903772386563,12.9478927820772,-6.59473271656963));
#57525=CARTESIAN_POINT('Ctrl Pts',(77.1569389883271,9.37730603443782,-6.18970317121555));
#57526=CARTESIAN_POINT('Ctrl Pts',(76.6501763150819,10.6273118023276,-6.01732352238457));
#57527=CARTESIAN_POINT('Ctrl Pts',(76.1434037774154,11.8780966175269,-5.8447821263057));
#57528=CARTESIAN_POINT('Ctrl Pts',(75.6366411041703,13.1281023854167,-5.67240247747472));
#57529=CARTESIAN_POINT('Ctrl Pts',(77.5413122691233,9.45942207531684,-5.67964638243731));
#57530=CARTESIAN_POINT('Ctrl Pts',(77.0326085523511,10.7074362929352,-5.49721546081316));
#57531=CARTESIAN_POINT('Ctrl Pts',(76.5239048355788,11.9554505105535,-5.314784539189));
#57532=CARTESIAN_POINT('Ctrl Pts',(76.0152011188066,13.2034647281718,-5.13235361756485));
#57533=CARTESIAN_POINT('',(76.778256693965,11.3314434017443,-5.40600000000103));
#57534=CARTESIAN_POINT('',(70.1760000000024,10.4219818659511,-11.4239999999984));
#57535=CARTESIAN_POINT('',(70.1760000000024,10.4219818659511,-11.4239999999984));
#57536=CARTESIAN_POINT('',(70.1760000000024,10.4219818659511,-11.4239999999984));
#57537=CARTESIAN_POINT('Ctrl Pts',(57.8135230791049,6.6905663225968,-18.0349157107808));
#57538=CARTESIAN_POINT('Ctrl Pts',(57.5247816344839,7.95941791373735,-17.6396385702601));
#57539=CARTESIAN_POINT('Ctrl Pts',(57.2360401898628,9.22826950487791,-17.2443614297393));
#57540=CARTESIAN_POINT('Ctrl Pts',(56.9472987452418,10.4971210960185,-16.8490842892186));
#57541=CARTESIAN_POINT('Ctrl Pts',(58.3834371192583,6.78492400902022,-17.921496800064));
#57542=CARTESIAN_POINT('Ctrl Pts',(58.0977762359506,8.04459708605881,-17.4923487139126));
#57543=CARTESIAN_POINT('Ctrl Pts',(57.8136373060536,9.30309323278309,-17.0647829526039));
#57544=CARTESIAN_POINT('Ctrl Pts',(57.5279764227459,10.5627663098217,-16.6356348664524));
#57545=CARTESIAN_POINT('Ctrl Pts',(60.069006328368,7.0315326697423,-17.5237672087188));
#57546=CARTESIAN_POINT('Ctrl Pts',(59.7958287466441,8.26340634490229,-17.0172277477915));
#57547=CARTESIAN_POINT('Ctrl Pts',(59.5221571822746,9.49577953239501,-16.5100213706393));
#57548=CARTESIAN_POINT('Ctrl Pts',(59.2489796005507,10.727653207555,-16.0034819097119));
#57549=CARTESIAN_POINT('Ctrl Pts',(62.2034160825709,7.1647901104433,-16.747451663188));
#57550=CARTESIAN_POINT('Ctrl Pts',(61.9177268933279,8.39487645389337,-16.2388750355847));
#57551=CARTESIAN_POINT('Ctrl Pts',(61.6326018983047,9.62476272199721,-15.7302755084792));
#57552=CARTESIAN_POINT('Ctrl Pts',(61.3469127090617,10.8548490654473,-15.2216988808759));
#57553=CARTESIAN_POINT('Ctrl Pts',(64.7264374328703,7.37946418630416,-15.4764719489058));
#57554=CARTESIAN_POINT('Ctrl Pts',(64.3595954246239,8.63587598557369,-15.0963863265111));
#57555=CARTESIAN_POINT('Ctrl Pts',(63.9932223004386,9.89184700111287,-14.7162842302533));
#57556=CARTESIAN_POINT('Ctrl Pts',(63.6263802921922,11.1482588003824,-14.3361986078586));
#57557=CARTESIAN_POINT('Ctrl Pts',(66.8940351574184,7.74903378142021,-14.2111203469359));
#57558=CARTESIAN_POINT('Ctrl Pts',(66.4695339814581,9.01812242902804,-13.9619266203826));
#57559=CARTESIAN_POINT('Ctrl Pts',(66.0445138974904,10.2868967403885,-13.7141750122686));
#57560=CARTESIAN_POINT('Ctrl Pts',(65.6200127215301,11.5559853879963,-13.4649812857152));
#57561=CARTESIAN_POINT('Ctrl Pts',(68.5152601688859,8.12096232366399,-13.2306538995856));
#57562=CARTESIAN_POINT('Ctrl Pts',(68.0991834125406,9.39567311929895,-13.0053211729385));
#57563=CARTESIAN_POINT('Ctrl Pts',(67.6826412354218,10.6707550048034,-12.7801625272814));
#57564=CARTESIAN_POINT('Ctrl Pts',(67.2665644790765,11.9454658004384,-12.5548298006343));
#57565=CARTESIAN_POINT('Ctrl Pts',(69.7958454230149,8.37193054851245,-12.4618050355517));
#57566=CARTESIAN_POINT('Ctrl Pts',(69.4062810684438,9.6486674313224,-12.1988738548688));
#57567=CARTESIAN_POINT('Ctrl Pts',(69.0168135363837,10.9250928657635,-11.93627796497));
#57568=CARTESIAN_POINT('Ctrl Pts',(68.6272491818126,12.2018297485735,-11.6733467842871));
#57569=CARTESIAN_POINT('Ctrl Pts',(70.4319511017933,8.47390908124125,-12.0750795994181));
#57570=CARTESIAN_POINT('Ctrl Pts',(70.0578486510975,9.74756100248359,-11.7792662482282));
#57571=CARTESIAN_POINT('Ctrl Pts',(69.6832582272912,11.0214634770417,-11.4837699563737));
#57572=CARTESIAN_POINT('Ctrl Pts',(69.3091557765954,12.295115398284,-11.1879566051838));
#57573=CARTESIAN_POINT('Ctrl Pts',(70.7282577522084,8.51486331986406,-11.8925191845565));
#57574=CARTESIAN_POINT('Ctrl Pts',(70.3600859174044,9.78627568392211,-11.5801730615178));
#57575=CARTESIAN_POINT('Ctrl Pts',(69.9919140826003,11.0576880479802,-11.267826938479));
#57576=CARTESIAN_POINT('Ctrl Pts',(69.6237422477963,12.3291004120382,-10.9554808154403));
#57577=CARTESIAN_POINT('',(57.3804109121731,8.59384370930882,-17.4419999999993));
#57578=CARTESIAN_POINT('',(57.3804109121734,8.59384370930763,-17.4419999999997));
#57579=CARTESIAN_POINT('',(57.3804109121734,8.59384370930763,-17.4419999999997));
#57580=CARTESIAN_POINT('Ctrl Pts',(44.864374876377,5.20597739807143,-23.9801519722225));
#57581=CARTESIAN_POINT('Ctrl Pts',(44.4545859760344,6.45554733375931,-23.6333839907407));
#57582=CARTESIAN_POINT('Ctrl Pts',(44.0447970756917,7.7051172694472,-23.286616009259));
#57583=CARTESIAN_POINT('Ctrl Pts',(43.635008175349,8.95468720513508,-22.9398480277772));
#57584=CARTESIAN_POINT('Ctrl Pts',(45.1224142763232,5.22734724195968,-23.7522227177446));
#57585=CARTESIAN_POINT('Ctrl Pts',(44.740324729997,6.47318492815149,-23.3556198386977));
#57586=CARTESIAN_POINT('Ctrl Pts',(44.3637122482329,7.7164483348677,-22.9542254972333));
#57587=CARTESIAN_POINT('Ctrl Pts',(43.9816227019066,8.96228602105951,-22.5576226181864));
#57588=CARTESIAN_POINT('Ctrl Pts',(45.9649684987856,5.22804284539893,-23.0069752550256));
#57589=CARTESIAN_POINT('Ctrl Pts',(45.6662512806454,6.45193039127154,-22.4921612743428));
#57590=CARTESIAN_POINT('Ctrl Pts',(45.36522683304,7.67699365561725,-21.9792150829581));
#57591=CARTESIAN_POINT('Ctrl Pts',(45.0665096148998,8.90088120148987,-21.4644011022753));
#57592=CARTESIAN_POINT('Ctrl Pts',(47.4758616466553,5.06915938849053,-21.7520512140078));
#57593=CARTESIAN_POINT('Ctrl Pts',(47.1533462028712,6.3023705311178,-21.2750662029529));
#57594=CARTESIAN_POINT('Ctrl Pts',(46.8283779466042,7.53667509779519,-20.8011913848345));
#57595=CARTESIAN_POINT('Ctrl Pts',(46.5058625028201,8.76988624042247,-20.3242063737796));
#57596=CARTESIAN_POINT('Ctrl Pts',(49.1569256056527,5.20366478491719,-20.7106555371184));
#57597=CARTESIAN_POINT('Ctrl Pts',(48.8012788734978,6.46168428440042,-20.3329464870476));
#57598=CARTESIAN_POINT('Ctrl Pts',(48.4486371023923,7.71873636075261,-19.9528495627537));
#57599=CARTESIAN_POINT('Ctrl Pts',(48.0929903702374,8.97675586023584,-19.5751405126828));
#57600=CARTESIAN_POINT('Ctrl Pts',(50.0106311017377,5.31735504507218,-20.255161743136));
#57601=CARTESIAN_POINT('Ctrl Pts',(49.6529273423844,6.58525639569541,-19.918243070567));
#57602=CARTESIAN_POINT('Ctrl Pts',(49.2940750004474,7.8538792563298,-19.5830916546927));
#57603=CARTESIAN_POINT('Ctrl Pts',(48.9363712410941,9.12178060695302,-19.2461729821237));
#57604=CARTESIAN_POINT('Ctrl Pts',(50.9536821648416,5.47540829520537,-19.8330327894735));
#57605=CARTESIAN_POINT('Ctrl Pts',(50.6007520305354,6.75386029493047,-19.5306366791759));
#57606=CARTESIAN_POINT('Ctrl Pts',(50.2500375292763,8.03187941866197,-19.2269995241046));
#57607=CARTESIAN_POINT('Ctrl Pts',(49.8971073949701,9.31033141838707,-18.924603413807));
#57608=CARTESIAN_POINT('Ctrl Pts',(52.3106429243915,5.72884656211269,-19.3291250816917));
#57609=CARTESIAN_POINT('Ctrl Pts',(51.980515160004,7.01824730214814,-19.0500355888166));
#57610=CARTESIAN_POINT('Ctrl Pts',(51.650702670309,8.30831373472467,-18.7724371720687));
#57611=CARTESIAN_POINT('Ctrl Pts',(51.3205749059214,9.59771447476012,-18.4933476791936));
#57612=CARTESIAN_POINT('Ctrl Pts',(54.584459674483,6.15313027810468,-18.7389663173459));
#57613=CARTESIAN_POINT('Ctrl Pts',(54.2914742766135,7.44767092452855,-18.4397413559177));
#57614=CARTESIAN_POINT('Ctrl Pts',(53.9970607847715,8.74061567008386,-18.1369221537377));
#57615=CARTESIAN_POINT('Ctrl Pts',(53.704075386902,10.0351563165077,-17.8376971923096));
#57616=CARTESIAN_POINT('Ctrl Pts',(56.7527899477957,6.52682846803759,-18.2841549642181));
#57617=CARTESIAN_POINT('Ctrl Pts',(56.4580200210017,7.80528056919744,-17.9241761601542));
#57618=CARTESIAN_POINT('Ctrl Pts',(56.1665627987475,9.08533845315947,-17.5667019119172));
#57619=CARTESIAN_POINT('Ctrl Pts',(55.8717928719535,10.3637905543193,-17.2067231078532));
#57620=CARTESIAN_POINT('Ctrl Pts',(57.8135230791049,6.69056632259679,-18.0349157107808));
#57621=CARTESIAN_POINT('Ctrl Pts',(57.5247816344839,7.95941791373734,-17.6396385702601));
#57622=CARTESIAN_POINT('Ctrl Pts',(57.2360401898628,9.2282695048779,-17.2443614297393));
#57623=CARTESIAN_POINT('Ctrl Pts',(56.9472987452418,10.4971210960185,-16.8490842892186));
#57624=CARTESIAN_POINT('',(44.249691525863,7.08033230160326,-23.4599999999998));
#57625=CARTESIAN_POINT('',(44.249691525863,7.08033230160326,-23.4599999999998));
#57626=CARTESIAN_POINT('',(44.249691525863,7.08033230160326,-23.4599999999998));
#57627=CARTESIAN_POINT('Ctrl Pts',(41.4215425945231,4.68791040664211,-29.7512671854166));
#57628=CARTESIAN_POINT('Ctrl Pts',(40.8936377463565,5.92799480013269,-29.5690918542356));
#57629=CARTESIAN_POINT('Ctrl Pts',(40.3657328989121,7.1680791888473,-29.3869165043121));
#57630=CARTESIAN_POINT('Ctrl Pts',(39.8378280507455,8.40816358233807,-29.2047411731319));
#57631=CARTESIAN_POINT('Ctrl Pts',(41.4802683438712,4.68413044508663,-29.5553621466157));
#57632=CARTESIAN_POINT('Ctrl Pts',(40.9494709539923,5.92282615948956,-29.3722187306946));
#57633=CARTESIAN_POINT('Ctrl Pts',(40.4186595175311,7.16161474998382,-29.1894397906751));
#57634=CARTESIAN_POINT('Ctrl Pts',(39.8878621282648,8.40031046033545,-29.0062963588554));
#57635=CARTESIAN_POINT('Ctrl Pts',(41.6778807320694,4.68063487456826,-28.9529176330051));
#57636=CARTESIAN_POINT('Ctrl Pts',(41.1360096258359,5.91450409764293,-28.768958382227));
#57637=CARTESIAN_POINT('Ctrl Pts',(40.5940809445236,7.14834387762203,-28.5849862352923));
#57638=CARTESIAN_POINT('Ctrl Pts',(40.0522098408016,8.38221310198101,-28.4010269850767));
#57639=CARTESIAN_POINT('Ctrl Pts',(42.0667678924717,4.70419304693246,-27.964824273678));
#57640=CARTESIAN_POINT('Ctrl Pts',(41.5010972238371,5.92783482634179,-27.7841784792369));
#57641=CARTESIAN_POINT('Ctrl Pts',(40.9357028569913,7.1514823641546,-27.6030152424684));
#57642=CARTESIAN_POINT('Ctrl Pts',(40.3700321763043,8.37512414331273,-27.4223694705982));
#57643=CARTESIAN_POINT('Ctrl Pts',(42.6729216974824,4.823611553925,-26.7992794766923));
#57644=CARTESIAN_POINT('Ctrl Pts',(42.0918120029199,6.04066662955073,-26.6236449949611));
#57645=CARTESIAN_POINT('Ctrl Pts',(41.5102646021906,7.25771063739046,-26.4488728648612));
#57646=CARTESIAN_POINT('Ctrl Pts',(40.929154926721,8.47476571349897,-26.2732383455139));
#57647=CARTESIAN_POINT('Ctrl Pts',(43.1602150679141,4.93691815783542,-26.0485095188922));
#57648=CARTESIAN_POINT('Ctrl Pts',(42.5955457707243,6.15965834108405,-25.8592274909061));
#57649=CARTESIAN_POINT('Ctrl Pts',(42.0312832814734,7.38237091318394,-25.6691749339123));
#57650=CARTESIAN_POINT('Ctrl Pts',(41.4666139665385,8.60511109763698,-25.4798929395369));
#57651=CARTESIAN_POINT('Ctrl Pts',(43.3508405942975,4.97964296442833,-25.7696090237298));
#57652=CARTESIAN_POINT('Ctrl Pts',(42.7960855748333,6.20551740122266,-25.5716146485843));
#57653=CARTESIAN_POINT('Ctrl Pts',(42.24110371321,7.43134209790289,-25.373966918556));
#57654=CARTESIAN_POINT('Ctrl Pts',(41.6863487036408,8.6572165368669,-25.1759725282897));
#57655=CARTESIAN_POINT('Ctrl Pts',(43.6185109451061,5.03817773651984,-25.3933166689187));
#57656=CARTESIAN_POINT('Ctrl Pts',(43.0800759415707,6.26907713023514,-25.1812823216724));
#57657=CARTESIAN_POINT('Ctrl Pts',(42.5417926904819,7.49987935633806,-24.9689147600707));
#57658=CARTESIAN_POINT('Ctrl Pts',(42.003357680327,8.73077875429183,-24.7568804273593));
#57659=CARTESIAN_POINT('Ctrl Pts',(44.1126628332362,5.13439778509021,-24.7624098976365));
#57660=CARTESIAN_POINT('Ctrl Pts',(43.61806572663,6.37718213105814,-24.5106662229177));
#57661=CARTESIAN_POINT('Ctrl Pts',(43.1231679405891,7.62001857940251,-24.2593794372098));
#57662=CARTESIAN_POINT('Ctrl Pts',(42.6285708470986,8.86280292309772,-24.0076357425614));
#57663=CARTESIAN_POINT('Ctrl Pts',(44.5974345578285,5.19049120521572,-24.2397960938373));
#57664=CARTESIAN_POINT('Ctrl Pts',(44.1586022338354,6.44060862595914,-23.9289029933399));
#57665=CARTESIAN_POINT('Ctrl Pts',(43.7201939318932,7.69040988955953,-23.6172776091317));
#57666=CARTESIAN_POINT('Ctrl Pts',(43.2813615894041,8.94052732409383,-23.3063845405767));
#57667=CARTESIAN_POINT('Ctrl Pts',(44.8644027152632,5.20597901315863,-23.9801248941554));
#57668=CARTESIAN_POINT('Ctrl Pts',(44.4546079053322,6.45557614794012,-23.6333456074787));
#57669=CARTESIAN_POINT('Ctrl Pts',(44.0448130511831,7.70517331569156,-23.2865663971665));
#57670=CARTESIAN_POINT('Ctrl Pts',(43.635018241254,8.9547704504716,-22.9397871104864));
#57671=CARTESIAN_POINT('',(40.6297053891129,6.5479961266057,-29.4780000000001));
#57672=CARTESIAN_POINT('Ctrl Pts',(40.1355624239865,4.76730440823259,-35.6660906786094));
#57673=CARTESIAN_POINT('Ctrl Pts',(39.7267542314648,6.05945057763009,-35.5526974481249));
#57674=CARTESIAN_POINT('Ctrl Pts',(39.3179460376291,7.35159674641259,-35.439304217727));
#57675=CARTESIAN_POINT('Ctrl Pts',(38.9091378451075,8.6437429158101,-35.3259109872425));
#57676=CARTESIAN_POINT('Ctrl Pts',(40.3022852108888,4.74136008557223,-34.7693748964185));
#57677=CARTESIAN_POINT('Ctrl Pts',(39.8830814907514,6.03145578103333,-34.6704501714334));
#57678=CARTESIAN_POINT('Ctrl Pts',(39.464473218501,7.3218301400057,-34.5714862261209));
#57679=CARTESIAN_POINT('Ctrl Pts',(39.0452694906739,8.61192583186812,-34.4725615016423));
#57680=CARTESIAN_POINT('Ctrl Pts',(40.5112835949553,4.72982185272993,-33.6344144304767));
#57681=CARTESIAN_POINT('Ctrl Pts',(40.0672938950195,6.01213072428518,-33.5400173560715));
#57682=CARTESIAN_POINT('Ctrl Pts',(39.6231973650581,7.29439145612538,-33.4457381236464));
#57683=CARTESIAN_POINT('Ctrl Pts',(39.1792076665018,8.57670032830231,-33.3513410477193));
#57684=CARTESIAN_POINT('Ctrl Pts',(40.7814488661554,4.71765074492916,-32.2936083574543));
#57685=CARTESIAN_POINT('Ctrl Pts',(40.30513540374,5.98679527850069,-32.1831482629611));
#57686=CARTESIAN_POINT('Ctrl Pts',(39.82883397811,7.25594573394774,-32.0726643871796));
#57687=CARTESIAN_POINT('Ctrl Pts',(39.3525205155391,8.52509026744278,-31.9622042929936));
#57688=CARTESIAN_POINT('Ctrl Pts',(40.942076978619,4.71061953663584,-31.5521512150188));
#57689=CARTESIAN_POINT('Ctrl Pts',(40.4480662906984,5.97166384408667,-31.427374520508));
#57690=CARTESIAN_POINT('Ctrl Pts',(39.9542499180149,7.23280392932176,-31.3028020868362));
#57691=CARTESIAN_POINT('Ctrl Pts',(39.460239227585,8.49384823553572,-31.1780253896876));
#57692=CARTESIAN_POINT('Ctrl Pts',(41.1407904972541,4.7010692865962,-30.7187856331133));
#57693=CARTESIAN_POINT('Ctrl Pts',(40.6287473002004,5.95259800346332,-30.5721760653661));
#57694=CARTESIAN_POINT('Ctrl Pts',(40.11632906848,7.20394181697493,-30.4251866697367));
#57695=CARTESIAN_POINT('Ctrl Pts',(39.6042858762695,8.45547053622989,-30.2785771068945));
#57696=CARTESIAN_POINT('Ctrl Pts',(41.3201731760795,4.69236269068941,-30.0753208265298));
#57697=CARTESIAN_POINT('Ctrl Pts',(40.7965442941259,5.936128776676,-29.9058793753165));
#57698=CARTESIAN_POINT('Ctrl Pts',(40.2734349337518,7.18014776732202,-29.7369323570816));
#57699=CARTESIAN_POINT('Ctrl Pts',(39.7498060450891,8.42391385004259,-29.5674908994831));
#57700=CARTESIAN_POINT('Ctrl Pts',(41.4215465127793,4.68791017280978,-29.7512542394393));
#57701=CARTESIAN_POINT('Ctrl Pts',(40.8936495828703,5.92797542331161,-29.5690815425449));
#57702=CARTESIAN_POINT('Ctrl Pts',(40.3657526483566,7.16804067157194,-29.3869088412683));
#57703=CARTESIAN_POINT('Ctrl Pts',(39.8378557184476,8.4081059220738,-29.204736144374));
#57704=CARTESIAN_POINT('',(39.5223544282475,6.70551108323301,-35.4960000000008));
#57705=CARTESIAN_POINT('Ctrl Pts',(38.8604541099242,4.82976572790836,-41.6539325852788));
#57706=CARTESIAN_POINT('Ctrl Pts',(38.4040326949894,6.10748900320916,-41.560644195093));
#57707=CARTESIAN_POINT('Ctrl Pts',(37.9476112800545,7.38521227850996,-41.4673558049072));
#57708=CARTESIAN_POINT('Ctrl Pts',(37.4911898651196,8.66293555381076,-41.3740674147214));
#57709=CARTESIAN_POINT('Ctrl Pts',(39.0048197292983,4.83127154325761,-40.9682358462176));
#57710=CARTESIAN_POINT('Ctrl Pts',(38.5631614180215,6.11417338749171,-40.8732587077797));
#57711=CARTESIAN_POINT('Ctrl Pts',(38.1218299586132,7.39711052016881,-40.7783273701692));
#57712=CARTESIAN_POINT('Ctrl Pts',(37.6801716473364,8.68001236440291,-40.6833502317314));
#57713=CARTESIAN_POINT('Ctrl Pts',(39.2693233059464,4.83474737532154,-39.8104175938772));
#57714=CARTESIAN_POINT('Ctrl Pts',(38.8540548662111,6.12623786385084,-39.7127351491205));
#57715=CARTESIAN_POINT('Ctrl Pts',(38.4385849974131,7.41770099535643,-39.6150176340949));
#57716=CARTESIAN_POINT('Ctrl Pts',(38.0233165576779,8.70919148388572,-39.5173351893382));
#57717=CARTESIAN_POINT('Ctrl Pts',(39.6452981730948,4.8199494242592,-38.1129891991618));
#57718=CARTESIAN_POINT('Ctrl Pts',(39.2474592055531,6.1164069836728,-38.0104489972814));
#57719=CARTESIAN_POINT('Ctrl Pts',(38.8497085452635,7.41288231613064,-37.9079311640875));
#57720=CARTESIAN_POINT('Ctrl Pts',(38.4518695777218,8.70933987554425,-37.8053909622071));
#57721=CARTESIAN_POINT('Ctrl Pts',(39.8853277117453,4.79858865457864,-36.9461294764195));
#57722=CARTESIAN_POINT('Ctrl Pts',(39.4866283556263,6.09442229132186,-36.839046741644));
#57723=CARTESIAN_POINT('Ctrl Pts',(39.0879084576719,7.39024881387909,-36.7319585207745));
#57724=CARTESIAN_POINT('Ctrl Pts',(38.6892091015529,8.68608245062232,-36.6248757859991));
#57725=CARTESIAN_POINT('Ctrl Pts',(40.0280907705529,4.78204396051868,-36.2245904908727));
#57726=CARTESIAN_POINT('Ctrl Pts',(39.6249516837898,6.0762191111159,-36.1141481442971));
#57727=CARTESIAN_POINT('Ctrl Pts',(39.2218674158251,7.37041538269592,-36.0037336147251));
#57728=CARTESIAN_POINT('Ctrl Pts',(38.818728329062,8.66459053329314,-35.8932912681495));
#57729=CARTESIAN_POINT('Ctrl Pts',(40.1031985714104,4.7719144148413,-35.8353019842399));
#57730=CARTESIAN_POINT('Ctrl Pts',(39.6962798859278,6.06473085465749,-35.722829449568));
#57731=CARTESIAN_POINT('Ctrl Pts',(39.2893811996143,7.35755308021419,-35.6103820624053));
#57732=CARTESIAN_POINT('Ctrl Pts',(38.8824625141317,8.65036952003038,-35.4979095277334));
#57733=CARTESIAN_POINT('Ctrl Pts',(40.1355627919427,4.76730435097364,-35.6660886995628));
#57734=CARTESIAN_POINT('Ctrl Pts',(39.7267572161459,6.05944217247988,-35.5526962331881));
#57735=CARTESIAN_POINT('Ctrl Pts',(39.3179516403491,7.35157999398613,-35.4393037668135));
#57736=CARTESIAN_POINT('Ctrl Pts',(38.9091460645523,8.64371781549238,-35.3259113004388));
#57737=CARTESIAN_POINT('',(38.1758219875219,6.74635064085956,-41.5140000000001));
#57738=CARTESIAN_POINT('Ctrl Pts',(38.0224643391856,4.86842248450045,-47.6590906035866));
#57739=CARTESIAN_POINT('Ctrl Pts',(37.5141154779131,6.12699419839355,-47.5743635345289));
#57740=CARTESIAN_POINT('Ctrl Pts',(37.0057666166406,7.38556591228665,-47.4896364654712));
#57741=CARTESIAN_POINT('Ctrl Pts',(36.497417755368,8.64413762617975,-47.4049093964135));
#57742=CARTESIAN_POINT('Ctrl Pts',(38.0629003858012,4.86150818139181,-47.3137728097505));
#57743=CARTESIAN_POINT('Ctrl Pts',(37.5511999079971,6.1190243894845,-47.2334402336884));
#57744=CARTESIAN_POINT('Ctrl Pts',(37.0394051258501,7.3765107446069,-47.1533372415835));
#57745=CARTESIAN_POINT('Ctrl Pts',(36.527704648046,8.63402695269959,-47.0730046655214));
#57746=CARTESIAN_POINT('Ctrl Pts',(38.1507053914965,4.8450084544398,-46.4729294774833));
#57747=CARTESIAN_POINT('Ctrl Pts',(37.6327442277917,6.10042701332241,-46.400485455692));
#57748=CARTESIAN_POINT('Ctrl Pts',(37.1149509225975,7.35590056277829,-46.3277870171961));
#57749=CARTESIAN_POINT('Ctrl Pts',(36.5969897588927,8.6113191216609,-46.2553429954049));
#57750=CARTESIAN_POINT('Ctrl Pts',(38.2620837951133,4.82664388150297,-45.3133943758124));
#57751=CARTESIAN_POINT('Ctrl Pts',(37.7433647107974,6.08193783777536,-45.2441132294512));
#57752=CARTESIAN_POINT('Ctrl Pts',(37.2245219104796,7.33719426285198,-45.1749682106718));
#57753=CARTESIAN_POINT('Ctrl Pts',(36.7058028261638,8.59248821912437,-45.1056870643106));
#57754=CARTESIAN_POINT('Ctrl Pts',(38.4228858295138,4.82107508008706,-44.0628313203019));
#57755=CARTESIAN_POINT('Ctrl Pts',(37.9176015720814,6.08163116257953,-43.9896189803569));
#57756=CARTESIAN_POINT('Ctrl Pts',(37.4123697296278,7.34219997720122,-43.9163618117411));
#57757=CARTESIAN_POINT('Ctrl Pts',(36.9070854721954,8.60275605969368,-43.8431494717961));
#57758=CARTESIAN_POINT('Ctrl Pts',(38.5993784816469,4.82325654371877,-42.9411023467542));
#57759=CARTESIAN_POINT('Ctrl Pts',(38.1135891457311,6.09108424087921,-42.8607129324259));
#57760=CARTESIAN_POINT('Ctrl Pts',(37.6277594573051,7.35891332881017,-42.7803490135197));
#57761=CARTESIAN_POINT('Ctrl Pts',(37.1419701213893,8.6267410259706,-42.6999595991915));
#57762=CARTESIAN_POINT('Ctrl Pts',(38.7504700253912,4.82820987401249,-42.170729376939));
#57763=CARTESIAN_POINT('Ctrl Pts',(38.2826040468472,6.10225649008106,-42.0828980653399));
#57764=CARTESIAN_POINT('Ctrl Pts',(37.8147453818706,7.37626900862381,-41.9951012812711));
#57765=CARTESIAN_POINT('Ctrl Pts',(37.3468794033266,8.65031562469239,-41.9072699696721));
#57766=CARTESIAN_POINT('Ctrl Pts',(38.8604541099242,4.82976572790836,-41.6539325852788));
#57767=CARTESIAN_POINT('Ctrl Pts',(38.4040326949894,6.10748900320916,-41.560644195093));
#57768=CARTESIAN_POINT('Ctrl Pts',(37.9476112800545,7.38521227850996,-41.4673558049072));
#57769=CARTESIAN_POINT('Ctrl Pts',(37.4911898651196,8.66293555381076,-41.3740674147214));
#57770=CARTESIAN_POINT('',(37.2599410472768,6.7562800553401,-47.532));
#57771=CARTESIAN_POINT('Ctrl Pts',(36.1829187178027,4.79789635062137,-53.6562454252777));
#57772=CARTESIAN_POINT('Ctrl Pts',(35.7573843424341,6.08767170594883,-53.5854166319681));
#57773=CARTESIAN_POINT('Ctrl Pts',(35.331849966191,7.37744705912874,-53.514587843528));
#57774=CARTESIAN_POINT('Ctrl Pts',(34.9063155908223,8.66722241445618,-53.4437590502184));
#57775=CARTESIAN_POINT('Ctrl Pts',(36.4945975641142,4.8692415372667,-53.0828797714532));
#57776=CARTESIAN_POINT('Ctrl Pts',(36.0607845903544,6.15396331395307,-52.9743935222565));
#57777=CARTESIAN_POINT('Ctrl Pts',(35.6272852524983,7.4394553746638,-52.8641606487343));
#57778=CARTESIAN_POINT('Ctrl Pts',(35.1934722815684,8.72417715829996,-52.7556743837789));
#57779=CARTESIAN_POINT('Ctrl Pts',(37.0196238186211,4.94621406635564,-52.0172199352926));
#57780=CARTESIAN_POINT('Ctrl Pts',(36.5725094960081,6.22274211276401,-51.8743508628265));
#57781=CARTESIAN_POINT('Ctrl Pts',(36.1253011361753,7.49898590806397,-51.7321837308753));
#57782=CARTESIAN_POINT('Ctrl Pts',(35.6781868127138,8.77551395190772,-51.5893146647424));
#57783=CARTESIAN_POINT('Ctrl Pts',(37.4961264547335,4.95593012911406,-50.632199053437));
#57784=CARTESIAN_POINT('Ctrl Pts',(37.0309089823822,6.22517924195192,-50.4826709817263));
#57785=CARTESIAN_POINT('Ctrl Pts',(36.5656417928408,7.49447486452825,-50.3328090769852));
#57786=CARTESIAN_POINT('Ctrl Pts',(36.1004243200409,8.76372397778573,-50.1832810022625));
#57787=CARTESIAN_POINT('Ctrl Pts',(37.8514088449462,4.91190498255859,-49.0406523578434));
#57788=CARTESIAN_POINT('Ctrl Pts',(37.3611948698808,6.17388941863381,-48.9098613797906));
#57789=CARTESIAN_POINT('Ctrl Pts',(36.8710842666241,7.43589006578039,-48.7793508906566));
#57790=CARTESIAN_POINT('Ctrl Pts',(36.3808702924914,8.69787450200186,-48.6485599151345));
#57791=CARTESIAN_POINT('Ctrl Pts',(37.9653755874324,4.87922727833883,-48.1624087409971));
#57792=CARTESIAN_POINT('Ctrl Pts',(37.4620517032201,6.13855052559459,-48.0582635515641));
#57793=CARTESIAN_POINT('Ctrl Pts',(36.9587801664333,7.39783829087798,-47.9542796924559));
#57794=CARTESIAN_POINT('Ctrl Pts',(36.4554562826933,8.65716153781361,-47.8501345044785));
#57795=CARTESIAN_POINT('Ctrl Pts',(38.0224713673792,4.86840542327654,-47.6590904423752));
#57796=CARTESIAN_POINT('Ctrl Pts',(37.5141201997668,6.12698281293256,-47.574363041552));
#57797=CARTESIAN_POINT('Ctrl Pts',(37.0057690320183,7.38556020268079,-47.4896356403095));
#57798=CARTESIAN_POINT('Ctrl Pts',(36.4974178644059,8.6441375923368,-47.4049082394863));
#57799=CARTESIAN_POINT('',(35.5446151095801,6.73256828905091,-53.5499999999998));
#57800=CARTESIAN_POINT('',(35.5446151095801,6.732568289051,-53.5499999999998));
#57801=CARTESIAN_POINT('',(35.5446151095801,6.732568289051,-53.5499999999998));
#57802=CARTESIAN_POINT('Ctrl Pts',(33.2870419060244,4.35253527707261,-59.9326413364725));
#57803=CARTESIAN_POINT('Ctrl Pts',(33.1297679354284,5.68135810058122,-59.6895471121569));
#57804=CARTESIAN_POINT('Ctrl Pts',(32.9724939648324,7.01018092408982,-59.4464528878414));
#57805=CARTESIAN_POINT('Ctrl Pts',(32.8152199942364,8.33900374759843,-59.2033586635258));
#57806=CARTESIAN_POINT('Ctrl Pts',(33.4229509461086,4.29496143663751,-59.5299975144865));
#57807=CARTESIAN_POINT('Ctrl Pts',(33.2540721505405,5.629703551151,-59.3266294513922));
#57808=CARTESIAN_POINT('Ctrl Pts',(33.0848228192888,6.96433962786048,-59.1233364488466));
#57809=CARTESIAN_POINT('Ctrl Pts',(32.9159440237207,8.29908174237397,-58.9199683857523));
#57810=CARTESIAN_POINT('Ctrl Pts',(33.6851862294326,4.2187977606422,-58.7810965318263));
#57811=CARTESIAN_POINT('Ctrl Pts',(33.4882387352318,5.56019112234171,-58.6494224775955));
#57812=CARTESIAN_POINT('Ctrl Pts',(33.2911863744521,6.90158317509347,-58.518229027166));
#57813=CARTESIAN_POINT('Ctrl Pts',(33.0942388802513,8.24297653679298,-58.3865549729352));
#57814=CARTESIAN_POINT('Ctrl Pts',(34.2073884246238,4.23730640106381,-57.4829997732066));
#57815=CARTESIAN_POINT('Ctrl Pts',(33.9441936148297,5.57213375970279,-57.4484139032383));
#57816=CARTESIAN_POINT('Ctrl Pts',(33.6810016174677,6.90699115801177,-57.4140188439892));
#57817=CARTESIAN_POINT('Ctrl Pts',(33.4178068076735,8.24181851665074,-57.3794329740209));
#57818=CARTESIAN_POINT('Ctrl Pts',(34.7098314415821,4.34420708527133,-56.3714098124856));
#57819=CARTESIAN_POINT('Ctrl Pts',(34.3867318358801,5.66571066712957,-56.3909712140127));
#57820=CARTESIAN_POINT('Ctrl Pts',(34.063764606468,6.98719531120586,-56.409854609254));
#57821=CARTESIAN_POINT('Ctrl Pts',(33.7406650007661,8.3086988930641,-56.4294160107811));
#57822=CARTESIAN_POINT('Ctrl Pts',(35.1927431574716,4.49494117626302,-55.4098063298174));
#57823=CARTESIAN_POINT('Ctrl Pts',(34.8214509904975,5.80298260475985,-55.4445840814943));
#57824=CARTESIAN_POINT('Ctrl Pts',(34.4501548296962,7.11104892816353,-55.4807062041802));
#57825=CARTESIAN_POINT('Ctrl Pts',(34.0788626627221,8.41909035666035,-55.5154839558572));
#57826=CARTESIAN_POINT('Ctrl Pts',(35.7305102690663,4.67496655037645,-54.4301029015604));
#57827=CARTESIAN_POINT('Ctrl Pts',(35.3205130214595,5.97210422303575,-54.4388227939225));
#57828=CARTESIAN_POINT('Ctrl Pts',(34.9105277929706,7.26920952621076,-54.445846095379));
#57829=CARTESIAN_POINT('Ctrl Pts',(34.5005305453637,8.56634719887006,-54.4545659877411));
#57830=CARTESIAN_POINT('Ctrl Pts',(36.0414358248271,4.76453118953972,-53.8983393183568));
#57831=CARTESIAN_POINT('Ctrl Pts',(35.6194610289143,6.05709958470143,-53.8565986935583));
#57832=CARTESIAN_POINT('Ctrl Pts',(35.1973562738383,7.34967284882424,-53.8172409820912));
#57833=CARTESIAN_POINT('Ctrl Pts',(34.7753814779255,8.64224124398597,-53.7755003572928));
#57834=CARTESIAN_POINT('Ctrl Pts',(36.1829138277446,4.79791400485598,-53.6562428681622));
#57835=CARTESIAN_POINT('Ctrl Pts',(35.7573813489682,6.08768352765266,-53.5854142893873));
#57836=CARTESIAN_POINT('Ctrl Pts',(35.3318488701919,7.37745305044934,-53.5145857106124));
#57837=CARTESIAN_POINT('Ctrl Pts',(34.9063163914155,8.66722257324602,-53.4437571318374));
#57838=CARTESIAN_POINT('',(33.0511309501304,6.3457695123354,-59.5679999999992));
#57839=CARTESIAN_POINT('',(33.0511309501304,6.34576951233552,-59.5679999999991));
#57840=CARTESIAN_POINT('',(33.0511309501304,6.34576951233552,-59.5679999999991));
#57841=CARTESIAN_POINT('Ctrl Pts',(30.375352617956,6.01695827937672,-66.3794252415248));
#57842=CARTESIAN_POINT('Ctrl Pts',(30.3626907742229,7.26983436695969,-65.8504689498228));
#57843=CARTESIAN_POINT('Ctrl Pts',(30.3500289284736,8.52271045531506,-65.321512657339));
#57844=CARTESIAN_POINT('Ctrl Pts',(30.3373670847405,9.77558654289799,-64.7925563656371));
#57845=CARTESIAN_POINT('Ctrl Pts',(30.7734080472794,5.72447156348205,-65.6771181764558));
#57846=CARTESIAN_POINT('Ctrl Pts',(30.7448485850692,6.99344565155228,-65.1864226761427));
#57847=CARTESIAN_POINT('Ctrl Pts',(30.7168558233171,8.26220262947483,-64.6959469190092));
#57848=CARTESIAN_POINT('Ctrl Pts',(30.6882963446928,9.53117672383348,-64.2052514123314));
#57849=CARTESIAN_POINT('Ctrl Pts',(31.4978212248027,5.28838709683457,-64.4647878013927));
#57850=CARTESIAN_POINT('Ctrl Pts',(31.4326417736021,6.58333296740239,-64.0472546764288));
#57851=CARTESIAN_POINT('Ctrl Pts',(31.3670636236145,7.87843336812688,-63.6295773598725));
#57852=CARTESIAN_POINT('Ctrl Pts',(31.3018841839619,9.17337923421885,-63.212044239085));
#57853=CARTESIAN_POINT('Ctrl Pts',(32.3856289559011,4.77997444759906,-62.3963211915439));
#57854=CARTESIAN_POINT('Ctrl Pts',(32.2825028323417,6.09671440776364,-62.0695151547111));
#57855=CARTESIAN_POINT('Ctrl Pts',(32.1795677235084,7.4133780774859,-61.7427677520746));
#57856=CARTESIAN_POINT('Ctrl Pts',(32.0764415944165,8.73011803986018,-61.4159617135434));
#57857=CARTESIAN_POINT('Ctrl Pts',(32.8375602373923,4.5442896682234,-61.1512919674956));
#57858=CARTESIAN_POINT('Ctrl Pts',(32.7118681225965,5.86835965228387,-60.8667666847735));
#57859=CARTESIAN_POINT('Ctrl Pts',(32.5860717505013,7.19248099999695,-60.5822170975346));
#57860=CARTESIAN_POINT('Ctrl Pts',(32.4603796387252,8.5165509825697,-60.2976918155163));
#57861=CARTESIAN_POINT('Ctrl Pts',(33.092150020816,4.4293908705056,-60.4613447566517));
#57862=CARTESIAN_POINT('Ctrl Pts',(32.9499790526618,5.75660571904382,-60.2002657624891));
#57863=CARTESIAN_POINT('Ctrl Pts',(32.8078113847281,7.08377427021025,-59.9392806852867));
#57864=CARTESIAN_POINT('Ctrl Pts',(32.6656404164781,8.41098912008943,-59.6782016884039));
#57865=CARTESIAN_POINT('Ctrl Pts',(33.2133454585014,4.37993800979747,-60.1301118440788));
#57866=CARTESIAN_POINT('Ctrl Pts',(33.0621641363232,5.70821979358271,-59.8801414619397));
#57867=CARTESIAN_POINT('Ctrl Pts',(32.9109493382996,7.03658498637352,-59.6302488962229));
#57868=CARTESIAN_POINT('Ctrl Pts',(32.7597680170911,8.36486676774288,-59.3802785118299));
#57869=CARTESIAN_POINT('Ctrl Pts',(33.287043479682,4.35253469193526,-59.9326371198377));
#57870=CARTESIAN_POINT('Ctrl Pts',(33.1297671012815,5.68137677156017,-59.6895395217589));
#57871=CARTESIAN_POINT('Ctrl Pts',(32.9724907235957,7.01021884940405,-59.4464419220186));
#57872=CARTESIAN_POINT('Ctrl Pts',(32.8152143451951,8.339060929029,-59.2033443239399));
#57873=CARTESIAN_POINT('',(30.3563614587248,7.89624424005165,-65.5859999999992));
#57874=CARTESIAN_POINT('Ctrl Pts',(27.8032099026773,9.23603570625547,-72.5577783044314));
#57875=CARTESIAN_POINT('Ctrl Pts',(27.8052592514418,10.4382369274192,-71.9219261014769));
#57876=CARTESIAN_POINT('Ctrl Pts',(27.8073086002062,11.6404381485829,-71.2860738985224));
#57877=CARTESIAN_POINT('Ctrl Pts',(27.8093579489706,12.8426393697467,-70.6502216955679));
#57878=CARTESIAN_POINT('Ctrl Pts',(28.1510242423018,8.65285503600956,-71.4562837782078));
#57879=CARTESIAN_POINT('Ctrl Pts',(28.1527242375236,9.84564349530056,-70.802192004818));
#57880=CARTESIAN_POINT('Ctrl Pts',(28.1514837747999,11.0390178223757,-70.1505238587518));
#57881=CARTESIAN_POINT('Ctrl Pts',(28.1531837700217,12.2318062816667,-69.496432085362));
#57882=CARTESIAN_POINT('Ctrl Pts',(28.8443112604251,7.45365732155485,-69.2995688107867));
#57883=CARTESIAN_POINT('Ctrl Pts',(28.8647942312408,8.64083812394836,-68.6377099178768));
#57884=CARTESIAN_POINT('Ctrl Pts',(28.8876145388117,9.82698901941381,-67.9773229033855));
#57885=CARTESIAN_POINT('Ctrl Pts',(28.9080975096274,11.0141698218073,-67.3154640104755));
#57886=CARTESIAN_POINT('Ctrl Pts',(29.7346820906896,6.49856484963839,-67.5354860661677));
#57887=CARTESIAN_POINT('Ctrl Pts',(29.7474671388954,7.71803436653537,-66.9293044052007));
#57888=CARTESIAN_POINT('Ctrl Pts',(29.7599684642251,8.93844313064385,-66.3179762113913));
#57889=CARTESIAN_POINT('Ctrl Pts',(29.7727535124309,10.1579126475408,-65.7117945504243));
#57890=CARTESIAN_POINT('Ctrl Pts',(30.3753540341101,6.01695723880264,-66.3794227429407));
#57891=CARTESIAN_POINT('Ctrl Pts',(30.3626923171866,7.26981523963531,-65.8504742476464));
#57892=CARTESIAN_POINT('Ctrl Pts',(30.3500306002631,8.52267324046798,-65.321525752352));
#57893=CARTESIAN_POINT('Ctrl Pts',(30.3373688833396,9.77553124130065,-64.7925772570577));
#57894=CARTESIAN_POINT('',(27.806283925824,11.0393375380011,-71.6039999999996));
#57895=CARTESIAN_POINT('Ctrl Pts',(25.9521939365417,12.4413225404487,-78.5797210091187));
#57896=CARTESIAN_POINT('Ctrl Pts',(25.9541384795002,13.6421300392938,-77.9412403363729));
#57897=CARTESIAN_POINT('Ctrl Pts',(25.9560830224588,14.842937538139,-77.3027596636271));
#57898=CARTESIAN_POINT('Ctrl Pts',(25.9580275654173,16.0437450369841,-76.6642789908813));
#57899=CARTESIAN_POINT('Ctrl Pts',(26.6489056111189,11.3582252904424,-76.5448332365292));
#57900=CARTESIAN_POINT('Ctrl Pts',(26.6512972678507,12.5584545103135,-75.9052703277155));
#57901=CARTESIAN_POINT('Ctrl Pts',(26.6535845911736,13.7589674719392,-75.2662287814246));
#57902=CARTESIAN_POINT('Ctrl Pts',(26.6559762479054,14.9591966918103,-74.6266658726109));
#57903=CARTESIAN_POINT('Ctrl Pts',(27.2714354678562,10.1515799210123,-74.2870773091685));
#57904=CARTESIAN_POINT('Ctrl Pts',(27.2756644534002,11.3518792281848,-73.6476429472785));
#57905=CARTESIAN_POINT('Ctrl Pts',(27.2793717433237,12.5524667929678,-73.0087316566374));
#57906=CARTESIAN_POINT('Ctrl Pts',(27.2836007288677,13.7527661001403,-72.3692972947473));
#57907=CARTESIAN_POINT('Ctrl Pts',(27.8032099026773,9.23603570625547,-72.5577783044313));
#57908=CARTESIAN_POINT('Ctrl Pts',(27.8052592514418,10.4382369274192,-71.9219261014769));
#57909=CARTESIAN_POINT('Ctrl Pts',(27.8073086002062,11.6404381485829,-71.2860738985224));
#57910=CARTESIAN_POINT('Ctrl Pts',(27.8093579489706,12.8426393697467,-70.6502216955679));
#57911=CARTESIAN_POINT('',(25.9551107509795,14.2425337887164,-77.622));
#57912=CARTESIAN_POINT('Ctrl Pts',(25.7013237933716,12.8213530409933,-79.2937211639668));
#57913=CARTESIAN_POINT('Ctrl Pts',(25.703107932115,14.0221614010657,-78.6552400332983));
#57914=CARTESIAN_POINT('Ctrl Pts',(25.7048920708584,15.222969761138,-78.0167589026299));
#57915=CARTESIAN_POINT('Ctrl Pts',(25.7066762096018,16.4237781212104,-77.3782777719614));
#57916=CARTESIAN_POINT('Ctrl Pts',(25.7858423841264,12.6969189363309,-79.0599308245275));
#57917=CARTESIAN_POINT('Ctrl Pts',(25.7876841876523,13.8977272296109,-78.4214497293732));
#57918=CARTESIAN_POINT('Ctrl Pts',(25.7895259902168,15.098535522888,-77.7829686342204));
#57919=CARTESIAN_POINT('Ctrl Pts',(25.7913677937427,16.299343816168,-77.1444875390661));
#57920=CARTESIAN_POINT('Ctrl Pts',(25.8694745378322,12.5700031119249,-78.8214820370544));
#57921=CARTESIAN_POINT('Ctrl Pts',(25.8713700338312,13.7708113397676,-78.1830009766937));
#57922=CARTESIAN_POINT('Ctrl Pts',(25.8732655270703,14.9716195676109,-77.5445199163328));
#57923=CARTESIAN_POINT('Ctrl Pts',(25.8751610230693,16.1724277954536,-76.9060388559721));
#57924=CARTESIAN_POINT('Ctrl Pts',(25.9521939365416,12.4413225404487,-78.5797210091187));
#57925=CARTESIAN_POINT('Ctrl Pts',(25.9541384805804,13.6421307063697,-77.9412399816823));
#57926=CARTESIAN_POINT('Ctrl Pts',(25.9560830246193,14.8429388722908,-77.302758954246));
#57927=CARTESIAN_POINT('Ctrl Pts',(25.9580275686581,16.0437470382118,-76.6642779268097));
#57928=CARTESIAN_POINT('',(25.704,14.6225645804879,-78.336));
#57929=CARTESIAN_POINT('Ctrl Pts',(16.6868359538665,-0.000191536951231605,
0.654121073022559));
#57930=CARTESIAN_POINT('Ctrl Pts',(16.6871130009561,1.35958001992956,0.626822611164732));
#57931=CARTESIAN_POINT('Ctrl Pts',(16.6873900829518,2.71935102913423,0.599523466282213));
#57932=CARTESIAN_POINT('Ctrl Pts',(16.6876671300389,4.07912258605159,0.572225004469986));
#57933=CARTESIAN_POINT('Ctrl Pts',(16.4198213451363,-0.0072139952602401,
0.301563721594622));
#57934=CARTESIAN_POINT('Ctrl Pts',(16.4149483564531,1.35222993480795,0.260719814132208));
#57935=CARTESIAN_POINT('Ctrl Pts',(16.4100641886526,2.71184728945692,0.220092277311395));
#57936=CARTESIAN_POINT('Ctrl Pts',(16.4051912007158,4.07129120794696,0.179248355403675));
#57937=CARTESIAN_POINT('Ctrl Pts',(15.9097730333143,-0.035107207618914,
-0.369838110396843));
#57938=CARTESIAN_POINT('Ctrl Pts',(15.8868427712196,1.32341742242539,-0.442089514816164));
#57939=CARTESIAN_POINT('Ctrl Pts',(15.8641357832454,2.68219337959501,-0.514193315526313));
#57940=CARTESIAN_POINT('Ctrl Pts',(15.8412055062445,4.04071799286026,-0.586444729799931));
#57941=CARTESIAN_POINT('Ctrl Pts',(15.1895782981127,-0.127632624932323,
-1.30811589893802));
#57942=CARTESIAN_POINT('Ctrl Pts',(15.1168866283587,1.22525531384823,-1.4352518979635));
#57943=CARTESIAN_POINT('Ctrl Pts',(15.0450007447708,2.57878997793115,-1.56159595966525));
#57944=CARTESIAN_POINT('Ctrl Pts',(14.972309021221,3.93167787353513,-1.68873201156193));
#57945=CARTESIAN_POINT('Ctrl Pts',(14.4478451522131,-0.294302251982803,
-2.24397964816492));
#57946=CARTESIAN_POINT('Ctrl Pts',(14.3065594477978,1.04741687112848,-2.42449959114297));
#57947=CARTESIAN_POINT('Ctrl Pts',(14.1657723022977,2.38986935560785,-2.60458130729388));
#57948=CARTESIAN_POINT('Ctrl Pts',(14.0244865645977,3.73158842975856,-2.78510127952877));
#57949=CARTESIAN_POINT('Ctrl Pts',(13.3090122220842,-0.649992640739952,
-3.60728200843994));
#57950=CARTESIAN_POINT('Ctrl Pts',(13.0576846605298,0.667403037119348,-3.84500082344613));
#57951=CARTESIAN_POINT('Ctrl Pts',(12.8072569661008,1.98553821670635,-4.08237633541932));
#57952=CARTESIAN_POINT('Ctrl Pts',(12.5559293444697,3.30293384519514,-4.32009517334507));
#57953=CARTESIAN_POINT('Ctrl Pts',(12.4227603814739,-1.01957344555764,-4.524504549358));
#57954=CARTESIAN_POINT('Ctrl Pts',(12.127008354679,0.290201594277321,-4.74199275926332));
#57955=CARTESIAN_POINT('Ctrl Pts',(11.8349318621356,1.60395062323898,-4.95610715005898));
#57956=CARTESIAN_POINT('Ctrl Pts',(11.5391795899552,2.91372539776307,-5.17359558520671));
#57957=CARTESIAN_POINT('Ctrl Pts',(11.7462901651811,-1.24921324929923,-5.16107659537416));
#57958=CARTESIAN_POINT('Ctrl Pts',(11.4529263608345,0.0686917034324408,
-5.32475380701892));
#57959=CARTESIAN_POINT('Ctrl Pts',(11.159558691757,1.38659247768001,-5.48843456601537));
#57960=CARTESIAN_POINT('Ctrl Pts',(10.8661948876683,2.70449743069063,-5.65211177742331));
#57961=CARTESIAN_POINT('',(11.3069663320366,0.727806741256165,-5.40599999999995));
#57962=CARTESIAN_POINT('',(11.3069663320366,0.727806741256156,-5.40599999999995));
#57963=CARTESIAN_POINT('',(16.6863859277573,2.03937401791753,0.612000000000006));
#57964=CARTESIAN_POINT('',(11.3069663320366,0.727806741256156,-5.40599999999995));
#57965=CARTESIAN_POINT('Ctrl Pts',(21.143061504949,0.000717013383189635,
6.63001173766479));
#57966=CARTESIAN_POINT('Ctrl Pts',(21.1420934966245,1.36071666886059,6.63000391255492));
#57967=CARTESIAN_POINT('Ctrl Pts',(21.1411254883,2.72071632433799,6.62999608744506));
#57968=CARTESIAN_POINT('Ctrl Pts',(21.1401574799756,4.0807159798154,6.62998826233519));
#57969=CARTESIAN_POINT('Ctrl Pts',(20.7896206018235,0.000462775210329253,
6.1661088491225));
#57970=CARTESIAN_POINT('Ctrl Pts',(20.7886536144186,1.36046223337728,6.16578937691944));
#57971=CARTESIAN_POINT('Ctrl Pts',(20.7876658550932,2.72046226560781,6.16549015689824));
#57972=CARTESIAN_POINT('Ctrl Pts',(20.7866988676883,4.08046172377477,6.16517068469518));
#57973=CARTESIAN_POINT('Ctrl Pts',(20.2242344700564,-0.000331798776586382,
5.42457815226979));
#57974=CARTESIAN_POINT('Ctrl Pts',(20.2234969692448,1.359668566771,5.42428041199225));
#57975=CARTESIAN_POINT('Ctrl Pts',(20.2227569926779,2.71966965367535,5.42402726122232));
#57976=CARTESIAN_POINT('Ctrl Pts',(20.2220194918663,4.07967001922293,5.42372952094477));
#57977=CARTESIAN_POINT('Ctrl Pts',(19.3349512314561,0.000515684789920872,
4.24013268454022));
#57978=CARTESIAN_POINT('Ctrl Pts',(19.3369098147026,1.36051510559572,4.24122795422388));
#57979=CARTESIAN_POINT('Ctrl Pts',(19.3388458619514,2.7205156633834,4.24232412204579));
#57980=CARTESIAN_POINT('Ctrl Pts',(19.3408044451979,4.08051508418919,4.24341939172945));
#57981=CARTESIAN_POINT('Ctrl Pts',(18.5712915581816,0.00384555894097715,
3.20912559098008));
#57982=CARTESIAN_POINT('Ctrl Pts',(18.5769308819044,1.36383440276467,3.21096269832565));
#57983=CARTESIAN_POINT('Ctrl Pts',(18.5826039971431,2.72382355018078,3.21280405416297));
#57984=CARTESIAN_POINT('Ctrl Pts',(18.5882433208659,4.08381239400447,3.21464116150854));
#57985=CARTESIAN_POINT('Ctrl Pts',(17.8944576250494,0.00817944857551684,
2.2875691909004));
#57986=CARTESIAN_POINT('Ctrl Pts',(17.9030245260052,1.36815405871329,2.28703275437041));
#57987=CARTESIAN_POINT('Ctrl Pts',(17.911586634633,2.7281306172685,2.28650324952679));
#57988=CARTESIAN_POINT('Ctrl Pts',(17.9201535355888,4.08810522740628,2.28596681299679));
#57989=CARTESIAN_POINT('Ctrl Pts',(17.2634879094926,0.00962372236703112,
1.42927972685571));
#57990=CARTESIAN_POINT('Ctrl Pts',(17.2717012892452,1.36958819872823,1.42064856538643));
#57991=CARTESIAN_POINT('Ctrl Pts',(17.2799243919317,2.72955178630459,1.41200698847874));
#57992=CARTESIAN_POINT('Ctrl Pts',(17.2881377716844,4.08951626266578,1.40337582700946));
#57993=CARTESIAN_POINT('Ctrl Pts',(16.875007029906,0.0048281666224073,0.905562213293497));
#57994=CARTESIAN_POINT('Ctrl Pts',(16.8789212630212,1.36470105924659,0.885765429291508));
#57995=CARTESIAN_POINT('Ctrl Pts',(16.882837602917,2.72458396387897,0.865986258071026));
#57996=CARTESIAN_POINT('Ctrl Pts',(16.8867518360321,4.08445685650315,0.846189474069038));
#57997=CARTESIAN_POINT('Ctrl Pts',(16.6859947282585,-0.000213685071588643,
0.653010349651272));
#57998=CARTESIAN_POINT('Ctrl Pts',(16.6862555279244,1.35951145025449,0.625670116550428));
#57999=CARTESIAN_POINT('Ctrl Pts',(16.6865163275903,2.71923658558057,0.598329883449584));
#58000=CARTESIAN_POINT('Ctrl Pts',(16.6867771272561,4.07896172090665,0.57098965034874));
#58001=CARTESIAN_POINT('',(21.1416094924623,2.04071649659929,6.62999999999999));
#58002=CARTESIAN_POINT('Ctrl Pts',(25.4512489060474,0.000557793871117651,
12.6480025703997));
#58003=CARTESIAN_POINT('Ctrl Pts',(25.453101108281,1.36055653259993,12.6480008567999));
#58004=CARTESIAN_POINT('Ctrl Pts',(25.4549533105147,2.72055527132873,12.6479991432001));
#58005=CARTESIAN_POINT('Ctrl Pts',(25.4568055127483,4.08055401005754,12.6479974296003));
#58006=CARTESIAN_POINT('Ctrl Pts',(25.2761532109731,0.000795927984841995,
12.3850804994989));
#58007=CARTESIAN_POINT('Ctrl Pts',(25.277851623458,1.36079487814099,12.3850766366272));
#58008=CARTESIAN_POINT('Ctrl Pts',(25.2795515965695,2.72079382022715,12.3850728170873));
#58009=CARTESIAN_POINT('Ctrl Pts',(25.2812500090543,4.0807927703833,12.3850689542157));
#58010=CARTESIAN_POINT('Ctrl Pts',(25.0385405727546,0.00107944402204348,
12.0284981506081));
#58011=CARTESIAN_POINT('Ctrl Pts',(25.040013789292,1.36107866148558,12.0284901984931));
#58012=CARTESIAN_POINT('Ctrl Pts',(25.0414879191271,2.72107788268626,12.0284822784796));
#58013=CARTESIAN_POINT('Ctrl Pts',(25.0429611356646,4.08107710014979,12.0284743263647));
#58014=CARTESIAN_POINT('Ctrl Pts',(24.5346770904967,0.00153952329737014,
11.2801401659155));
#58015=CARTESIAN_POINT('Ctrl Pts',(24.5356564959609,1.36153920365418,11.2801229600891));
#58016=CARTESIAN_POINT('Ctrl Pts',(24.5366361205139,2.72153887642349,11.2801057514123));
#58017=CARTESIAN_POINT('Ctrl Pts',(24.5376155259781,4.08153855678031,11.2800885455859));
#58018=CARTESIAN_POINT('Ctrl Pts',(23.7748717062593,0.00195060306715209,
10.1720733370841));
#58019=CARTESIAN_POINT('Ctrl Pts',(23.7751011060668,1.36195069280139,10.1720434504722));
#58020=CARTESIAN_POINT('Ctrl Pts',(23.7753283620544,2.72195078848062,10.1720135255144));
#58021=CARTESIAN_POINT('Ctrl Pts',(23.7755577618618,4.08195087821486,10.1719836389024));
#58022=CARTESIAN_POINT('Ctrl Pts',(22.5874547933106,0.00176250665503241,
8.52818644438044));
#58023=CARTESIAN_POINT('Ctrl Pts',(22.5867557909889,1.36176241103452,8.52815645805608));
#58024=CARTESIAN_POINT('Ctrl Pts',(22.5860591031456,2.72176230689818,8.52812649967298));
#58025=CARTESIAN_POINT('Ctrl Pts',(22.5853601008239,4.08176221127767,8.52809651334861));
#58026=CARTESIAN_POINT('Ctrl Pts',(21.7214346225638,0.00113305483753488,
7.38990420970681));
#58027=CARTESIAN_POINT('Ctrl Pts',(21.7204825968315,1.36113270990459,7.38988970735517));
#58028=CARTESIAN_POINT('Ctrl Pts',(21.7195116027229,2.72113238671198,7.38987483226514));
#58029=CARTESIAN_POINT('Ctrl Pts',(21.7185595769906,4.08113204177903,7.3898603299135));
#58030=CARTESIAN_POINT('Ctrl Pts',(21.143061504949,0.000717013383189635,
6.63001173766479));
#58031=CARTESIAN_POINT('Ctrl Pts',(21.1420934966245,1.36071666886059,6.63000391255492));
#58032=CARTESIAN_POINT('Ctrl Pts',(21.1411254883,2.72071632433799,6.62999608744506));
#58033=CARTESIAN_POINT('Ctrl Pts',(21.1401574799756,4.0807159798154,6.62998826233519));
#58034=CARTESIAN_POINT('',(25.4540272093978,2.04055590196433,12.648));
#58035=CARTESIAN_POINT('Ctrl Pts',(30.3222847700924,-0.00413483878088493,
18.6660068644751));
#58036=CARTESIAN_POINT('Ctrl Pts',(30.319338154389,1.35586263314915,18.6660022881605));
#58037=CARTESIAN_POINT('Ctrl Pts',(30.3163915386857,2.71586010507919,18.6659977118459));
#58038=CARTESIAN_POINT('Ctrl Pts',(30.3134449229822,4.07585757700923,18.6659931355313));
#58039=CARTESIAN_POINT('Ctrl Pts',(28.1822868666683,-0.00877780704942276,
16.7706615754742));
#58040=CARTESIAN_POINT('Ctrl Pts',(28.1864353099662,1.35122688309983,16.7706138302738));
#58041=CARTESIAN_POINT('Ctrl Pts',(28.1920233651988,2.71125915457337,16.7706168674462));
#58042=CARTESIAN_POINT('Ctrl Pts',(28.1961718099026,4.07126384474955,16.7705691222953));
#58043=CARTESIAN_POINT('Ctrl Pts',(26.9814250093985,-0.0015252724597002,
14.9457017822533));
#58044=CARTESIAN_POINT('Ctrl Pts',(26.9842959290968,1.35846869411807,14.9457149724762));
#58045=CARTESIAN_POINT('Ctrl Pts',(26.9881290061344,2.71847349676129,14.9457374841088));
#58046=CARTESIAN_POINT('Ctrl Pts',(26.9909999267723,4.07846746334965,14.9457506743408));
#58047=CARTESIAN_POINT('Ctrl Pts',(25.4512489033343,0.000555801717781314,
12.6480025704022));
#58048=CARTESIAN_POINT('Ctrl Pts',(25.4531011064722,1.36055520449771,12.6480008568016));
#58049=CARTESIAN_POINT('Ctrl Pts',(25.4549533096103,2.72055460727762,12.6479991432009));
#58050=CARTESIAN_POINT('Ctrl Pts',(25.4568055127483,4.08055401005754,12.6479974296003));
#58051=CARTESIAN_POINT('',(30.3178648443792,2.03586236518943,18.6659999999999));
#58052=CARTESIAN_POINT('Ctrl Pts',(44.3060709912999,0.501825342747216,24.6840442872876));
#58053=CARTESIAN_POINT('Ctrl Pts',(44.2037274807061,1.85798098503677,24.684066745284));
#58054=CARTESIAN_POINT('Ctrl Pts',(44.1013837137367,3.21413663472216,24.684089198907));
#58055=CARTESIAN_POINT('Ctrl Pts',(43.9990402031475,4.5702922770116,24.6841116569036));
#58056=CARTESIAN_POINT('Ctrl Pts',(43.5190253308226,0.442431104389339,24.6077945998755));
#58057=CARTESIAN_POINT('Ctrl Pts',(43.4225063663672,1.79903503321773,24.6078001904995));
#58058=CARTESIAN_POINT('Ctrl Pts',(43.3262381461302,3.15563172830434,24.6078100586932));
#58059=CARTESIAN_POINT('Ctrl Pts',(43.2297191772901,4.51223565725923,24.6078156492424));
#58060=CARTESIAN_POINT('Ctrl Pts',(42.281953252035,0.357580859065014,24.4341272831452));
#58061=CARTESIAN_POINT('Ctrl Pts',(42.1948238660848,1.71481412833685,24.434108345902));
#58062=CARTESIAN_POINT('Ctrl Pts',(42.1075870938005,3.0720521269536,24.434087295295));
#58063=CARTESIAN_POINT('Ctrl Pts',(42.0204577097281,4.42928539614273,24.4340683580887));
#58064=CARTESIAN_POINT('Ctrl Pts',(39.7590447329804,0.209255798855571,23.9283169242352));
#58065=CARTESIAN_POINT('Ctrl Pts',(39.6912109919964,1.5676408818353,23.9282776137135));
#58066=CARTESIAN_POINT('Ctrl Pts',(39.6235574611987,2.92602127280361,23.9282403159865));
#58067=CARTESIAN_POINT('Ctrl Pts',(39.5557237170632,4.2844063558654,23.9282010054296));
#58068=CARTESIAN_POINT('Ctrl Pts',(36.2988021098604,0.0624334299665293,
22.7904348263529));
#58069=CARTESIAN_POINT('Ctrl Pts',(36.259739607807,1.42202689650176,22.7904573128975));
#58070=CARTESIAN_POINT('Ctrl Pts',(36.2205336224352,2.78162409564511,22.7904779882549));
#58071=CARTESIAN_POINT('Ctrl Pts',(36.1814711228908,4.14121756211507,22.7905004748311));
#58072=CARTESIAN_POINT('Ctrl Pts',(33.2830669754168,0.0134785075079505,
20.9642163836828));
#58073=CARTESIAN_POINT('Ctrl Pts',(33.266042022136,1.3733999950468,20.9642333108646));
#58074=CARTESIAN_POINT('Ctrl Pts',(33.2490275122761,2.73332557982227,20.964248077881));
#58075=CARTESIAN_POINT('Ctrl Pts',(33.2320025588127,4.09324706728946,20.9642650051006));
#58076=CARTESIAN_POINT('Ctrl Pts',(31.3600228082259,-0.00140329014482304,
19.5545670903082));
#58077=CARTESIAN_POINT('Ctrl Pts',(31.3529985429648,1.3585971916633,19.5545657430667));
#58078=CARTESIAN_POINT('Ctrl Pts',(31.3460228944958,2.71859422757804,19.554566141491));
#58079=CARTESIAN_POINT('Ctrl Pts',(31.3389986283846,4.07859470944643,19.5545647942189));
#58080=CARTESIAN_POINT('Ctrl Pts',(30.6632779300613,-0.00339318635361294,
18.9680312409348));
#58081=CARTESIAN_POINT('Ctrl Pts',(30.6591100208208,1.35661121146251,18.9680286797402));
#58082=CARTESIAN_POINT('Ctrl Pts',(30.6549852558424,2.71662066980922,18.968023788134));
#58083=CARTESIAN_POINT('Ctrl Pts',(30.6508173458474,4.07662506753684,18.9680212269803));
#58084=CARTESIAN_POINT('Ctrl Pts',(30.321935879594,-0.00413360349513863,
18.6656978544223));
#58085=CARTESIAN_POINT('Ctrl Pts',(30.318990489166,1.35587510023538,18.6656932760086));
#58086=CARTESIAN_POINT('Ctrl Pts',(30.3160450546095,2.71588379879152,18.6656886999778));
#58087=CARTESIAN_POINT('Ctrl Pts',(30.3130996641822,4.07589250252213,18.6656841215641));
#58088=CARTESIAN_POINT('',(44.1517615497858,2.53598100128542,24.684));
#58089=CARTESIAN_POINT('Ctrl Pts',(49.367596314931,0.956500241803234,24.6840252060176));
#58090=CARTESIAN_POINT('Ctrl Pts',(49.2262927990192,2.30914179729203,24.6840084019793));
#58091=CARTESIAN_POINT('Ctrl Pts',(49.0849892831073,3.66178335278082,24.6839915979409));
#58092=CARTESIAN_POINT('Ctrl Pts',(48.9436857671955,5.01442490826962,24.6839747939026));
#58093=CARTESIAN_POINT('Ctrl Pts',(48.9249563174813,0.91026051062961,24.7319912218939));
#58094=CARTESIAN_POINT('Ctrl Pts',(48.7870744516188,2.26326030531412,24.7319949786716));
#58095=CARTESIAN_POINT('Ctrl Pts',(48.6493002916307,3.61626896125776,24.7319975111381));
#58096=CARTESIAN_POINT('Ctrl Pts',(48.5114184254269,4.96926875591419,24.7320012679197));
#58097=CARTESIAN_POINT('Ctrl Pts',(48.2454451876077,0.842024097628023,24.7841312821754));
#58098=CARTESIAN_POINT('Ctrl Pts',(48.1129276720479,2.19556213273895,24.7841582385071));
#58099=CARTESIAN_POINT('Ctrl Pts',(47.9803793431562,3.54909669207479,24.7841839725438));
#58100=CARTESIAN_POINT('Ctrl Pts',(47.8478618276941,4.90263472719673,24.7842109288793));
#58101=CARTESIAN_POINT('Ctrl Pts',(46.6888479202391,0.694486082024801,24.8361224907741));
#58102=CARTESIAN_POINT('Ctrl Pts',(46.5684234944341,2.04917028244214,24.8361780798375));
#58103=CARTESIAN_POINT('Ctrl Pts',(46.4481124839905,3.40386435489333,24.8362331625796));
#58104=CARTESIAN_POINT('Ctrl Pts',(46.3276880578261,4.75854855527939,24.8362887516446));
#58105=CARTESIAN_POINT('Ctrl Pts',(45.4053646426555,0.584777912483909,24.7905806974873));
#58106=CARTESIAN_POINT('Ctrl Pts',(45.2947746656324,1.94030222186044,24.7906247929504));
#58107=CARTESIAN_POINT('Ctrl Pts',(45.1841696299648,3.29582325494898,24.7906652802213));
#58108=CARTESIAN_POINT('Ctrl Pts',(45.0735796529894,4.65134756433589,24.7907093756959));
#58109=CARTESIAN_POINT('Ctrl Pts',(44.3052665433902,0.501764637226404,24.6839663391593));
#58110=CARTESIAN_POINT('Ctrl Pts',(44.202929718831,1.85791102879411,24.6839887797553));
#58111=CARTESIAN_POINT('Ctrl Pts',(44.1005928942718,3.21405742036182,24.6840112203513));
#58112=CARTESIAN_POINT('Ctrl Pts',(43.9982560697126,4.57020381192954,24.6840336609473));
#58113=CARTESIAN_POINT('',(49.1556413769138,2.98545936007418,24.684));
#58114=CARTESIAN_POINT('Ctrl Pts',(61.5167105273182,2.54668955743568,18.6668749079439));
#58115=CARTESIAN_POINT('Ctrl Pts',(61.3290483861646,3.89369298763947,18.6662363925884));
#58116=CARTESIAN_POINT('Ctrl Pts',(61.1413862320074,5.24069641592315,18.6655978761149));
#58117=CARTESIAN_POINT('Ctrl Pts',(60.9537240908538,6.58769984612695,18.6649593607594));
#58118=CARTESIAN_POINT('Ctrl Pts',(61.263103455342,2.51156902512523,19.1131892935311));
#58119=CARTESIAN_POINT('Ctrl Pts',(61.0749027843424,3.85849731336309,19.1127174727806));
#58120=CARTESIAN_POINT('Ctrl Pts',(60.8867721832384,5.20543594818961,19.1122516770937));
#58121=CARTESIAN_POINT('Ctrl Pts',(60.6985715121748,6.55236423641801,19.1117798563378));
#58122=CARTESIAN_POINT('Ctrl Pts',(60.590040319334,2.41777554679417,20.1912494551796));
#58123=CARTESIAN_POINT('Ctrl Pts',(60.4003560171827,3.76449700545968,20.191255703466));
#58124=CARTESIAN_POINT('Ctrl Pts',(60.2106481477568,5.1112145815907,20.1912513624428));
#58125=CARTESIAN_POINT('Ctrl Pts',(60.0209638456271,6.45793604025974,20.1912576107388));
#58126=CARTESIAN_POINT('Ctrl Pts',(59.4895781905362,2.26151401138549,21.4128488549465));
#58127=CARTESIAN_POINT('Ctrl Pts',(59.2977245032483,3.60792694709506,21.4133840492524));
#58128=CARTESIAN_POINT('Ctrl Pts',(59.1058315470634,4.9543338671036,21.413920162527));
#58129=CARTESIAN_POINT('Ctrl Pts',(58.9139778598114,6.30074680281867,21.414455356832));
#58130=CARTESIAN_POINT('Ctrl Pts',(57.9960406900284,2.04849564503984,22.3558602231261));
#58131=CARTESIAN_POINT('Ctrl Pts',(57.8047660818527,3.39499098804245,22.3564123469393));
#58132=CARTESIAN_POINT('Ctrl Pts',(57.6135147306327,4.74148873290627,22.3569599420449));
#58133=CARTESIAN_POINT('Ctrl Pts',(57.4222401224356,6.08798407590668,22.3575120658621));
#58134=CARTESIAN_POINT('Ctrl Pts',(57.0698741394985,1.91749687991536,22.7723218917253));
#58135=CARTESIAN_POINT('Ctrl Pts',(56.8805882431121,3.2642740689222,22.7727214343706));
#58136=CARTESIAN_POINT('Ctrl Pts',(56.6912424961737,4.61104196764428,22.7731176132384));
#58137=CARTESIAN_POINT('Ctrl Pts',(56.501956599842,5.95781915665962,22.7735171558868));
#58138=CARTESIAN_POINT('Ctrl Pts',(56.3512933832801,1.81739755300788,23.0411120395903));
#58139=CARTESIAN_POINT('Ctrl Pts',(56.1644223104387,3.16451153197724,23.041370704679));
#58140=CARTESIAN_POINT('Ctrl Pts',(55.9776124637286,4.51163236434906,23.0416218085428));
#58141=CARTESIAN_POINT('Ctrl Pts',(55.7907413908312,5.85874634331215,23.0418804736386));
#58142=CARTESIAN_POINT('Ctrl Pts',(55.9375938125836,1.76021042751909,23.1895737845226));
#58143=CARTESIAN_POINT('Ctrl Pts',(55.7523080868053,3.10754254014476,23.1897559420741));
#58144=CARTESIAN_POINT('Ctrl Pts',(55.5670201212181,4.45487370505996,23.189930543941));
#58145=CARTESIAN_POINT('Ctrl Pts',(55.3817343954418,5.8022058176865,23.1901127014995));
#58146=CARTESIAN_POINT('Ctrl Pts',(54.7224264440694,1.59337924540381,23.5835239931621));
#58147=CARTESIAN_POINT('Ctrl Pts',(54.5425349310206,2.94145569457832,23.5834560816272));
#58148=CARTESIAN_POINT('Ctrl Pts',(54.362649133093,4.28952928057054,23.5833833295269));
#58149=CARTESIAN_POINT('Ctrl Pts',(54.182757620039,5.63760572974766,23.5833154179965));
#58150=CARTESIAN_POINT('Ctrl Pts',(52.3183753604669,1.28300286500095,24.2171514519698));
#58151=CARTESIAN_POINT('Ctrl Pts',(52.1541392715394,2.63311089716375,24.2169378345412));
#58152=CARTESIAN_POINT('Ctrl Pts',(51.9899010441846,3.98322045499549,24.2167309505167));
#58153=CARTESIAN_POINT('Ctrl Pts',(51.825664955259,5.3333284871569,24.2165173330819));
#58154=CARTESIAN_POINT('Ctrl Pts',(50.3762919306573,1.06185100093138,24.574737313459));
#58155=CARTESIAN_POINT('Ctrl Pts',(50.2270882512909,2.41367972324444,24.574684778323));
#58156=CARTESIAN_POINT('Ctrl Pts',(50.0779440671583,3.76551046496078,24.5746027634213));
#58157=CARTESIAN_POINT('Ctrl Pts',(49.9287403877375,5.11733918727201,24.5745502283122));
#58158=CARTESIAN_POINT('Ctrl Pts',(49.3672237994714,0.956442455724845,24.6840657814739));
#58159=CARTESIAN_POINT('Ctrl Pts',(49.2259220751389,2.30909523778757,24.6840489905667));
#58160=CARTESIAN_POINT('Ctrl Pts',(49.0846203287234,3.66174801910072,24.6840322106014));
#58161=CARTESIAN_POINT('Ctrl Pts',(48.943318604391,5.01440080116346,24.6840154196942));
#58162=CARTESIAN_POINT('',(61.2351702347366,4.56718724108023,18.6660000000004));
#58163=CARTESIAN_POINT('Ctrl Pts',(64.4551411469049,2.94895124118378,12.643128511618));
#58164=CARTESIAN_POINT('Ctrl Pts',(64.2634490243396,4.29537004039075,12.6463761705398));
#58165=CARTESIAN_POINT('Ctrl Pts',(64.0717569017743,5.64178883959772,12.6496238294616));
#58166=CARTESIAN_POINT('Ctrl Pts',(63.880064779209,6.9882076388047,12.6528714883835));
#58167=CARTESIAN_POINT('Ctrl Pts',(64.3479516013103,2.93312045091166,12.879447083032));
#58168=CARTESIAN_POINT('Ctrl Pts',(64.1565846949601,4.27958819113799,12.8820318362782));
#58169=CARTESIAN_POINT('Ctrl Pts',(63.9654114328152,5.6260806947179,12.8844859516373));
#58170=CARTESIAN_POINT('Ctrl Pts',(63.7740445264651,6.97254843494423,12.8870707048835));
#58171=CARTESIAN_POINT('Ctrl Pts',(64.1837627981494,2.90927418572721,13.2358935474039));
#58172=CARTESIAN_POINT('Ctrl Pts',(63.9933586114422,4.25587812903196,13.2373129480525));
#58173=CARTESIAN_POINT('Ctrl Pts',(63.8027403511282,5.60245438568209,13.2388840392621));
#58174=CARTESIAN_POINT('Ctrl Pts',(63.6123361644209,6.94905832898685,13.2403034399106));
#58175=CARTESIAN_POINT('Ctrl Pts',(63.8565165085826,2.86262631538198,13.9401757025571));
#58176=CARTESIAN_POINT('Ctrl Pts',(63.6676797875646,4.2094547640839,13.9398268183957));
#58177=CARTESIAN_POINT('Ctrl Pts',(63.4788891542148,5.5562885775365,13.9394767506199));
#58178=CARTESIAN_POINT('Ctrl Pts',(63.2900524331968,6.90311702623842,13.9391278664585));
#58179=CARTESIAN_POINT('Ctrl Pts',(63.0373241745919,2.7503468228343,15.6623359995965));
#58180=CARTESIAN_POINT('Ctrl Pts',(62.853358990902,4.09784400417783,15.6578276836229));
#58181=CARTESIAN_POINT('Ctrl Pts',(62.6693095807093,5.44533158427596,15.6533087285849));
#58182=CARTESIAN_POINT('Ctrl Pts',(62.4853443970193,6.79282876561949,15.6488004126113));
#58183=CARTESIAN_POINT('Ctrl Pts',(62.1072697672375,2.62849234465526,17.6291609829972));
#58184=CARTESIAN_POINT('Ctrl Pts',(61.9211507613171,3.97569482112501,17.6267449384719));
#58185=CARTESIAN_POINT('Ctrl Pts',(61.7340069286968,5.3227604947646,17.625311906549));
#58186=CARTESIAN_POINT('Ctrl Pts',(61.5478879227764,6.66996297123436,17.6228958620238));
#58187=CARTESIAN_POINT('Ctrl Pts',(61.5166608776681,2.54670163095592,18.6669577173854));
#58188=CARTESIAN_POINT('Ctrl Pts',(61.3290004490471,3.89369203770546,18.6663192391287));
#58189=CARTESIAN_POINT('Ctrl Pts',(61.1413400204261,5.240682444455,18.665680760872));
#58190=CARTESIAN_POINT('Ctrl Pts',(60.9536795918051,6.58767285120455,18.6650422826153));
#58191=CARTESIAN_POINT('',(64.167602963057,4.96857943999424,12.6480000000007));
#58192=CARTESIAN_POINT('Ctrl Pts',(66.7631910634513,3.27249821468361,6.63302015235614));
#58193=CARTESIAN_POINT('Ctrl Pts',(66.6090104253407,4.6237288674264,6.63100671745196));
#58194=CARTESIAN_POINT('Ctrl Pts',(66.4548297872301,5.97495952016919,6.62899328254778));
#58195=CARTESIAN_POINT('Ctrl Pts',(66.3006491491196,7.32619017291198,6.62697984764361));
#58196=CARTESIAN_POINT('Ctrl Pts',(66.5144891466017,3.24514897378173,7.32332685183486));
#58197=CARTESIAN_POINT('Ctrl Pts',(66.3551290019871,4.59580056453943,7.32187855047366));
#58198=CARTESIAN_POINT('Ctrl Pts',(66.1953212237692,5.94636797561221,7.32055770621773));
#58199=CARTESIAN_POINT('Ctrl Pts',(66.0359610791546,7.29701956636991,7.31910940485653));
#58200=CARTESIAN_POINT('Ctrl Pts',(66.1915309888886,3.20756373571229,8.33471690257991));
#58201=CARTESIAN_POINT('Ctrl Pts',(66.0196634412346,4.55670888345873,8.33655180786372));
#58202=CARTESIAN_POINT('Ctrl Pts',(65.8477742059612,5.90585017783967,8.33839439268998));
#58203=CARTESIAN_POINT('Ctrl Pts',(65.6759066583072,7.25499532558611,8.34022929797379));
#58204=CARTESIAN_POINT('Ctrl Pts',(65.6053523490308,3.12335915915328,9.92777824589967));
#58205=CARTESIAN_POINT('Ctrl Pts',(65.4195611156543,4.47060257180804,9.93331106670633));
#58206=CARTESIAN_POINT('Ctrl Pts',(65.2336127473442,5.81781667090629,9.93888534635652));
#58207=CARTESIAN_POINT('Ctrl Pts',(65.0478215139677,7.16506008356105,9.94441816716317));
#58208=CARTESIAN_POINT('Ctrl Pts',(65.2980709440698,3.07680103779862,10.698179922846));
#58209=CARTESIAN_POINT('Ctrl Pts',(65.1081306893196,4.42345821365678,10.7044812911298));
#58210=CARTESIAN_POINT('Ctrl Pts',(64.9181117320464,5.77010091702523,10.7108042261835));
#58211=CARTESIAN_POINT('Ctrl Pts',(64.7281714772961,7.11675809288339,10.7171055944672));
#58212=CARTESIAN_POINT('Ctrl Pts',(64.9198814657602,3.01893190960619,11.6037177274062));
#58213=CARTESIAN_POINT('Ctrl Pts',(64.7272386716612,4.3652056163787,11.6098061088883));
#58214=CARTESIAN_POINT('Ctrl Pts',(64.5345650233203,5.71147224923531,11.6158943535898));
#58215=CARTESIAN_POINT('Ctrl Pts',(64.3419222292212,7.05774595600782,11.6219827350719));
#58216=CARTESIAN_POINT('Ctrl Pts',(64.6569638176777,2.97875922081063,12.1978206672481));
#58217=CARTESIAN_POINT('Ctrl Pts',(64.4645407384521,4.3250695329532,12.2026347082501));
#58218=CARTESIAN_POINT('Ctrl Pts',(64.2721091536059,5.67138056268601,12.2074466881067));
#58219=CARTESIAN_POINT('Ctrl Pts',(64.0796860743802,7.01769087482858,12.2122607291087));
#58220=CARTESIAN_POINT('Ctrl Pts',(64.4551411469049,2.94895124118378,12.643128511618));
#58221=CARTESIAN_POINT('Ctrl Pts',(64.2634490243396,4.29537004039075,12.6463761705398));
#58222=CARTESIAN_POINT('Ctrl Pts',(64.0717569017743,5.64178883959772,12.6496238294616));
#58223=CARTESIAN_POINT('Ctrl Pts',(63.880064779209,6.9882076388047,12.6528714883835));
#58224=CARTESIAN_POINT('',(66.5319201062854,5.2993441937978,6.62999999999987));
#58225=CARTESIAN_POINT('Ctrl Pts',(73.6772000252932,5.16855773887608,0.190556358283422));
#58226=CARTESIAN_POINT('Ctrl Pts',(73.0223213239028,6.32715830579005,0.471418061534128));
#58227=CARTESIAN_POINT('Ctrl Pts',(72.3674437003221,7.48575858003024,0.752278931816456));
#58228=CARTESIAN_POINT('Ctrl Pts',(71.7125649990545,8.64435914691087,1.03314063497225));
#58229=CARTESIAN_POINT('Ctrl Pts',(73.3568906352367,4.96394356197773,0.287771904083843));
#58230=CARTESIAN_POINT('Ctrl Pts',(72.7322924584517,6.14260682030999,0.555547261873308));
#58231=CARTESIAN_POINT('Ctrl Pts',(72.1070367739604,7.32144864826471,0.823830761013211));
#58232=CARTESIAN_POINT('Ctrl Pts',(71.4824385222558,8.500111926944,1.09160617670262));
#58233=CARTESIAN_POINT('Ctrl Pts',(72.6506490423299,4.5449564025123,0.519060452703995));
#58234=CARTESIAN_POINT('Ctrl Pts',(72.0995945512668,5.77032628529454,0.752863921322597));
#58235=CARTESIAN_POINT('Ctrl Pts',(71.5484722850479,6.99561665985264,0.986731326285281));
#58236=CARTESIAN_POINT('Ctrl Pts',(70.9974177862621,8.22098653357535,1.22053480218908));
#58237=CARTESIAN_POINT('Ctrl Pts',(71.7208328945397,4.12810236418734,0.920670038259505));
#58238=CARTESIAN_POINT('Ctrl Pts',(71.2816558446986,5.40575802043638,1.09320539300391));
#58239=CARTESIAN_POINT('Ctrl Pts',(70.8428390686283,6.68358189489245,1.26556719727816));
#58240=CARTESIAN_POINT('Ctrl Pts',(70.4036620598385,7.96123757030904,1.43810253224744));
#58241=CARTESIAN_POINT('Ctrl Pts',(71.1121435558323,3.91335904361009,1.24156644857775));
#58242=CARTESIAN_POINT('Ctrl Pts',(70.7451023181714,5.21686775824389,1.37107739155829));
#58243=CARTESIAN_POINT('Ctrl Pts',(70.3769195816328,6.52017282873975,1.50138101937032));
#58244=CARTESIAN_POINT('Ctrl Pts',(70.0098782139044,7.82368152016941,1.63089205267299));
#58245=CARTESIAN_POINT('Ctrl Pts',(70.7268083932345,3.79039665573098,1.45971612003484));
#58246=CARTESIAN_POINT('Ctrl Pts',(70.4038475319979,5.10816401749319,1.56223160793066));
#58247=CARTESIAN_POINT('Ctrl Pts',(70.0802934739855,6.42586804043829,1.66518735010833));
#58248=CARTESIAN_POINT('Ctrl Pts',(69.7573325451574,7.74363539498338,1.76770288816874));
#58249=CARTESIAN_POINT('Ctrl Pts',(70.2740603998417,3.66820000092256,1.74447590965103));
#58250=CARTESIAN_POINT('Ctrl Pts',(70.0004869733914,4.99923228800803,1.81550491446754));
#58251=CARTESIAN_POINT('Ctrl Pts',(69.7261539195068,6.33012671143447,1.88708998584075));
#58252=CARTESIAN_POINT('Ctrl Pts',(69.452580406501,7.66115898281112,1.95811905401802));
#58253=CARTESIAN_POINT('Ctrl Pts',(69.8645442359654,3.58028617064753,2.03975339886061));
#58254=CARTESIAN_POINT('Ctrl Pts',(69.6308079493548,4.91966896788311,2.08422343244304));
#58255=CARTESIAN_POINT('Ctrl Pts',(69.3961593101812,6.25895087375893,2.12935401774862));
#58256=CARTESIAN_POINT('Ctrl Pts',(69.162422919613,7.59833365949849,2.17382412659732));
#58257=CARTESIAN_POINT('Ctrl Pts',(69.6001682821458,3.53233689289179,2.25060622748988));
#58258=CARTESIAN_POINT('Ctrl Pts',(69.3891578707081,4.87579662728807,2.27944637857042));
#58259=CARTESIAN_POINT('Ctrl Pts',(69.177764953627,6.21917813634206,2.30861486850998));
#58260=CARTESIAN_POINT('Ctrl Pts',(68.9667544986049,7.56263786182499,2.33745505700294));
#58261=CARTESIAN_POINT('Ctrl Pts',(69.4542644409521,3.50811556510099,2.37266587496734));
#58262=CARTESIAN_POINT('Ctrl Pts',(69.2554779909857,4.85353840156605,2.39299440880989));
#58263=CARTESIAN_POINT('Ctrl Pts',(69.0551783441871,6.19878494315157,2.41437407306302));
#58264=CARTESIAN_POINT('Ctrl Pts',(68.8563917218001,7.54420775952879,2.43470272667616));
#58265=CARTESIAN_POINT('Ctrl Pts',(69.1063126801324,3.45392517384496,2.67613303504415));
#58266=CARTESIAN_POINT('Ctrl Pts',(68.9327041121834,4.80332717113759,2.67855721319536));
#58267=CARTESIAN_POINT('Ctrl Pts',(68.7619611221849,6.15298634546019,2.67921927385303));
#58268=CARTESIAN_POINT('Ctrl Pts',(68.5883528807529,7.50238837205674,2.68164325122055));
#58269=CARTESIAN_POINT('Ctrl Pts',(68.5226423483623,3.38434890663629,3.23347205056578));
#58270=CARTESIAN_POINT('Ctrl Pts',(68.3870872529164,4.73769746898268,3.20779650773751));
#58271=CARTESIAN_POINT('Ctrl Pts',(68.2523866052647,6.09104928826278,3.18180222884627));
#58272=CARTESIAN_POINT('Ctrl Pts',(68.1168316071785,7.44439785098028,3.15612664969976));
#58273=CARTESIAN_POINT('Ctrl Pts',(67.694496492102,3.33750087776864,4.42270985506997));
#58274=CARTESIAN_POINT('Ctrl Pts',(67.5680466748002,4.69126331549113,4.38548802714617));
#58275=CARTESIAN_POINT('Ctrl Pts',(67.4410408793703,6.04506547121618,4.34835845428985));
#58276=CARTESIAN_POINT('Ctrl Pts',(67.3145909987177,7.39882791346432,4.31113663687802));
#58277=CARTESIAN_POINT('Ctrl Pts',(67.1258634544533,3.30676257207483,5.67411595656781));
#58278=CARTESIAN_POINT('Ctrl Pts',(66.9814730735797,4.65918845340503,5.65288869680402));
#58279=CARTESIAN_POINT('Ctrl Pts',(66.83772386963,6.01163361516273,5.63136136659782));
#58280=CARTESIAN_POINT('Ctrl Pts',(66.693333561815,7.36405949868983,5.61013407264264));
#58281=CARTESIAN_POINT('Ctrl Pts',(66.8856192780979,3.28558579390195,6.3034280330774));
#58282=CARTESIAN_POINT('Ctrl Pts',(66.734365096802,4.63730028384587,6.29421068413704));
#58283=CARTESIAN_POINT('Ctrl Pts',(66.58213266316,5.9889814423923,6.28545083230468));
#58284=CARTESIAN_POINT('Ctrl Pts',(66.4308783703976,7.3406959285383,6.27623353549363));
#58285=CARTESIAN_POINT('Ctrl Pts',(66.7628337599032,3.27206241735065,6.63410327899077));
#58286=CARTESIAN_POINT('Ctrl Pts',(66.6086224407573,4.62347610990505,6.6321132270148));
#58287=CARTESIAN_POINT('Ctrl Pts',(66.4544143284188,5.97488991172763,6.63012167531874));
#58288=CARTESIAN_POINT('Ctrl Pts',(66.3002030096383,7.32630360429448,6.62813162317191));
#58289=CARTESIAN_POINT('',(72.6943757632035,6.90627177260518,0.612000000000049));
#58290=CARTESIAN_POINT('Ctrl Pts',(79.5980561168973,9.79488102600527,-1.92025417906537));
#58291=CARTESIAN_POINT('Ctrl Pts',(79.0286742320677,11.0149409033542,-1.72808096639347));
#58292=CARTESIAN_POINT('Ctrl Pts',(78.4592923472381,12.2350007807032,-1.53590775372157));
#58293=CARTESIAN_POINT('Ctrl Pts',(77.8899104624086,13.4550606580522,-1.34373454104967));
#58294=CARTESIAN_POINT('Ctrl Pts',(79.1741566879662,9.55093781207194,-1.62747314540123));
#58295=CARTESIAN_POINT('Ctrl Pts',(78.5266575000171,10.7270377262137,-1.38765912524391));
#58296=CARTESIAN_POINT('Ctrl Pts',(77.8806952279844,11.9041863724067,-1.14995078261078));
#58297=CARTESIAN_POINT('Ctrl Pts',(77.2331959798932,13.0802862455097,-0.910136680054649));
#58298=CARTESIAN_POINT('Ctrl Pts',(78.5111339416338,9.08098342033927,-1.27556034622203));
#58299=CARTESIAN_POINT('Ctrl Pts',(77.7749706051526,10.187565205955,-0.978114370073764));
#58300=CARTESIAN_POINT('Ctrl Pts',(77.0384203562647,11.2937880799109,-0.680365554578324));
#58301=CARTESIAN_POINT('Ctrl Pts',(76.3022570349242,12.4003698795714,-0.382919590280686));
#58302=CARTESIAN_POINT('Ctrl Pts',(77.4831763160976,8.21812193305731,-0.881741433435836));
#58303=CARTESIAN_POINT('Ctrl Pts',(76.6879687540478,9.26872864098366,-0.543920625490695));
#58304=CARTESIAN_POINT('Ctrl Pts',(75.8930514554952,10.3194801010249,-0.206524782939603));
#58305=CARTESIAN_POINT('Ctrl Pts',(75.0978438820867,11.3700868032869,0.131296041635168));
#58306=CARTESIAN_POINT('Ctrl Pts',(76.6699028312841,7.50475073429994,-0.627389809719394));
#58307=CARTESIAN_POINT('Ctrl Pts',(75.8605684319178,8.54015089006858,-0.277402530357528));
#58308=CARTESIAN_POINT('Ctrl Pts',(75.0508678458463,9.57527060317076,0.0726661668725478));
#58309=CARTESIAN_POINT('Ctrl Pts',(74.2415334608095,10.6106707699136,0.422653443048392));
#58310=CARTESIAN_POINT('Ctrl Pts',(75.80573025497,6.75707546613834,-0.393749096424453));
#58311=CARTESIAN_POINT('Ctrl Pts',(75.0101325640915,7.80439560667266,-0.0470408174776192));
#58312=CARTESIAN_POINT('Ctrl Pts',(74.2147230665259,8.85183366407264,0.299507495459954));
#58313=CARTESIAN_POINT('Ctrl Pts',(73.4191253682831,9.89915379999267,0.646215780666534));
#58314=CARTESIAN_POINT('Ctrl Pts',(75.0458066034774,6.13922536294966,-0.198996877529824));
#58315=CARTESIAN_POINT('Ctrl Pts',(74.2854803652574,7.21759061042868,0.132625058966034));
#58316=CARTESIAN_POINT('Ctrl Pts',(73.5239941762248,8.29496715825229,0.464731466750703));
#58317=CARTESIAN_POINT('Ctrl Pts',(72.7636679833957,9.37333244442084,0.796353384288361));
#58318=CARTESIAN_POINT('Ctrl Pts',(74.3631103004922,5.62958316749681,-0.0144852711055081));
#58319=CARTESIAN_POINT('Ctrl Pts',(73.6484856916462,6.74484315518654,0.295796529234268));
#58320=CARTESIAN_POINT('Ctrl Pts',(72.934428597165,7.86059742247381,0.60581285019285));
#58321=CARTESIAN_POINT('Ctrl Pts',(72.2198039661113,8.97585739082152,0.916094660921293));
#58322=CARTESIAN_POINT('Ctrl Pts',(73.9160929284303,5.32217497724758,0.115709478461592));
#58323=CARTESIAN_POINT('Ctrl Pts',(73.2392816264558,6.46557061287508,0.407584897130259));
#58324=CARTESIAN_POINT('Ctrl Pts',(72.5615875732502,7.60823306211348,0.699849561231062));
#58325=CARTESIAN_POINT('Ctrl Pts',(71.8847763058192,8.75162872643185,0.991724964667882));
#58326=CARTESIAN_POINT('Ctrl Pts',(73.6763794821108,5.16849021502026,0.190830237853467));
#58327=CARTESIAN_POINT('Ctrl Pts',(73.0216365149966,6.32699523020028,0.471632851257021));
#58328=CARTESIAN_POINT('Ctrl Pts',(72.3668939389581,7.48550057019518,0.752435292217885));
#58329=CARTESIAN_POINT('Ctrl Pts',(71.7121509718286,8.6440055853625,1.03323790562819));
#58330=CARTESIAN_POINT('',(78.744,11.6249350354382,-1.632));
#58331=CARTESIAN_POINT('Ctrl Pts',(-66.7631905323708,3.2722402959031,6.63310021356383));
#58332=CARTESIAN_POINT('Ctrl Pts',(-66.6089890872461,4.62364551905875,6.63108830419267));
#58333=CARTESIAN_POINT('Ctrl Pts',(-66.454788368593,5.97505083079199,6.62907615047543));
#58334=CARTESIAN_POINT('Ctrl Pts',(-66.3005869234631,7.32645605394699,6.62706424110603));
#58335=CARTESIAN_POINT('Ctrl Pts',(-66.8801520480825,3.28511688844106,6.31812745992113));
#58336=CARTESIAN_POINT('Ctrl Pts',(-66.7294154291688,4.63691492746342,6.30905636882779));
#58337=CARTESIAN_POINT('Ctrl Pts',(-66.5758074951115,5.98836287185121,6.30095103402918));
#58338=CARTESIAN_POINT('Ctrl Pts',(-66.425070897001,7.34016091341009,6.29187993593875));
#58339=CARTESIAN_POINT('Ctrl Pts',(-67.2656923328878,3.32461709132614,5.28712579307929));
#58340=CARTESIAN_POINT('Ctrl Pts',(-67.1240316027416,4.67718487149427,5.25864400138529));
#58341=CARTESIAN_POINT('Ctrl Pts',(-66.983738489829,6.02990026804461,5.22971048647717));
#58342=CARTESIAN_POINT('Ctrl Pts',(-66.8420777497741,7.38246804714321,5.201228698056));
#58343=CARTESIAN_POINT('Ctrl Pts',(-68.0947647618052,3.34327433626794,3.65883664280228));
#58344=CARTESIAN_POINT('Ctrl Pts',(-67.9826229514963,4.698415843162,3.61464625653939));
#58345=CARTESIAN_POINT('Ctrl Pts',(-67.8693904320237,6.05332680022653,3.57118515922622));
#58346=CARTESIAN_POINT('Ctrl Pts',(-67.7572486296174,7.40846830879098,3.52699476767946));
#58347=CARTESIAN_POINT('Ctrl Pts',(-69.6077567772536,3.50670424092515,2.17712360811833));
#58348=CARTESIAN_POINT('Ctrl Pts',(-69.4065126173048,4.85388456367134,2.20093078770444));
#58349=CARTESIAN_POINT('Ctrl Pts',(-69.2043637928767,6.20103120513092,2.22527031105748));
#58350=CARTESIAN_POINT('Ctrl Pts',(-69.0031196394824,7.54821152812113,2.24907748678665));
#58351=CARTESIAN_POINT('Ctrl Pts',(-71.0306840271174,3.84389883696231,1.23932043725278));
#58352=CARTESIAN_POINT('Ctrl Pts',(-70.6764707998785,5.15752311784233,1.3634613121629));
#58353=CARTESIAN_POINT('Ctrl Pts',(-70.320394059464,6.47117910808559,1.48914321767995));
#58354=CARTESIAN_POINT('Ctrl Pts',(-69.9661808457267,7.78480338873587,1.61328408142497));
#58355=CARTESIAN_POINT('Ctrl Pts',(-72.5341132600611,4.47318246023834,0.554474346147679));
#58356=CARTESIAN_POINT('Ctrl Pts',(-71.9943868391019,5.7067749223203,0.783587502056807));
#58357=CARTESIAN_POINT('Ctrl Pts',(-71.4576484705403,6.9409738913966,1.01048513921957));
#58358=CARTESIAN_POINT('Ctrl Pts',(-70.917922027932,8.17456634908429,1.23959831118061));
#58359=CARTESIAN_POINT('Ctrl Pts',(-73.321583078895,4.94156553523102,0.298504751819751));
#58360=CARTESIAN_POINT('Ctrl Pts',(-72.7013339116048,6.1223415340885,0.56395096502215));
#58361=CARTESIAN_POINT('Ctrl Pts',(-72.0773277659962,7.30357890889758,0.832614564183271));
#58362=CARTESIAN_POINT('Ctrl Pts',(-71.4570786259261,8.4843549044123,1.09806075407501));
#58363=CARTESIAN_POINT('Ctrl Pts',(-73.676698823977,5.16839729396267,0.190716795481847));
#58364=CARTESIAN_POINT('Ctrl Pts',(-73.0218655138857,6.32701710217377,0.471559009605434));
#58365=CARTESIAN_POINT('Ctrl Pts',(-72.367033153576,7.48563679373651,0.75240041035525));
#58366=CARTESIAN_POINT('Ctrl Pts',(-71.7121998434778,8.64425660194844,1.03324262448473));
#58367=CARTESIAN_POINT('',(-72.6943757632042,6.90627177261614,0.611999999999845));
#58368=CARTESIAN_POINT('',(-66.5319201062853,5.29934419379849,6.63000000000032));
#58369=CARTESIAN_POINT('Ctrl Pts',(-64.4551381252455,2.94895079490255,12.6431351787018));
#58370=CARTESIAN_POINT('Ctrl Pts',(-64.2634452441834,4.29537501555654,12.6463828262949));
#58371=CARTESIAN_POINT('Ctrl Pts',(-64.0717523568639,5.64179923490367,12.6496304767655));
#58372=CARTESIAN_POINT('Ctrl Pts',(-63.8800594758019,6.98822345555767,12.6528781243586));
#58373=CARTESIAN_POINT('Ctrl Pts',(-64.8619779760282,3.00903854327299,11.7454712505408));
#58374=CARTESIAN_POINT('Ctrl Pts',(-64.6685250414154,4.35518589975374,11.7520042315012));
#58375=CARTESIAN_POINT('Ctrl Pts',(-64.4759146079884,5.70150921150542,11.7581498076534));
#58376=CARTESIAN_POINT('Ctrl Pts',(-64.2824616665933,7.04765656656971,11.7646827917324));
#58377=CARTESIAN_POINT('Ctrl Pts',(-65.5054391943955,3.11095638268489,10.2498035257975));
#58378=CARTESIAN_POINT('Ctrl Pts',(-65.3148558476391,4.45757013432088,10.256832933587));
#58379=CARTESIAN_POINT('Ctrl Pts',(-65.1241323613641,5.80417075067127,10.2638960513912));
#58380=CARTESIAN_POINT('Ctrl Pts',(-64.9335490157358,7.150784502413,10.2709254589092));
#58381=CARTESIAN_POINT('Ctrl Pts',(-66.2655547628832,3.21663712022031,8.09409275195383));
#58382=CARTESIAN_POINT('Ctrl Pts',(-66.0972008564802,4.5662428952645,8.09485849997599));
#58383=CARTESIAN_POINT('Ctrl Pts',(-65.9290633872416,5.91588626629592,8.09554030404865));
#58384=CARTESIAN_POINT('Ctrl Pts',(-65.7607094790964,7.26549204103747,8.09630605274657));
#58385=CARTESIAN_POINT('Ctrl Pts',(-66.6023005642846,3.25480541981896,7.07959378173536));
#58386=CARTESIAN_POINT('Ctrl Pts',(-66.4447225077453,4.6056467360467,7.07797597725202));
#58387=CARTESIAN_POINT('Ctrl Pts',(-66.286993061246,5.95649409802222,7.07635049023918));
#58388=CARTESIAN_POINT('Ctrl Pts',(-66.1294150059254,7.30733541420128,7.07473268581768));
#58389=CARTESIAN_POINT('Ctrl Pts',(-66.7631928097984,3.27249840672654,6.63301530513675));
#58390=CARTESIAN_POINT('Ctrl Pts',(-66.6090115879722,4.62373450251277,6.63100185783403));
#58391=CARTESIAN_POINT('Ctrl Pts',(-66.4548303677893,5.97497059823337,6.62898841061472));
#58392=CARTESIAN_POINT('Ctrl Pts',(-66.3006491459632,7.32620669401961,6.626974963312));
#58393=CARTESIAN_POINT('',(-64.1676029630583,4.96857943999383,12.6479999999978));
#58394=CARTESIAN_POINT('Ctrl Pts',(-61.5166608776679,2.54670163095537,18.6669577173835));
#58395=CARTESIAN_POINT('Ctrl Pts',(-61.3290004490477,3.89369203770503,18.6663192391269));
#58396=CARTESIAN_POINT('Ctrl Pts',(-61.1413400204275,5.24068244445468,18.6656807608702));
#58397=CARTESIAN_POINT('Ctrl Pts',(-60.9536795918073,6.58767285120433,18.6650422826135));
#58398=CARTESIAN_POINT('Ctrl Pts',(-61.6684697611081,2.56772494628588,18.4002045982419));
#58399=CARTESIAN_POINT('Ctrl Pts',(-61.481119730636,3.91475839918527,18.3991907381346));
#58400=CARTESIAN_POINT('Ctrl Pts',(-61.2937636986685,5.26179108000234,18.3981849892633));
#58401=CARTESIAN_POINT('Ctrl Pts',(-61.1064136681965,6.60882453290174,18.397171129156));
#58402=CARTESIAN_POINT('Ctrl Pts',(-61.9625499390985,2.60814245928146,17.8557473383311));
#58403=CARTESIAN_POINT('Ctrl Pts',(-61.7759183873088,3.95527510074787,17.8539100263603));
#58404=CARTESIAN_POINT('Ctrl Pts',(-61.5892849394696,5.30240735844617,17.8520724136354));
#58405=CARTESIAN_POINT('Ctrl Pts',(-61.4026533876799,6.64953999991258,17.8502351016645));
#58406=CARTESIAN_POINT('Ctrl Pts',(-62.4381571638254,2.67212888504903,16.9059398732426));
#58407=CARTESIAN_POINT('Ctrl Pts',(-62.2525608544797,4.01940233987682,16.9030239595655));
#58408=CARTESIAN_POINT('Ctrl Pts',(-62.0669474352095,5.36667330876553,16.900120839887));
#58409=CARTESIAN_POINT('Ctrl Pts',(-61.8813511258638,6.71394676359331,16.8972049262099));
#58410=CARTESIAN_POINT('Ctrl Pts',(-62.869845927729,2.72945153992658,16.0124392072496));
#58411=CARTESIAN_POINT('Ctrl Pts',(-62.684458435686,4.07675300841687,16.0092492045648));
#58412=CARTESIAN_POINT('Ctrl Pts',(-62.499061548445,5.4240528772164,16.006063213451));
#58413=CARTESIAN_POINT('Ctrl Pts',(-62.313674056402,6.7713543457067,16.0028732107663));
#58414=CARTESIAN_POINT('Ctrl Pts',(-63.2631611554505,2.78184209774869,15.1899665862504));
#58415=CARTESIAN_POINT('Ctrl Pts',(-63.0770761206611,4.12904873315006,15.1872846774923));
#58416=CARTESIAN_POINT('Ctrl Pts',(-62.8909567545222,5.47624991104894,15.1846198515837));
#58417=CARTESIAN_POINT('Ctrl Pts',(-62.7048717197328,6.82345654645031,15.1819379428255));
#58418=CARTESIAN_POINT('Ctrl Pts',(-63.8033258621819,2.85494775855224,14.0529811384669));
#58419=CARTESIAN_POINT('Ctrl Pts',(-63.6151133268446,4.20186286915551,14.0520637506875));
#58420=CARTESIAN_POINT('Ctrl Pts',(-63.4268980880177,5.5487774251691,14.0511481765562));
#58421=CARTESIAN_POINT('Ctrl Pts',(-63.2386855526803,6.89569253577236,14.0502307887768));
#58422=CARTESIAN_POINT('Ctrl Pts',(-64.1974111237398,2.91088717513149,13.2113405564316));
#58423=CARTESIAN_POINT('Ctrl Pts',(-64.0067045174499,4.25745129117103,13.2128652412228));
#58424=CARTESIAN_POINT('Ctrl Pts',(-63.8158528480224,5.60399202465122,13.2144630026497));
#58425=CARTESIAN_POINT('Ctrl Pts',(-63.6251462417326,6.95055614069076,13.2159876874408));
#58426=CARTESIAN_POINT('Ctrl Pts',(-64.4551411469067,2.94895124118343,12.643128511615));
#58427=CARTESIAN_POINT('Ctrl Pts',(-64.2634490243411,4.29537004039036,12.6463761705368));
#58428=CARTESIAN_POINT('Ctrl Pts',(-64.0717569017755,5.64178883959729,12.6496238294587));
#58429=CARTESIAN_POINT('Ctrl Pts',(-63.88006477921,6.98820763880422,12.6528714883805));
#58430=CARTESIAN_POINT('',(-61.2351702347376,4.56718724107985,18.6659999999985));
#58431=CARTESIAN_POINT('Ctrl Pts',(-49.3675859352765,0.95649915750836,24.6840263307957));
#58432=CARTESIAN_POINT('Ctrl Pts',(-49.2262718634984,2.30924252806422,24.6840095259536));
#58433=CARTESIAN_POINT('Ctrl Pts',(-49.0849577968025,3.66198589988169,24.6839927211353));
#58434=CARTESIAN_POINT('Ctrl Pts',(-48.9436437250236,5.01472927043735,24.6839759162932));
#58435=CARTESIAN_POINT('Ctrl Pts',(-50.8584017018464,1.11223489879812,24.5224763946979));
#58436=CARTESIAN_POINT('Ctrl Pts',(-50.7056849804841,2.46382207459278,24.5223933820322));
#58437=CARTESIAN_POINT('Ctrl Pts',(-50.5522383262356,3.8152280469866,24.5223069484186));
#58438=CARTESIAN_POINT('Ctrl Pts',(-50.3995217170639,5.16681525063223,24.5222239362787));
#58439=CARTESIAN_POINT('Ctrl Pts',(-53.5751416624051,1.4341043041265,23.9491058552266));
#58440=CARTESIAN_POINT('Ctrl Pts',(-53.4005789255763,2.78302562289254,23.9487852654754));
#58441=CARTESIAN_POINT('Ctrl Pts',(-53.2260564170108,4.13196065521127,23.9484657624716));
#58442=CARTESIAN_POINT('Ctrl Pts',(-53.0514936739988,5.48088197186954,23.9481451725534));
#58443=CARTESIAN_POINT('Ctrl Pts',(-56.685826170517,1.86305916206279,22.9608139368193));
#58444=CARTESIAN_POINT('Ctrl Pts',(-56.4969209650842,3.2099809398552,22.9611535371675));
#58445=CARTESIAN_POINT('Ctrl Pts',(-56.3079639218489,4.55688980206708,22.9614916488461));
#58446=CARTESIAN_POINT('Ctrl Pts',(-56.1190587243836,5.90381158184462,22.9618312494231));
#58447=CARTESIAN_POINT('Ctrl Pts',(-58.1934501574325,2.0765014749507,22.2614053479118));
#58448=CARTESIAN_POINT('Ctrl Pts',(-58.0019534508983,3.42305945926425,22.2619900909815));
#58449=CARTESIAN_POINT('Ctrl Pts',(-57.8104611513907,4.76961709641986,22.2625761875077));
#58450=CARTESIAN_POINT('Ctrl Pts',(-57.6189644441791,6.11617508078676,22.2631609303694));
#58451=CARTESIAN_POINT('Ctrl Pts',(-59.4665491367357,2.25831996402558,21.3906391167669));
#58452=CARTESIAN_POINT('Ctrl Pts',(-59.2748532413305,3.60484625129877,21.3911333943376));
#58453=CARTESIAN_POINT('Ctrl Pts',(-59.083244425966,4.95138635507911,21.3916338266604));
#58454=CARTESIAN_POINT('Ctrl Pts',(-58.8915485171766,6.29791264022871,21.3921281032851));
#58455=CARTESIAN_POINT('Ctrl Pts',(-60.5958537618148,2.41846851546986,20.1757409355903));
#58456=CARTESIAN_POINT('Ctrl Pts',(-60.4061290637618,3.76527728555233,20.1757511768844));
#58457=CARTESIAN_POINT('Ctrl Pts',(-60.2163577444682,5.11207779893297,20.1757546912248));
#58458=CARTESIAN_POINT('Ctrl Pts',(-60.0266330535809,6.4588865702845,20.1757649335528));
#58459=CARTESIAN_POINT('Ctrl Pts',(-61.2120167280186,2.50451325219275,19.2030857378747));
#58460=CARTESIAN_POINT('Ctrl Pts',(-61.023694343456,3.85151637169761,19.2026480404633));
#58461=CARTESIAN_POINT('Ctrl Pts',(-60.8354578933919,5.19853352201533,19.2022158597943));
#58462=CARTESIAN_POINT('Ctrl Pts',(-60.6471354956212,6.54553663936365,19.201778161535));
#58463=CARTESIAN_POINT('Ctrl Pts',(-61.5166651210464,2.54670221859596,18.6669502496772));
#58464=CARTESIAN_POINT('Ctrl Pts',(-61.3289902797436,3.89379614280972,18.6663117195562));
#58465=CARTESIAN_POINT('Ctrl Pts',(-61.1413154372439,5.24089006682804,18.6656731893582));
#58466=CARTESIAN_POINT('Ctrl Pts',(-60.9536405959413,6.58798399104182,18.6650346592371));
#58467=CARTESIAN_POINT('',(-49.1556413769138,2.98545936007412,24.684));
#58468=CARTESIAN_POINT('Ctrl Pts',(-44.3052665433893,0.501764637226471,
24.6839663391592));
#58469=CARTESIAN_POINT('Ctrl Pts',(-44.2029297843719,1.85791016024482,24.6839887797408));
#58470=CARTESIAN_POINT('Ctrl Pts',(-44.1005930253547,3.21405568326316,24.6840112203225));
#58471=CARTESIAN_POINT('Ctrl Pts',(-43.9982562663373,4.57020120628151,24.6840336609041));
#58472=CARTESIAN_POINT('Ctrl Pts',(-45.8824543200059,0.620779044324047,
24.8368171284471));
#58473=CARTESIAN_POINT('Ctrl Pts',(-45.7683449707959,1.9760391843988,24.8368709823476));
#58474=CARTESIAN_POINT('Ctrl Pts',(-45.6540347061159,3.33127517894173,24.8369185616456));
#58475=CARTESIAN_POINT('Ctrl Pts',(-45.5399253572853,4.68653531906208,24.8369724155581));
#58476=CARTESIAN_POINT('Ctrl Pts',(-47.6223636079185,0.774187094160568,
24.8731447167143));
#58477=CARTESIAN_POINT('Ctrl Pts',(-47.4947624703292,2.12826193920829,24.8732119796069));
#58478=CARTESIAN_POINT('Ctrl Pts',(-47.3669515564575,3.48230662826334,24.8732654147927));
#58479=CARTESIAN_POINT('Ctrl Pts',(-47.2393504192644,4.836381473368,24.8733326777113));
#58480=CARTESIAN_POINT('Ctrl Pts',(-49.3675963149307,0.956500241803143,
24.6840252060176));
#58481=CARTESIAN_POINT('Ctrl Pts',(-49.2262928895174,2.30914093098729,24.68400840199));
#58482=CARTESIAN_POINT('Ctrl Pts',(-49.0849894641042,3.66178162017143,24.6839915979625));
#58483=CARTESIAN_POINT('Ctrl Pts',(-48.9436860386909,5.01442230935558,24.6839747939349));
#58484=CARTESIAN_POINT('',(-44.1517615497847,2.53598100128547,24.6839999999998));
#58485=CARTESIAN_POINT('Ctrl Pts',(-30.3222847657765,-0.00413284663027091,
18.6660068644689));
#58486=CARTESIAN_POINT('Ctrl Pts',(-30.3193380428039,1.35591413499973,18.6660022879877));
#58487=CARTESIAN_POINT('Ctrl Pts',(-30.3163913198313,2.71596111662972,18.6659977115065));
#58488=CARTESIAN_POINT('Ctrl Pts',(-30.3134445968586,4.07600809825972,18.6659931350253));
#58489=CARTESIAN_POINT('Ctrl Pts',(-30.7285587386581,-0.00325138912786291,
19.0258393291216));
#58490=CARTESIAN_POINT('Ctrl Pts',(-30.7242038094781,1.35678904299654,19.0258352491989));
#58491=CARTESIAN_POINT('Ctrl Pts',(-30.7197590861058,2.71683977628968,19.0258341061951));
#58492=CARTESIAN_POINT('Ctrl Pts',(-30.7154041635513,4.07688020765401,19.0258300260557));
#58493=CARTESIAN_POINT('Ctrl Pts',(-31.3846390634535,-0.00108090020159251,
19.5676919050105));
#58494=CARTESIAN_POINT('Ctrl Pts',(-31.3774453264759,1.35895950731376,19.5676938356344));
#58495=CARTESIAN_POINT('Ctrl Pts',(-31.3704111723482,2.7189902139802,19.5676927166136));
#58496=CARTESIAN_POINT('Ctrl Pts',(-31.3632174235957,4.07903062221134,19.5676946474626));
#58497=CARTESIAN_POINT('Ctrl Pts',(-32.4133598840372,0.00689348995379523,
20.3244421620242));
#58498=CARTESIAN_POINT('Ctrl Pts',(-32.4008153837116,1.36688359155885,20.3244484473944));
#58499=CARTESIAN_POINT('Ctrl Pts',(-32.3880844526511,2.72688562198433,20.3244585987986));
#58500=CARTESIAN_POINT('Ctrl Pts',(-32.3755399660813,4.08687572270922,20.3244648838835));
#58501=CARTESIAN_POINT('Ctrl Pts',(-34.9086113550027,0.0335760566375183,
22.0306340145341));
#58502=CARTESIAN_POINT('Ctrl Pts',(-34.8807089306754,1.39342690355597,22.0306646909123));
#58503=CARTESIAN_POINT('Ctrl Pts',(-34.8531425913375,2.75325176630356,22.0306876482546));
#58504=CARTESIAN_POINT('Ctrl Pts',(-34.8252401422121,4.11310261513926,22.0307183252023));
#58505=CARTESIAN_POINT('Ctrl Pts',(-37.6978937468501,0.11693363945437,23.2888479293169));
#58506=CARTESIAN_POINT('Ctrl Pts',(-37.6467464569746,1.4761094188233,23.288839788297));
#58507=CARTESIAN_POINT('Ctrl Pts',(-37.5956678603332,2.83529753697036,23.2888329740954));
#58508=CARTESIAN_POINT('Ctrl Pts',(-37.5445205653891,4.19447331542888,23.2888248329776));
#58509=CARTESIAN_POINT('Ctrl Pts',(-39.7806058664349,0.216865324193402,
23.8826917702588));
#58510=CARTESIAN_POINT('Ctrl Pts',(-39.7130039220979,1.57523767019141,23.88266191101));
#58511=CARTESIAN_POINT('Ctrl Pts',(-39.6451963213448,2.93360250982931,23.8826327869049));
#58512=CARTESIAN_POINT('Ctrl Pts',(-39.5775943921822,4.29197485638117,23.8826029276017));
#58513=CARTESIAN_POINT('Ctrl Pts',(-40.597421702395,0.259993271724183,24.084560939485));
#58514=CARTESIAN_POINT('Ctrl Pts',(-40.5232228932742,1.6180231184918,24.0845316720413));
#58515=CARTESIAN_POINT('Ctrl Pts',(-40.4491669163617,2.97605728903849,24.0845017165109));
#58516=CARTESIAN_POINT('Ctrl Pts',(-40.3749680967022,4.33408713548708,24.084472449118));
#58517=CARTESIAN_POINT('Ctrl Pts',(-41.4486629431555,0.307991395735675,
24.2719159198737));
#58518=CARTESIAN_POINT('Ctrl Pts',(-41.3679223481086,1.66564807615995,24.2718886820322));
#58519=CARTESIAN_POINT('Ctrl Pts',(-41.2870893775298,3.02330276774818,24.2718620297276));
#58520=CARTESIAN_POINT('Ctrl Pts',(-41.2063487892987,4.38095944831921,24.2718347918428));
#58521=CARTESIAN_POINT('Ctrl Pts',(-42.6707056826778,0.383592726711738,
24.4939878032503));
#58522=CARTESIAN_POINT('Ctrl Pts',(-42.5805406284222,1.7406702197844,24.4939762987861));
#58523=CARTESIAN_POINT('Ctrl Pts',(-42.4905339901398,3.09775247806375,24.493963982215));
#58524=CARTESIAN_POINT('Ctrl Pts',(-42.4003689241955,4.45482997078481,24.4939524778108));
#58525=CARTESIAN_POINT('Ctrl Pts',(-43.7457382365382,0.459542695930701,
24.6297413546134));
#58526=CARTESIAN_POINT('Ctrl Pts',(-43.6476399272098,1.81605527587309,24.6297525178164));
#58527=CARTESIAN_POINT('Ctrl Pts',(-43.5494164060833,3.17256384303449,24.6297645822975));
#58528=CARTESIAN_POINT('Ctrl Pts',(-43.4513181059938,4.52907642327296,24.629775745434));
#58529=CARTESIAN_POINT('Ctrl Pts',(-44.3052665433893,0.501764637226471,
24.6839663391592));
#58530=CARTESIAN_POINT('Ctrl Pts',(-44.2029261055258,1.85795891155164,24.6839887805475));
#58531=CARTESIAN_POINT('Ctrl Pts',(-44.1005856676623,3.21415318587681,24.6840112219359));
#58532=CARTESIAN_POINT('Ctrl Pts',(-43.9982452297988,4.57034746020199,24.6840336633242));
#58533=CARTESIAN_POINT('',(-30.3178648443797,2.03586236518953,18.6660000000004));
#58534=CARTESIAN_POINT('Ctrl Pts',(-25.4512489060473,0.000557793871136247,
12.6480025703997));
#58535=CARTESIAN_POINT('Ctrl Pts',(-25.453101108281,1.36055653259994,12.6480008567999));
#58536=CARTESIAN_POINT('Ctrl Pts',(-25.4549533105147,2.72055527132875,12.6479991432001));
#58537=CARTESIAN_POINT('Ctrl Pts',(-25.4568055127484,4.08055401005756,12.6479974296003));
#58538=CARTESIAN_POINT('Ctrl Pts',(-27.0230520916476,-0.00157989408392619,
15.008208642719));
#58539=CARTESIAN_POINT('Ctrl Pts',(-27.025967107362,1.35841338001428,15.0082212028861));
#58540=CARTESIAN_POINT('Ctrl Pts',(-27.0298213035499,2.71841742660675,15.0082464445362));
#58541=CARTESIAN_POINT('Ctrl Pts',(-27.0327363192644,4.07841070070495,15.0082590047032));
#58542=CARTESIAN_POINT('Ctrl Pts',(-28.204865633569,-0.00872682770445543,
16.7906590474112));
#58543=CARTESIAN_POINT('Ctrl Pts',(-28.2089295504538,1.35127726481958,16.7906114791363));
#58544=CARTESIAN_POINT('Ctrl Pts',(-28.2144468884787,2.71130821992859,16.7906149931826));
#58545=CARTESIAN_POINT('Ctrl Pts',(-28.2185108053635,4.07131231245263,16.7905674249077));
#58546=CARTESIAN_POINT('Ctrl Pts',(-30.3222847657765,-0.00413284663027091,
18.6660068644689));
#58547=CARTESIAN_POINT('Ctrl Pts',(-30.319338151512,1.3558639612496,18.6660022881565));
#58548=CARTESIAN_POINT('Ctrl Pts',(-30.3163915372475,2.71586076912947,18.6659977118442));
#58549=CARTESIAN_POINT('Ctrl Pts',(-30.3134449229829,4.07585757700934,18.6659931355318));
#58550=CARTESIAN_POINT('',(-25.4540272093979,2.04055590196435,12.648));
#58551=CARTESIAN_POINT('Ctrl Pts',(-21.1430615049491,0.000717013383229603,
6.63001173766484));
#58552=CARTESIAN_POINT('Ctrl Pts',(-21.1420934966246,1.36071666886063,6.63000391255497));
#58553=CARTESIAN_POINT('Ctrl Pts',(-21.1411254883001,2.72071632433803,6.6299960874451));
#58554=CARTESIAN_POINT('Ctrl Pts',(-21.1401574799756,4.08071597981543,6.62998826233523));
#58555=CARTESIAN_POINT('Ctrl Pts',(-21.8005099855675,0.00118993616216897,
7.49379695859226));
#58556=CARTESIAN_POINT('Ctrl Pts',(-21.7995582366668,1.3611895530325,7.493782020727));
#58557=CARTESIAN_POINT('Ctrl Pts',(-21.7985906509679,2.72118930903738,7.4937652269592));
#58558=CARTESIAN_POINT('Ctrl Pts',(-21.7976389020672,4.08118892590771,7.49375028909394));
#58559=CARTESIAN_POINT('Ctrl Pts',(-22.8275445640793,0.00197688629320044,
8.83972141456318));
#58560=CARTESIAN_POINT('Ctrl Pts',(-22.8269415478554,1.36197695395413,8.83968617050489));
#58561=CARTESIAN_POINT('Ctrl Pts',(-22.8263393218972,2.72197703099325,8.83965028373617));
#58562=CARTESIAN_POINT('Ctrl Pts',(-22.8257363056734,4.08197709865418,8.83961503967788));
#58563=CARTESIAN_POINT('Ctrl Pts',(-24.3932856767672,0.00180919175862648,
11.05541899507));
#58564=CARTESIAN_POINT('Ctrl Pts',(-24.3940975319706,1.36180915945558,11.0553960222686));
#58565=CARTESIAN_POINT('Ctrl Pts',(-24.3949048701553,2.72180914970329,11.0553728965359));
#58566=CARTESIAN_POINT('Ctrl Pts',(-24.3957167253587,4.08180911740025,11.0553499237346));
#58567=CARTESIAN_POINT('Ctrl Pts',(-25.1061238118938,0.0010271718212213,
12.1297659316509));
#58568=CARTESIAN_POINT('Ctrl Pts',(-25.1076729687202,1.36102630813001,12.12976051533));
#58569=CARTESIAN_POINT('Ctrl Pts',(-25.1092249488343,2.72102548600383,12.1297535835151));
#58570=CARTESIAN_POINT('Ctrl Pts',(-25.1107741056607,4.08102462231262,12.1297481671942));
#58571=CARTESIAN_POINT('Ctrl Pts',(-25.4512489060473,0.000557793871136247,
12.6480025703997));
#58572=CARTESIAN_POINT('Ctrl Pts',(-25.453101108281,1.36055653259994,12.6480008567999));
#58573=CARTESIAN_POINT('Ctrl Pts',(-25.4549533105147,2.72055527132875,12.6479991432001));
#58574=CARTESIAN_POINT('Ctrl Pts',(-25.4568055127484,4.08055401005756,12.6479974296003));
#58575=CARTESIAN_POINT('',(-21.1416094924623,2.04071649659933,6.63000000000004));
#58576=CARTESIAN_POINT('Ctrl Pts',(-16.6859947282585,-0.000213685071575598,
0.653010349651237));
#58577=CARTESIAN_POINT('Ctrl Pts',(-16.6862555279244,1.3595114502545,0.625670116550412));
#58578=CARTESIAN_POINT('Ctrl Pts',(-16.6865163275903,2.71923658558058,0.598329883449587));
#58579=CARTESIAN_POINT('Ctrl Pts',(-16.6867771272561,4.07896172090666,0.570989650348762));
#58580=CARTESIAN_POINT('Ctrl Pts',(-17.1283146873041,0.0115850794287345,
1.24402336313977));
#58581=CARTESIAN_POINT('Ctrl Pts',(-17.1369212648133,1.37157656223025,1.23410219696274));
#58582=CARTESIAN_POINT('Ctrl Pts',(-17.1461443494675,2.73182976169598,1.22492379185217));
#58583=CARTESIAN_POINT('Ctrl Pts',(-17.1547509269767,4.09182124449749,1.21500262567514));
#58584=CARTESIAN_POINT('Ctrl Pts',(-17.7995093414147,0.00861285405854421,
2.15897284032503));
#58585=CARTESIAN_POINT('Ctrl Pts',(-17.8086067249379,1.36857803218947,2.1586056624823));
#58586=CARTESIAN_POINT('Ctrl Pts',(-17.817701749899,2.72852490191836,2.15820377353535));
#58587=CARTESIAN_POINT('Ctrl Pts',(-17.8267991334222,4.08849008004929,2.15783659569263));
#58588=CARTESIAN_POINT('Ctrl Pts',(-18.6500576004548,0.00359926355307256,
3.31551610923036));
#58589=CARTESIAN_POINT('Ctrl Pts',(-18.6553153931928,1.36359151605813,3.31726183535392));
#58590=CARTESIAN_POINT('Ctrl Pts',(-18.6606491109907,2.72362743141132,3.31912211797675));
#58591=CARTESIAN_POINT('Ctrl Pts',(-18.6659069037288,4.08361968391638,3.32086784410031));
#58592=CARTESIAN_POINT('Ctrl Pts',(-19.2949742331925,0.000749258977111304,
4.18600514145956));
#58593=CARTESIAN_POINT('Ctrl Pts',(-19.2971395770759,1.36074705522213,4.18714822626292));
#58594=CARTESIAN_POINT('Ctrl Pts',(-19.2993388889085,2.72076348791444,4.18835516320786));
#58595=CARTESIAN_POINT('Ctrl Pts',(-19.3015042327919,4.08076128415945,4.18949824801122));
#58596=CARTESIAN_POINT('Ctrl Pts',(-20.1855381343016,-0.000360669926822324,
5.37385984414699));
#58597=CARTESIAN_POINT('Ctrl Pts',(-20.1848339213132,1.35964105651181,5.37362227555459));
#58598=CARTESIAN_POINT('Ctrl Pts',(-20.1841478714708,2.71966507969474,5.37343458389977));
#58599=CARTESIAN_POINT('Ctrl Pts',(-20.1834436584824,4.07966680613337,5.37319701530737));
#58600=CARTESIAN_POINT('Ctrl Pts',(-20.7645962878633,0.000444774645616996,
6.13326360844075));
#58601=CARTESIAN_POINT('Ctrl Pts',(-20.7636457870061,1.3604434450274,6.13291231871182));
#58602=CARTESIAN_POINT('Ctrl Pts',(-20.7626238007416,2.7204450515632,6.13261197194776));
#58603=CARTESIAN_POINT('Ctrl Pts',(-20.7616732998844,4.08044372194498,6.13226068221884));
#58604=CARTESIAN_POINT('Ctrl Pts',(-21.1430615049491,0.000717013383229603,
6.63001173766484));
#58605=CARTESIAN_POINT('Ctrl Pts',(-21.1420934966246,1.36071666886063,6.63000391255497));
#58606=CARTESIAN_POINT('Ctrl Pts',(-21.1411254883001,2.72071632433803,6.6299960874451));
#58607=CARTESIAN_POINT('Ctrl Pts',(-21.1401574799756,4.08071597981543,6.62998826233523));
#58608=CARTESIAN_POINT('',(-16.6863859277573,2.03937401791754,0.611999999999999));
#58609=CARTESIAN_POINT('Ctrl Pts',(-11.7469519845649,-1.24898856655025,
-5.1604537901259));
#58610=CARTESIAN_POINT('Ctrl Pts',(-11.4535903397776,0.0688879795759836,
-5.3241809848708));
#58611=CARTESIAN_POINT('Ctrl Pts',(-11.1602285866567,1.38676445662711,-5.4879087785922));
#58612=CARTESIAN_POINT('Ctrl Pts',(-10.8668669418732,2.70464100275581,-5.65163597331566));
#58613=CARTESIAN_POINT('Ctrl Pts',(-12.0050933687692,-1.16134492936906,
-4.91752211089309));
#58614=CARTESIAN_POINT('Ctrl Pts',(-11.711107008775,0.153817187963984,-5.10239435840529));
#58615=CARTESIAN_POINT('Ctrl Pts',(-11.4176900288694,1.46934235066558,-5.2841184918417));
#58616=CARTESIAN_POINT('Ctrl Pts',(-11.1237036484762,2.78450445499191,-5.4689908521404));
#58617=CARTESIAN_POINT('Ctrl Pts',(-12.7010765381262,-0.905927472950019,
-4.23328860522664));
#58618=CARTESIAN_POINT('Ctrl Pts',(-12.4199418855767,0.406194899132227,
-4.45475204341524));
#58619=CARTESIAN_POINT('Ctrl Pts',(-12.1385802960752,1.71818448859926,-4.67783714572155));
#58620=CARTESIAN_POINT('Ctrl Pts',(-11.8574456516561,3.03030686543866,-4.89930052581131));
#58621=CARTESIAN_POINT('Ctrl Pts',(-13.4034560583173,-0.630382964431516,
-3.47895409086386));
#58622=CARTESIAN_POINT('Ctrl Pts',(-13.1657297111913,0.690309717783447,
-3.70499001167999));
#58623=CARTESIAN_POINT('Ctrl Pts',(-12.9282670445964,2.01114267174908,-3.93059648835147));
#58624=CARTESIAN_POINT('Ctrl Pts',(-12.6905406880236,3.33183534893858,-4.15663242455316));
#58625=CARTESIAN_POINT('Ctrl Pts',(-14.2693062595799,-0.346358717812154,
-2.463047534852));
#58626=CARTESIAN_POINT('Ctrl Pts',(-14.1094732202099,0.991288087753195,
-2.65490390307943));
#58627=CARTESIAN_POINT('Ctrl Pts',(-13.9495030479015,2.3289080887949,-2.8465979544352));
#58628=CARTESIAN_POINT('Ctrl Pts',(-13.7896700134444,3.66655489532056,-3.03845432847791));
#58629=CARTESIAN_POINT('Ctrl Pts',(-14.9655514589865,-0.169147364522696,
-1.59527625944176));
#58630=CARTESIAN_POINT('Ctrl Pts',(-14.8738731361902,1.18114798058698,-1.7391436974675));
#58631=CARTESIAN_POINT('Ctrl Pts',(-14.7820906943996,2.53150537188668,-1.88363575390914));
#58632=CARTESIAN_POINT('Ctrl Pts',(-14.6904123753336,3.88180071477345,-2.02750316955686));
#58633=CARTESIAN_POINT('Ctrl Pts',(-15.8024771762679,-0.039623100750617,
-0.512730537069246));
#58634=CARTESIAN_POINT('Ctrl Pts',(-15.7752096756165,1.31866535626611,-0.59285342408472));
#58635=CARTESIAN_POINT('Ctrl Pts',(-15.7480885002328,2.67691275138139,-0.672116635479013));
#58636=CARTESIAN_POINT('Ctrl Pts',(-15.7208209943389,4.03520120986923,-0.752239553293818));
#58637=CARTESIAN_POINT('Ctrl Pts',(-16.3914419547385,-0.00797615819818137,
0.264094830899975));
#58638=CARTESIAN_POINT('Ctrl Pts',(-16.3862014526881,1.35143079639208,0.222423946339894));
#58639=CARTESIAN_POINT('Ctrl Pts',(-16.3803829115459,2.71097183412246,0.179138036275036));
#58640=CARTESIAN_POINT('Ctrl Pts',(-16.3751424302047,4.07037878390896,0.137467209575971));
#58641=CARTESIAN_POINT('Ctrl Pts',(-16.6860507767434,-0.000212207904980436,
0.653084353789295));
#58642=CARTESIAN_POINT('Ctrl Pts',(-16.6863126279545,1.35953734982766,0.625746357783578));
#58643=CARTESIAN_POINT('Ctrl Pts',(-16.6865745891456,2.71928688204919,0.598408669055888));
#58644=CARTESIAN_POINT('Ctrl Pts',(-16.6868364403527,4.07903643978274,0.571070673039161));
#58645=CARTESIAN_POINT('',(-11.3069663320367,0.727806741256162,-5.40599999999988));
#58646=CARTESIAN_POINT('',(-11.3069663320367,0.727806741256166,-5.40599999999988));
#58647=CARTESIAN_POINT('',(-11.3069663320367,0.727806741256166,-5.40599999999988));
#58648=CARTESIAN_POINT('Ctrl Pts',(6.41902973990636E-15,-1.93207323326078,
-8.62957429809281));
#58649=CARTESIAN_POINT('Ctrl Pts',(2.80278610805871E-15,-0.572138762410863,
-8.64292476603094));
#58650=CARTESIAN_POINT('Ctrl Pts',(-8.13457523788951E-16,0.78779570843905,
-8.65627523396906));
#58651=CARTESIAN_POINT('Ctrl Pts',(-4.42970115563661E-15,2.14773017928896,
-8.66962570190719));
#58652=CARTESIAN_POINT('Ctrl Pts',(-0.658062683030888,-1.93165972294369,
-8.58745240866785));
#58653=CARTESIAN_POINT('Ctrl Pts',(-0.682573404813958,-0.571376327075844,
-8.60175832749374));
#58654=CARTESIAN_POINT('Ctrl Pts',(-0.708277726456336,0.78782854621592,
-8.61643182898499));
#58655=CARTESIAN_POINT('Ctrl Pts',(-0.732788448239405,2.14811194208377,
-8.63073774781089));
#58656=CARTESIAN_POINT('Ctrl Pts',(-2.46516391286739,-1.98743098295203,
-8.49849688064982));
#58657=CARTESIAN_POINT('Ctrl Pts',(-2.55711848213956,-0.630595668642713,
-8.51587687470825));
#58658=CARTESIAN_POINT('Ctrl Pts',(-2.6481713222656,0.726813060125434,-8.53306426500673));
#58659=CARTESIAN_POINT('Ctrl Pts',(-2.74012589153777,2.08364837443475,-8.55044425906516));
#58660=CARTESIAN_POINT('Ctrl Pts',(-4.39676963179061,-2.13852225314529,
-8.46329578588585));
#58661=CARTESIAN_POINT('Ctrl Pts',(-4.48313054872813,-0.781026877589576,
-8.48236683893671));
#58662=CARTESIAN_POINT('Ctrl Pts',(-4.56966303709027,0.576336747779195,
-8.50142575891667));
#58663=CARTESIAN_POINT('Ctrl Pts',(-4.65602395402778,1.93383212333491,-8.52049681196753));
#58664=CARTESIAN_POINT('Ctrl Pts',(-6.35409454450772,-2.18205385875907,
-8.11784826271868));
#58665=CARTESIAN_POINT('Ctrl Pts',(-6.35325914215375,-0.821354211984902,
-8.1496301634349));
#58666=CARTESIAN_POINT('Ctrl Pts',(-6.35262424881583,0.539250997990761,
-8.18151670217025));
#58667=CARTESIAN_POINT('Ctrl Pts',(-6.35178884646186,1.89995064476493,-8.21329860288647));
#58668=CARTESIAN_POINT('Ctrl Pts',(-8.15537660210863,-2.1050270665009,-7.52858105609529));
#58669=CARTESIAN_POINT('Ctrl Pts',(-8.03377897269566,-0.748914208094495,
-7.58528703948586));
#58670=CARTESIAN_POINT('Ctrl Pts',(-7.91087017389806,0.607551140645141,
-7.64175911617833));
#58671=CARTESIAN_POINT('Ctrl Pts',(-7.78927254448508,1.96366399905155,-7.6984650995689));
#58672=CARTESIAN_POINT('Ctrl Pts',(-10.2097165609597,-1.7375710793364,-6.40958181990177));
#58673=CARTESIAN_POINT('Ctrl Pts',(-9.94448455848953,-0.405812797944965,
-6.52029409947421));
#58674=CARTESIAN_POINT('Ctrl Pts',(-9.68069833114861,0.925421674998247,
-6.63131671765967));
#58675=CARTESIAN_POINT('Ctrl Pts',(-9.41546632867843,2.25717995638968,-6.7420289972321));
#58676=CARTESIAN_POINT('Ctrl Pts',(-11.2781006865412,-1.40420632664524,
-5.56975094644535));
#58677=CARTESIAN_POINT('Ctrl Pts',(-10.9870984387785,-0.0845518570703568,
-5.71805524906024));
#58678=CARTESIAN_POINT('Ctrl Pts',(-10.6930379962096,1.23642612169233,-5.86563953187011));
#58679=CARTESIAN_POINT('Ctrl Pts',(-10.4020357484469,2.55608059126722,-6.013943834485));
#58680=CARTESIAN_POINT('Ctrl Pts',(-11.7470010949101,-1.24897189262896,
-5.16040757324739));
#58681=CARTESIAN_POINT('Ctrl Pts',(-11.4536445863279,0.0688805299611238,
-5.32413585774905));
#58682=CARTESIAN_POINT('Ctrl Pts',(-11.1602880777456,1.38673295255121,-5.48786414225071));
#58683=CARTESIAN_POINT('Ctrl Pts',(-10.8669315691633,2.70458537514129,-5.65159242675238));
#58684=CARTESIAN_POINT('',(0.,0.107828473014093,-8.6496));
#58685=CARTESIAN_POINT('Ctrl Pts',(-73.6764856602474,5.168558288494,0.190796964362639));
#58686=CARTESIAN_POINT('Ctrl Pts',(-73.0217457288853,6.32703394457543,0.471598988120776));
#58687=CARTESIAN_POINT('Ctrl Pts',(-72.3670057975232,7.48550960065686,0.752401011878913));
#58688=CARTESIAN_POINT('Ctrl Pts',(-71.7122658661611,8.64398525673828,1.03320303563705));
#58689=CARTESIAN_POINT('Ctrl Pts',(-74.7404207630834,5.85068057265868,-0.142609694242852));
#58690=CARTESIAN_POINT('Ctrl Pts',(-73.9872728090383,6.93979153504156,0.186818345160544));
#58691=CARTESIAN_POINT('Ctrl Pts',(-73.2316019247904,8.03256413589653,0.519523811415036));
#58692=CARTESIAN_POINT('Ctrl Pts',(-72.4784539707453,9.12167509827942,0.848951850818431));
#58693=CARTESIAN_POINT('Ctrl Pts',(-75.9741648812485,6.89428690872944,-0.412567225194581));
#58694=CARTESIAN_POINT('Ctrl Pts',(-75.1564827140154,7.91936761120769,-0.0547049712921969));
#58695=CARTESIAN_POINT('Ctrl Pts',(-74.3386463722817,8.94330795351427,0.302963615183627));
#58696=CARTESIAN_POINT('Ctrl Pts',(-73.5209642050486,9.96838865599251,0.66082586908601));
#58697=CARTESIAN_POINT('Ctrl Pts',(-77.4581499404949,8.19662250468364,-0.873282366765809));
#58698=CARTESIAN_POINT('Ctrl Pts',(-76.6611237143454,9.24570529771174,-0.534158754431353));
#58699=CARTESIAN_POINT('Ctrl Pts',(-75.8638070483209,10.2958056899081,-0.194566350790663));
#58700=CARTESIAN_POINT('Ctrl Pts',(-75.0667808221714,11.3448884829362,0.144557261543794));
#58701=CARTESIAN_POINT('Ctrl Pts',(-78.1080385927614,8.74315679055215,-1.12050093759123));
#58702=CARTESIAN_POINT('Ctrl Pts',(-77.3487456616466,9.82768503189974,-0.807299633395332));
#58703=CARTESIAN_POINT('Ctrl Pts',(-76.5890175462894,10.9122676252282,-0.493818169521655));
#58704=CARTESIAN_POINT('Ctrl Pts',(-75.8297246151746,11.9967958665758,-0.180616865325761));
#58705=CARTESIAN_POINT('Ctrl Pts',(-78.8357086373011,9.31133939639374,-1.44888811728152));
#58706=CARTESIAN_POINT('Ctrl Pts',(-78.1426077220294,10.4518303214309,-1.17933446484409));
#58707=CARTESIAN_POINT('Ctrl Pts',(-77.450171149787,11.592893117714,-0.910220255034814));
#58708=CARTESIAN_POINT('Ctrl Pts',(-76.7570702345152,12.7333840427512,-0.640666602597381));
#58709=CARTESIAN_POINT('Ctrl Pts',(-79.2776917908501,9.61051959968398,-1.69898330179011));
#58710=CARTESIAN_POINT('Ctrl Pts',(-78.6499410387911,10.7976671952425,-1.47139959830661));
#58711=CARTESIAN_POINT('Ctrl Pts',(-78.0213825166128,11.9846055748152,-1.24363766834935));
#58712=CARTESIAN_POINT('Ctrl Pts',(-77.3936317645538,13.1717531703737,-1.01605396486585));
#58713=CARTESIAN_POINT('Ctrl Pts',(-79.5980561168787,9.79488102596951,-1.92025417907613));
#58714=CARTESIAN_POINT('Ctrl Pts',(-79.0286853722929,11.0149170322628,-1.72808472635871));
#58715=CARTESIAN_POINT('Ctrl Pts',(-78.4593146277071,12.2349530385561,-1.53591527364129));
#58716=CARTESIAN_POINT('Ctrl Pts',(-77.8899438831213,13.4549890448494,-1.34374582092387));
#58717=CARTESIAN_POINT('Ctrl Pts',(11.7470010949101,-1.24897189262897,-5.16040757324743));
#58718=CARTESIAN_POINT('Ctrl Pts',(11.4536445863278,0.068880529961115,-5.32413585774911));
#58719=CARTESIAN_POINT('Ctrl Pts',(11.1602880777455,1.3867329525512,-5.48786414225079));
#58720=CARTESIAN_POINT('Ctrl Pts',(10.8669315691632,2.70458537514128,-5.65159242675248));
#58721=CARTESIAN_POINT('Ctrl Pts',(10.7125397951466,-1.59144123476306,-6.0634775436082));
#58722=CARTESIAN_POINT('Ctrl Pts',(10.4228755853451,-0.267776435549922,
-6.19166121896685));
#58723=CARTESIAN_POINT('Ctrl Pts',(10.1309691717591,1.05329780357478,-6.32280773148431));
#58724=CARTESIAN_POINT('Ctrl Pts',(9.84130496195755,2.37696260278792,-6.45099140684296));
#58725=CARTESIAN_POINT('Ctrl Pts',(9.24118021009056,-1.93913982160653,-6.97487125430323));
#58726=CARTESIAN_POINT('Ctrl Pts',(9.04250186351073,-0.593814054742301,
-7.05753687418105));
#58727=CARTESIAN_POINT('Ctrl Pts',(8.84452012731969,0.751814771731771,-7.13977225849378));
#58728=CARTESIAN_POINT('Ctrl Pts',(8.64584178073985,2.097140538596,-7.22243787837159));
#58729=CARTESIAN_POINT('Ctrl Pts',(7.87873760695008,-2.09354224390961,-7.58570787305198));
#58730=CARTESIAN_POINT('Ctrl Pts',(7.77530583020013,-0.738307891227118,
-7.64064961915395));
#58731=CARTESIAN_POINT('Ctrl Pts',(7.67158568832869,0.616720958047741,-7.69590312735252));
#58732=CARTESIAN_POINT('Ctrl Pts',(7.56815391157874,1.97195531073023,-7.75084487345448));
#58733=CARTESIAN_POINT('Ctrl Pts',(7.28211573159564,-2.13599647613335,-7.80368259116433));
#58734=CARTESIAN_POINT('Ctrl Pts',(7.21917418428538,-0.777984989202499,
-7.84880269620889));
#58735=CARTESIAN_POINT('Ctrl Pts',(7.15587550655931,0.579887102874036,-7.89407576492449));
#58736=CARTESIAN_POINT('Ctrl Pts',(7.09293395924904,1.93789858980489,-7.93919586996905));
#58737=CARTESIAN_POINT('Ctrl Pts',(6.7745203245172,-2.15695778989224,-7.96476246664597));
#58738=CARTESIAN_POINT('Ctrl Pts',(6.74319842093572,-0.797829234317486,
-8.00316656823017));
#58739=CARTESIAN_POINT('Ctrl Pts',(6.71211273967383,0.561308730497167,-8.04161829655868));
#58740=CARTESIAN_POINT('Ctrl Pts',(6.68079083609235,1.92043728607192,-8.08002239814288));
#58741=CARTESIAN_POINT('Ctrl Pts',(6.29786588949097,-2.16773371799523,-8.09674109067091));
#58742=CARTESIAN_POINT('Ctrl Pts',(6.29530177097099,-0.807935606154201,
-8.12958458865204));
#58743=CARTESIAN_POINT('Ctrl Pts',(6.29129857304258,0.551617246522031,-8.1627464890655));
#58744=CARTESIAN_POINT('Ctrl Pts',(6.2887344545226,1.91141535836306,-8.19558998704663));
#58745=CARTESIAN_POINT('Ctrl Pts',(5.00815621212858,-2.16216752644387,-8.38292053232245));
#58746=CARTESIAN_POINT('Ctrl Pts',(5.06969455888082,-0.803042657470201,
-8.40482373966323));
#58747=CARTESIAN_POINT('Ctrl Pts',(5.13036288577363,0.556263586031991,-8.42660503066042));
#58748=CARTESIAN_POINT('Ctrl Pts',(5.19190123252587,1.91538845500566,-8.4485082380012));
#58749=CARTESIAN_POINT('Ctrl Pts',(3.22852047111695,-2.04767166606362,-8.49451211875645));
#58750=CARTESIAN_POINT('Ctrl Pts',(3.33405646482314,-0.692138611224734,
-8.51233430927317));
#58751=CARTESIAN_POINT('Ctrl Pts',(3.44288808239679,0.663146437524625,-8.53025242833666));
#58752=CARTESIAN_POINT('Ctrl Pts',(3.54842407610298,2.01867949236351,-8.54807461885338));
#58753=CARTESIAN_POINT('Ctrl Pts',(1.19527622155365,-1.93132215124059,-8.55306594389669));
#58754=CARTESIAN_POINT('Ctrl Pts',(1.24356632046841,-0.571512548852095,
-8.56835748664852));
#58755=CARTESIAN_POINT('Ctrl Pts',(1.28271472812635,0.788613994112341,-8.58369978338118));
#58756=CARTESIAN_POINT('Ctrl Pts',(1.33100482704111,2.14842359650083,-8.598991326133));
#58757=CARTESIAN_POINT('Ctrl Pts',(6.41902973990636E-15,-1.93207323326078,
-8.62957429809281));
#58758=CARTESIAN_POINT('Ctrl Pts',(2.80278610805871E-15,-0.572138762410868,
-8.64292476603094));
#58759=CARTESIAN_POINT('Ctrl Pts',(-8.13457523788951E-16,0.787795708439045,
-8.65627523396906));
#58760=CARTESIAN_POINT('Ctrl Pts',(-4.42970115563661E-15,2.14773017928896,
-8.66962570190719));
#58761=CARTESIAN_POINT('Ctrl Pts',(77.5413122691233,9.45942207531684,-5.67964638243731));
#58762=CARTESIAN_POINT('Ctrl Pts',(77.0326085523511,10.7074362929352,-5.49721546081316));
#58763=CARTESIAN_POINT('Ctrl Pts',(76.5239048355788,11.9554505105535,-5.314784539189));
#58764=CARTESIAN_POINT('Ctrl Pts',(76.0152011188066,13.2034647281718,-5.13235361756485));
#58765=CARTESIAN_POINT('Ctrl Pts',(78.375913647818,9.63522559747283,-4.55505891458532));
#58766=CARTESIAN_POINT('Ctrl Pts',(77.8612559061973,10.8797481339151,-4.36483973542567));
#58767=CARTESIAN_POINT('Ctrl Pts',(77.3499789374201,12.1246925927886,-4.16959241162605));
#58768=CARTESIAN_POINT('Ctrl Pts',(76.8353211957994,13.3692151292309,-3.97937323246641));
#58769=CARTESIAN_POINT('Ctrl Pts',(79.119383339007,9.77540103482857,-3.21481989604027));
#58770=CARTESIAN_POINT('Ctrl Pts',(78.5708662074078,11.0105688473922,-3.05739091744627));
#58771=CARTESIAN_POINT('Ctrl Pts',(78.028068075148,12.247228353462,-2.89111167264609));
#58772=CARTESIAN_POINT('Ctrl Pts',(77.4795509435488,13.4823961660256,-2.73368269405209));
#58773=CARTESIAN_POINT('Ctrl Pts',(79.5980561168973,9.79488102600527,-1.92025417906537));
#58774=CARTESIAN_POINT('Ctrl Pts',(79.0286853722991,11.0149170322939,-1.72808472635512));
#58775=CARTESIAN_POINT('Ctrl Pts',(78.4593146277009,12.2349530385826,-1.53591527364488));
#58776=CARTESIAN_POINT('Ctrl Pts',(77.8899438831027,13.4549890448712,-1.34374582093463));
#58777=CARTESIAN_POINT('Ctrl Pts',(20.8093219165299,12.6047206302974,-78.8857217870086));
#58778=CARTESIAN_POINT('Ctrl Pts',(20.8084406388433,13.8055291044746,-78.2472405956695));
#58779=CARTESIAN_POINT('Ctrl Pts',(20.8075593611567,15.0063375786519,-77.6087594043304));
#58780=CARTESIAN_POINT('Ctrl Pts',(20.8066780834701,16.2071460528291,-76.9702782129913));
#58781=CARTESIAN_POINT('Ctrl Pts',(20.7840585070756,12.6878742959502,-79.0421459570682));
#58782=CARTESIAN_POINT('Ctrl Pts',(20.7831790034045,13.8886827711699,-78.4036647651749));
#58783=CARTESIAN_POINT('Ctrl Pts',(20.7822994476123,15.0894912462774,-77.7651835733411));
#58784=CARTESIAN_POINT('Ctrl Pts',(20.7814199439412,16.2902997214971,-77.1267023814477));
#58785=CARTESIAN_POINT('Ctrl Pts',(20.7537282342997,12.8597759562963,-79.3654873575285));
#58786=CARTESIAN_POINT('Ctrl Pts',(20.7528512698888,14.0605844328848,-78.7270061649073));
#58787=CARTESIAN_POINT('Ctrl Pts',(20.7519739839115,15.2613929097475,-78.0885249721403));
#58788=CARTESIAN_POINT('Ctrl Pts',(20.7510970195006,16.462201386336,-77.4500437795191));
#58789=CARTESIAN_POINT('Ctrl Pts',(20.8081933777383,13.1149063735043,-79.8452428571726));
#58790=CARTESIAN_POINT('Ctrl Pts',(20.8073117469505,14.3157148475504,-79.2067616659032));
#58791=CARTESIAN_POINT('Ctrl Pts',(20.8064299122934,15.5165233221614,-78.5682804743334));
#58792=CARTESIAN_POINT('Ctrl Pts',(20.8055482815057,16.7173317962075,-77.9297992830641));
#58793=CARTESIAN_POINT('Ctrl Pts',(21.0036168912534,13.3497532744261,-80.2866546117358));
#58794=CARTESIAN_POINT('Ctrl Pts',(21.0027239008197,14.5505617417736,-79.6481734240281));
#58795=CARTESIAN_POINT('Ctrl Pts',(21.0018296748422,15.7513702095747,-79.0096922360792));
#58796=CARTESIAN_POINT('Ctrl Pts',(21.0009366844085,16.9521786769222,-78.3712110483715));
#58797=CARTESIAN_POINT('Ctrl Pts',(21.2743902926592,13.4924836387241,-80.5547123821854));
#58798=CARTESIAN_POINT('Ctrl Pts',(21.273503030042,14.6932921096191,-79.9162311925915));
#58799=CARTESIAN_POINT('Ctrl Pts',(21.2726153038638,15.8941005812516,-79.2777500026055));
#58800=CARTESIAN_POINT('Ctrl Pts',(21.2717280412466,17.0949090521466,-78.6392688130115));
#58801=CARTESIAN_POINT('Ctrl Pts',(21.4904278237746,13.5660008548253,-80.6926839980435));
#58802=CARTESIAN_POINT('Ctrl Pts',(21.4895656787975,14.7668093397565,-80.0542028009863));
#58803=CARTESIAN_POINT('Ctrl Pts',(21.488702230328,15.9676178254005,-79.4157216035502));
#58804=CARTESIAN_POINT('Ctrl Pts',(21.4878400853508,17.1684263103318,-78.777240406493));
#58805=CARTESIAN_POINT('Ctrl Pts',(21.6433045087496,13.6103006059301,-80.7757949442799));
#58806=CARTESIAN_POINT('Ctrl Pts',(21.6424648381891,14.8111091037285,-80.1373137403811));
#58807=CARTESIAN_POINT('Ctrl Pts',(21.6416248265819,16.011917601909,-79.4988325362792));
#58808=CARTESIAN_POINT('Ctrl Pts',(21.6407851560214,17.2127260997074,-78.8603513323804));
#58809=CARTESIAN_POINT('Ctrl Pts',(21.928242214773,13.6734021326948,-80.8941044180776));
#58810=CARTESIAN_POINT('Ctrl Pts',(21.9274618395652,14.8742106613855,-80.2556231977532));
#58811=CARTESIAN_POINT('Ctrl Pts',(21.9266795141814,16.0750191913452,-79.6171419767539));
#58812=CARTESIAN_POINT('Ctrl Pts',(21.9258991389736,17.2758277200359,-78.9786607564294));
#58813=CARTESIAN_POINT('Ctrl Pts',(22.3613428584683,13.7286395353824,-80.997489165121));
#58814=CARTESIAN_POINT('Ctrl Pts',(22.3607015893129,14.9294481342844,-80.3590079074645));
#58815=CARTESIAN_POINT('Ctrl Pts',(22.3600607034172,16.1302567329206,-79.7205266499492));
#58816=CARTESIAN_POINT('Ctrl Pts',(22.3594194342618,17.3310653318226,-79.0820453922927));
#58817=CARTESIAN_POINT('Ctrl Pts',(22.9135127166986,13.7517748296916,-81.0405604775543));
#58818=CARTESIAN_POINT('Ctrl Pts',(22.9131468583814,14.9525835222783,-80.4020791700847));
#58819=CARTESIAN_POINT('Ctrl Pts',(22.9127804823919,16.1533922160744,-79.763597861972));
#58820=CARTESIAN_POINT('Ctrl Pts',(22.9124146240747,17.3542009086611,-79.1251165545024));
#58821=CARTESIAN_POINT('Ctrl Pts',(23.5417513911928,13.736769442166,-81.0121414409379));
#58822=CARTESIAN_POINT('Ctrl Pts',(23.5417933622192,14.9375781946617,-80.3736601016141));
#58823=CARTESIAN_POINT('Ctrl Pts',(23.5418352267392,16.138386947973,-79.7351787618567));
#58824=CARTESIAN_POINT('Ctrl Pts',(23.5418771977656,17.3391957004687,-79.0966974225329));
#58825=CARTESIAN_POINT('Ctrl Pts',(24.2730525164329,13.660545753115,-80.8691286744826));
#58826=CARTESIAN_POINT('Ctrl Pts',(24.273680519978,14.8613544010243,-80.2306473907684));
#58827=CARTESIAN_POINT('Ctrl Pts',(24.2743085928193,16.0621630471265,-79.5921661080151));
#58828=CARTESIAN_POINT('Ctrl Pts',(24.2749365963644,17.2629716950359,-78.9536848243009));
#58829=CARTESIAN_POINT('Ctrl Pts',(24.9170787624367,13.5062400436736,-80.579914018049));
#58830=CARTESIAN_POINT('Ctrl Pts',(24.9182622477484,14.7070483369479,-79.9414329228976));
#58831=CARTESIAN_POINT('Ctrl Pts',(24.9194463038521,15.9078566299141,-79.3029518279101));
#58832=CARTESIAN_POINT('Ctrl Pts',(24.9206297891638,17.1086649231884,-78.6644707327587));
#58833=CARTESIAN_POINT('Ctrl Pts',(25.3658123504925,13.2974001437394,-80.1881404327209));
#58834=CARTESIAN_POINT('Ctrl Pts',(25.3673554971624,14.4982081031418,-79.5496595150923));
#58835=CARTESIAN_POINT('Ctrl Pts',(25.368899272135,15.6990160619414,-78.9111785977844));
#58836=CARTESIAN_POINT('Ctrl Pts',(25.3704424188049,16.8998240213439,-78.2726976801559));
#58837=CARTESIAN_POINT('Ctrl Pts',(25.6155655213289,13.0717748423381,-79.7644556106849));
#58838=CARTESIAN_POINT('Ctrl Pts',(25.6172915372986,14.2725826029869,-79.1259747987356));
#58839=CARTESIAN_POINT('Ctrl Pts',(25.6190177037389,15.4733903636591,-78.4874939867739));
#58840=CARTESIAN_POINT('Ctrl Pts',(25.6207437197086,16.674198124308,-77.8490131748246));
#58841=CARTESIAN_POINT('Ctrl Pts',(25.6858818663905,12.9054712360564,-79.4518813295147));
#58842=CARTESIAN_POINT('Ctrl Pts',(25.687655531541,14.1062789411321,-78.8134005471141));
#58843=CARTESIAN_POINT('Ctrl Pts',(25.6894290078439,15.3070866465801,-78.1749197645157));
#58844=CARTESIAN_POINT('Ctrl Pts',(25.6912026729945,16.5078943516558,-77.5364389821151));
#58845=CARTESIAN_POINT('Ctrl Pts',(25.7013237933716,12.8213530409933,-79.2937211639668));
#58846=CARTESIAN_POINT('Ctrl Pts',(25.7031079311239,14.0221607339897,-78.6552403879889));
#58847=CARTESIAN_POINT('Ctrl Pts',(25.7048920688761,15.222968426986,-78.0167596120111));
#58848=CARTESIAN_POINT('Ctrl Pts',(25.7066762066284,16.4237761199824,-77.3782788360332));
#58849=CARTESIAN_POINT('',(20.808,14.4059333415632,-77.928));
#58850=CARTESIAN_POINT('Ctrl Pts',(21.0430574415837,12.442190173977,-78.5797217830346));
#58851=CARTESIAN_POINT('Ctrl Pts',(21.0421674979575,13.6429988456018,-77.9412404867108));
#58852=CARTESIAN_POINT('Ctrl Pts',(21.0412775543313,14.8438075172267,-77.3027591903869));
#58853=CARTESIAN_POINT('Ctrl Pts',(21.0403876107051,16.0446161888516,-76.664277894063));
#58854=CARTESIAN_POINT('Ctrl Pts',(20.9663933429453,12.4981850222955,-78.6851396340205));
#58855=CARTESIAN_POINT('Ctrl Pts',(20.9655036927131,13.6989936940884,-78.0466583376072));
#58856=CARTESIAN_POINT('Ctrl Pts',(20.9646140452926,14.8998023658873,-77.4081770411908));
#58857=CARTESIAN_POINT('Ctrl Pts',(20.9637243950605,16.1006110376802,-76.7696957447776));
#58858=CARTESIAN_POINT('Ctrl Pts',(20.8885043097157,12.5523824450204,-78.7871786835729));
#58859=CARTESIAN_POINT('Ctrl Pts',(20.887617525105,13.7531911184756,-78.1486973862758));
#58860=CARTESIAN_POINT('Ctrl Pts',(20.8867307434391,14.953999791937,-77.5102160889755));
#58861=CARTESIAN_POINT('Ctrl Pts',(20.8858439588284,16.1548084653921,-76.8717347916784));
#58862=CARTESIAN_POINT('Ctrl Pts',(20.8093219165299,12.6047206302974,-78.8857217870086));
#58863=CARTESIAN_POINT('Ctrl Pts',(20.8084406386947,13.8055293069047,-78.2472404880355));
#58864=CARTESIAN_POINT('Ctrl Pts',(20.8075593608596,15.0063379835122,-77.6087591890624));
#58865=CARTESIAN_POINT('Ctrl Pts',(20.8066780830244,16.2071466601195,-76.9702778900892));
#58866=CARTESIAN_POINT('Ctrl Pts',(-18.084171536322,0.0168069507424406,
-47.6825133195673));
#58867=CARTESIAN_POINT('Ctrl Pts',(-18.0828648825787,1.37310817598614,-47.5821760815471));
#58868=CARTESIAN_POINT('Ctrl Pts',(-18.0815581911822,2.72940939835026,-47.4818388069225));
#58869=CARTESIAN_POINT('Ctrl Pts',(-18.0802515374385,4.08571062359393,-47.3815015689019));
#58870=CARTESIAN_POINT('Ctrl Pts',(-17.506930629517,0.00163240881209737,
-47.4849099125784));
#58871=CARTESIAN_POINT('Ctrl Pts',(-17.5065137114848,1.35865940324804,-47.3943886329251));
#58872=CARTESIAN_POINT('Ctrl Pts',(-17.5071471183302,2.71576672268321,-47.3048884241277));
#58873=CARTESIAN_POINT('Ctrl Pts',(-17.506730212951,4.07279371808681,-47.2143671567752));
#58874=CARTESIAN_POINT('Ctrl Pts',(-16.1265953574943,-0.0239511115510788,
-47.0702290864536));
#58875=CARTESIAN_POINT('Ctrl Pts',(-16.132609651975,1.33467278918204,-47.0042231917552));
#58876=CARTESIAN_POINT('Ctrl Pts',(-16.1380915006763,2.69325718740651,-46.9377585627012));
#58877=CARTESIAN_POINT('Ctrl Pts',(-16.1441057887425,4.05188108766375,-46.8717526624765));
#58878=CARTESIAN_POINT('Ctrl Pts',(-14.10127225119,-0.0283229642908482,
-46.5960988598152));
#58879=CARTESIAN_POINT('Ctrl Pts',(-14.1075627501349,1.3313449215142,-46.5628949517334));
#58880=CARTESIAN_POINT('Ctrl Pts',(-14.1138926365074,2.69101592083309,-46.5296830060939));
#58881=CARTESIAN_POINT('Ctrl Pts',(-14.1201831359268,4.05068380667564,-46.4964790979153));
#58882=CARTESIAN_POINT('Ctrl Pts',(-12.7955484756759,-0.0284838878760417,
-46.3416616237862));
#58883=CARTESIAN_POINT('Ctrl Pts',(-12.7985366234782,1.33141633282946,-46.3244926843625));
#58884=CARTESIAN_POINT('Ctrl Pts',(-12.802000111894,2.69135191874657,-46.3078249592564));
#58885=CARTESIAN_POINT('Ctrl Pts',(-12.8049882654227,4.05125213987811,-46.2906560258708));
#58886=CARTESIAN_POINT('Ctrl Pts',(-11.470436949813,-0.0285771185290155,
-46.1028837411342));
#58887=CARTESIAN_POINT('Ctrl Pts',(-11.4702745894939,1.33147515866783,-46.1004393686973));
#58888=CARTESIAN_POINT('Ctrl Pts',(-11.4703724837302,2.69154460495323,-46.0980807984626));
#58889=CARTESIAN_POINT('Ctrl Pts',(-11.4702101265463,4.0515968823569,-46.0956364270593));
#58890=CARTESIAN_POINT('Ctrl Pts',(-9.98689553497245,-0.0298699386781541,
-45.8979097929726));
#58891=CARTESIAN_POINT('Ctrl Pts',(-9.98372271526217,1.3301121906159,-45.9055403357692));
#58892=CARTESIAN_POINT('Ctrl Pts',(-9.98085564305265,2.69011600325979,-45.9134768161035));
#58893=CARTESIAN_POINT('Ctrl Pts',(-9.97768282702567,4.05009813281506,-45.9211073625856));
#58894=CARTESIAN_POINT('Ctrl Pts',(-8.14237944721806,-0.0324247744844724,
-45.7230625805931));
#58895=CARTESIAN_POINT('Ctrl Pts',(-8.13997400378338,1.32751302340312,-45.7374232436365));
#58896=CARTESIAN_POINT('Ctrl Pts',(-8.1376557237031,2.68745306043262,-45.7518461445845));
#58897=CARTESIAN_POINT('Ctrl Pts',(-8.13525028131847,4.04739085834718,-45.7662068083777));
#58898=CARTESIAN_POINT('Ctrl Pts',(-6.87097468423606,-0.0328533238228722,
-45.6419015366938));
#58899=CARTESIAN_POINT('Ctrl Pts',(-6.87002039103409,1.32705155847938,-45.658581401155));
#58900=CARTESIAN_POINT('Ctrl Pts',(-6.86920619802231,2.6869629011669,-45.6753523082089));
#58901=CARTESIAN_POINT('Ctrl Pts',(-6.8682519065081,4.04686778354698,-45.692032173767));
#58902=CARTESIAN_POINT('Ctrl Pts',(-5.13083769090565,-0.0319736651072693,
-45.5581580996358));
#58903=CARTESIAN_POINT('Ctrl Pts',(-5.1319190187102,1.32790705483533,-45.5768752722455));
#58904=CARTESIAN_POINT('Ctrl Pts',(-5.1330666952011,2.68779052666114,-45.5956441954884));
#58905=CARTESIAN_POINT('Ctrl Pts',(-5.13414802380493,4.04767124663689,-45.6143613687216));
#58906=CARTESIAN_POINT('Ctrl Pts',(-2.82311055870927,-0.0277859137287846,
-45.4820465344085));
#58907=CARTESIAN_POINT('Ctrl Pts',(-2.82542111997424,1.33207058630606,-45.5021622318001));
#58908=CARTESIAN_POINT('Ctrl Pts',(-2.82765880245458,2.69193303472359,-45.5223443526086));
#58909=CARTESIAN_POINT('Ctrl Pts',(-2.8299693628416,4.0517895348301,-45.5424600508003));
#58910=CARTESIAN_POINT('Ctrl Pts',(-0.827876248095319,-0.0254184256084418,
-45.4363857618409));
#58911=CARTESIAN_POINT('Ctrl Pts',(-0.828401955565921,1.33442934851277,
-45.4573391307405));
#58912=CARTESIAN_POINT('Ctrl Pts',(-0.829171501015099,2.69427440248123,
-45.4782808761721));
#58913=CARTESIAN_POINT('Ctrl Pts',(-0.829697211423176,4.05412217656967,
-45.4992342449317));
#58914=CARTESIAN_POINT('Ctrl Pts',(2.96793475906394E-5,-0.0251511567891935,
-45.4192962601408));
#58915=CARTESIAN_POINT('Ctrl Pts',(2.96981943129004E-5,1.33469071903223,
-45.4405648948134));
#58916=CARTESIAN_POINT('Ctrl Pts',(2.97257824282988E-5,2.69453259495117,
-45.4618335299028));
#58917=CARTESIAN_POINT('Ctrl Pts',(2.97446292558659E-5,4.05437447077259,
-45.4831021645754));
#58918=CARTESIAN_POINT('Ctrl Pts',(-25.7013237899579,12.8213507429086,-79.29372238588));
#58919=CARTESIAN_POINT('Ctrl Pts',(-25.7020884215611,13.3359833773638,-79.0200873602994));
#58920=CARTESIAN_POINT('Ctrl Pts',(-25.703872560451,14.5367918363885,-78.3816061770171));
#58921=CARTESIAN_POINT('Ctrl Pts',(-25.7056566993409,15.737600295413,-77.7431249937349));
#58922=CARTESIAN_POINT('Ctrl Pts',(-25.7066762066276,16.4237761199824,-77.3782788360333));
#58923=CARTESIAN_POINT('Ctrl Pts',(-25.6858655966018,12.9055575473563,-79.4520491559888));
#58924=CARTESIAN_POINT('Ctrl Pts',(-25.6866261120234,13.4201901873017,-79.178414127489));
#58925=CARTESIAN_POINT('Ctrl Pts',(-25.6883996507926,14.620998658509,-78.5399329377291));
#58926=CARTESIAN_POINT('Ctrl Pts',(-25.6901723542552,15.8218071291893,-77.9014517482493));
#58927=CARTESIAN_POINT('Ctrl Pts',(-25.6911863733062,16.507982961079,-77.5366055866555));
#58928=CARTESIAN_POINT('Ctrl Pts',(-25.6167632558673,13.0699277926588,-79.7609931774108));
#58929=CARTESIAN_POINT('Ctrl Pts',(-25.6175025156277,13.5845604555093,-79.4873581367321));
#58930=CARTESIAN_POINT('Ctrl Pts',(-25.6192286397047,14.7853689809119,-78.8488769181561));
#58931=CARTESIAN_POINT('Ctrl Pts',(-25.6209557588151,15.9861775064173,-78.2103956995253));
#58932=CARTESIAN_POINT('Ctrl Pts',(-25.6219414370306,16.672353368847,-77.845549521693));
#58933=CARTESIAN_POINT('Ctrl Pts',(-25.2826927947797,13.3728687263107,-80.3298613001038));
#58934=CARTESIAN_POINT('Ctrl Pts',(-25.283329806226,13.887501503606,-80.0562261985736));
#58935=CARTESIAN_POINT('Ctrl Pts',(-25.2848135698082,15.0883102951698,-79.4177448384771));
#58936=CARTESIAN_POINT('Ctrl Pts',(-25.2862951562559,16.2891190861009,-78.7792634787171));
#58937=CARTESIAN_POINT('Ctrl Pts',(-25.2871445035823,16.9752951011235,-78.4144172197497));
#58938=CARTESIAN_POINT('Ctrl Pts',(-24.6852313330219,13.5767391583647,-80.7120457511261));
#58939=CARTESIAN_POINT('Ctrl Pts',(-24.6856528650133,14.0913721211625,-80.4384105509626));
#58940=CARTESIAN_POINT('Ctrl Pts',(-24.6866372266374,15.2921813464143,-79.7999289602702));
#58941=CARTESIAN_POINT('Ctrl Pts',(-24.6876222491661,16.4929905717456,-79.1614473695355));
#58942=CARTESIAN_POINT('Ctrl Pts',(-24.6881842909862,17.1791668341045,-78.7966009790571));
#58943=CARTESIAN_POINT('Ctrl Pts',(-24.0040551378999,13.6893795635206,-80.9232212941775));
#58944=CARTESIAN_POINT('Ctrl Pts',(-24.004230358018,14.2040126262127,-80.6495860408992));
#58945=CARTESIAN_POINT('Ctrl Pts',(-24.004639900488,15.4048220842307,-80.0111043264428));
#58946=CARTESIAN_POINT('Ctrl Pts',(-24.0050500267346,16.6056315420595,-79.372622612087));
#58947=CARTESIAN_POINT('Ctrl Pts',(-24.0052836532123,17.2918079376106,-79.007776150789));
#58948=CARTESIAN_POINT('Ctrl Pts',(-23.4548778566481,13.7384359365402,-81.0153105837569));
#58949=CARTESIAN_POINT('Ctrl Pts',(-23.4548724406338,14.253069021085,-80.7416753188595));
#58950=CARTESIAN_POINT('Ctrl Pts',(-23.4548599684916,15.4538785303795,-80.1031935771389));
#58951=CARTESIAN_POINT('Ctrl Pts',(-23.4548476349486,16.654688039726,-79.4647118353906));
#58952=CARTESIAN_POINT('Ctrl Pts',(-23.4548404136072,17.3408644644138,-79.0998653586004));
#58953=CARTESIAN_POINT('Ctrl Pts',(-22.9164771617764,13.7513551462076,-81.0397745016549));
#58954=CARTESIAN_POINT('Ctrl Pts',(-22.9163209973395,14.2659882094511,-80.7661392480834));
#58955=CARTESIAN_POINT('Ctrl Pts',(-22.9159572365429,15.4667976692766,-80.127657532666));
#58956=CARTESIAN_POINT('Ctrl Pts',(-22.9155939980342,16.6676071293499,-79.4891758171168));
#58957=CARTESIAN_POINT('Ctrl Pts',(-22.915385779096,17.3537835256363,-79.1243293554279));
#58958=CARTESIAN_POINT('Ctrl Pts',(-22.4549655367611,13.7323867778409,-81.0044664289556));
#58959=CARTESIAN_POINT('Ctrl Pts',(-22.4547109103277,14.2470198074144,-80.7308311932868));
#58960=CARTESIAN_POINT('Ctrl Pts',(-22.4541168974148,15.447829188375,-80.0923495198026));
#58961=CARTESIAN_POINT('Ctrl Pts',(-22.4535229809148,16.6486385693303,-79.4538678463211));
#58962=CARTESIAN_POINT('Ctrl Pts',(-22.453183479509,17.3348149207234,-79.0890214085024));
#58963=CARTESIAN_POINT('Ctrl Pts',(-22.1430512368791,13.6992998972659,-80.9425723760123));
#58964=CARTESIAN_POINT('Ctrl Pts',(-22.1427473388653,14.2139329047488,-80.6689371520894));
#58965=CARTESIAN_POINT('Ctrl Pts',(-22.1420384096197,15.4147422343653,-80.0304555059053));
#58966=CARTESIAN_POINT('Ctrl Pts',(-22.1413296192275,16.6155515641451,-79.3919738596343));
#58967=CARTESIAN_POINT('Ctrl Pts',(-22.1409244224793,17.3017278860839,-79.0271274374767));
#58968=CARTESIAN_POINT('Ctrl Pts',(-21.9706189386793,13.6744394516519,-80.8960170933706));
#58969=CARTESIAN_POINT('Ctrl Pts',(-21.9702923495131,14.1890724482461,-80.6223818752372));
#58970=CARTESIAN_POINT('Ctrl Pts',(-21.9695304663557,15.3898817523233,-79.9839002426326));
#58971=CARTESIAN_POINT('Ctrl Pts',(-21.9687687153957,16.5906910564529,-79.3454186100002));
#58972=CARTESIAN_POINT('Ctrl Pts',(-21.9683332638225,17.2768673638735,-78.980572195562));
#58973=CARTESIAN_POINT('Ctrl Pts',(-21.8446726909401,13.6525925417021,-80.8550829230538));
#58974=CARTESIAN_POINT('Ctrl Pts',(-21.844331772734,14.1672255309889,-80.5814477088058));
#58975=CARTESIAN_POINT('Ctrl Pts',(-21.8435364464263,15.3680348180929,-79.942966085226));
#58976=CARTESIAN_POINT('Ctrl Pts',(-21.8427412449731,16.5688441053144,-79.3044844615836));
#58977=CARTESIAN_POINT('Ctrl Pts',(-21.842286688042,17.2550204029918,-78.9396380523261));
#58978=CARTESIAN_POINT('Ctrl Pts',(-21.721746177194,13.6272172866624,-80.8075149514255));
#58979=CARTESIAN_POINT('Ctrl Pts',(-21.7213933708601,14.1418502697189,-80.5338797404902));
#58980=CARTESIAN_POINT('Ctrl Pts',(-21.7205703008806,15.3426595422183,-79.8953981246758));
#58981=CARTESIAN_POINT('Ctrl Pts',(-21.7197473517875,16.5434688147785,-79.2569165088291));
#58982=CARTESIAN_POINT('Ctrl Pts',(-21.7192769440428,17.2296451041489,-78.8920701039884));
#58983=CARTESIAN_POINT('Ctrl Pts',(-21.6228148027256,13.6030088775296,-80.7621149641663));
#58984=CARTESIAN_POINT('Ctrl Pts',(-21.6224540937013,14.1176418562761,-80.4884797555227));
#58985=CARTESIAN_POINT('Ctrl Pts',(-21.6216125658996,15.318451118753,-79.8499981450373));
#58986=CARTESIAN_POINT('Ctrl Pts',(-21.6207711436935,16.5192603813193,-79.2115165345044));
#58987=CARTESIAN_POINT('Ctrl Pts',(-21.6202901990439,17.2054366649431,-78.8466701327192));
#58988=CARTESIAN_POINT('Ctrl Pts',(-21.5604515982842,13.5856860066143,-80.7296183597009));
#58989=CARTESIAN_POINT('Ctrl Pts',(-21.5600866332627,14.1003189830252,-80.4559831522991));
#58990=CARTESIAN_POINT('Ctrl Pts',(-21.5592351816853,15.3011282400274,-79.8175015447247));
#58991=CARTESIAN_POINT('Ctrl Pts',(-21.5583838414717,16.501937497098,-79.1790199371138));
#58992=CARTESIAN_POINT('Ctrl Pts',(-21.5578972221677,17.1881137776076,-78.8141735369845));
#58993=CARTESIAN_POINT('Ctrl Pts',(-21.5226324038841,13.574613873599,-80.7088453355964));
#58994=CARTESIAN_POINT('Ctrl Pts',(-21.5222650446281,14.0892468486761,-80.4352101289038));
#58995=CARTESIAN_POINT('Ctrl Pts',(-21.521408000631,15.2900561025754,-79.7967285229793));
#58996=CARTESIAN_POINT('Ctrl Pts',(-21.5205510630675,16.4908653565509,-79.1582469170141));
#58997=CARTESIAN_POINT('Ctrl Pts',(-21.5200612514553,17.1770416352821,-78.7934005178304));
#58998=CARTESIAN_POINT('Ctrl Pts',(-21.4945991349715,13.5660570588058,-80.6927900206057));
#58999=CARTESIAN_POINT('Ctrl Pts',(-21.4942301067783,14.0806900329552,-80.4191548144064));
#59000=CARTESIAN_POINT('Ctrl Pts',(-21.4933691690818,15.2814992846826,-79.7806732096367));
#59001=CARTESIAN_POINT('Ctrl Pts',(-21.4925083382252,16.4823085364802,-79.1421916048296));
#59002=CARTESIAN_POINT('Ctrl Pts',(-21.4920163013668,17.1684848139744,-78.7773452063036));
#59003=CARTESIAN_POINT('Ctrl Pts',(-21.4624099987218,13.5557020135771,-80.6733585467387));
#59004=CARTESIAN_POINT('Ctrl Pts',(-21.4620392051584,14.0703349867346,-80.3997233410669));
#59005=CARTESIAN_POINT('Ctrl Pts',(-21.4611741483302,15.271144236153,-79.7612417375249));
#59006=CARTESIAN_POINT('Ctrl Pts',(-21.4603091983932,16.4719534856458,-79.1227601339433));
#59007=CARTESIAN_POINT('Ctrl Pts',(-21.4598148077115,17.1581297618176,-78.7579137361204));
#59008=CARTESIAN_POINT('Ctrl Pts',(-21.435185616044,13.5465681568376,-80.6562172227997));
#59009=CARTESIAN_POINT('Ctrl Pts',(-21.4348134318159,14.0612011292143,-80.3825820175431));
#59010=CARTESIAN_POINT('Ctrl Pts',(-21.4339451256095,15.2620103768036,-79.7441004149736));
#59011=CARTESIAN_POINT('Ctrl Pts',(-21.4330769225221,16.4628196244617,-79.1056188123675));
#59012=CARTESIAN_POINT('Ctrl Pts',(-21.4325806776235,17.1489958995923,-78.7407724150982));
#59013=CARTESIAN_POINT('Ctrl Pts',(-21.412809848635,13.5387370119342,-80.6415194725682));
#59014=CARTESIAN_POINT('Ctrl Pts',(-21.4124365976858,14.0533699837061,-80.367884267633));
#59015=CARTESIAN_POINT('Ctrl Pts',(-21.4115658102438,15.254179229894,-79.7294026658087));
#59016=CARTESIAN_POINT('Ctrl Pts',(-21.4106951324464,16.4549884761586,-79.0909210639435));
#59017=CARTESIAN_POINT('Ctrl Pts',(-21.410197465255,17.1411647504829,-78.726074667103));
#59018=CARTESIAN_POINT('Ctrl Pts',(-21.3951093791352,13.5323422126205,-80.6295167784899));
#59019=CARTESIAN_POINT('Ctrl Pts',(-21.3947353396864,14.0469751839487,-80.3558815737907));
#59020=CARTESIAN_POINT('Ctrl Pts',(-21.393862699644,15.2477844290876,-79.7173999725242));
#59021=CARTESIAN_POINT('Ctrl Pts',(-21.3929901585335,16.4485936742919,-79.0789183712227));
#59022=CARTESIAN_POINT('Ctrl Pts',(-21.392491440011,17.1347699480245,-78.7140719746968));
#59023=CARTESIAN_POINT('Ctrl Pts',(-21.2456739047379,13.4771896612147,-80.5259944040367));
#59024=CARTESIAN_POINT('Ctrl Pts',(-21.2452933752653,13.9918226288365,-80.2523592013081));
#59025=CARTESIAN_POINT('Ctrl Pts',(-21.2444057029843,15.1926318654482,-79.6138776045755));
#59026=CARTESIAN_POINT('Ctrl Pts',(-21.2435182228696,16.3934411022267,-78.9753960077542));
#59027=CARTESIAN_POINT('Ctrl Pts',(-21.2430108509951,17.0796173710175,-78.6105496138558));
#59028=CARTESIAN_POINT('Ctrl Pts',(-21.0039921951822,13.3500335523429,-80.2871869099115));
#59029=CARTESIAN_POINT('Ctrl Pts',(-21.0036094681115,13.8646665186922,-80.0135517078596));
#59030=CARTESIAN_POINT('Ctrl Pts',(-21.0027164067956,15.0654757521404,-79.3750701128091));
#59031=CARTESIAN_POINT('Ctrl Pts',(-21.0018233184298,16.2662849855924,-78.7365885177565));
#59032=CARTESIAN_POINT('Ctrl Pts',(-21.0013130164285,16.9524612526866,-78.3717421247602));
#59033=CARTESIAN_POINT('Ctrl Pts',(-20.7414740910803,13.032826850117,-79.6909716241468));
#59034=CARTESIAN_POINT('Ctrl Pts',(-20.7410979762074,13.5474598202787,-79.4173364200678));
#59035=CARTESIAN_POINT('Ctrl Pts',(-20.7402205762101,14.7482690627728,-78.7788548202075));
#59036=CARTESIAN_POINT('Ctrl Pts',(-20.7393433445201,15.9490783053969,-78.140373220278));
#59037=CARTESIAN_POINT('Ctrl Pts',(-20.7388418587697,16.6352545775742,-77.7755268245789));
#59038=CARTESIAN_POINT('Ctrl Pts',(-20.7586989978057,12.7713419783598,-79.1991663833854));
#59039=CARTESIAN_POINT('Ctrl Pts',(-20.7583231666064,13.2859749486613,-78.9255311792321));
#59040=CARTESIAN_POINT('Ctrl Pts',(-20.7574453618225,14.4867841908561,-78.2870495795309));
#59041=CARTESIAN_POINT('Ctrl Pts',(-20.7565668304884,15.6875934326558,-77.6485679800397));
#59042=CARTESIAN_POINT('Ctrl Pts',(-20.7560657229672,16.3737697050196,-77.2837215842416));
#59043=CARTESIAN_POINT('Ctrl Pts',(-20.8093219182155,12.6047183322107,-78.8857230089227));
#59044=CARTESIAN_POINT('Ctrl Pts',(-20.8089442272165,13.1193513014583,-78.6120878053298));
#59045=CARTESIAN_POINT('Ctrl Pts',(-20.8080629489683,14.3201605416643,-77.9736062066861));
#59046=CARTESIAN_POINT('Ctrl Pts',(-20.8071816707202,15.5209697818703,-77.3351246080423));
#59047=CARTESIAN_POINT('Ctrl Pts',(-20.8066780834711,16.2071460528287,-76.9702782129914));
#59048=CARTESIAN_POINT('',(-25.704,14.6225645804878,-78.336));
#59049=CARTESIAN_POINT('Ctrl Pts',(-25.9521939365424,12.4413225404486,-78.5797210091185));
#59050=CARTESIAN_POINT('Ctrl Pts',(-25.9541384795005,13.6421300392938,-77.9412403363727));
#59051=CARTESIAN_POINT('Ctrl Pts',(-25.9560830224586,14.8429375381389,-77.3027596636269));
#59052=CARTESIAN_POINT('Ctrl Pts',(-25.9580275654167,16.0437450369841,-76.6642789908811));
#59053=CARTESIAN_POINT('Ctrl Pts',(-25.8694498071432,12.5700415836659,-78.8215543165566));
#59054=CARTESIAN_POINT('Ctrl Pts',(-25.8713452879931,13.7708491444509,-78.1830736108767));
#59055=CARTESIAN_POINT('Ctrl Pts',(-25.8732407643774,14.9716567052373,-77.5445929051962));
#59056=CARTESIAN_POINT('Ctrl Pts',(-25.8751362452272,16.1724642660223,-76.9061121995164));
#59057=CARTESIAN_POINT('Ctrl Pts',(-25.7857936084007,12.6969907473229,-79.0600657450643));
#59058=CARTESIAN_POINT('Ctrl Pts',(-25.7876353781899,13.8977983735652,-78.4215850045802));
#59059=CARTESIAN_POINT('Ctrl Pts',(-25.7894771453224,15.0986059998054,-77.7831042640973));
#59060=CARTESIAN_POINT('Ctrl Pts',(-25.7913189151116,16.2994136260477,-77.1446235236132));
#59061=CARTESIAN_POINT('Ctrl Pts',(-25.7013237933724,12.8213530409933,-79.2937211639668));
#59062=CARTESIAN_POINT('Ctrl Pts',(-25.7031079311241,14.0221607339896,-78.6552403879889));
#59063=CARTESIAN_POINT('Ctrl Pts',(-25.7048920688759,15.222968426986,-78.0167596120111));
#59064=CARTESIAN_POINT('Ctrl Pts',(-25.7066762066276,16.4237761199824,-77.3782788360333));
#99993=UNCERTAINTY_MEASURE_WITH_UNIT(LENGTH_MEASURE(0.01),#100032,
'DISTANCE_ACCURACY_VALUE',
'Maximum model space distance between geometric entities at asserted c
onnectivities');
#100011=UNCERTAINTY_MEASURE_WITH_UNIT(LENGTH_MEASURE(0.01),#100032,
'DISTANCE_ACCURACY_VALUE',
'Maximum model space distance between geometric entities at asserted c
onnectivities');
#100013=(
GEOMETRIC_REPRESENTATION_CONTEXT(3)
GLOBAL_UNCERTAINTY_ASSIGNED_CONTEXT((#99993))
GLOBAL_UNIT_ASSIGNED_CONTEXT((#100032,#100034,#100035))
REPRESENTATION_CONTEXT('','3D')
);
#100031=(
GEOMETRIC_REPRESENTATION_CONTEXT(3)
GLOBAL_UNCERTAINTY_ASSIGNED_CONTEXT((#100011))
GLOBAL_UNIT_ASSIGNED_CONTEXT((#100032,#100034,#100035))
REPRESENTATION_CONTEXT('','3D')
);
#100032=(
LENGTH_UNIT()
NAMED_UNIT(*)
SI_UNIT(.MILLI.,.METRE.)
);
#100034=(
NAMED_UNIT(*)
PLANE_ANGLE_UNIT()
SI_UNIT($,.RADIAN.)
);
#100035=(
NAMED_UNIT(*)
SI_UNIT($,.STERADIAN.)
SOLID_ANGLE_UNIT()
);
#100037=SHAPE_DEFINITION_REPRESENTATION(#100056,#100101);
#100056=PRODUCT_DEFINITION_SHAPE('',$,#100121);
#100101=SHAPE_REPRESENTATION('',(#20335),#100013);
#100119=PRODUCT_DEFINITION_CONTEXT('part definition',#100178,'design');
#100121=PRODUCT_DEFINITION('2026-10-12-11-54-00-493',
'01_Release_Fork_Lever_Fork-A',#100140,#100119);
#100140=PRODUCT_DEFINITION_FORMATION('',$,#100181);
#100178=APPLICATION_CONTEXT(
'Core Data for Automotive Mechanical Design Process');
#100179=PRODUCT_CONTEXT('part definition',#100178,'mechanical');
#100181=PRODUCT('2026-10-12-11-54-00-493',
'01_Release_Fork_Lever_Fork-A',$,(#100179));
#100200=PRESENTATION_STYLE_ASSIGNMENT((#100206));
#100206=SURFACE_STYLE_USAGE(.BOTH.,#100212);
#100212=SURFACE_SIDE_STYLE('',(#100218));
#100218=SURFACE_STYLE_FILL_AREA(#100224);
#100224=FILL_AREA_STYLE('Opaque(227,224,212)',(#100230));
#100230=FILL_AREA_STYLE_COLOUR('Opaque(227,224,212)',#100236);
#100236=COLOUR_RGB('Opaque(227,224,212)',0.890196078431372,0.87843137254902,
0.831372549019608);
ENDSEC;
END-ISO-10303-21;
